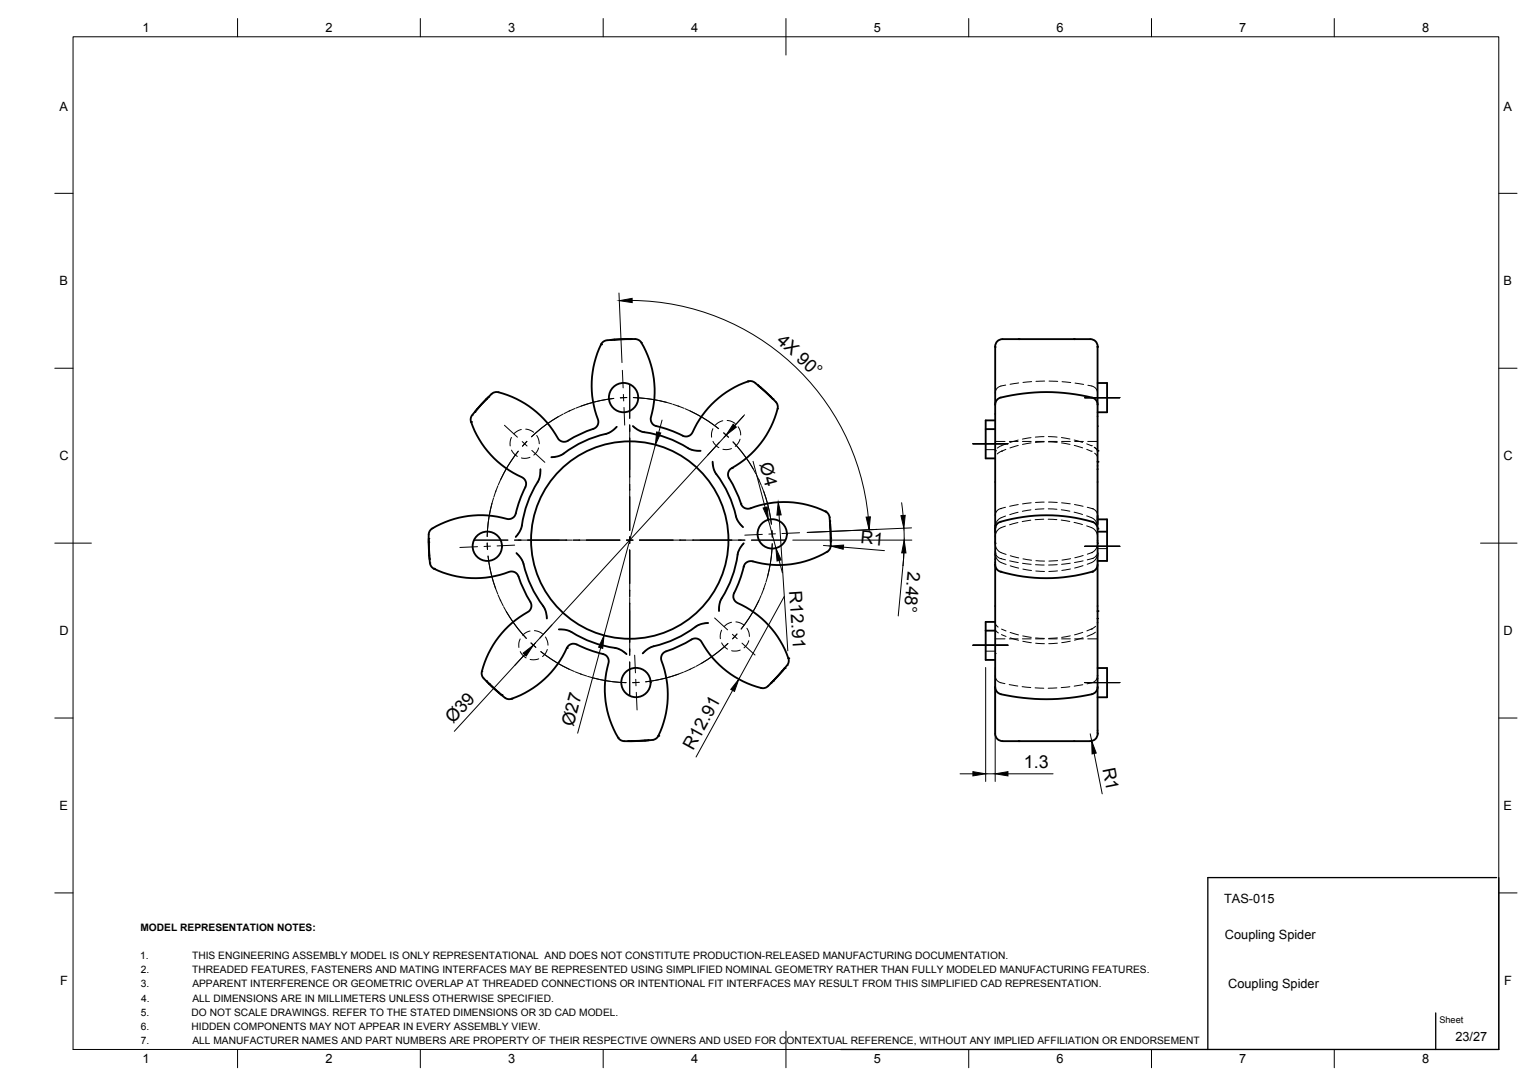
ISO-10303-21;
HEADER;
/* Generated by software containing ST-Developer
 * from STEP Tools, Inc. (www.steptools.com) 
 */

FILE_DESCRIPTION(
/* description */ ('STEP AP214'),
/* implementation_level */ '2;1');

FILE_NAME(
/* name */ 'Coupling Spider.step',
/* time_stamp */ '2026-11-15T14:49:54-08:00',
/* author */ (''),
/* organization */ (''),
/* preprocessor_version */ 'ST-DEVELOPER v20.2',
/* originating_system */ 'Autodesk Translation Framework v15.17.0.0',
/* authorisation */ '');

FILE_SCHEMA (('AUTOMOTIVE_DESIGN { 1 0 10303 214 3 1 1 }'));
ENDSEC;

DATA;
#10=MECHANICAL_DESIGN_GEOMETRIC_PRESENTATION_REPRESENTATION('',(#1115),#66721);
#11=B_SPLINE_SURFACE_WITH_KNOTS('',3,3,((#41982,#41983,#41984,#41985,#41986),
(#41987,#41988,#41989,#41990,#41991),(#41992,#41993,#41994,#41995,#41996),
(#41997,#41998,#41999,#42000,#42001),(#42002,#42003,#42004,#42005,#42006),
(#42007,#42008,#42009,#42010,#42011),(#42012,#42013,#42014,#42015,#42016)),
 .UNSPECIFIED.,.F.,.F.,.F.,(4,1,1,1,4),(4,1,4),(0.02704890409976,0.25,0.5,
0.75,0.9277040914243),(0.6266253876044,7.194455259721,13.76279800701),
 .UNSPECIFIED.);
#12=B_SPLINE_SURFACE_WITH_KNOTS('',3,3,((#43036,#43037,#43038,#43039,#43040),
(#43041,#43042,#43043,#43044,#43045),(#43046,#43047,#43048,#43049,#43050),
(#43051,#43052,#43053,#43054,#43055)),.UNSPECIFIED.,.F.,.F.,.F.,(4,4),(4,
1,4),(0.07560247213886,0.9246170074165),(0.97123707704753,7.194455259721,
13.4176757847934),.UNSPECIFIED.);
#13=B_SPLINE_SURFACE_WITH_KNOTS('',3,3,((#43854,#43855,#43856,#43857,#43858),
(#43859,#43860,#43861,#43862,#43863),(#43864,#43865,#43866,#43867,#43868),
(#43869,#43870,#43871,#43872,#43873),(#43874,#43875,#43876,#43877,#43878),
(#43879,#43880,#43881,#43882,#43883),(#43884,#43885,#43886,#43887,#43888)),
 .UNSPECIFIED.,.F.,.F.,.F.,(4,1,1,1,4),(4,1,4),(0.07229619653719,0.25,0.5,
0.75,0.9729510902578),(0.6266257504199,7.194455259721,13.76275812373),
 .UNSPECIFIED.);
#14=B_SPLINE_SURFACE_WITH_KNOTS('',3,3,((#44879,#44880,#44881,#44882,#44883),
(#44884,#44885,#44886,#44887,#44888),(#44889,#44890,#44891,#44892,#44893),
(#44894,#44895,#44896,#44897,#44898),(#44899,#44900,#44901,#44902,#44903),
(#44904,#44905,#44906,#44907,#44908),(#44909,#44910,#44911,#44912,#44913)),
 .UNSPECIFIED.,.F.,.F.,.F.,(4,1,1,1,4),(4,1,4),(0.02704960022791,0.25,0.5,
0.75,0.9276685882704),(0.6266253876465,7.194455259721,13.76279800699),
 .UNSPECIFIED.);
#15=B_SPLINE_SURFACE_WITH_KNOTS('',3,3,((#45852,#45853,#45854,#45855,#45856),
(#45857,#45858,#45859,#45860,#45861),(#45862,#45863,#45864,#45865,#45866),
(#45867,#45868,#45869,#45870,#45871)),.UNSPECIFIED.,.F.,.F.,.F.,(4,4),(4,
1,4),(0.07560247213886,0.9246170074164),(0.971237077045854,7.194455259721,
13.4176757847952),.UNSPECIFIED.);
#16=B_SPLINE_SURFACE_WITH_KNOTS('',3,3,((#46672,#46673,#46674,#46675,#46676),
(#46677,#46678,#46679,#46680,#46681),(#46682,#46683,#46684,#46685,#46686),
(#46687,#46688,#46689,#46690,#46691),(#46692,#46693,#46694,#46695,#46696),
(#46697,#46698,#46699,#46700,#46701),(#46702,#46703,#46704,#46705,#46706)),
 .UNSPECIFIED.,.F.,.F.,.F.,(4,1,1,1,4),(4,1,4),(0.07233141172687,0.25,0.5,
0.75,0.972950399776),(0.6266257504498,7.194455259721,13.76275812375),
 .UNSPECIFIED.);
#17=B_SPLINE_SURFACE_WITH_KNOTS('',3,3,((#47663,#47664,#47665,#47666,#47667),
(#47668,#47669,#47670,#47671,#47672),(#47673,#47674,#47675,#47676,#47677),
(#47678,#47679,#47680,#47681,#47682),(#47683,#47684,#47685,#47686,#47687),
(#47688,#47689,#47690,#47691,#47692),(#47693,#47694,#47695,#47696,#47697)),
 .UNSPECIFIED.,.F.,.F.,.F.,(4,1,1,1,4),(4,1,4),(0.02704894056375,0.25,0.5,
0.75,0.9277022317281),(0.6266253876037,7.194455259721,13.76279800701),
 .UNSPECIFIED.);
#18=B_SPLINE_SURFACE_WITH_KNOTS('',3,3,((#48705,#48706,#48707,#48708,#48709),
(#48710,#48711,#48712,#48713,#48714),(#48715,#48716,#48717,#48718,#48719),
(#48720,#48721,#48722,#48723,#48724)),.UNSPECIFIED.,.F.,.F.,.F.,(4,4),(4,
1,4),(0.07561105541477,0.9246169072522),(0.971199375698935,7.194455259721,
13.4177134902227),.UNSPECIFIED.);
#19=B_SPLINE_SURFACE_WITH_KNOTS('',3,3,((#49555,#49556,#49557,#49558,#49559),
(#49560,#49561,#49562,#49563,#49564),(#49565,#49566,#49567,#49568,#49569),
(#49570,#49571,#49572,#49573,#49574),(#49575,#49576,#49577,#49578,#49579),
(#49580,#49581,#49582,#49583,#49584),(#49585,#49586,#49587,#49588,#49589)),
 .UNSPECIFIED.,.F.,.F.,.F.,(4,1,1,1,4),(4,1,4),(0.07233141172959,0.25,0.5,
0.75,0.9729503997759),(0.6266257504616,7.194455259721,13.76275812376),
 .UNSPECIFIED.);
#20=B_SPLINE_SURFACE_WITH_KNOTS('',3,3,((#50503,#50504,#50505,#50506,#50507),
(#50508,#50509,#50510,#50511,#50512),(#50513,#50514,#50515,#50516,#50517),
(#50518,#50519,#50520,#50521,#50522),(#50523,#50524,#50525,#50526,#50527),
(#50528,#50529,#50530,#50531,#50532),(#50533,#50534,#50535,#50536,#50537)),
 .UNSPECIFIED.,.F.,.F.,.F.,(4,1,1,1,4),(4,1,4),(0.0270489040004,0.25,0.5,
0.75,0.9277040964915),(0.6266253875094,7.194455259721,13.76279800735),
 .UNSPECIFIED.);
#21=B_SPLINE_SURFACE_WITH_KNOTS('',3,3,((#51508,#51509,#51510,#51511,#51512),
(#51513,#51514,#51515,#51516,#51517),(#51518,#51519,#51520,#51521,#51522),
(#51523,#51524,#51525,#51526,#51527)),.UNSPECIFIED.,.F.,.F.,.F.,(4,4),(4,
1,4),(0.07561105541523,0.9246169072518),(0.971199375716696,7.194455259721,
13.4177134861273),.UNSPECIFIED.);
#22=B_SPLINE_SURFACE_WITH_KNOTS('',3,3,((#52356,#52357,#52358,#52359,#52360),
(#52361,#52362,#52363,#52364,#52365),(#52366,#52367,#52368,#52369,#52370),
(#52371,#52372,#52373,#52374,#52375),(#52376,#52377,#52378,#52379,#52380),
(#52381,#52382,#52383,#52384,#52385),(#52386,#52387,#52388,#52389,#52390)),
 .UNSPECIFIED.,.F.,.F.,.F.,(4,1,1,1,4),(4,1,4),(0.07229571648343,0.25,0.5,
0.75,0.9729510996705),(0.6266257503296,7.194455259721,13.76275812362),
 .UNSPECIFIED.);
#23=B_SPLINE_SURFACE_WITH_KNOTS('',3,3,((#53369,#53370,#53371,#53372,#53373),
(#53374,#53375,#53376,#53377,#53378),(#53379,#53380,#53381,#53382,#53383),
(#53384,#53385,#53386,#53387,#53388),(#53389,#53390,#53391,#53392,#53393),
(#53394,#53395,#53396,#53397,#53398),(#53399,#53400,#53401,#53402,#53403)),
 .UNSPECIFIED.,.F.,.F.,.F.,(4,1,1,1,4),(4,1,4),(0.02704960022791,0.25,0.5,
0.75,0.9276685882704),(0.6266253875523,7.194455259721,13.76279800732),
 .UNSPECIFIED.);
#24=B_SPLINE_SURFACE_WITH_KNOTS('',3,3,((#54369,#54370,#54371,#54372,#54373),
(#54374,#54375,#54376,#54377,#54378),(#54379,#54380,#54381,#54382,#54383),
(#54384,#54385,#54386,#54387,#54388)),.UNSPECIFIED.,.F.,.F.,.F.,(4,4),(4,
1,4),(0.07561112179917,0.9246168071327),(0.971161649229297,7.194455259721,
13.4177512126147),.UNSPECIFIED.);
#25=B_SPLINE_SURFACE_WITH_KNOTS('',3,3,((#55289,#55290,#55291,#55292,#55293),
(#55294,#55295,#55296,#55297,#55298),(#55299,#55300,#55301,#55302,#55303),
(#55304,#55305,#55306,#55307,#55308),(#55309,#55310,#55311,#55312,#55313),
(#55314,#55315,#55316,#55317,#55318),(#55319,#55320,#55321,#55322,#55323)),
 .UNSPECIFIED.,.F.,.F.,.F.,(4,1,1,1,4),(4,1,4),(0.07230494309637,0.25,0.5,
0.75,0.9729509187597),(0.626625750321,7.194455259721,13.76275812361),
 .UNSPECIFIED.);
#26=B_SPLINE_SURFACE_WITH_KNOTS('',3,3,((#56290,#56291,#56292,#56293,#56294),
(#56295,#56296,#56297,#56298,#56299),(#56300,#56301,#56302,#56303,#56304),
(#56305,#56306,#56307,#56308,#56309),(#56310,#56311,#56312,#56313,#56314),
(#56315,#56316,#56317,#56318,#56319),(#56320,#56321,#56322,#56323,#56324)),
 .UNSPECIFIED.,.F.,.F.,.F.,(4,1,1,1,4),(4,1,4),(0.02704894454492,0.25,0.5,
0.75,0.927702028685),(0.6266253875099,7.194455259721,13.76279800735),
 .UNSPECIFIED.);
#27=B_SPLINE_SURFACE_WITH_KNOTS('',3,3,((#57264,#57265,#57266,#57267,#57268),
(#57269,#57270,#57271,#57272,#57273),(#57274,#57275,#57276,#57277,#57278),
(#57279,#57280,#57281,#57282,#57283)),.UNSPECIFIED.,.F.,.F.,.F.,(4,4),(4,
1,4),(0.07561112179916,0.9246168071327),(0.971161649224581,7.194455259721,
13.4177512126194),.UNSPECIFIED.);
#28=B_SPLINE_SURFACE_WITH_KNOTS('',3,3,((#58109,#58110,#58111,#58112,#58113),
(#58114,#58115,#58116,#58117,#58118),(#58119,#58120,#58121,#58122,#58123),
(#58124,#58125,#58126,#58127,#58128),(#58129,#58130,#58131,#58132,#58133),
(#58134,#58135,#58136,#58137,#58138),(#58139,#58140,#58141,#58142,#58143)),
 .UNSPECIFIED.,.F.,.F.,.F.,(4,1,1,1,4),(4,1,4),(0.07233141172959,0.25,0.5,
0.75,0.9729503997759),(0.6266257503696,7.194455259721,13.76275812364),
 .UNSPECIFIED.);
#29=B_SPLINE_SURFACE_WITH_KNOTS('',3,3,((#58957,#58958,#58959,#58960,#58961),
(#58962,#58963,#58964,#58965,#58966),(#58967,#58968,#58969,#58970,#58971),
(#58972,#58973,#58974,#58975,#58976),(#58977,#58978,#58979,#58980,#58981),
(#58982,#58983,#58984,#58985,#58986),(#58987,#58988,#58989,#58990,#58991)),
 .UNSPECIFIED.,.F.,.F.,.F.,(4,1,1,1,4),(4,1,4),(0.02704893649799,0.25,0.5,
0.75,0.9277024390857),(0.6266253876044,7.194455259721,13.76279800701),
 .UNSPECIFIED.);
#30=B_SPLINE_SURFACE_WITH_KNOTS('',3,3,((#59443,#59444,#59445,#59446,#59447),
(#59448,#59449,#59450,#59451,#59452),(#59453,#59454,#59455,#59456,#59457),
(#59458,#59459,#59460,#59461,#59462)),.UNSPECIFIED.,.F.,.F.,.F.,(4,4),(4,
1,4),(0.07560233772369,0.9246171082587),(0.971274990731998,7.194455259721,
13.4176378711108),.UNSPECIFIED.);
#31=B_SPLINE_SURFACE_WITH_KNOTS('',3,3,((#60261,#60262,#60263,#60264,#60265),
(#60266,#60267,#60268,#60269,#60270),(#60271,#60272,#60273,#60274,#60275),
(#60276,#60277,#60278,#60279,#60280),(#60281,#60282,#60283,#60284,#60285),
(#60286,#60287,#60288,#60289,#60290),(#60291,#60292,#60293,#60294,#60295)),
 .UNSPECIFIED.,.F.,.F.,.F.,(4,1,1,1,4),(4,1,4),(0.07233141172722,0.25,0.5,
0.75,0.9729503997759),(0.6266257504058,7.194455259721,13.76275812373),
 .UNSPECIFIED.);
#32=B_SPLINE_SURFACE_WITH_KNOTS('',3,3,((#61841,#61842,#61843,#61844,#61845),
(#61846,#61847,#61848,#61849,#61850),(#61851,#61852,#61853,#61854,#61855),
(#61856,#61857,#61858,#61859,#61860),(#61861,#61862,#61863,#61864,#61865),
(#61866,#61867,#61868,#61869,#61870),(#61871,#61872,#61873,#61874,#61875)),
 .UNSPECIFIED.,.F.,.F.,.F.,(4,1,1,1,4),(4,1,4),(0.02704957693913,0.25,0.5,
0.75,0.9276697760189),(0.6266253874895,7.194455259721,13.76279800736),
 .UNSPECIFIED.);
#33=B_SPLINE_SURFACE_WITH_KNOTS('',3,3,((#62817,#62818,#62819,#62820,#62821),
(#62822,#62823,#62824,#62825,#62826),(#62827,#62828,#62829,#62830,#62831),
(#62832,#62833,#62834,#62835,#62836)),.UNSPECIFIED.,.F.,.F.,.F.,(4,4),(4,
1,4),(0.07561118765193,0.9246167076829),(0.971124132828661,7.194455259721,
13.4177887331011),.UNSPECIFIED.);
#34=B_SPLINE_SURFACE_WITH_KNOTS('',3,3,((#63659,#63660,#63661,#63662,#63663),
(#63664,#63665,#63666,#63667,#63668),(#63669,#63670,#63671,#63672,#63673),
(#63674,#63675,#63676,#63677,#63678),(#63679,#63680,#63681,#63682,#63683),
(#63684,#63685,#63686,#63687,#63688),(#63689,#63690,#63691,#63692,#63693)),
 .UNSPECIFIED.,.F.,.F.,.F.,(4,1,1,1,4),(4,1,4),(0.07233021543657,0.25,0.5,
0.75,0.9729504232322),(0.6266257503101,7.194455259721,13.7627581236),
 .UNSPECIFIED.);
#37=SPHERICAL_SURFACE('',#27729,1.000000122615);
#38=SPHERICAL_SURFACE('',#27733,1.000005019194);
#39=SPHERICAL_SURFACE('',#27736,1.000005006638);
#40=SPHERICAL_SURFACE('',#27742,1.000000000939);
#41=SPHERICAL_SURFACE('',#27750,1.000000122615);
#42=SPHERICAL_SURFACE('',#27755,1.000005019194);
#43=SPHERICAL_SURFACE('',#27758,1.000005006638);
#44=SPHERICAL_SURFACE('',#27764,1.000000000939);
#45=SPHERICAL_SURFACE('',#27772,1.000000122615);
#46=SPHERICAL_SURFACE('',#27776,1.000005019194);
#47=SPHERICAL_SURFACE('',#27779,1.000005006638);
#48=SPHERICAL_SURFACE('',#27785,1.000000000939);
#49=SPHERICAL_SURFACE('',#27794,1.000000122615);
#50=SPHERICAL_SURFACE('',#27798,1.0000050192);
#51=SPHERICAL_SURFACE('',#27802,1.000005006635);
#52=SPHERICAL_SURFACE('',#27808,1.000000000939);
#53=SPHERICAL_SURFACE('',#27816,1.000000122616);
#54=SPHERICAL_SURFACE('',#27821,1.0000050192);
#55=SPHERICAL_SURFACE('',#27824,1.000005006635);
#56=SPHERICAL_SURFACE('',#27830,1.000000000939);
#57=SPHERICAL_SURFACE('',#27837,1.000000122616);
#58=SPHERICAL_SURFACE('',#27841,1.0000050192);
#59=SPHERICAL_SURFACE('',#27845,1.000005006635);
#60=SPHERICAL_SURFACE('',#27851,1.000000000939);
#61=SPHERICAL_SURFACE('',#27857,1.000000122614);
#62=SPHERICAL_SURFACE('',#27865,1.00000000094);
#63=SPHERICAL_SURFACE('',#27870,1.000005006638);
#64=SPHERICAL_SURFACE('',#27874,1.000005019194);
#65=SPHERICAL_SURFACE('',#27882,1.000000122616);
#66=SPHERICAL_SURFACE('',#27887,1.0000050192);
#67=SPHERICAL_SURFACE('',#27890,1.000005006635);
#68=SPHERICAL_SURFACE('',#27896,1.000000000939);
#134=B_SPLINE_CURVE_WITH_KNOTS('',3,(#41289,#41290,#41291,#41292,#41293,
#41294,#41295,#41296,#41297,#41298,#41299,#41300,#41301,#41302,#41303,#41304,
#41305,#41306,#41307,#41308,#41309,#41310,#41311,#41312,#41313),
 .UNSPECIFIED.,.F.,.F.,(4,3,3,3,3,3,3,3,4),(9.24769724780462E-8,0.181995241036136,
0.253432963792377,0.436116740020438,0.5,0.680286934730948,0.806407517387765,
0.983702854489084,0.999931275933686),.UNSPECIFIED.);
#135=B_SPLINE_CURVE_WITH_KNOTS('',3,(#41315,#41316,#41317,#41318,#41319,
#41320,#41321,#41322),.UNSPECIFIED.,.F.,.F.,(4,2,2,4),(-0.00419299133317873,
0.,0.077185673586945,0.146698242999108),.UNSPECIFIED.);
#136=B_SPLINE_CURVE_WITH_KNOTS('',3,(#41323,#41324,#41325,#41326,#41327,
#41328,#41329,#41330,#41331,#41332,#41333,#41334,#41335,#41336,#41337,#41338,
#41339,#41340,#41341,#41342,#41343,#41344,#41345,#41346,#41347,#41348,#41349,
#41350,#41351,#41352,#41353,#41354,#41355,#41356,#41357,#41358,#41359,#41360,
#41361,#41362,#41363,#41364,#41365,#41366,#41367,#41368,#41369,#41370,#41371,
#41372,#41373,#41374,#41375,#41376,#41377,#41378,#41379,#41380),
 .UNSPECIFIED.,.F.,.F.,(4,3,3,3,3,3,3,3,3,3,3,3,3,3,3,3,3,3,3,4),(4.16556781324293E-6,
0.0545549619977905,0.125044525011968,0.198839838903777,0.203311262230742,
0.250000000000011,0.329872235461808,0.393021743570836,0.437500000000021,
0.468750000000022,0.484375000000022,0.492187500000022,0.498252272700136,
0.500000000000022,0.587854638271154,0.686590869203439,0.758727477162275,
0.861163120425338,0.935778689900579,0.999972466661225),.UNSPECIFIED.);
#137=B_SPLINE_CURVE_WITH_KNOTS('',3,(#41426,#41427,#41428,#41429,#41430,
#41431,#41432,#41433,#41434,#41435,#41436,#41437,#41438,#41439,#41440,#41441,
#41442,#41443,#41444,#41445,#41446,#41447,#41448,#41449,#41450,#41451,#41452,
#41453,#41454,#41455,#41456,#41457,#41458,#41459,#41460,#41461,#41462,#41463,
#41464,#41465,#41466,#41467,#41468,#41469,#41470,#41471,#41472,#41473,#41474,
#41475,#41476,#41477,#41478,#41479,#41480,#41481,#41482,#41483,#41484,#41485,
#41486,#41487,#41488,#41489,#41490,#41491,#41492,#41493,#41494,#41495,#41496,
#41497,#41498),.UNSPECIFIED.,.F.,.F.,(4,3,3,3,3,3,3,3,3,3,3,3,3,3,3,3,3,
3,3,3,3,3,3,3,4),(1.45421582652742E-9,0.0431191288977147,0.0863267801336832,
0.129382372680128,0.1428571428571,0.153643687206596,0.204633364771825,0.255730828842296,
0.2857142857143,0.306392920688462,0.370923133763148,0.4285714285714,0.459411527501898,
0.526892611023658,0.5714285714286,0.61248828595501,0.677675114413515,0.7142857142857,
0.765391735319569,0.819871243515933,0.8571428571429,0.900979351776543,0.918140216543459,
0.961789699495013,0.999999262769871),.UNSPECIFIED.);
#138=B_SPLINE_CURVE_WITH_KNOTS('',3,(#41501,#41502,#41503,#41504,#41505,
#41506,#41507,#41508,#41509,#41510,#41511,#41512,#41513,#41514,#41515,#41516,
#41517,#41518,#41519,#41520,#41521,#41522,#41523,#41524,#41525,#41526,#41527,
#41528,#41529,#41530,#41531,#41532,#41533,#41534,#41535,#41536,#41537,#41538,
#41539,#41540,#41541,#41542,#41543,#41544,#41545,#41546,#41547,#41548,#41549,
#41550,#41551,#41552,#41553,#41554,#41555,#41556,#41557,#41558,#41559,#41560,
#41561,#41562,#41563,#41564,#41565,#41566,#41567,#41568,#41569,#41570,#41571,
#41572,#41573),.UNSPECIFIED.,.F.,.F.,(4,3,3,3,3,3,3,3,3,3,3,3,3,3,3,3,3,
3,3,3,3,3,3,3,4),(0.,0.0558892508712823,0.112669232828285,0.156953133493156,
0.215051931585836,0.249999999999996,0.30931624195629,0.324310166689452,
0.385390344530509,0.437499999999994,0.468749999999994,0.484374999999995,
0.492187499999994,0.498949344576874,0.499999999999994,0.504582992163155,
0.573408026089892,0.641343139258655,0.680145622776148,0.749999999999997,
0.815926535907529,0.847891707736826,0.914669445287438,0.980716713244497,
1.),.UNSPECIFIED.);
#139=B_SPLINE_CURVE_WITH_KNOTS('',3,(#41672,#41673,#41674,#41675,#41676,
#41677,#41678,#41679,#41680,#41681,#41682,#41683,#41684,#41685,#41686,#41687,
#41688,#41689,#41690,#41691,#41692,#41693,#41694,#41695,#41696,#41697,#41698,
#41699,#41700,#41701,#41702,#41703,#41704,#41705,#41706,#41707,#41708,#41709,
#41710,#41711,#41712,#41713,#41714,#41715,#41716,#41717,#41718,#41719,#41720,
#41721,#41722,#41723,#41724,#41725,#41726,#41727,#41728,#41729,#41730,#41731,
#41732,#41733,#41734,#41735,#41736,#41737,#41738,#41739,#41740,#41741,#41742,
#41743,#41744,#41745,#41746,#41747,#41748,#41749,#41750,#41751,#41752,#41753,
#41754,#41755,#41756,#41757,#41758,#41759,#41760,#41761,#41762,#41763,#41764,
#41765,#41766,#41767,#41768,#41769,#41770,#41771,#41772,#41773,#41774,#41775,
#41776,#41777,#41778,#41779,#41780,#41781,#41782,#41783,#41784,#41785,#41786,
#41787,#41788,#41789,#41790,#41791,#41792,#41793,#41794,#41795,#41796,#41797,
#41798,#41799,#41800,#41801,#41802,#41803,#41804,#41805,#41806,#41807,#41808,
#41809,#41810,#41811,#41812,#41813,#41814,#41815,#41816,#41817,#41818,#41819,
#41820,#41821,#41822,#41823,#41824,#41825,#41826,#41827,#41828,#41829,#41830,
#41831,#41832,#41833,#41834,#41835,#41836,#41837),.UNSPECIFIED.,.F.,.F.,
(4,3,3,3,3,3,3,3,3,3,3,3,3,3,3,3,3,3,3,3,3,3,3,3,3,3,3,3,3,3,3,3,3,3,3,
3,3,3,3,3,3,3,3,3,3,3,3,3,3,3,3,3,3,3,3,4),(8.91960532295663E-8,0.0341912247086381,
0.0625000000000045,0.0800358633121934,0.0937500000000066,0.109375000000008,
0.117187500000008,0.121093750000008,0.123046875000008,0.125000000000009,
0.156917166494981,0.187500000000006,0.218750000000004,0.234375000000004,
0.237569461420448,0.242187500000003,0.246093750000003,0.248046875000003,
0.250000000000003,0.29085498421434,0.312500000000001,0.328958102746394,
0.343750000000001,0.359375,0.3671875,0.37109375,0.373046875,0.375,0.425233690755064,
0.437499999999999,0.468749999999999,0.484374999999998,0.492187499999998,
0.496093749999998,0.499999999999998,0.520148610503687,0.572572263765387,
0.616888106029241,0.624999999999998,0.651356261923537,0.678280550361872,
0.687499999999997,0.709145029414828,0.749999999999997,0.781249999999997,
0.789062499999997,0.796874999999997,0.799058374611912,0.812499999999997,
0.858403727307891,0.874999999999998,0.885484813980563,0.932677545234238,
0.980789386086282,0.985729992648815,1.),.UNSPECIFIED.);
#140=B_SPLINE_CURVE_WITH_KNOTS('',3,(#41840,#41841,#41842,#41843,#41844,
#41845,#41846,#41847,#41848,#41849,#41850,#41851,#41852,#41853,#41854,#41855,
#41856,#41857,#41858,#41859,#41860,#41861,#41862,#41863,#41864,#41865,#41866,
#41867,#41868,#41869,#41870,#41871,#41872,#41873,#41874,#41875,#41876,#41877,
#41878,#41879,#41880,#41881,#41882,#41883,#41884,#41885,#41886,#41887,#41888,
#41889,#41890,#41891,#41892,#41893,#41894,#41895,#41896,#41897,#41898,#41899,
#41900,#41901,#41902,#41903,#41904,#41905,#41906,#41907,#41908,#41909,#41910,
#41911,#41912,#41913,#41914,#41915,#41916,#41917,#41918,#41919,#41920,#41921,
#41922,#41923,#41924,#41925,#41926,#41927,#41928,#41929,#41930,#41931,#41932,
#41933,#41934,#41935,#41936,#41937,#41938,#41939,#41940,#41941,#41942,#41943,
#41944,#41945,#41946,#41947,#41948,#41949,#41950,#41951,#41952,#41953,#41954,
#41955,#41956,#41957,#41958,#41959,#41960,#41961,#41962,#41963,#41964,#41965,
#41966,#41967,#41968,#41969,#41970,#41971,#41972,#41973,#41974,#41975,#41976,
#41977,#41978,#41979,#41980,#41981),.UNSPECIFIED.,.F.,.F.,(4,3,3,3,3,3,
3,3,3,3,3,3,3,3,3,3,3,3,3,3,3,3,3,3,3,3,3,3,3,3,3,3,3,3,3,3,3,3,3,3,3,3,
3,3,3,3,3,4),(2.34638080134641E-7,0.0315958273278338,0.0628964684736565,
0.0937122522464384,0.104172084247666,0.125000000000001,0.15483717259373,
0.184674345187458,0.213175665860292,0.218750000000002,0.234375000000002,
0.242187500000002,0.246093750000002,0.248046875000002,0.250000000000002,
0.257790219373145,0.29564225982583,0.334483268009838,0.354335017264441,
0.392683323993403,0.431399052907306,0.470482126073725,0.482380370753286,
0.484375,0.496585862215116,0.5,0.540377620125422,0.580372331205939,0.609458164571178,
0.649168975008536,0.687499999999999,0.700833597540945,0.718749999999998,
0.734374999999998,0.742187499999998,0.746093749999998,0.748046874999998,
0.749999999999998,0.769092149884525,0.798967231624578,0.82884231336463,
0.858577220360793,0.874999999999999,0.896782429934653,0.927914366070493,
0.95958256675185,0.98564178257925,1.),.UNSPECIFIED.);
#141=B_SPLINE_CURVE_WITH_KNOTS('',3,(#42018,#42019,#42020,#42021,#42022,
#42023,#42024,#42025,#42026,#42027,#42028,#42029,#42030,#42031,#42032,#42033,
#42034,#42035,#42036,#42037,#42038,#42039,#42040,#42041,#42042,#42043,#42044,
#42045,#42046,#42047,#42048,#42049,#42050,#42051,#42052,#42053,#42054,#42055,
#42056,#42057,#42058,#42059,#42060,#42061,#42062,#42063,#42064,#42065,#42066,
#42067,#42068,#42069,#42070,#42071,#42072,#42073,#42074,#42075,#42076,#42077,
#42078),.UNSPECIFIED.,.F.,.F.,(4,3,3,3,3,3,3,3,3,3,3,3,3,3,3,3,3,3,3,3,
4),(3.81437103769371E-8,0.0594692300663259,0.119461345109324,0.180335245486518,
0.228233348289148,0.249999999999999,0.312499999999999,0.375,0.420629724919854,
0.466480844646722,0.5,0.532982688237145,0.595584389353294,0.657507323728288,
0.718468634500906,0.75,0.809830753855516,0.831293930438418,0.890887175430362,
0.949594406087391,1.),.UNSPECIFIED.);
#142=B_SPLINE_CURVE_WITH_KNOTS('',3,(#42079,#42080,#42081,#42082,#42083,
#42084,#42085,#42086,#42087,#42088,#42089,#42090,#42091,#42092,#42093,#42094,
#42095,#42096,#42097,#42098,#42099,#42100,#42101,#42102,#42103,#42104,#42105,
#42106,#42107,#42108,#42109,#42110,#42111,#42112,#42113,#42114,#42115,#42116,
#42117,#42118,#42119,#42120,#42121,#42122,#42123,#42124,#42125,#42126,#42127,
#42128,#42129,#42130,#42131,#42132,#42133,#42134,#42135,#42136),
 .UNSPECIFIED.,.F.,.F.,(4,3,3,3,3,3,3,3,3,3,3,3,3,3,3,3,3,3,3,4),(0.,0.0702349095256629,
0.13620442752083,0.197545800075418,0.25,0.30836677615071,0.365838196629605,
0.422901067133475,0.479527712569993,0.5,0.500089402413344,0.55569689606091,
0.61174830735272,0.66815419823378,0.725240325901832,0.75,0.8125,0.876775284237813,
0.947108494211004,1.),.UNSPECIFIED.);
#143=B_SPLINE_CURVE_WITH_KNOTS('',3,(#42182,#42183,#42184,#42185,#42186,
#42187,#42188,#42189,#42190,#42191,#42192,#42193,#42194,#42195,#42196,#42197,
#42198,#42199,#42200,#42201,#42202,#42203,#42204,#42205,#42206,#42207,#42208,
#42209,#42210,#42211,#42212,#42213,#42214,#42215,#42216,#42217,#42218,#42219,
#42220,#42221,#42222,#42223,#42224,#42225,#42226,#42227,#42228,#42229,#42230,
#42231,#42232,#42233,#42234,#42235,#42236,#42237,#42238,#42239),
 .UNSPECIFIED.,.F.,.F.,(4,3,3,3,3,3,3,3,3,3,3,3,3,3,3,3,3,3,3,4),(0.,0.0625,
0.123429278282135,0.183419387197853,0.242355422377173,0.25,0.30804097321092,
0.365338384048261,0.422299346255784,0.479067052552964,0.535783677854112,
0.592776690073264,0.649990216849972,0.707861099650818,0.75,0.80890331665661,
0.86915409584812,0.930297294952518,0.992906805699324,1.),.UNSPECIFIED.);
#144=B_SPLINE_CURVE_WITH_KNOTS('',3,(#42240,#42241,#42242,#42243,#42244,
#42245,#42246,#42247,#42248,#42249,#42250,#42251,#42252,#42253,#42254,#42255,
#42256,#42257,#42258,#42259,#42260,#42261,#42262,#42263,#42264,#42265,#42266,
#42267,#42268,#42269,#42270,#42271,#42272,#42273,#42274,#42275,#42276,#42277,
#42278,#42279,#42280,#42281,#42282,#42283,#42284,#42285,#42286,#42287,#42288,
#42289,#42290,#42291,#42292,#42293,#42294,#42295,#42296,#42297,#42298,#42299,
#42300,#42301,#42302,#42303,#42304,#42305,#42306,#42307,#42308,#42309,#42310,
#42311,#42312,#42313,#42314,#42315,#42316,#42317,#42318,#42319,#42320,#42321,
#42322,#42323,#42324,#42325,#42326,#42327,#42328,#42329,#42330,#42331,#42332,
#42333,#42334,#42335,#42336),.UNSPECIFIED.,.F.,.F.,(4,3,3,3,3,3,3,3,3,3,
3,3,3,3,3,3,3,3,3,3,3,3,3,3,3,3,3,3,3,3,3,3,4),(0.,0.00532220101307443,
0.0890067021312148,0.125000000000003,0.164995757695198,0.187500000000004,
0.218750000000005,0.234375000000005,0.242187500000005,0.246093750000005,
0.248046875000005,0.250000000000005,0.31582733556036,0.332758332189703,
0.397828850996205,0.462484106543816,0.499894434528747,0.500000000000007,
0.564413907449876,0.625000000000007,0.667038424876444,0.687500000000008,
0.718750000000008,0.734375000000008,0.742187500000008,0.746093750000008,
0.748046875000008,0.750000000000008,0.83044354525046,0.834793539095448,
0.91763781052554,0.994492135647195,1.),.UNSPECIFIED.);
#145=B_SPLINE_CURVE_WITH_KNOTS('',3,(#42379,#42380,#42381,#42382,#42383,
#42384,#42385,#42386,#42387,#42388,#42389,#42390,#42391,#42392,#42393,#42394,
#42395,#42396,#42397,#42398,#42399,#42400,#42401,#42402,#42403,#42404,#42405,
#42406,#42407,#42408,#42409),.UNSPECIFIED.,.F.,.F.,(4,3,3,3,3,3,3,3,3,3,
4),(0.,0.125,0.1875,0.218749999999999,0.234374999999999,0.2421875,0.250000000000002,
0.375000000000002,0.500000000000003,0.750000000000001,1.),.UNSPECIFIED.);
#146=B_SPLINE_CURVE_WITH_KNOTS('',3,(#42410,#42411,#42412,#42413,#42414,
#42415,#42416,#42417,#42418,#42419,#42420,#42421,#42422,#42423,#42424,#42425,
#42426,#42427,#42428,#42429,#42430,#42431,#42432,#42433,#42434),
 .UNSPECIFIED.,.F.,.F.,(4,3,3,3,3,3,3,3,4),(0.,0.177267179225085,0.212270675218487,
0.392511246506684,0.5,0.6825796579365,0.768811549889082,0.950690004118258,
0.999999216908986),.UNSPECIFIED.);
#147=B_SPLINE_CURVE_WITH_KNOTS('',3,(#42435,#42436,#42437,#42438,#42439,
#42440,#42441,#42442,#42443,#42444,#42445,#42446,#42447,#42448,#42449,#42450,
#42451,#42452,#42453,#42454,#42455,#42456,#42457,#42458,#42459,#42460,#42461,
#42462,#42463,#42464,#42465,#42466,#42467,#42468,#42469,#42470,#42471,#42472,
#42473,#42474,#42475,#42476,#42477,#42478,#42479,#42480,#42481,#42482,#42483,
#42484,#42485,#42486,#42487,#42488,#42489,#42490,#42491,#42492,#42493,#42494,
#42495),.UNSPECIFIED.,.F.,.F.,(4,3,3,3,3,3,3,3,3,3,3,3,3,3,3,3,3,3,3,3,
4),(1.62994004756316E-10,0.0701192575230677,0.172402183913519,0.247519373739165,
0.250000000000014,0.348340704489105,0.418430075331828,0.437500000000026,
0.468750000000027,0.484375000000028,0.492187500000028,0.497906193415308,
0.500000000000029,0.583530827624541,0.615517371368563,0.695249493382949,
0.750000000000014,0.803653832952724,0.877332170663887,0.95101050837505,
0.999999999995795),.UNSPECIFIED.);
#148=B_SPLINE_CURVE_WITH_KNOTS('',3,(#42538,#42539,#42540,#42541,#42542,
#42543,#42544,#42545,#42546,#42547,#42548,#42549,#42550,#42551,#42552,#42553,
#42554,#42555,#42556,#42557,#42558,#42559,#42560,#42561,#42562,#42563,#42564,
#42565,#42566,#42567,#42568,#42569,#42570,#42571,#42572,#42573,#42574,#42575,
#42576,#42577,#42578,#42579,#42580,#42581,#42582,#42583,#42584,#42585,#42586,
#42587,#42588,#42589,#42590,#42591,#42592,#42593,#42594,#42595,#42596,#42597,
#42598,#42599,#42600,#42601,#42602,#42603,#42604,#42605,#42606,#42607,#42608,
#42609,#42610,#42611,#42612,#42613,#42614,#42615,#42616,#42617,#42618,#42619,
#42620,#42621,#42622,#42623,#42624,#42625,#42626,#42627,#42628),
 .UNSPECIFIED.,.F.,.F.,(4,3,3,3,3,3,3,3,3,3,3,3,3,3,3,3,3,3,3,3,3,3,3,3,
3,3,3,3,3,3,4),(1.98871961878171E-7,0.0470903044064453,0.0950885766096769,
0.109526530581052,0.125000000000003,0.176685447285025,0.187500000000004,
0.195574875474865,0.203125000000005,0.218750000000006,0.250000000000007,
0.270621367580011,0.334103671117463,0.398264749549881,0.430414452825836,
0.437500000000011,0.468750000000012,0.484375000000012,0.492187500000012,
0.498034135032468,0.500000000000012,0.55992471255586,0.600124996024313,
0.65847531809809,0.715889408777046,0.764251055329571,0.821850438300925,
0.878616573497263,0.918179749391936,0.970963256196437,1.),.UNSPECIFIED.);
#149=B_SPLINE_CURVE_WITH_KNOTS('',3,(#42669,#42670,#42671,#42672,#42673,
#42674,#42675,#42676,#42677,#42678,#42679,#42680,#42681,#42682,#42683,#42684,
#42685,#42686,#42687,#42688,#42689,#42690,#42691,#42692,#42693,#42694,#42695,
#42696,#42697,#42698,#42699,#42700,#42701,#42702,#42703,#42704,#42705,#42706,
#42707,#42708,#42709,#42710,#42711,#42712,#42713,#42714,#42715,#42716,#42717,
#42718,#42719,#42720,#42721,#42722,#42723,#42724,#42725,#42726),
 .UNSPECIFIED.,.F.,.F.,(4,3,3,3,3,3,3,3,3,3,3,3,3,3,3,3,3,3,3,4),(0.,0.0625,
0.123439847866003,0.183439966319605,0.242385271483663,0.25,0.308039825256485,
0.365336094435668,0.422295901803994,0.47906242754066,0.535777838573044,
0.59276959415212,0.649981840047596,0.707851458465103,0.75,0.808901973781704,
0.869151463537593,0.930293405763861,0.992901748291823,1.),.UNSPECIFIED.);
#150=B_SPLINE_CURVE_WITH_KNOTS('',3,(#42728,#42729,#42730,#42731,#42732,
#42733,#42734,#42735,#42736,#42737,#42738,#42739,#42740,#42741,#42742,#42743,
#42744,#42745,#42746,#42747,#42748,#42749),.UNSPECIFIED.,.F.,.F.,(4,3,3,
3,3,3,3,4),(1.63034965610995E-6,0.120934083274333,0.310467041637166,0.5,
0.679851456363595,0.706412177213256,0.883436908989188,0.99999999999965),
 .UNSPECIFIED.);
#151=B_SPLINE_CURVE_WITH_KNOTS('',3,(#42751,#42752,#42753,#42754,#42755,
#42756,#42757,#42758,#42759,#42760,#42761),.UNSPECIFIED.,.F.,.F.,(4,1,2,
2,2,4),(0.,0.125000000000001,0.187500000000001,0.250000000000001,0.5,1.),
 .UNSPECIFIED.);
#152=B_SPLINE_CURVE_WITH_KNOTS('',3,(#42762,#42763,#42764,#42765,#42766,
#42767,#42768,#42769,#42770,#42771,#42772,#42773,#42774,#42775,#42776,#42777,
#42778,#42779,#42780,#42781,#42782,#42783,#42784,#42785,#42786,#42787,#42788,
#42789,#42790,#42791,#42792,#42793,#42794,#42795,#42796,#42797,#42798,#42799,
#42800,#42801,#42802,#42803,#42804,#42805,#42806,#42807,#42808,#42809,#42810,
#42811,#42812,#42813,#42814,#42815,#42816),.UNSPECIFIED.,.F.,.F.,(4,3,3,
3,3,3,3,3,3,3,3,3,3,3,3,3,3,3,4),(0.,0.0654579176760958,0.124936894080836,
0.195216251626205,0.250000000000005,0.306913806087027,0.375000000000006,
0.437500000000007,0.468750000000008,0.484375000000007,0.492187500000006,
0.498304645828867,0.500000000000006,0.531997326816961,0.633294552820071,
0.713452118082794,0.819819671501897,0.902138566641423,1.),.UNSPECIFIED.);
#153=B_SPLINE_CURVE_WITH_KNOTS('',3,(#42858,#42859,#42860,#42861,#42862,
#42863,#42864,#42865,#42866,#42867,#42868,#42869,#42870,#42871,#42872,#42873,
#42874,#42875,#42876,#42877,#42878,#42879,#42880,#42881,#42882,#42883,#42884,
#42885,#42886,#42887,#42888,#42889,#42890,#42891,#42892,#42893,#42894,#42895,
#42896,#42897,#42898,#42899,#42900,#42901,#42902,#42903,#42904,#42905,#42906,
#42907,#42908,#42909,#42910,#42911,#42912,#42913,#42914,#42915,#42916,#42917,
#42918,#42919,#42920,#42921,#42922,#42923,#42924,#42925,#42926,#42927,#42928,
#42929,#42930,#42931,#42932,#42933,#42934,#42935,#42936,#42937,#42938,#42939,
#42940,#42941,#42942,#42943,#42944,#42945),.UNSPECIFIED.,.F.,.F.,(4,3,3,
3,3,3,3,3,3,3,3,3,3,3,3,3,3,3,3,3,3,3,3,3,3,3,3,3,3,4),(1.06363783600673E-11,
0.0527820457982438,0.0818205403105205,0.13847230199092,0.195944376723133,
0.235749539973447,0.293011705111073,0.351192940284653,0.399875412946191,
0.437500000000032,0.468750000000034,0.484375000000035,0.492187500000036,
0.496093750000037,0.499508598162751,0.500000000000037,0.565860966296461,
0.629575210849187,0.693959314619374,0.725751295243402,0.78125000000002,
0.790730874186265,0.796875000000019,0.812500000000018,0.869043431531303,
0.875000000000012,0.884835807418444,0.938700912490986,0.993360836141555,
0.999999777750321),.UNSPECIFIED.);
#154=B_SPLINE_CURVE_WITH_KNOTS('',3,(#42948,#42949,#42950,#42951,#42952,
#42953,#42954,#42955,#42956,#42957,#42958,#42959,#42960,#42961,#42962,#42963,
#42964,#42965,#42966,#42967,#42968,#42969,#42970,#42971,#42972,#42973,#42974,
#42975,#42976,#42977,#42978,#42979,#42980,#42981,#42982,#42983,#42984,#42985,
#42986,#42987,#42988,#42989,#42990,#42991,#42992,#42993,#42994,#42995,#42996,
#42997,#42998,#42999,#43000,#43001,#43002,#43003,#43004,#43005),
 .UNSPECIFIED.,.F.,.F.,(4,3,3,3,3,3,3,3,3,3,3,3,3,3,3,3,3,3,3,4),(1.08539660247806E-11,
0.0585629649075452,0.117996402253644,0.168707850187142,0.228541404633181,
0.250000000000001,0.312500000000001,0.375,0.421054239194796,0.467108478389592,
0.5,0.563532901979659,0.626399534598786,0.688223254771881,0.75,0.771768828134012,
0.832605865340398,0.892881427639851,0.952306983535057,0.999999961863696),
 .UNSPECIFIED.);
#155=B_SPLINE_CURVE_WITH_KNOTS('',3,(#43056,#43057,#43058,#43059,#43060,
#43061,#43062,#43063,#43064,#43065,#43066,#43067,#43068,#43069,#43070,#43071,
#43072,#43073,#43074,#43075,#43076,#43077,#43078,#43079,#43080,#43081,#43082,
#43083,#43084,#43085,#43086,#43087,#43088,#43089,#43090,#43091,#43092,#43093,
#43094,#43095,#43096,#43097,#43098,#43099,#43100,#43101,#43102,#43103,#43104,
#43105,#43106,#43107,#43108,#43109,#43110,#43111,#43112,#43113,#43114,#43115,
#43116,#43117,#43118,#43119,#43120,#43121,#43122,#43123,#43124,#43125,#43126,
#43127,#43128,#43129,#43130,#43131,#43132,#43133,#43134,#43135,#43136,#43137,
#43138,#43139,#43140,#43141,#43142,#43143,#43144,#43145,#43146,#43147,#43148,
#43149,#43150,#43151,#43152,#43153,#43154,#43155,#43156,#43157,#43158,#43159,
#43160,#43161,#43162,#43163,#43164,#43165,#43166,#43167,#43168,#43169,#43170,
#43171,#43172,#43173,#43174,#43175,#43176,#43177,#43178,#43179,#43180,#43181,
#43182,#43183,#43184,#43185,#43186,#43187,#43188,#43189,#43190,#43191,#43192,
#43193,#43194,#43195,#43196,#43197,#43198,#43199,#43200,#43201,#43202,#43203,
#43204,#43205,#43206,#43207,#43208,#43209,#43210,#43211,#43212,#43213,#43214,
#43215,#43216,#43217,#43218,#43219,#43220,#43221,#43222,#43223,#43224,#43225,
#43226,#43227,#43228,#43229,#43230,#43231,#43232,#43233,#43234,#43235,#43236,
#43237,#43238,#43239,#43240,#43241,#43242,#43243,#43244,#43245,#43246,#43247,
#43248,#43249,#43250,#43251,#43252,#43253,#43254,#43255,#43256,#43257,#43258,
#43259,#43260,#43261,#43262,#43263,#43264,#43265,#43266,#43267,#43268,#43269),
 .UNSPECIFIED.,.F.,.F.,(4,3,3,3,3,3,3,3,3,3,3,3,3,3,3,3,3,3,3,3,3,3,3,3,
3,3,3,3,3,3,3,3,3,3,3,3,3,3,3,3,3,3,3,3,3,3,3,3,3,3,3,3,3,3,3,3,3,3,3,3,
3,3,3,3,3,3,3,3,3,3,3,4),(1.2412779566191E-7,0.0158915622078175,0.0300286939597752,
0.0432212519303281,0.0555779177000604,0.0624999999999985,0.0703124999999984,
0.0712890624999984,0.0722656249999983,0.0742187499999983,0.0781249999999982,
0.0928060999306038,0.0937499999999979,0.107515814939851,0.109374999999998,
0.117187499999998,0.121093749999997,0.123046874999997,0.124023437499998,
0.124999999999998,0.14566277553096,0.156249999999996,0.171874999999996,
0.179687499999995,0.186597992196647,0.187499999999995,0.218749999999993,
0.234374999999993,0.242187499999992,0.249023437499992,0.249999999999992,
0.273932641657877,0.297753405180433,0.312499999999987,0.336671055421645,
0.343749999999985,0.359374999999983,0.367187499999983,0.371093749999982,
0.373046874999982,0.374023437499982,0.374999999999982,0.40243511856254,
0.437499999999977,0.468749999999975,0.484374999999973,0.492187499999973,
0.496093749999972,0.498046874999972,0.499023437499972,0.499511718749972,
0.499999999999972,0.531460035353748,0.563796477714746,0.598894275607205,
0.624999999999975,0.661169639291458,0.687499999999976,0.712240746432469,
0.718749999999977,0.734374999999977,0.742187499999977,0.746093749999978,
0.748046874999978,0.749023437499978,0.749999999999978,0.795746766320124,
0.840593249693797,0.884608194904253,0.928337958215087,0.971865961827789,
1.),.UNSPECIFIED.);
#156=B_SPLINE_CURVE_WITH_KNOTS('',3,(#43352,#43353,#43354,#43355,#43356,
#43357,#43358,#43359,#43360,#43361,#43362,#43363,#43364,#43365,#43366,#43367,
#43368,#43369,#43370,#43371,#43372,#43373,#43374,#43375,#43376,#43377,#43378,
#43379,#43380,#43381,#43382,#43383,#43384,#43385,#43386,#43387,#43388,#43389,
#43390,#43391,#43392,#43393,#43394,#43395,#43396,#43397,#43398,#43399,#43400,
#43401,#43402,#43403,#43404,#43405,#43406,#43407,#43408,#43409,#43410,#43411,
#43412,#43413,#43414,#43415,#43416,#43417,#43418,#43419,#43420,#43421,#43422,
#43423,#43424,#43425,#43426,#43427,#43428,#43429,#43430,#43431,#43432,#43433,
#43434,#43435,#43436,#43437,#43438,#43439,#43440,#43441,#43442,#43443,#43444,
#43445,#43446,#43447,#43448,#43449,#43450,#43451,#43452,#43453,#43454,#43455,
#43456,#43457,#43458,#43459,#43460,#43461,#43462,#43463,#43464,#43465,#43466,
#43467,#43468,#43469,#43470,#43471,#43472,#43473,#43474,#43475,#43476,#43477,
#43478,#43479,#43480,#43481,#43482,#43483,#43484,#43485,#43486,#43487,#43488,
#43489,#43490,#43491,#43492,#43493,#43494,#43495,#43496,#43497,#43498,#43499,
#43500,#43501,#43502,#43503,#43504,#43505,#43506,#43507,#43508),
 .UNSPECIFIED.,.F.,.F.,(4,3,3,3,3,3,3,3,3,3,3,3,3,3,3,3,3,3,3,3,3,3,3,3,
3,3,3,3,3,3,3,3,3,3,3,3,3,3,3,3,3,3,3,3,3,3,3,3,3,3,3,3,4),(1.72726539323858E-7,
0.0434573072252328,0.0863338334529781,0.0932169511728678,0.125000000000006,
0.165840004054606,0.177273506760352,0.18750000000001,0.218750000000011,
0.234375000000012,0.242187500000012,0.246093750000012,0.249511718750012,
0.250000000000012,0.260113688380183,0.284905128547609,0.309602232522142,
0.312500000000013,0.33693232508302,0.343750000000013,0.359375000000013,
0.359741527395825,0.367187500000013,0.371093750000013,0.373046875000013,
0.374023437500013,0.375000000000013,0.427162056479387,0.437500000000012,
0.446539057397644,0.468750000000012,0.484375000000012,0.492187500000012,
0.499058238757587,0.500000000000012,0.529372232586504,0.59548856329429,
0.601624357332882,0.62500000000001,0.666786326506838,0.68750000000001,0.718750000000009,
0.726754195536815,0.734375000000009,0.746093750000009,0.750000000000009,
0.777564712781969,0.821930060067123,0.864143824382507,0.906141087264632,
0.949726024687935,0.995918324447688,0.999999956001254),.UNSPECIFIED.);
#157=B_SPLINE_CURVE_WITH_KNOTS('',3,(#43553,#43554,#43555,#43556,#43557,
#43558,#43559,#43560,#43561,#43562,#43563,#43564,#43565,#43566,#43567,#43568,
#43569,#43570,#43571,#43572,#43573,#43574,#43575,#43576,#43577,#43578,#43579,
#43580,#43581,#43582,#43583),.UNSPECIFIED.,.F.,.F.,(4,3,3,3,3,3,3,3,3,3,
4),(0.,0.125000000000005,0.187500000000009,0.21875000000001,0.234375000000012,
0.242187500000012,0.250000000000013,0.37500000000001,0.500000000000008,
0.750000000000004,1.),.UNSPECIFIED.);
#158=B_SPLINE_CURVE_WITH_KNOTS('',3,(#43585,#43586,#43587,#43588,#43589,
#43590,#43591,#43592,#43593,#43594,#43595,#43596,#43597,#43598,#43599,#43600,
#43601,#43602,#43603,#43604,#43605,#43606),.UNSPECIFIED.,.F.,.F.,(4,3,3,
3,3,3,3,4),(0.,0.177097286425541,0.275749261875936,0.455644460001368,0.5,
0.682208683855311,0.858274270782353,0.999997472804992),.UNSPECIFIED.);
#159=B_SPLINE_CURVE_WITH_KNOTS('',3,(#43609,#43610,#43611,#43612,#43613,
#43614,#43615,#43616,#43617,#43618,#43619,#43620,#43621,#43622,#43623,#43624,
#43625,#43626,#43627,#43628,#43629,#43630,#43631,#43632,#43633,#43634,#43635,
#43636,#43637,#43638,#43639,#43640,#43641,#43642,#43643,#43644,#43645,#43646,
#43647,#43648,#43649,#43650,#43651,#43652,#43653,#43654,#43655,#43656,#43657,
#43658,#43659,#43660,#43661,#43662,#43663,#43664,#43665,#43666,#43667,#43668,
#43669),.UNSPECIFIED.,.F.,.F.,(4,3,3,3,3,3,3,3,3,3,3,3,3,3,3,3,3,3,3,3,
4),(4.81164541590028E-11,0.0921587474837998,0.199886082229405,0.25000000000007,
0.280572618510311,0.383373795510249,0.437500000000123,0.46235563760934,
0.468750000000132,0.484375000000136,0.492187500000137,0.497992580687344,
0.500000000000139,0.58065428471115,0.656974692236562,0.686606290161625,
0.750000000000069,0.819755783565435,0.869885555531241,0.934942777765621,
1.),.UNSPECIFIED.);
#160=B_SPLINE_CURVE_WITH_KNOTS('',3,(#43714,#43715,#43716,#43717,#43718,
#43719,#43720,#43721,#43722,#43723,#43724,#43725,#43726,#43727,#43728,#43729,
#43730,#43731,#43732,#43733,#43734,#43735,#43736,#43737,#43738,#43739,#43740,
#43741,#43742,#43743,#43744,#43745,#43746,#43747,#43748,#43749,#43750,#43751,
#43752,#43753,#43754,#43755,#43756,#43757,#43758,#43759,#43760,#43761,#43762,
#43763,#43764,#43765,#43766,#43767,#43768,#43769,#43770,#43771,#43772,#43773,
#43774,#43775,#43776,#43777,#43778,#43779,#43780,#43781,#43782,#43783),
 .UNSPECIFIED.,.F.,.F.,(4,3,3,3,3,3,3,3,3,3,3,3,3,3,3,3,3,3,3,3,3,3,3,4),
(0.,0.0436825138500011,0.0764108556936313,0.12024489353654,0.125,0.179962631311872,
0.223835206461935,0.25,0.32005987930766,0.371520384359274,0.375,0.470560141195038,
0.5,0.519394716784299,0.625,0.667284314982272,0.741666952850946,0.75,0.808039667335501,
0.814941774796512,0.875,0.919746522907813,0.962448186336766,0.999999720265828),
 .UNSPECIFIED.);
#161=B_SPLINE_CURVE_WITH_KNOTS('',3,(#43784,#43785,#43786,#43787,#43788,
#43789,#43790,#43791,#43792,#43793,#43794,#43795,#43796,#43797,#43798,#43799,
#43800,#43801,#43802,#43803,#43804,#43805,#43806,#43807,#43808,#43809,#43810,
#43811,#43812,#43813,#43814,#43815,#43816,#43817,#43818,#43819,#43820,#43821,
#43822,#43823,#43824,#43825,#43826,#43827,#43828,#43829,#43830,#43831,#43832,
#43833,#43834,#43835,#43836,#43837,#43838,#43839,#43840,#43841,#43842,#43843,
#43844,#43845,#43846,#43847,#43848,#43849,#43850,#43851,#43852,#43853),
 .UNSPECIFIED.,.F.,.F.,(4,3,3,3,3,3,3,3,3,3,3,3,3,3,3,3,3,3,3,3,3,3,3,4),
(0.,0.0642449794749212,0.129222656061305,0.139648728602552,0.203363627428338,
0.249999999999998,0.300656431288555,0.369078215644276,0.437499999999997,
0.468749999999997,0.469711746121642,0.484374999999997,0.495155037334243,
0.499999999999997,0.563334769370525,0.625630857709008,0.644014771287496,
0.704246977442631,0.749999999999999,0.80787964620637,0.868482376177339,
0.928163403676397,0.961962296535731,0.99999999244352),.UNSPECIFIED.);
#162=B_SPLINE_CURVE_WITH_KNOTS('',3,(#43889,#43890,#43891,#43892,#43893,
#43894,#43895,#43896,#43897,#43898,#43899,#43900,#43901,#43902,#43903,#43904,
#43905,#43906,#43907,#43908,#43909,#43910,#43911,#43912,#43913,#43914,#43915,
#43916,#43917,#43918,#43919,#43920,#43921,#43922,#43923,#43924,#43925,#43926,
#43927,#43928,#43929,#43930,#43931,#43932,#43933,#43934,#43935,#43936,#43937,
#43938,#43939,#43940,#43941,#43942,#43943,#43944,#43945,#43946),
 .UNSPECIFIED.,.F.,.F.,(4,3,3,3,3,3,3,3,3,3,3,3,3,3,3,3,3,3,3,4),(4.71111344520772E-12,
0.0702702444833502,0.136263297817551,0.197619286303806,0.25,0.306673607267195,
0.362575654085062,0.418136880841742,0.473343199707359,0.5,0.500025791695673,
0.555648512148746,0.611709252031375,0.668121083567431,0.725208108345234,
0.75,0.8125,0.876728896060771,0.946991441238258,1.),.UNSPECIFIED.);
#163=B_SPLINE_CURVE_WITH_KNOTS('',3,(#43991,#43992,#43993,#43994,#43995,
#43996,#43997,#43998,#43999,#44000,#44001,#44002,#44003,#44004,#44005,#44006,
#44007,#44008,#44009,#44010,#44011,#44012,#44013,#44014,#44015,#44016,#44017,
#44018,#44019,#44020,#44021,#44022,#44023,#44024,#44025,#44026,#44027,#44028,
#44029,#44030,#44031,#44032,#44033,#44034,#44035,#44036,#44037,#44038,#44039,
#44040,#44041,#44042,#44043,#44044,#44045,#44046,#44047,#44048,#44049,#44050,
#44051,#44052,#44053,#44054,#44055,#44056,#44057,#44058,#44059,#44060,#44061,
#44062,#44063,#44064,#44065,#44066,#44067,#44068,#44069,#44070,#44071,#44072,
#44073,#44074,#44075,#44076,#44077,#44078,#44079,#44080,#44081,#44082,#44083,
#44084,#44085,#44086,#44087),.UNSPECIFIED.,.F.,.F.,(4,3,3,3,3,3,3,3,3,3,
3,3,3,3,3,3,3,3,3,3,3,3,3,3,3,3,3,3,3,3,3,3,4),(0.,0.00594665339781489,
0.0895009799070571,0.125,0.165331914099726,0.1875,0.218750000000001,0.234375000000001,
0.242187500000001,0.246093750000001,0.248046875000001,0.250000000000001,
0.316494860292734,0.33296054544575,0.39869139222638,0.463982918532056,0.499997299161403,
0.499999999999997,0.564240267140175,0.624999999999996,0.667039051318783,
0.687499999999995,0.718749999999995,0.734374999999994,0.742187499999994,
0.746093749999994,0.748046874999994,0.749999999999994,0.830398363043457,
0.834658925664481,0.917512726931569,0.994047937985235,1.),.UNSPECIFIED.);
#164=B_SPLINE_CURVE_WITH_KNOTS('',3,(#44130,#44131,#44132,#44133,#44134,
#44135,#44136,#44137,#44138,#44139,#44140,#44141,#44142,#44143,#44144,#44145,
#44146,#44147,#44148,#44149,#44150,#44151,#44152,#44153,#44154,#44155,#44156,
#44157,#44158,#44159,#44160,#44161,#44162,#44163,#44164,#44165,#44166,#44167,
#44168,#44169,#44170,#44171,#44172,#44173,#44174,#44175,#44176,#44177,#44178,
#44179,#44180,#44181,#44182,#44183,#44184,#44185,#44186,#44187),
 .UNSPECIFIED.,.F.,.F.,(4,3,3,3,3,3,3,3,3,3,3,3,3,3,3,3,3,3,3,4),(2.22959895026036E-11,
0.062500000016722,0.123437489174482,0.18343535644588,0.242378550489876,
0.25,0.308039612199808,0.365335670799369,0.422295269265173,0.47906158737644,
0.535776791619929,0.592768342853833,0.649980384318985,0.707849804328303,
0.75,0.808900802778059,0.869149031444851,0.930289647710724,0.99289660835092,
1.),.UNSPECIFIED.);
#165=B_SPLINE_CURVE_WITH_KNOTS('',3,(#44189,#44190,#44191,#44192,#44193,
#44194,#44195,#44196,#44197,#44198,#44199,#44200,#44201,#44202,#44203,#44204,
#44205,#44206,#44207,#44208,#44209,#44210),.UNSPECIFIED.,.F.,.F.,(4,3,3,
3,3,3,3,4),(1.50414810706118E-6,0.142631091283063,0.3248384812943,0.5,0.679893770870687,
0.7249391298164,0.902038302978679,1.),.UNSPECIFIED.);
#166=B_SPLINE_CURVE_WITH_KNOTS('',3,(#44212,#44213,#44214,#44215,#44216,
#44217,#44218,#44219,#44220,#44221,#44222),.UNSPECIFIED.,.F.,.F.,(4,1,2,
2,2,4),(0.,0.125000000000001,0.187500000000001,0.250000000000002,0.500000000000002,
1.),.UNSPECIFIED.);
#167=B_SPLINE_CURVE_WITH_KNOTS('',3,(#44223,#44224,#44225,#44226,#44227,
#44228,#44229,#44230,#44231,#44232,#44233,#44234,#44235,#44236,#44237,#44238,
#44239,#44240,#44241,#44242,#44243,#44244,#44245,#44246,#44247,#44248,#44249,
#44250,#44251,#44252,#44253,#44254,#44255,#44256,#44257,#44258,#44259,#44260,
#44261,#44262,#44263,#44264,#44265,#44266,#44267,#44268,#44269,#44270,#44271,
#44272,#44273,#44274,#44275,#44276,#44277),.UNSPECIFIED.,.F.,.F.,(4,3,3,
3,3,3,3,3,3,3,3,3,3,3,3,3,3,3,4),(0.,0.0650994509143261,0.130198901828652,
0.199793623724663,0.249999999999971,0.31347395756223,0.374999999999955,
0.437499999999947,0.468749999999944,0.484374999999942,0.492187499999943,
0.498312113079734,0.499999999999943,0.537870474179042,0.639813169747279,
0.719670993878168,0.826636066600404,0.908057815773878,0.999999999950719),
 .UNSPECIFIED.);
#168=B_SPLINE_CURVE_WITH_KNOTS('',3,(#44323,#44324,#44325,#44326,#44327,
#44328,#44329,#44330,#44331,#44332,#44333,#44334,#44335,#44336,#44337,#44338,
#44339,#44340,#44341,#44342,#44343,#44344,#44345,#44346,#44347,#44348,#44349,
#44350,#44351,#44352,#44353,#44354,#44355,#44356,#44357,#44358,#44359,#44360,
#44361,#44362,#44363,#44364,#44365,#44366,#44367,#44368,#44369,#44370,#44371,
#44372,#44373,#44374,#44375,#44376,#44377,#44378,#44379,#44380,#44381,#44382,
#44383,#44384,#44385,#44386,#44387,#44388,#44389,#44390,#44391,#44392,#44393,
#44394,#44395),.UNSPECIFIED.,.F.,.F.,(4,3,3,3,3,3,3,3,3,3,3,3,3,3,3,3,3,
3,3,3,3,3,3,3,4),(1.45412474122944E-9,0.0431191288920647,0.0863267801229386,
0.129382372664879,0.1428571428571,0.153643687206222,0.204633364768752,0.255730828837679,
0.2857142857143,0.30639292068803,0.370923133797652,0.4285714285714,0.459411527501627,
0.526892611231432,0.5714285714286,0.612488285952903,0.677675115314794,0.7142857142857,
0.765391735325212,0.819871244956775,0.8571428571429,0.900979355292703,0.918140216524895,
0.961789700094182,1.),.UNSPECIFIED.);
#169=B_SPLINE_CURVE_WITH_KNOTS('',3,(#44398,#44399,#44400,#44401,#44402,
#44403,#44404,#44405,#44406,#44407,#44408,#44409,#44410,#44411,#44412,#44413,
#44414,#44415,#44416,#44417,#44418,#44419,#44420,#44421,#44422,#44423,#44424,
#44425,#44426,#44427,#44428,#44429,#44430,#44431,#44432,#44433,#44434,#44435,
#44436,#44437,#44438,#44439,#44440,#44441,#44442,#44443,#44444,#44445,#44446,
#44447,#44448,#44449,#44450,#44451,#44452,#44453,#44454,#44455,#44456,#44457,
#44458,#44459,#44460,#44461,#44462,#44463,#44464,#44465,#44466,#44467,#44468,
#44469,#44470),.UNSPECIFIED.,.F.,.F.,(4,3,3,3,3,3,3,3,3,3,3,3,3,3,3,3,3,
3,3,3,3,3,3,3,4),(0.,0.0558892468671691,0.112669224393364,0.156953102315014,
0.215051895881817,0.249999999999986,0.309316236751042,0.32431009672252,
0.38539026908212,0.437499999999976,0.468749999999975,0.484374999999974,
0.492187499999974,0.49894938686157,0.499999999999974,0.504582882651568,
0.573407791512473,0.641342774132795,0.68014561739347,0.749999999999987,
0.815926296753662,0.847891736141458,0.914669262374538,0.980716193528038,
1.),.UNSPECIFIED.);
#170=B_SPLINE_CURVE_WITH_KNOTS('',3,(#44569,#44570,#44571,#44572,#44573,
#44574,#44575,#44576,#44577,#44578,#44579,#44580,#44581,#44582,#44583,#44584,
#44585,#44586,#44587,#44588,#44589,#44590,#44591,#44592,#44593,#44594,#44595,
#44596,#44597,#44598,#44599,#44600,#44601,#44602,#44603,#44604,#44605,#44606,
#44607,#44608,#44609,#44610,#44611,#44612,#44613,#44614,#44615,#44616,#44617,
#44618,#44619,#44620,#44621,#44622,#44623,#44624,#44625,#44626,#44627,#44628,
#44629,#44630,#44631,#44632,#44633,#44634,#44635,#44636,#44637,#44638,#44639,
#44640,#44641,#44642,#44643,#44644,#44645,#44646,#44647,#44648,#44649,#44650,
#44651,#44652,#44653,#44654,#44655,#44656,#44657,#44658,#44659,#44660,#44661,
#44662,#44663,#44664,#44665,#44666,#44667,#44668,#44669,#44670,#44671,#44672,
#44673,#44674,#44675,#44676,#44677,#44678,#44679,#44680,#44681,#44682,#44683,
#44684,#44685,#44686,#44687,#44688,#44689,#44690,#44691,#44692,#44693,#44694,
#44695,#44696,#44697,#44698,#44699,#44700,#44701,#44702,#44703,#44704,#44705,
#44706,#44707,#44708,#44709,#44710,#44711,#44712,#44713,#44714,#44715,#44716,
#44717,#44718,#44719,#44720,#44721,#44722,#44723,#44724,#44725,#44726,#44727,
#44728,#44729,#44730,#44731,#44732,#44733,#44734),.UNSPECIFIED.,.F.,.F.,
(4,3,3,3,3,3,3,3,3,3,3,3,3,3,3,3,3,3,3,3,3,3,3,3,3,3,3,3,3,3,3,3,3,3,3,
3,3,3,3,3,3,3,3,3,3,3,3,3,3,3,3,3,3,3,3,4),(8.91959169339166E-8,0.034191224757925,
0.0624999999999919,0.0800358633020966,0.0937499999999878,0.109374999999986,
0.117187499999985,0.121093749999984,0.123046874999984,0.124999999999984,
0.15691716645829,0.187499999999983,0.218749999999983,0.234374999999983,
0.2375694614058,0.242187499999983,0.246093749999983,0.248046874999983,0.249999999999983,
0.290854984415917,0.312499999999984,0.328958102706763,0.343749999999985,
0.359374999999985,0.367187499999986,0.371093749999986,0.373046874999986,
0.374999999999986,0.425233690794145,0.437499999999987,0.468749999999988,
0.484374999999988,0.492187499999988,0.496093749999988,0.499999999999989,
0.520148610554065,0.572572264461685,0.616888106095276,0.624999999999991,
0.651356262019081,0.678280550572746,0.687499999999993,0.709145029379915,
0.749999999999994,0.781249999999995,0.789062499999995,0.796874999999995,
0.799058374602463,0.812499999999995,0.858403727209328,0.874999999999997,
0.885484813929701,0.932677545181923,0.980789386022011,0.985729992633788,
1.),.UNSPECIFIED.);
#171=B_SPLINE_CURVE_WITH_KNOTS('',3,(#44737,#44738,#44739,#44740,#44741,
#44742,#44743,#44744,#44745,#44746,#44747,#44748,#44749,#44750,#44751,#44752,
#44753,#44754,#44755,#44756,#44757,#44758,#44759,#44760,#44761,#44762,#44763,
#44764,#44765,#44766,#44767,#44768,#44769,#44770,#44771,#44772,#44773,#44774,
#44775,#44776,#44777,#44778,#44779,#44780,#44781,#44782,#44783,#44784,#44785,
#44786,#44787,#44788,#44789,#44790,#44791,#44792,#44793,#44794,#44795,#44796,
#44797,#44798,#44799,#44800,#44801,#44802,#44803,#44804,#44805,#44806,#44807,
#44808,#44809,#44810,#44811,#44812,#44813,#44814,#44815,#44816,#44817,#44818,
#44819,#44820,#44821,#44822,#44823,#44824,#44825,#44826,#44827,#44828,#44829,
#44830,#44831,#44832,#44833,#44834,#44835,#44836,#44837,#44838,#44839,#44840,
#44841,#44842,#44843,#44844,#44845,#44846,#44847,#44848,#44849,#44850,#44851,
#44852,#44853,#44854,#44855,#44856,#44857,#44858,#44859,#44860,#44861,#44862,
#44863,#44864,#44865,#44866,#44867,#44868,#44869,#44870,#44871,#44872,#44873,
#44874,#44875,#44876,#44877,#44878),.UNSPECIFIED.,.F.,.F.,(4,3,3,3,3,3,
3,3,3,3,3,3,3,3,3,3,3,3,3,3,3,3,3,3,3,3,3,3,3,3,3,3,3,3,3,3,3,3,3,3,3,3,
3,3,3,3,3,4),(2.34637977869052E-7,0.0315958280909132,0.0628964699770943,
0.0937122544741528,0.104172082727763,0.124999999999996,0.154837172127899,
0.184674344255801,0.213175665615131,0.218749999999993,0.234374999999993,
0.242187499999993,0.246093749999993,0.248046874999992,0.249999999999992,
0.257790219441197,0.295642260513954,0.33448326935675,0.35433501791698,0.392683325318844,
0.431399054924811,0.47048212880613,0.482380370998591,0.484374999999998,
0.496585862827081,0.499999999999998,0.540377620589275,0.580372332112356,
0.609458164164579,0.649168974998843,0.687500000000002,0.700833597323562,
0.718750000000003,0.734375000000003,0.742187500000004,0.746093750000004,
0.748046875000004,0.750000000000004,0.769092149904531,0.798967231669278,
0.828842313434025,0.858577220457806,0.875000000000002,0.896782430031144,
0.927914366240707,0.959582566990659,0.985641782611402,1.),.UNSPECIFIED.);
#172=B_SPLINE_CURVE_WITH_KNOTS('',3,(#44915,#44916,#44917,#44918,#44919,
#44920,#44921,#44922,#44923,#44924,#44925,#44926,#44927,#44928,#44929,#44930,
#44931,#44932,#44933,#44934,#44935,#44936,#44937,#44938,#44939,#44940,#44941,
#44942,#44943,#44944,#44945,#44946,#44947,#44948,#44949,#44950,#44951,#44952,
#44953,#44954,#44955,#44956,#44957,#44958,#44959,#44960,#44961,#44962,#44963,
#44964,#44965,#44966,#44967,#44968,#44969,#44970,#44971,#44972,#44973,#44974,
#44975),.UNSPECIFIED.,.F.,.F.,(4,3,3,3,3,3,3,3,3,3,3,3,3,3,3,3,3,3,3,3,
4),(3.81436882533441E-8,0.0594692292641814,0.119461343227841,0.180335241910882,
0.228233302192543,0.25,0.3125,0.375,0.420627292107485,0.46647604053592,
0.499999999999999,0.532982596178094,0.595584220707157,0.657507075875902,
0.718468302664308,0.75,0.809830575581488,0.831293958244676,0.890887062348566,
0.949594080453884,1.),.UNSPECIFIED.);
#173=B_SPLINE_CURVE_WITH_KNOTS('',3,(#44976,#44977,#44978,#44979,#44980,
#44981,#44982,#44983,#44984,#44985,#44986,#44987,#44988,#44989,#44990,#44991,
#44992,#44993,#44994,#44995,#44996,#44997,#44998,#44999,#45000,#45001,#45002,
#45003,#45004,#45005,#45006,#45007,#45008,#45009,#45010,#45011,#45012,#45013,
#45014,#45015,#45016,#45017,#45018,#45019,#45020,#45021,#45022,#45023,#45024,
#45025,#45026,#45027,#45028,#45029,#45030,#45031,#45032,#45033),
 .UNSPECIFIED.,.F.,.F.,(4,3,3,3,3,3,3,3,3,3,3,3,3,3,3,3,3,3,3,4),(0.,0.0707847140878596,
0.137148906725362,0.198769341270042,0.25,0.307617645699735,0.364360102685869,
0.4207050229385,0.476620929621341,0.499999807619985,0.5,0.555639372550431,
0.61176570697656,0.668272077500309,0.725497591406648,0.75,0.8125,0.877170019129078,
0.948088467729899,1.),.UNSPECIFIED.);
#174=B_SPLINE_CURVE_WITH_KNOTS('',3,(#45072,#45073,#45074,#45075,#45076,
#45077,#45078,#45079,#45080,#45081,#45082,#45083,#45084,#45085,#45086,#45087,
#45088,#45089,#45090,#45091,#45092,#45093,#45094,#45095,#45096,#45097,#45098,
#45099,#45100,#45101,#45102,#45103,#45104,#45105,#45106,#45107,#45108,#45109,
#45110,#45111,#45112,#45113,#45114,#45115,#45116,#45117,#45118,#45119,#45120,
#45121,#45122,#45123,#45124,#45125,#45126,#45127,#45128,#45129,#45130,#45131,
#45132,#45133,#45134,#45135,#45136,#45137,#45138,#45139,#45140,#45141,#45142,
#45143,#45144,#45145,#45146,#45147,#45148,#45149,#45150,#45151,#45152,#45153),
 .UNSPECIFIED.,.F.,.F.,(4,3,3,3,3,3,3,3,3,3,3,3,3,3,3,3,3,3,3,3,3,3,3,3,
3,3,3,4),(0.,0.0730383845014315,0.124999999999999,0.126434974013761,0.187499999999999,
0.218749999999999,0.234374999999999,0.242187499999999,0.248228963404092,
0.249999999999999,0.312644125642674,0.385286363662978,0.457286745548691,
0.499988468763114,0.499999999999998,0.570610476397242,0.624999999999998,
0.687338261753051,0.687499999999998,0.718749999999998,0.734374999999998,
0.742187499999998,0.748270407592068,0.749999999999998,0.819257343725233,
0.873533773999793,0.945731297648729,1.),.UNSPECIFIED.);
#175=B_SPLINE_CURVE_WITH_KNOTS('',3,(#45192,#45193,#45194,#45195,#45196,
#45197,#45198,#45199,#45200,#45201,#45202,#45203,#45204,#45205,#45206,#45207,
#45208,#45209,#45210,#45211,#45212,#45213,#45214,#45215,#45216,#45217,#45218,
#45219,#45220,#45221,#45222),.UNSPECIFIED.,.F.,.F.,(4,3,3,3,3,3,3,3,3,3,
4),(0.,0.125000000000001,0.187500000000002,0.218750000000002,0.234375000000002,
0.242187500000002,0.250000000000001,0.375000000000001,0.5,0.75,1.),
 .UNSPECIFIED.);
#176=B_SPLINE_CURVE_WITH_KNOTS('',3,(#45223,#45224,#45225,#45226,#45227,
#45228,#45229,#45230,#45231,#45232,#45233,#45234,#45235,#45236,#45237,#45238,
#45239,#45240,#45241,#45242,#45243,#45244),.UNSPECIFIED.,.F.,.F.,(4,3,3,
3,3,3,3,4),(4.84241338254634E-12,0.177024513735652,0.292989133330021,0.472837100420863,
0.5,0.689142380603627,0.878284761207255,0.999997308141097),
 .UNSPECIFIED.);
#177=B_SPLINE_CURVE_WITH_KNOTS('',3,(#45245,#45246,#45247,#45248,#45249,
#45250,#45251,#45252,#45253,#45254,#45255,#45256,#45257,#45258,#45259,#45260,
#45261,#45262,#45263,#45264,#45265,#45266,#45267,#45268,#45269,#45270,#45271,
#45272,#45273,#45274,#45275,#45276,#45277,#45278,#45279,#45280,#45281,#45282,
#45283,#45284,#45285,#45286,#45287,#45288,#45289,#45290,#45291,#45292,#45293,
#45294,#45295,#45296,#45297,#45298,#45299,#45300,#45301,#45302,#45303,#45304,
#45305),.UNSPECIFIED.,.F.,.F.,(4,3,3,3,3,3,3,3,3,3,3,3,3,3,3,3,3,3,3,3,
4),(0.,0.0976856411360946,0.205020683798958,0.250000000000005,0.286357315729757,
0.375000000000006,0.437500000000007,0.467815787221745,0.468750000000008,
0.484375000000009,0.49218750000001,0.497983320418243,0.500000000000011,
0.581183162052572,0.657948135236424,0.692880007830916,0.750000000000006,
0.820238740720444,0.874892108161841,0.940309020316848,0.999999999888383),
 .UNSPECIFIED.);
#178=B_SPLINE_CURVE_WITH_KNOTS('',3,(#45348,#45349,#45350,#45351,#45352,
#45353,#45354,#45355,#45356,#45357,#45358,#45359,#45360,#45361,#45362,#45363,
#45364,#45365,#45366,#45367,#45368,#45369,#45370,#45371,#45372,#45373,#45374,
#45375,#45376,#45377,#45378,#45379,#45380,#45381,#45382,#45383,#45384,#45385,
#45386,#45387,#45388,#45389,#45390,#45391,#45392,#45393,#45394,#45395,#45396,
#45397,#45398,#45399,#45400,#45401,#45402,#45403,#45404,#45405,#45406,#45407,
#45408,#45409,#45410,#45411,#45412,#45413,#45414,#45415,#45416,#45417,#45418,
#45419,#45420,#45421,#45422,#45423,#45424,#45425,#45426,#45427,#45428,#45429,
#45430,#45431,#45432,#45433,#45434,#45435,#45436,#45437,#45438),
 .UNSPECIFIED.,.F.,.F.,(4,3,3,3,3,3,3,3,3,3,3,3,3,3,3,3,3,3,3,3,3,3,3,3,
3,3,3,3,3,3,4),(1.98906711270074E-7,0.0470898341245432,0.0950876494948429,
0.1095264169096,0.125000000000007,0.176684966067105,0.187500000000011,0.195574834408008,
0.203125000000011,0.218750000000012,0.250000000000014,0.27062137095328,
0.33410369741832,0.398264798166895,0.430414456184177,0.437500000000022,
0.468750000000023,0.484375000000023,0.492187500000023,0.498034134485692,
0.500000000000023,0.55992471700438,0.600124993316173,0.658475320026033,
0.715889417182772,0.764251050351263,0.821850438516385,0.878616579115469,
0.918179745628572,0.970963257604969,1.),.UNSPECIFIED.);
#179=B_SPLINE_CURVE_WITH_KNOTS('',3,(#45479,#45480,#45481,#45482,#45483,
#45484,#45485,#45486,#45487,#45488,#45489,#45490,#45491,#45492,#45493,#45494,
#45495,#45496,#45497,#45498,#45499,#45500,#45501,#45502,#45503,#45504,#45505,
#45506,#45507,#45508,#45509,#45510,#45511,#45512,#45513,#45514,#45515,#45516,
#45517,#45518,#45519,#45520,#45521,#45522,#45523,#45524,#45525,#45526,#45527,
#45528,#45529,#45530,#45531,#45532,#45533,#45534,#45535,#45536),
 .UNSPECIFIED.,.F.,.F.,(4,3,3,3,3,3,3,3,3,3,3,3,3,3,3,3,3,3,3,4),(0.,0.0625,
0.123439752661815,0.183439781150676,0.24238500236667,0.25,0.308039822981183,
0.365336089933782,0.422295895259794,0.479062419223563,0.535777828796871,
0.592769583389136,0.649981828485573,0.707851446289196,0.75,0.808901159247775,
0.869149758611648,0.930290761113668,0.992898128268879,0.999999999982197),
 .UNSPECIFIED.);
#180=B_SPLINE_CURVE_WITH_KNOTS('',3,(#45538,#45539,#45540,#45541,#45542,
#45543,#45544,#45545,#45546,#45547,#45548,#45549,#45550,#45551,#45552,#45553,
#45554,#45555,#45556,#45557,#45558,#45559,#45560,#45561,#45562),
 .UNSPECIFIED.,.F.,.F.,(4,3,3,3,3,3,3,3,4),(4.25096523957949E-6,0.113054396572424,
0.286551692876521,0.3333333333333,0.588518474908942,0.6666666666667,0.699795484080798,
0.8687115644679,1.),.UNSPECIFIED.);
#181=B_SPLINE_CURVE_WITH_KNOTS('',3,(#45564,#45565,#45566,#45567,#45568,
#45569,#45570,#45571),.UNSPECIFIED.,.F.,.F.,(4,2,2,4),(-0.13616939866078,
-0.132213942079058,-0.0631200687627756,-1.0304878651527E-6),
 .UNSPECIFIED.);
#182=B_SPLINE_CURVE_WITH_KNOTS('',3,(#45572,#45573,#45574,#45575,#45576,
#45577,#45578,#45579,#45580,#45581,#45582,#45583,#45584,#45585,#45586,#45587,
#45588,#45589,#45590,#45591,#45592,#45593,#45594,#45595,#45596,#45597,#45598,
#45599,#45600,#45601,#45602,#45603,#45604,#45605,#45606,#45607,#45608,#45609,
#45610,#45611,#45612,#45613,#45614,#45615,#45616,#45617,#45618,#45619,#45620,
#45621,#45622,#45623,#45624,#45625,#45626,#45627,#45628,#45629,#45630,#45631,
#45632),.UNSPECIFIED.,.F.,.F.,(4,3,3,3,3,3,3,3,3,3,3,3,3,3,3,3,3,3,3,3,
4),(0.,0.0668222533452538,0.087636582994685,0.15721165197603,0.23020818876474,
0.25000000000003,0.275402007440453,0.35162875929872,0.431503649816666,0.437500000000052,
0.468750000000056,0.484375000000057,0.492187500000057,0.49890918886054,
0.500000000000057,0.504259889031405,0.612227588888961,0.697520590118762,
0.811484576508768,0.895767648762923,1.),.UNSPECIFIED.);
#183=B_SPLINE_CURVE_WITH_KNOTS('',3,(#45674,#45675,#45676,#45677,#45678,
#45679,#45680,#45681,#45682,#45683,#45684,#45685,#45686,#45687,#45688,#45689,
#45690,#45691,#45692,#45693,#45694,#45695,#45696,#45697,#45698,#45699,#45700,
#45701,#45702,#45703,#45704,#45705,#45706,#45707,#45708,#45709,#45710,#45711,
#45712,#45713,#45714,#45715,#45716,#45717,#45718,#45719,#45720,#45721,#45722,
#45723,#45724,#45725,#45726,#45727,#45728,#45729,#45730,#45731,#45732,#45733,
#45734,#45735,#45736,#45737,#45738,#45739,#45740,#45741,#45742,#45743,#45744,
#45745,#45746,#45747,#45748,#45749,#45750,#45751,#45752,#45753,#45754,#45755,
#45756,#45757,#45758,#45759,#45760,#45761),.UNSPECIFIED.,.F.,.F.,(4,3,3,
3,3,3,3,3,3,3,3,3,3,3,3,3,3,3,3,3,3,3,3,3,3,3,3,3,3,4),(0.,0.0527820478293045,
0.0818205404607765,0.138472304327033,0.195944381325339,0.235749541322639,
0.293011700541857,0.351192937824961,0.399875414183099,0.437499999999972,
0.46874999999997,0.484374999999969,0.492187499999969,0.496093749999968,
0.499508598312834,0.499999999999968,0.565860967008055,0.629575216253443,
0.693959324596289,0.725751295992003,0.781249999999986,0.790730946880879,
0.796874999999988,0.812499999999989,0.869044149651082,0.874999999999992,
0.884835922785512,0.938701683102266,0.993362240378366,0.999999777713918),
 .UNSPECIFIED.);
#184=B_SPLINE_CURVE_WITH_KNOTS('',3,(#45764,#45765,#45766,#45767,#45768,
#45769,#45770,#45771,#45772,#45773,#45774,#45775,#45776,#45777,#45778,#45779,
#45780,#45781,#45782,#45783,#45784,#45785,#45786,#45787,#45788,#45789,#45790,
#45791,#45792,#45793,#45794,#45795,#45796,#45797,#45798,#45799,#45800,#45801,
#45802,#45803,#45804,#45805,#45806,#45807,#45808,#45809,#45810,#45811,#45812,
#45813,#45814,#45815,#45816,#45817,#45818,#45819,#45820,#45821),
 .UNSPECIFIED.,.F.,.F.,(4,3,3,3,3,3,3,3,3,3,3,3,3,3,3,3,3,3,3,4),(1.54018677598839E-11,
0.0585628929030956,0.117996269618339,0.168707840865122,0.228541332439228,
0.25,0.3125,0.375,0.421054279485964,0.467108558971928,0.5,0.563532900722117,
0.626399532373606,0.688223252003269,0.75,0.771768860363025,0.832605896968812,
0.892881458907284,0.952307014882936,0.999999961863681),.UNSPECIFIED.);
#185=B_SPLINE_CURVE_WITH_KNOTS('',3,(#45872,#45873,#45874,#45875,#45876,
#45877,#45878,#45879,#45880,#45881,#45882,#45883,#45884,#45885,#45886,#45887,
#45888,#45889,#45890,#45891,#45892,#45893,#45894,#45895,#45896,#45897,#45898,
#45899,#45900,#45901,#45902,#45903,#45904,#45905,#45906,#45907,#45908,#45909,
#45910,#45911,#45912,#45913,#45914,#45915,#45916,#45917,#45918,#45919,#45920,
#45921,#45922,#45923,#45924,#45925,#45926,#45927,#45928,#45929,#45930,#45931,
#45932,#45933,#45934,#45935,#45936,#45937,#45938,#45939,#45940,#45941,#45942,
#45943,#45944,#45945,#45946,#45947,#45948,#45949,#45950,#45951,#45952,#45953,
#45954,#45955,#45956,#45957,#45958,#45959,#45960,#45961,#45962,#45963,#45964,
#45965,#45966,#45967,#45968,#45969,#45970,#45971,#45972,#45973,#45974,#45975,
#45976,#45977,#45978,#45979,#45980,#45981,#45982,#45983,#45984,#45985,#45986,
#45987,#45988,#45989,#45990,#45991,#45992,#45993,#45994,#45995,#45996,#45997,
#45998,#45999,#46000,#46001,#46002,#46003,#46004,#46005,#46006,#46007,#46008,
#46009,#46010,#46011,#46012,#46013,#46014,#46015,#46016,#46017,#46018,#46019,
#46020,#46021,#46022,#46023,#46024,#46025,#46026,#46027,#46028,#46029,#46030,
#46031,#46032,#46033,#46034,#46035,#46036,#46037,#46038,#46039,#46040,#46041,
#46042,#46043,#46044,#46045,#46046,#46047,#46048,#46049,#46050,#46051,#46052,
#46053,#46054,#46055,#46056,#46057,#46058,#46059,#46060,#46061,#46062,#46063,
#46064,#46065,#46066,#46067,#46068,#46069,#46070,#46071,#46072,#46073,#46074,
#46075,#46076,#46077,#46078,#46079,#46080,#46081,#46082,#46083,#46084,#46085),
 .UNSPECIFIED.,.F.,.F.,(4,3,3,3,3,3,3,3,3,3,3,3,3,3,3,3,3,3,3,3,3,3,3,3,
3,3,3,3,3,3,3,3,3,3,3,3,3,3,3,3,3,3,3,3,3,3,3,3,3,3,3,3,3,3,3,3,3,3,3,3,
3,3,3,3,3,3,3,3,3,3,3,4),(1.24128043371927E-7,0.015891562160926,0.0300286940322461,
0.0432212521704566,0.05557791814208,0.0625000000000095,0.0703125000000105,
0.0712890625000107,0.0722656250000108,0.0742187500000111,0.0781250000000118,
0.0928053510640078,0.0937500000000149,0.107516496092903,0.109375000000018,
0.117187500000019,0.12109375000002,0.12304687500002,0.124023437500021,0.125000000000021,
0.145662774835165,0.156250000000027,0.17187500000003,0.179687500000032,
0.186597991532914,0.187500000000034,0.21875000000004,0.234375000000043,
0.242187500000045,0.249023437500046,0.250000000000046,0.273932641896201,
0.297753405674291,0.312500000000052,0.336671055712276,0.343750000000055,
0.359375000000056,0.367187500000057,0.371093750000057,0.373046875000057,
0.374023437500057,0.375000000000057,0.402435118120539,0.437500000000063,
0.468750000000065,0.484375000000066,0.492187500000067,0.496093750000067,
0.498046875000068,0.499023437500068,0.499511718750068,0.500000000000068,
0.531460033117952,0.563796472906449,0.598894267150548,0.625000000000055,
0.661169640469963,0.687500000000049,0.712240745703438,0.718750000000046,
0.734375000000044,0.742187500000043,0.746093750000043,0.748046875000043,
0.749023437500043,0.750000000000043,0.795746761194119,0.840593239925973,
0.884608181145608,0.928337940845234,0.971865941438119,1.),.UNSPECIFIED.);
#186=B_SPLINE_CURVE_WITH_KNOTS('',3,(#46168,#46169,#46170,#46171,#46172,
#46173,#46174,#46175,#46176,#46177,#46178,#46179,#46180,#46181,#46182,#46183,
#46184,#46185,#46186,#46187,#46188,#46189,#46190,#46191,#46192,#46193,#46194,
#46195,#46196,#46197,#46198,#46199,#46200,#46201,#46202,#46203,#46204,#46205,
#46206,#46207,#46208,#46209,#46210,#46211,#46212,#46213,#46214,#46215,#46216,
#46217,#46218,#46219,#46220,#46221,#46222,#46223,#46224,#46225,#46226,#46227,
#46228,#46229,#46230,#46231,#46232,#46233,#46234,#46235,#46236,#46237,#46238,
#46239,#46240,#46241,#46242,#46243,#46244,#46245,#46246,#46247,#46248,#46249,
#46250,#46251,#46252,#46253,#46254,#46255,#46256,#46257,#46258,#46259,#46260,
#46261,#46262,#46263,#46264,#46265,#46266,#46267,#46268,#46269,#46270,#46271,
#46272,#46273,#46274,#46275,#46276,#46277,#46278,#46279,#46280,#46281,#46282,
#46283,#46284,#46285,#46286,#46287,#46288,#46289,#46290,#46291,#46292,#46293,
#46294,#46295,#46296,#46297,#46298,#46299,#46300,#46301,#46302,#46303,#46304,
#46305,#46306,#46307,#46308,#46309,#46310,#46311,#46312,#46313,#46314,#46315,
#46316,#46317,#46318,#46319,#46320,#46321,#46322,#46323,#46324),
 .UNSPECIFIED.,.F.,.F.,(4,3,3,3,3,3,3,3,3,3,3,3,3,3,3,3,3,3,3,3,3,3,3,3,
3,3,3,3,3,3,3,3,3,3,3,3,3,3,3,3,3,3,3,3,3,3,3,3,3,3,3,3,4),(1.72726522874983E-7,
0.0434573072685472,0.0863338335472871,0.0932169511630213,0.12499999999998,
0.165840004073318,0.177273506753014,0.18749999999997,0.218749999999965,
0.234374999999962,0.242187499999961,0.246093749999961,0.24951171874996,
0.24999999999996,0.260113690588123,0.284905125085302,0.309602223495068,
0.312499999999967,0.336932319725918,0.34374999999997,0.359374999999972,
0.359741529143133,0.367187499999972,0.371093749999973,0.373046874999973,
0.374023437499973,0.374999999999973,0.427161963218175,0.437499999999976,
0.446539047580839,0.468749999999977,0.484374999999978,0.492187499999978,
0.49905822671156,0.499999999999979,0.529372232587649,0.595488563256059,
0.601624357332451,0.624999999999984,0.666786326505097,0.687499999999987,
0.718749999999988,0.726754195533532,0.734374999999989,0.746093749999989,
0.74999999999999,0.777564712519763,0.821930059504363,0.864143823680217,
0.906141086582859,0.94972602421565,0.995918324433868,0.999999956010986),
 .UNSPECIFIED.);
#187=B_SPLINE_CURVE_WITH_KNOTS('',3,(#46365,#46366,#46367,#46368,#46369,
#46370,#46371,#46372,#46373,#46374,#46375,#46376,#46377,#46378,#46379,#46380,
#46381,#46382,#46383,#46384,#46385,#46386,#46387,#46388,#46389,#46390,#46391,
#46392,#46393,#46394,#46395),.UNSPECIFIED.,.F.,.F.,(4,3,3,3,3,3,3,3,3,3,
4),(0.,0.125000000000005,0.187500000000008,0.218750000000008,0.234375000000008,
0.242187500000007,0.250000000000007,0.375000000000007,0.500000000000006,
0.750000000000003,1.),.UNSPECIFIED.);
#188=B_SPLINE_CURVE_WITH_KNOTS('',3,(#46397,#46398,#46399,#46400,#46401,
#46402,#46403,#46404,#46405,#46406,#46407,#46408,#46409,#46410,#46411,#46412,
#46413,#46414,#46415,#46416,#46417,#46418,#46419,#46420,#46421),
 .UNSPECIFIED.,.F.,.F.,(4,3,3,3,3,3,3,3,4),(6.00778538742285E-12,0.168745739560462,
0.282139878481535,0.3333333333333,0.590532057928784,0.6666666666667,0.840266058577053,
0.865637391095598,0.999997478430659),.UNSPECIFIED.);
#189=B_SPLINE_CURVE_WITH_KNOTS('',3,(#46424,#46425,#46426,#46427,#46428,
#46429,#46430,#46431,#46432,#46433,#46434,#46435,#46436,#46437,#46438,#46439,
#46440,#46441,#46442,#46443,#46444,#46445,#46446,#46447,#46448,#46449,#46450,
#46451,#46452,#46453,#46454,#46455,#46456,#46457,#46458,#46459,#46460,#46461,
#46462,#46463,#46464,#46465,#46466,#46467,#46468,#46469,#46470,#46471,#46472,
#46473,#46474,#46475,#46476,#46477,#46478,#46479,#46480,#46481,#46482,#46483,
#46484,#46485,#46486,#46487),.UNSPECIFIED.,.F.,.F.,(4,3,3,3,3,3,3,3,3,3,
3,3,3,3,3,3,3,3,3,3,3,4),(0.,0.0982799701893736,0.213482755431675,0.250000000000042,
0.295950559396774,0.375000000000063,0.437500000000075,0.468750000000081,
0.484375000000084,0.488569176919273,0.492187500000084,0.498693625937138,
0.500000000000084,0.581892466489566,0.659367760809361,0.71516477614781,
0.750000000000042,0.822980248697091,0.892544871534579,0.904183472300278,
0.970836803729396,1.),.UNSPECIFIED.);
#190=B_SPLINE_CURVE_WITH_KNOTS('',3,(#46532,#46533,#46534,#46535,#46536,
#46537,#46538,#46539,#46540,#46541,#46542,#46543,#46544,#46545,#46546,#46547,
#46548,#46549,#46550,#46551,#46552,#46553,#46554,#46555,#46556,#46557,#46558,
#46559,#46560,#46561,#46562,#46563,#46564,#46565,#46566,#46567,#46568,#46569,
#46570,#46571,#46572,#46573,#46574,#46575,#46576,#46577,#46578,#46579,#46580,
#46581,#46582,#46583,#46584,#46585,#46586,#46587,#46588,#46589,#46590,#46591,
#46592,#46593,#46594,#46595,#46596,#46597,#46598,#46599,#46600,#46601),
 .UNSPECIFIED.,.F.,.F.,(4,3,3,3,3,3,3,3,3,3,3,3,3,3,3,3,3,3,3,3,3,3,3,4),
(0.,0.0435516393491532,0.076471965080317,0.120148484350007,0.125,0.178495710860988,
0.223908387543282,0.25,0.318709089634349,0.371577560495655,0.375,0.469052171169697,
0.5,0.519438375467887,0.625,0.667314602754769,0.741711825535796,0.75,0.808035501625466,
0.814958553106824,0.875,0.91974261032604,0.962451614850442,0.999999720291478),
 .UNSPECIFIED.);
#191=B_SPLINE_CURVE_WITH_KNOTS('',3,(#46602,#46603,#46604,#46605,#46606,
#46607,#46608,#46609,#46610,#46611,#46612,#46613,#46614,#46615,#46616,#46617,
#46618,#46619,#46620,#46621,#46622,#46623,#46624,#46625,#46626,#46627,#46628,
#46629,#46630,#46631,#46632,#46633,#46634,#46635,#46636,#46637,#46638,#46639,
#46640,#46641,#46642,#46643,#46644,#46645,#46646,#46647,#46648,#46649,#46650,
#46651,#46652,#46653,#46654,#46655,#46656,#46657,#46658,#46659,#46660,#46661,
#46662,#46663,#46664,#46665,#46666,#46667,#46668,#46669,#46670,#46671),
 .UNSPECIFIED.,.F.,.F.,(4,3,3,3,3,3,3,3,3,3,3,3,3,3,3,3,3,3,3,3,3,3,3,4),
(0.,0.0642448454708453,0.129222404838902,0.139648705363206,0.20336349094211,
0.25,0.30065642377295,0.369078211886475,0.437500000000001,0.468750000000001,
0.469711808549797,0.484375000000001,0.495155161137369,0.5,0.563334814263254,
0.625630949976613,0.644014791014155,0.704247046610669,0.75,0.807879635213996,
0.868482419985881,0.928163504115579,0.9619622907836,0.999999992443124),
 .UNSPECIFIED.);
#192=B_SPLINE_CURVE_WITH_KNOTS('',3,(#46707,#46708,#46709,#46710,#46711,
#46712,#46713,#46714,#46715,#46716,#46717,#46718,#46719,#46720,#46721,#46722,
#46723,#46724,#46725,#46726,#46727,#46728,#46729,#46730,#46731,#46732,#46733,
#46734,#46735,#46736,#46737,#46738,#46739,#46740,#46741,#46742,#46743,#46744,
#46745,#46746,#46747,#46748,#46749,#46750,#46751,#46752,#46753,#46754,#46755,
#46756,#46757,#46758,#46759,#46760,#46761,#46762,#46763,#46764),
 .UNSPECIFIED.,.F.,.F.,(4,3,3,3,3,3,3,3,3,3,3,3,3,3,3,3,3,3,3,4),(1.01449595492675E-11,
0.0705966753463834,0.136832386883981,0.198363721951571,0.25,0.306585362611179,
0.362372014726767,0.417803058925887,0.472856063303982,0.499998113896311,
0.5,0.555653427215775,0.611786177000757,0.668294513633687,0.725515077026516,
0.75,0.8125,0.876968707688738,0.94757495842845,1.),.UNSPECIFIED.);
#193=B_SPLINE_CURVE_WITH_KNOTS('',3,(#46801,#46802,#46803,#46804,#46805,
#46806,#46807,#46808,#46809,#46810,#46811,#46812,#46813,#46814,#46815,#46816,
#46817,#46818,#46819,#46820,#46821,#46822,#46823,#46824,#46825,#46826,#46827,
#46828,#46829,#46830,#46831,#46832,#46833,#46834,#46835,#46836,#46837,#46838,
#46839,#46840,#46841,#46842,#46843,#46844,#46845,#46846,#46847,#46848,#46849,
#46850,#46851,#46852,#46853,#46854,#46855,#46856,#46857,#46858,#46859,#46860,
#46861,#46862,#46863,#46864,#46865,#46866,#46867,#46868,#46869,#46870),
 .UNSPECIFIED.,.F.,.F.,(4,3,3,3,3,3,3,3,3,3,3,3,3,3,3,3,3,3,3,3,3,3,3,4),
(0.,0.080844790934893,0.125,0.133450088539653,0.1875,0.21875,0.235735057515083,
0.25,0.318589046603858,0.38951330554323,0.461228032467734,0.5,0.500070526558878,
0.569716537362397,0.625,0.681559788616792,0.6875,0.71875,0.735656425285893,
0.75,0.825645197998783,0.866690726110233,0.943548522664466,1.),
 .UNSPECIFIED.);
#194=B_SPLINE_CURVE_WITH_KNOTS('',3,(#46909,#46910,#46911,#46912,#46913,
#46914,#46915,#46916,#46917,#46918,#46919,#46920,#46921,#46922,#46923,#46924,
#46925,#46926,#46927,#46928,#46929,#46930,#46931,#46932,#46933,#46934,#46935,
#46936,#46937,#46938,#46939,#46940,#46941,#46942,#46943,#46944,#46945,#46946,
#46947,#46948,#46949,#46950,#46951,#46952,#46953,#46954,#46955,#46956,#46957,
#46958,#46959,#46960,#46961,#46962,#46963,#46964,#46965,#46966),
 .UNSPECIFIED.,.F.,.F.,(4,3,3,3,3,3,3,3,3,3,3,3,3,3,3,3,3,3,3,4),(2.82054536219499E-11,
0.0625000000211541,0.123435816746246,0.183432146452882,0.242373947342859,
0.25,0.308039798384561,0.365336042404427,0.422295827820954,0.479062336025,
0.535777734589141,0.592769485322273,0.649981729622503,0.707851349801787,
0.75,0.80890213970272,0.869151808551022,0.93029395044618,0.992902535032498,
1.),.UNSPECIFIED.);
#195=B_SPLINE_CURVE_WITH_KNOTS('',3,(#46968,#46969,#46970,#46971,#46972,
#46973,#46974,#46975,#46976,#46977,#46978,#46979,#46980,#46981,#46982,#46983,
#46984,#46985,#46986,#46987,#46988,#46989,#46990,#46991,#46992),
 .UNSPECIFIED.,.F.,.F.,(4,3,3,3,3,3,3,3,4),(1.26985457340339E-6,0.173312592767027,
0.210273395635445,0.3333333333333,0.613202238647455,0.6666666666667,0.775173469127502,
0.943222799720604,0.999999999999632),.UNSPECIFIED.);
#196=B_SPLINE_CURVE_WITH_KNOTS('',3,(#46994,#46995,#46996,#46997,#46998,
#46999,#47000,#47001,#47002,#47003,#47004,#47005,#47006),.UNSPECIFIED.,
 .F.,.F.,(4,3,3,3,4),(0.,0.187500000000003,0.250000000000004,0.500000000000003,
1.),.UNSPECIFIED.);
#197=B_SPLINE_CURVE_WITH_KNOTS('',3,(#47007,#47008,#47009,#47010,#47011,
#47012,#47013,#47014,#47015,#47016,#47017,#47018,#47019,#47020,#47021,#47022,
#47023,#47024,#47025,#47026,#47027,#47028,#47029,#47030,#47031,#47032,#47033,
#47034,#47035,#47036,#47037,#47038,#47039,#47040,#47041,#47042,#47043,#47044,
#47045,#47046,#47047,#47048,#47049,#47050,#47051,#47052,#47053,#47054,#47055,
#47056,#47057,#47058,#47059,#47060,#47061),.UNSPECIFIED.,.F.,.F.,(4,3,3,
3,3,3,3,3,3,3,3,3,3,3,3,3,3,3,4),(0.,0.0638950390766455,0.126878094455892,
0.195427827297906,0.249999999999974,0.317220939245595,0.392664016611647,
0.437499999999954,0.46874999999995,0.484374999999948,0.492187499999948,
0.498924460179924,0.499999999999948,0.53547877547165,0.642764494845113,
0.725136941874545,0.836917893499071,0.92006383085474,0.999999999858759),
 .UNSPECIFIED.);
#198=B_SPLINE_CURVE_WITH_KNOTS('',3,(#47107,#47108,#47109,#47110,#47111,
#47112,#47113,#47114,#47115,#47116,#47117,#47118,#47119,#47120,#47121,#47122,
#47123,#47124,#47125,#47126,#47127,#47128,#47129,#47130,#47131,#47132,#47133,
#47134,#47135,#47136,#47137,#47138,#47139,#47140,#47141,#47142,#47143,#47144,
#47145,#47146,#47147,#47148,#47149,#47150,#47151,#47152,#47153,#47154,#47155,
#47156,#47157,#47158,#47159,#47160,#47161,#47162,#47163,#47164,#47165,#47166,
#47167,#47168,#47169,#47170,#47171,#47172,#47173,#47174,#47175,#47176,#47177,
#47178,#47179),.UNSPECIFIED.,.F.,.F.,(4,3,3,3,3,3,3,3,3,3,3,3,3,3,3,3,3,
3,3,3,3,3,3,3,4),(1.45401629951061E-9,0.0431123239999773,0.0863131632793753,
0.129361943345478,0.1428571428571,0.153622120796769,0.204599117366318,0.255683865453928,
0.2857142857143,0.306349836570465,0.370801351683843,0.4285714285714,0.459346573254742,
0.526502052474814,0.5714285714286,0.6124033147054,0.676566373102767,0.7142857142857,
0.765276986306117,0.818291690290777,0.8571428571429,0.900814093153431,0.918051250558587,
0.961570051922101,1.),.UNSPECIFIED.);
#199=B_SPLINE_CURVE_WITH_KNOTS('',3,(#47182,#47183,#47184,#47185,#47186,
#47187,#47188,#47189,#47190,#47191,#47192,#47193,#47194,#47195,#47196,#47197,
#47198,#47199,#47200,#47201,#47202,#47203,#47204,#47205,#47206,#47207,#47208,
#47209,#47210,#47211,#47212,#47213,#47214,#47215,#47216,#47217,#47218,#47219,
#47220,#47221,#47222,#47223,#47224,#47225,#47226,#47227,#47228,#47229,#47230,
#47231,#47232,#47233,#47234,#47235,#47236,#47237,#47238,#47239,#47240,#47241,
#47242,#47243,#47244,#47245,#47246,#47247,#47248,#47249,#47250,#47251,#47252,
#47253,#47254),.UNSPECIFIED.,.F.,.F.,(4,3,3,3,3,3,3,3,3,3,3,3,3,3,3,3,3,
3,3,3,3,3,3,3,4),(0.,0.0558892484596122,0.112669228063845,0.156953132120896,
0.215051927917948,0.249999999999994,0.309316239775135,0.324310165349072,
0.385390341081382,0.437499999999991,0.468749999999991,0.484374999999991,
0.49218749999999,0.498949344757548,0.499999999999989,0.504582992961993,
0.573408021618643,0.641343129323671,0.680145625695793,0.749999999999995,
0.815926496427531,0.847891711430229,0.914669420517686,0.980716617979016,
1.),.UNSPECIFIED.);
#200=B_SPLINE_CURVE_WITH_KNOTS('',3,(#47353,#47354,#47355,#47356,#47357,
#47358,#47359,#47360,#47361,#47362,#47363,#47364,#47365,#47366,#47367,#47368,
#47369,#47370,#47371,#47372,#47373,#47374,#47375,#47376,#47377,#47378,#47379,
#47380,#47381,#47382,#47383,#47384,#47385,#47386,#47387,#47388,#47389,#47390,
#47391,#47392,#47393,#47394,#47395,#47396,#47397,#47398,#47399,#47400,#47401,
#47402,#47403,#47404,#47405,#47406,#47407,#47408,#47409,#47410,#47411,#47412,
#47413,#47414,#47415,#47416,#47417,#47418,#47419,#47420,#47421,#47422,#47423,
#47424,#47425,#47426,#47427,#47428,#47429,#47430,#47431,#47432,#47433,#47434,
#47435,#47436,#47437,#47438,#47439,#47440,#47441,#47442,#47443,#47444,#47445,
#47446,#47447,#47448,#47449,#47450,#47451,#47452,#47453,#47454,#47455,#47456,
#47457,#47458,#47459,#47460,#47461,#47462,#47463,#47464,#47465,#47466,#47467,
#47468,#47469,#47470,#47471,#47472,#47473,#47474,#47475,#47476,#47477,#47478,
#47479,#47480,#47481,#47482,#47483,#47484,#47485,#47486,#47487,#47488,#47489,
#47490,#47491,#47492,#47493,#47494,#47495,#47496,#47497,#47498,#47499,#47500,
#47501,#47502,#47503,#47504,#47505,#47506,#47507,#47508,#47509,#47510,#47511,
#47512,#47513,#47514,#47515,#47516,#47517,#47518),.UNSPECIFIED.,.F.,.F.,
(4,3,3,3,3,3,3,3,3,3,3,3,3,3,3,3,3,3,3,3,3,3,3,3,3,3,3,3,3,3,3,3,3,3,3,
3,3,3,3,3,3,3,3,3,3,3,3,3,3,3,3,3,3,3,3,4),(8.91796408023666E-8,0.0341889233158358,
0.0625000000000036,0.0800235801138546,0.0937500000000054,0.109375000000006,
0.117187500000007,0.121093750000007,0.123046875000007,0.125000000000007,
0.156896093638754,0.187500000000008,0.218750000000008,0.234375000000008,
0.237544069792359,0.242187500000008,0.246093750000008,0.248046875000008,
0.250000000000008,0.29085297613211,0.312500000000008,0.328940100260377,
0.343750000000007,0.359375000000007,0.367187500000007,0.371093750000007,
0.373046875000007,0.375000000000007,0.425222667492041,0.437500000000007,
0.468750000000007,0.484375000000007,0.492187500000007,0.496093750000007,
0.500000000000007,0.520152743002406,0.572584842158793,0.616900729702386,
0.625000000000005,0.651342131071929,0.678251292688293,0.687500000000004,
0.709160584351542,0.750000000000004,0.781250000000003,0.789062500000003,
0.796875000000003,0.799072641440133,0.812500000000003,0.858399949290242,
0.875000000000002,0.885492822282815,0.932681905157277,0.980790028010998,
0.985730934543369,1.),.UNSPECIFIED.);
#201=B_SPLINE_CURVE_WITH_KNOTS('',3,(#47521,#47522,#47523,#47524,#47525,
#47526,#47527,#47528,#47529,#47530,#47531,#47532,#47533,#47534,#47535,#47536,
#47537,#47538,#47539,#47540,#47541,#47542,#47543,#47544,#47545,#47546,#47547,
#47548,#47549,#47550,#47551,#47552,#47553,#47554,#47555,#47556,#47557,#47558,
#47559,#47560,#47561,#47562,#47563,#47564,#47565,#47566,#47567,#47568,#47569,
#47570,#47571,#47572,#47573,#47574,#47575,#47576,#47577,#47578,#47579,#47580,
#47581,#47582,#47583,#47584,#47585,#47586,#47587,#47588,#47589,#47590,#47591,
#47592,#47593,#47594,#47595,#47596,#47597,#47598,#47599,#47600,#47601,#47602,
#47603,#47604,#47605,#47606,#47607,#47608,#47609,#47610,#47611,#47612,#47613,
#47614,#47615,#47616,#47617,#47618,#47619,#47620,#47621,#47622,#47623,#47624,
#47625,#47626,#47627,#47628,#47629,#47630,#47631,#47632,#47633,#47634,#47635,
#47636,#47637,#47638,#47639,#47640,#47641,#47642,#47643,#47644,#47645,#47646,
#47647,#47648,#47649,#47650,#47651,#47652,#47653,#47654,#47655,#47656,#47657,
#47658,#47659,#47660,#47661,#47662),.UNSPECIFIED.,.F.,.F.,(4,3,3,3,3,3,
3,3,3,3,3,3,3,3,3,3,3,3,3,3,3,3,3,3,3,3,3,3,3,3,3,3,3,3,3,3,3,3,3,3,3,3,
3,3,3,3,3,4),(2.34638067050473E-7,0.0315958280048414,0.0628964697291262,
0.0937122537280348,0.104172143004049,0.125000000000003,0.154837231687147,
0.184674463374292,0.213175783877095,0.218750000000005,0.234375000000006,
0.242187500000006,0.246093750000006,0.248046875000006,0.250000000000006,
0.257790373821085,0.295642404986771,0.334483401403744,0.354334938901152,
0.392683241215207,0.431398966624688,0.470482034495911,0.482378819653905,
0.484375000000001,0.496585822661942,0.500000000000001,0.540377618734413,
0.580372331510874,0.609456767722748,0.649167581317096,0.687499999999997,
0.700832884820975,0.718749999999996,0.734374999999996,0.742187499999996,
0.746093749999996,0.748046874999996,0.749999999999996,0.76909192808113,
0.798967073993967,0.828842219906804,0.858577127007425,0.874999999999998,
0.896782378211392,0.927914314370241,0.959582515324487,0.985641745354497,
1.),.UNSPECIFIED.);
#202=B_SPLINE_CURVE_WITH_KNOTS('',3,(#47699,#47700,#47701,#47702,#47703,
#47704,#47705,#47706,#47707,#47708,#47709,#47710,#47711,#47712,#47713,#47714,
#47715,#47716,#47717,#47718,#47719,#47720,#47721,#47722,#47723,#47724,#47725,
#47726,#47727,#47728,#47729,#47730,#47731,#47732,#47733,#47734,#47735,#47736,
#47737,#47738,#47739,#47740,#47741,#47742,#47743,#47744,#47745,#47746,#47747,
#47748,#47749,#47750,#47751,#47752,#47753,#47754,#47755,#47756,#47757,#47758,
#47759),.UNSPECIFIED.,.F.,.F.,(4,3,3,3,3,3,3,3,3,3,3,3,3,3,3,3,3,3,3,3,
4),(3.81437099953529E-8,0.0594692301267317,0.11946134523179,0.180335245674018,
0.22823334864808,0.25,0.3125,0.375,0.420629664625766,0.4664807256031,0.5,
0.532982689971054,0.595584386743332,0.657507316660725,0.71846862277759,
0.75,0.809830725006028,0.831293934527991,0.890887161148583,0.949594354583762,
1.),.UNSPECIFIED.);
#203=B_SPLINE_CURVE_WITH_KNOTS('',3,(#47760,#47761,#47762,#47763,#47764,
#47765,#47766,#47767,#47768,#47769,#47770,#47771,#47772,#47773,#47774,#47775,
#47776,#47777,#47778,#47779,#47780,#47781,#47782,#47783,#47784,#47785,#47786,
#47787,#47788,#47789,#47790,#47791,#47792,#47793,#47794,#47795,#47796,#47797,
#47798,#47799,#47800,#47801,#47802,#47803,#47804,#47805,#47806,#47807,#47808,
#47809,#47810,#47811,#47812,#47813,#47814,#47815,#47816,#47817),
 .UNSPECIFIED.,.F.,.F.,(4,3,3,3,3,3,3,3,3,3,3,3,3,3,3,3,3,3,3,4),(0.,0.0701431897639297,
0.13604417473497,0.197334652086801,0.25,0.307833948589721,0.364819438044064,
0.421421997850492,0.477619532142297,0.5,0.500034450215325,0.555641456198574,
0.611685710202809,0.668080534996765,0.725149887541437,0.75,0.8125,0.876721757771727,
0.946972970382545,1.),.UNSPECIFIED.);
#204=B_SPLINE_CURVE_WITH_KNOTS('',3,(#47863,#47864,#47865,#47866,#47867,
#47868,#47869,#47870,#47871,#47872,#47873,#47874,#47875,#47876,#47877,#47878,
#47879,#47880,#47881,#47882,#47883,#47884,#47885,#47886,#47887,#47888,#47889,
#47890,#47891,#47892,#47893,#47894,#47895,#47896,#47897,#47898,#47899,#47900,
#47901,#47902,#47903,#47904,#47905,#47906,#47907,#47908,#47909,#47910,#47911,
#47912,#47913,#47914,#47915,#47916,#47917,#47918,#47919,#47920),
 .UNSPECIFIED.,.F.,.F.,(4,3,3,3,3,3,3,3,3,3,3,3,3,3,3,3,3,3,3,4),(0.,0.0625,
0.123429164348376,0.183419166724562,0.24235510130439,0.25,0.308040960610337,
0.365338359396875,0.422299309833655,0.479067004587782,0.535783618539891,
0.592776619814919,0.649990135834089,0.707861008608383,0.75,0.808903107716075,
0.869153662199582,0.930296626253199,0.992905895259067,1.),.UNSPECIFIED.);
#205=B_SPLINE_CURVE_WITH_KNOTS('',3,(#47921,#47922,#47923,#47924,#47925,
#47926,#47927,#47928,#47929,#47930,#47931,#47932,#47933,#47934,#47935,#47936,
#47937,#47938,#47939,#47940,#47941,#47942,#47943,#47944,#47945,#47946,#47947,
#47948,#47949,#47950,#47951,#47952,#47953,#47954,#47955,#47956,#47957,#47958,
#47959,#47960,#47961,#47962,#47963,#47964,#47965,#47966,#47967,#47968,#47969,
#47970,#47971,#47972,#47973,#47974,#47975,#47976,#47977,#47978,#47979,#47980,
#47981,#47982,#47983,#47984,#47985,#47986,#47987,#47988,#47989,#47990,#47991,
#47992,#47993,#47994,#47995,#47996,#47997,#47998,#47999,#48000,#48001,#48002,
#48003,#48004,#48005,#48006,#48007,#48008,#48009,#48010,#48011,#48012,#48013,
#48014,#48015,#48016,#48017,#48018,#48019,#48020),.UNSPECIFIED.,.F.,.F.,
(4,3,3,3,3,3,3,3,3,3,3,3,3,3,3,3,3,3,3,3,3,3,3,3,3,3,3,3,3,3,3,3,3,4),(0.,
0.00328733869888417,0.0753749786215322,0.124999999999997,0.164356278458853,
0.187499999999995,0.218749999999994,0.234374999999994,0.242187499999994,
0.246093749999994,0.24961089402613,0.249999999999994,0.315510705211053,
0.331931331987761,0.396997846930877,0.460736474732702,0.499909864635484,
0.499999999999991,0.563260702089509,0.624999999999989,0.667901539577085,
0.687499999999989,0.718749999999988,0.734374999999988,0.742187499999988,
0.746093749999988,0.749555837689128,0.749999999999988,0.820384404417581,
0.835461566544658,0.907599319949528,0.981379542643532,0.996551188491584,
1.),.UNSPECIFIED.);
#206=B_SPLINE_CURVE_WITH_KNOTS('',3,(#48059,#48060,#48061,#48062,#48063,
#48064,#48065,#48066,#48067,#48068,#48069,#48070,#48071,#48072,#48073,#48074,
#48075,#48076,#48077,#48078,#48079,#48080,#48081,#48082,#48083,#48084,#48085,
#48086,#48087,#48088,#48089),.UNSPECIFIED.,.F.,.F.,(4,3,3,3,3,3,3,3,3,3,
4),(0.,0.124999999999988,0.187499999999983,0.21874999999998,0.234374999999979,
0.24218749999998,0.24999999999998,0.374999999999982,0.499999999999985,0.749999999999992,
1.),.UNSPECIFIED.);
#207=B_SPLINE_CURVE_WITH_KNOTS('',3,(#48090,#48091,#48092,#48093,#48094,
#48095),.UNSPECIFIED.,.F.,.F.,(4,1,1,4),(0.,0.3333333333333,0.6666666666667,
0.999998511429527),.UNSPECIFIED.);
#208=B_SPLINE_CURVE_WITH_KNOTS('',3,(#48096,#48097,#48098,#48099,#48100,
#48101,#48102,#48103,#48104,#48105,#48106,#48107,#48108,#48109,#48110,#48111,
#48112,#48113,#48114,#48115,#48116,#48117,#48118,#48119,#48120,#48121,#48122,
#48123,#48124,#48125,#48126,#48127,#48128,#48129,#48130,#48131,#48132,#48133,
#48134,#48135,#48136,#48137,#48138,#48139,#48140,#48141,#48142,#48143,#48144,
#48145,#48146,#48147,#48148,#48149,#48150,#48151,#48152,#48153,#48154,#48155,
#48156),.UNSPECIFIED.,.F.,.F.,(4,3,3,3,3,3,3,3,3,3,3,3,3,3,3,3,3,3,3,3,
4),(1.42553447152832E-10,0.0839810989411267,0.196377742902089,0.24999999999996,
0.279015455686927,0.37499999999994,0.437499999999929,0.468749999999923,
0.468865232487923,0.484374999999921,0.492187499999922,0.498689296997412,
0.499999999999923,0.579361224328497,0.654563668474195,0.68797699979001,
0.749999999999961,0.818702539099431,0.877832781625891,0.941885020163088,
0.999999999925446),.UNSPECIFIED.);
#209=B_SPLINE_CURVE_WITH_KNOTS('',3,(#48199,#48200,#48201,#48202,#48203,
#48204,#48205,#48206,#48207,#48208,#48209,#48210,#48211,#48212,#48213,#48214,
#48215,#48216,#48217,#48218,#48219,#48220,#48221,#48222,#48223,#48224,#48225,
#48226,#48227,#48228,#48229,#48230,#48231,#48232,#48233,#48234,#48235,#48236,
#48237,#48238,#48239,#48240,#48241,#48242,#48243,#48244,#48245,#48246,#48247,
#48248,#48249,#48250,#48251,#48252,#48253,#48254,#48255,#48256,#48257,#48258,
#48259,#48260,#48261,#48262,#48263,#48264,#48265,#48266,#48267,#48268,#48269,
#48270,#48271,#48272,#48273,#48274,#48275,#48276,#48277,#48278,#48279,#48280,
#48281,#48282,#48283,#48284,#48285,#48286,#48287,#48288,#48289),
 .UNSPECIFIED.,.F.,.F.,(4,3,3,3,3,3,3,3,3,3,3,3,3,3,3,3,3,3,3,3,3,3,3,3,
3,3,3,3,3,3,4),(1.9887196109883E-7,0.0470903055258525,0.0950885788175302,
0.109526530949826,0.125000000000002,0.176685448395246,0.187500000000003,
0.195574875832608,0.203125000000002,0.218750000000002,0.250000000000001,
0.270621369536984,0.334103679086635,0.398264763362707,0.43041445463061,
0.437499999999997,0.468749999999996,0.484374999999996,0.492187499999997,
0.498034134221128,0.499999999999997,0.559924709834862,0.600124997687488,
0.658475316866043,0.715889402365164,0.764251055692731,0.821850435693596,
0.87861656776704,0.918179747173176,0.97096325070799,1.),.UNSPECIFIED.);
#210=B_SPLINE_CURVE_WITH_KNOTS('',3,(#48330,#48331,#48332,#48333,#48334,
#48335,#48336,#48337,#48338,#48339,#48340,#48341,#48342,#48343,#48344,#48345,
#48346,#48347,#48348,#48349,#48350,#48351,#48352,#48353,#48354,#48355,#48356,
#48357,#48358,#48359,#48360,#48361,#48362,#48363,#48364,#48365,#48366,#48367,
#48368,#48369,#48370,#48371,#48372,#48373,#48374,#48375,#48376,#48377,#48378,
#48379,#48380,#48381,#48382,#48383,#48384,#48385,#48386,#48387),
 .UNSPECIFIED.,.F.,.F.,(4,3,3,3,3,3,3,3,3,3,3,3,3,3,3,3,3,3,3,4),(0.,0.0625,
0.123439667231836,0.183439614487077,0.242384759211611,0.25,0.308039807183335,
0.365336058327834,0.422295847686103,0.479062355395686,0.535777748341937,
0.592769485850589,0.64998171356429,0.707851314182894,0.75,0.808900888439781,
0.869149194465956,0.930289889916406,0.992896943668474,1.),.UNSPECIFIED.);
#211=B_SPLINE_CURVE_WITH_KNOTS('',3,(#48389,#48390,#48391,#48392,#48393,
#48394,#48395,#48396,#48397,#48398,#48399,#48400,#48401,#48402,#48403,#48404,
#48405,#48406,#48407,#48408,#48409,#48410,#48411,#48412,#48413),
 .UNSPECIFIED.,.F.,.F.,(4,3,3,3,3,3,3,3,4),(2.75410129806085E-6,0.104998984641379,
0.285738798613509,0.468553914078819,0.5,0.679723771264366,0.694842839233207,
0.871856624429499,0.999999999992336),.UNSPECIFIED.);
#212=B_SPLINE_CURVE_WITH_KNOTS('',3,(#48415,#48416,#48417,#48418,#48419,
#48420,#48421,#48422,#48423,#48424,#48425,#48426,#48427),.UNSPECIFIED.,
 .F.,.F.,(4,3,3,3,4),(0.,0.218750000000002,0.250000000000002,0.500000000000001,
1.),.UNSPECIFIED.);
#213=B_SPLINE_CURVE_WITH_KNOTS('',3,(#48428,#48429,#48430,#48431,#48432,
#48433,#48434,#48435,#48436,#48437,#48438,#48439,#48440,#48441,#48442,#48443,
#48444,#48445,#48446,#48447,#48448,#48449,#48450,#48451,#48452,#48453,#48454,
#48455,#48456,#48457,#48458,#48459,#48460,#48461,#48462,#48463,#48464,#48465,
#48466,#48467,#48468,#48469,#48470,#48471,#48472,#48473,#48474,#48475,#48476,
#48477,#48478,#48479,#48480,#48481,#48482,#48483,#48484,#48485),
 .UNSPECIFIED.,.F.,.F.,(4,3,3,3,3,3,3,3,3,3,3,3,3,3,3,3,3,3,3,4),(0.,0.0665772925752716,
0.0719281228356136,0.141169980961546,0.214018425126579,0.249999999999986,
0.264563302840939,0.341169571707878,0.374999999999978,0.437499999999976,
0.468749999999975,0.484374999999976,0.486525989533565,0.496474805711493,
0.499999999999976,0.607879987507896,0.687145580677176,0.799955784674695,
0.890947396547385,1.),.UNSPECIFIED.);
#214=B_SPLINE_CURVE_WITH_KNOTS('',3,(#48527,#48528,#48529,#48530,#48531,
#48532,#48533,#48534,#48535,#48536,#48537,#48538,#48539,#48540,#48541,#48542,
#48543,#48544,#48545,#48546,#48547,#48548,#48549,#48550,#48551,#48552,#48553,
#48554,#48555,#48556,#48557,#48558,#48559,#48560,#48561,#48562,#48563,#48564,
#48565,#48566,#48567,#48568,#48569,#48570,#48571,#48572,#48573,#48574,#48575,
#48576,#48577,#48578,#48579,#48580,#48581,#48582,#48583,#48584,#48585,#48586,
#48587,#48588,#48589,#48590,#48591,#48592,#48593,#48594,#48595,#48596,#48597,
#48598,#48599,#48600,#48601,#48602,#48603,#48604,#48605,#48606,#48607,#48608,
#48609,#48610,#48611,#48612,#48613,#48614),.UNSPECIFIED.,.F.,.F.,(4,3,3,
3,3,3,3,3,3,3,3,3,3,3,3,3,3,3,3,3,3,3,3,3,3,3,3,3,3,4),(0.,0.0527820704689245,
0.081820550075384,0.138472337731971,0.195944438078264,0.23574955951297,
0.293011727177245,0.351192985818588,0.399875426522106,0.437499999999996,
0.468749999999997,0.484374999999997,0.492187499999997,0.496093749999997,
0.499508599033293,0.499999999999998,0.56586096599558,0.629575206715251,
0.693959306753081,0.725751294986733,0.781250000000004,0.790730946680812,
0.796875000000004,0.812500000000004,0.86904415250083,0.875000000000003,
0.884835923229597,0.938701686179648,0.993362246004367,0.999999777714025),
 .UNSPECIFIED.);
#215=B_SPLINE_CURVE_WITH_KNOTS('',3,(#48617,#48618,#48619,#48620,#48621,
#48622,#48623,#48624,#48625,#48626,#48627,#48628,#48629,#48630,#48631,#48632,
#48633,#48634,#48635,#48636,#48637,#48638,#48639,#48640,#48641,#48642,#48643,
#48644,#48645,#48646,#48647,#48648,#48649,#48650,#48651,#48652,#48653,#48654,
#48655,#48656,#48657,#48658,#48659,#48660,#48661,#48662,#48663,#48664,#48665,
#48666,#48667,#48668,#48669,#48670,#48671,#48672,#48673,#48674),
 .UNSPECIFIED.,.F.,.F.,(4,3,3,3,3,3,3,3,3,3,3,3,3,3,3,3,3,3,3,4),(1.82694913577423E-11,
0.0585628393002113,0.117996178041119,0.168707834458927,0.22854128310571,
0.249999999999999,0.312499999999999,0.374999999999999,0.421054295308903,
0.467108590617808,0.499999999999999,0.56353289982233,0.626399530677736,
0.688223249658798,0.749999999999999,0.771768873464095,0.832605909367747,
0.892881470692987,0.952307026214462,0.999999961863703),.UNSPECIFIED.);
#216=B_SPLINE_CURVE_WITH_KNOTS('',3,(#48725,#48726,#48727,#48728,#48729,
#48730,#48731,#48732,#48733,#48734,#48735,#48736,#48737,#48738,#48739,#48740,
#48741,#48742,#48743,#48744,#48745,#48746,#48747,#48748,#48749,#48750,#48751,
#48752,#48753,#48754,#48755,#48756,#48757,#48758,#48759,#48760,#48761,#48762,
#48763,#48764,#48765,#48766,#48767,#48768,#48769,#48770,#48771,#48772,#48773,
#48774,#48775,#48776,#48777,#48778,#48779,#48780,#48781,#48782,#48783,#48784,
#48785,#48786,#48787,#48788,#48789,#48790,#48791,#48792,#48793,#48794,#48795,
#48796,#48797,#48798,#48799,#48800,#48801,#48802,#48803,#48804,#48805,#48806,
#48807,#48808,#48809,#48810,#48811,#48812,#48813,#48814,#48815,#48816,#48817,
#48818,#48819,#48820,#48821,#48822,#48823,#48824,#48825,#48826,#48827,#48828,
#48829,#48830,#48831,#48832,#48833,#48834,#48835,#48836,#48837,#48838,#48839,
#48840,#48841,#48842,#48843,#48844,#48845,#48846,#48847,#48848,#48849,#48850,
#48851,#48852,#48853,#48854,#48855,#48856,#48857,#48858,#48859,#48860,#48861,
#48862,#48863,#48864,#48865,#48866,#48867,#48868,#48869,#48870,#48871,#48872,
#48873,#48874,#48875,#48876,#48877,#48878,#48879,#48880,#48881,#48882,#48883,
#48884,#48885,#48886,#48887,#48888,#48889,#48890,#48891,#48892,#48893,#48894,
#48895,#48896,#48897,#48898,#48899,#48900,#48901,#48902,#48903,#48904,#48905,
#48906,#48907,#48908,#48909,#48910,#48911,#48912,#48913,#48914,#48915,#48916,
#48917,#48918,#48919,#48920,#48921,#48922,#48923,#48924,#48925,#48926,#48927,
#48928,#48929,#48930,#48931,#48932,#48933,#48934,#48935,#48936,#48937,#48938,
#48939,#48940,#48941,#48942,#48943,#48944,#48945,#48946,#48947,#48948,#48949,
#48950,#48951,#48952,#48953,#48954,#48955,#48956,#48957,#48958,#48959,#48960,
#48961,#48962,#48963,#48964,#48965,#48966,#48967,#48968,#48969,#48970,#48971),
 .UNSPECIFIED.,.F.,.F.,(4,3,3,3,3,3,3,3,3,3,3,3,3,3,3,3,3,3,3,3,3,3,3,3,
3,3,3,3,3,3,3,3,3,3,3,3,3,3,3,3,3,3,3,3,3,3,3,3,3,3,3,3,3,3,3,3,3,3,3,3,
3,3,3,3,3,3,3,3,3,3,3,3,3,3,3,3,3,3,3,3,3,3,4),(9.75973301747209E-8,0.0159118695155719,
0.0312500000000116,0.0468750000000174,0.0546875000000203,0.0585937500000218,
0.0623038556224994,0.0625000000000233,0.064880126691803,0.0838067325806669,
0.102671826588194,0.109375000000042,0.117187500000045,0.121093750000046,
0.123046875000047,0.124023437500047,0.124511718750048,0.125000000000048,
0.130903386642066,0.145647760556128,0.16030635703608,0.171875000000055,
0.179687500000056,0.183593750000057,0.185546875000057,0.186523437500057,
0.187500000000057,0.198318862785137,0.209096158356209,0.213486683424382,
0.224229801399845,0.234902287104572,0.242187500000057,0.246093750000057,
0.248046875000057,0.249023437500057,0.249755859375057,0.250000000000057,
0.286148785115262,0.331156930318982,0.373125773103967,0.413994518747176,
0.43750000000003,0.442035565805872,0.468750000000026,0.484375000000024,
0.492187500000022,0.496093750000022,0.498046875000022,0.498793771580626,
0.499023437500022,0.499511718750022,0.500000000000021,0.52780801953624,
0.555633916578266,0.58020272164201,0.608271007010268,0.634689717609213,
0.640624999999996,0.645733764714709,0.648437499999995,0.665743528084154,
0.677861217283039,0.695360989880092,0.712946719081514,0.730621384502898,
0.734374999999979,0.742187499999977,0.746093749999977,0.748046874999976,
0.749023437499976,0.749511718749976,0.749999999999976,0.752465380543056,
0.797962909276469,0.804120644423907,0.850530768471112,0.858778904853475,
0.906286042923783,0.920200820756934,0.968991302096034,0.993035530701956,
1.),.UNSPECIFIED.);
#217=B_SPLINE_CURVE_WITH_KNOTS('',3,(#49054,#49055,#49056,#49057,#49058,
#49059,#49060,#49061,#49062,#49063,#49064,#49065,#49066,#49067,#49068,#49069,
#49070,#49071,#49072,#49073,#49074,#49075,#49076,#49077,#49078,#49079,#49080,
#49081,#49082,#49083,#49084,#49085,#49086,#49087,#49088,#49089,#49090,#49091,
#49092,#49093,#49094,#49095,#49096,#49097,#49098,#49099,#49100,#49101,#49102,
#49103,#49104,#49105,#49106,#49107,#49108,#49109,#49110,#49111,#49112,#49113,
#49114,#49115,#49116,#49117,#49118,#49119,#49120,#49121,#49122,#49123,#49124,
#49125,#49126,#49127,#49128,#49129,#49130,#49131,#49132,#49133,#49134,#49135,
#49136,#49137,#49138,#49139,#49140,#49141,#49142,#49143,#49144,#49145,#49146,
#49147,#49148,#49149,#49150,#49151,#49152,#49153,#49154,#49155,#49156,#49157,
#49158,#49159,#49160,#49161,#49162,#49163,#49164,#49165,#49166,#49167,#49168,
#49169,#49170,#49171,#49172,#49173,#49174,#49175,#49176,#49177,#49178,#49179,
#49180,#49181,#49182,#49183,#49184,#49185,#49186,#49187,#49188,#49189,#49190,
#49191,#49192,#49193,#49194,#49195,#49196,#49197,#49198,#49199,#49200,#49201,
#49202,#49203,#49204,#49205,#49206,#49207,#49208,#49209,#49210),
 .UNSPECIFIED.,.F.,.F.,(4,3,3,3,3,3,3,3,3,3,3,3,3,3,3,3,3,3,3,3,3,3,3,3,
3,3,3,3,3,3,3,3,3,3,3,3,3,3,3,3,3,3,3,3,3,3,3,3,3,3,3,3,4),(1.72726539092123E-7,
0.043457309737723,0.0863338395015235,0.0932167347872756,0.124999999999967,
0.165840006934032,0.177273215764065,0.18749999999995,0.218749999999942,
0.234374999999937,0.242187499999935,0.246093749999934,0.249511718749934,
0.249999999999933,0.260113268690261,0.284904696510657,0.309601788337845,
0.31249999999994,0.336932312064704,0.343749999999943,0.359374999999945,
0.359741477424532,0.367187499999946,0.371093749999946,0.373046874999946,
0.374023437499947,0.374999999999947,0.427161972770903,0.437499999999952,
0.446539278308906,0.468749999999955,0.484374999999956,0.492187499999957,
0.499058228052342,0.499999999999957,0.52937268418032,0.595489014678813,
0.601624978398085,0.624999999999968,0.666787080930481,0.687499999999974,
0.718749999999976,0.726755041126725,0.734374999999978,0.746093749999979,
0.749999999999979,0.777565452150545,0.821930738816808,0.864144411456503,
0.906141574463173,0.949726410631746,0.995918599599637,0.999999956001335),
 .UNSPECIFIED.);
#218=B_SPLINE_CURVE_WITH_KNOTS('',3,(#49251,#49252,#49253,#49254,#49255,
#49256,#49257,#49258,#49259,#49260,#49261,#49262,#49263,#49264,#49265,#49266,
#49267,#49268,#49269,#49270,#49271,#49272,#49273,#49274,#49275,#49276,#49277,
#49278,#49279,#49280,#49281),.UNSPECIFIED.,.F.,.F.,(4,3,3,3,3,3,3,3,3,3,
4),(0.,0.125,0.1875,0.218750000000001,0.234375000000001,0.242187500000001,
0.250000000000001,0.375000000000001,0.500000000000001,0.75,1.),
 .UNSPECIFIED.);
#219=B_SPLINE_CURVE_WITH_KNOTS('',3,(#49283,#49284,#49285,#49286,#49287,
#49288,#49289,#49290,#49291,#49292,#49293,#49294,#49295,#49296,#49297,#49298,
#49299,#49300,#49301,#49302,#49303,#49304,#49305,#49306,#49307),
 .UNSPECIFIED.,.F.,.F.,(4,3,3,3,3,3,3,3,4),(0.,0.177032879059826,0.297841464654054,
0.477609256376899,0.5,0.682857180362573,0.863757928480276,0.887961286767199,
0.999997248082941),.UNSPECIFIED.);
#220=B_SPLINE_CURVE_WITH_KNOTS('',3,(#49310,#49311,#49312,#49313,#49314,
#49315,#49316,#49317,#49318,#49319,#49320,#49321,#49322,#49323,#49324,#49325,
#49326,#49327,#49328,#49329,#49330,#49331,#49332,#49333,#49334,#49335,#49336,
#49337,#49338,#49339,#49340,#49341,#49342,#49343,#49344,#49345,#49346,#49347,
#49348,#49349,#49350,#49351,#49352,#49353,#49354,#49355,#49356,#49357,#49358,
#49359,#49360,#49361,#49362,#49363,#49364,#49365,#49366,#49367,#49368,#49369,
#49370),.UNSPECIFIED.,.F.,.F.,(4,3,3,3,3,3,3,3,3,3,3,3,3,3,3,3,3,3,3,3,
4),(0.,0.106434110907981,0.221226834799591,0.249999999999998,0.31037540950159,
0.374999999999998,0.437499999999997,0.468749999999998,0.484374999999999,
0.494167919221464,0.5,0.510705335967005,0.592733299703605,0.670419047251969,
0.732755379993678,0.75,0.823662512114083,0.893640330195904,0.925951097491995,
0.992933814532853,0.99999999981018),.UNSPECIFIED.);
#221=B_SPLINE_CURVE_WITH_KNOTS('',3,(#49415,#49416,#49417,#49418,#49419,
#49420,#49421,#49422,#49423,#49424,#49425,#49426,#49427,#49428,#49429,#49430,
#49431,#49432,#49433,#49434,#49435,#49436,#49437,#49438,#49439,#49440,#49441,
#49442,#49443,#49444,#49445,#49446,#49447,#49448,#49449,#49450,#49451,#49452,
#49453,#49454,#49455,#49456,#49457,#49458,#49459,#49460,#49461,#49462,#49463,
#49464,#49465,#49466,#49467,#49468,#49469,#49470,#49471,#49472,#49473,#49474,
#49475,#49476,#49477,#49478,#49479,#49480,#49481,#49482,#49483,#49484),
 .UNSPECIFIED.,.F.,.F.,(4,3,3,3,3,3,3,3,3,3,3,3,3,3,3,3,3,3,3,3,3,3,3,4),
(1.12531523137531E-11,0.0435574969286064,0.0764692287957928,0.120152779061659,
0.125,0.178557276903457,0.223905113123066,0.25,0.318766865591617,0.371575001885328,
0.375,0.469117767069314,0.5,0.519436421805622,0.625,0.667313247416635,0.741709817797934,
0.75,0.808035688025396,0.814957802298849,0.875,0.919742785397221,0.96245146142866,
0.999999720290089),.UNSPECIFIED.);
#222=B_SPLINE_CURVE_WITH_KNOTS('',3,(#49485,#49486,#49487,#49488,#49489,
#49490,#49491,#49492,#49493,#49494,#49495,#49496,#49497,#49498,#49499,#49500,
#49501,#49502,#49503,#49504,#49505,#49506,#49507,#49508,#49509,#49510,#49511,
#49512,#49513,#49514,#49515,#49516,#49517,#49518,#49519,#49520,#49521,#49522,
#49523,#49524,#49525,#49526,#49527,#49528,#49529,#49530,#49531,#49532,#49533,
#49534,#49535,#49536,#49537,#49538,#49539,#49540,#49541,#49542,#49543,#49544,
#49545,#49546,#49547,#49548,#49549,#49550,#49551,#49552,#49553,#49554),
 .UNSPECIFIED.,.F.,.F.,(4,3,3,3,3,3,3,3,3,3,3,3,3,3,3,3,3,3,3,3,3,3,3,4),
(0.,0.0642447266186201,0.129222196775793,0.139648686470079,0.203363383249967,
0.250000000000004,0.300656411054288,0.369078205527147,0.437500000000007,
0.468750000000006,0.469711834217933,0.484375000000006,0.495155243842182,
0.500000000000006,0.563334858178523,0.625631040088055,0.644014782496406,
0.704247086115865,0.750000000000003,0.807879611466452,0.868482449145389,
0.928163587732209,0.96196228291215,0.999999992441464),.UNSPECIFIED.);
#223=B_SPLINE_CURVE_WITH_KNOTS('',3,(#49590,#49591,#49592,#49593,#49594,
#49595,#49596,#49597,#49598,#49599,#49600,#49601,#49602,#49603,#49604,#49605,
#49606,#49607,#49608,#49609,#49610,#49611,#49612,#49613,#49614,#49615,#49616,
#49617,#49618,#49619,#49620,#49621,#49622,#49623,#49624,#49625,#49626,#49627,
#49628,#49629,#49630,#49631,#49632,#49633,#49634,#49635,#49636,#49637,#49638,
#49639,#49640,#49641,#49642,#49643,#49644,#49645,#49646,#49647),
 .UNSPECIFIED.,.F.,.F.,(4,3,3,3,3,3,3,3,3,3,3,3,3,3,3,3,3,3,3,4),(1.7829606324839E-11,
0.0708213913417186,0.13721260991132,0.198853000409921,0.25,0.306729430221608,
0.362647740453726,0.418203642728849,0.473372817506931,0.5,0.500000496896627,
0.555649586140288,0.611781191912524,0.668290257959578,0.725514453399843,
0.75,0.8125,0.877125626676368,0.947977205464318,1.),.UNSPECIFIED.);
#224=B_SPLINE_CURVE_WITH_KNOTS('',3,(#49684,#49685,#49686,#49687,#49688,
#49689,#49690,#49691,#49692,#49693,#49694,#49695,#49696,#49697,#49698,#49699,
#49700,#49701,#49702,#49703,#49704,#49705,#49706,#49707,#49708,#49709,#49710,
#49711,#49712,#49713,#49714,#49715,#49716,#49717,#49718,#49719,#49720,#49721,
#49722,#49723,#49724,#49725,#49726,#49727,#49728,#49729,#49730,#49731,#49732,
#49733,#49734,#49735,#49736,#49737,#49738,#49739,#49740,#49741,#49742,#49743,
#49744,#49745,#49746,#49747,#49748,#49749,#49750,#49751,#49752,#49753,#49754,
#49755,#49756,#49757,#49758,#49759,#49760,#49761,#49762,#49763,#49764,#49765),
 .UNSPECIFIED.,.F.,.F.,(4,3,3,3,3,3,3,3,3,3,3,3,3,3,3,3,3,3,3,3,3,3,3,3,
3,3,3,4),(0.,0.0665074781408924,0.124999999999997,0.128587305872536,0.187499999999996,
0.218749999999995,0.234374999999995,0.242187499999995,0.246093749999995,
0.249999999999995,0.31357815937848,0.385910368691815,0.457052959592689,
0.499999999999993,0.500014077280664,0.570198395648231,0.624999999999993,
0.686457107520193,0.687499999999992,0.718749999999992,0.734374999999992,
0.742187499999992,0.746093749999992,0.749999999999992,0.813997647135706,
0.871428993161989,0.938277857776933,1.),.UNSPECIFIED.);
#225=B_SPLINE_CURVE_WITH_KNOTS('',3,(#49810,#49811,#49812,#49813,#49814,
#49815,#49816,#49817,#49818,#49819,#49820,#49821,#49822,#49823,#49824,#49825,
#49826,#49827,#49828,#49829,#49830,#49831,#49832,#49833,#49834),
 .UNSPECIFIED.,.F.,.F.,(4,3,3,3,3,3,3,3,4),(1.36947301852406E-7,0.18198259021518,
0.249918134546699,0.432569342894789,0.5,0.68030149702564,0.803687769765186,
0.980976573749724,0.999933076643282),.UNSPECIFIED.);
#226=B_SPLINE_CURVE_WITH_KNOTS('',3,(#49836,#49837,#49838,#49839,#49840,
#49841,#49842,#49843),.UNSPECIFIED.,.F.,.F.,(4,2,2,4),(-0.00420679853302169,
0.,0.0656255554488885,0.124431075933089),.UNSPECIFIED.);
#227=B_SPLINE_CURVE_WITH_KNOTS('',3,(#49844,#49845,#49846,#49847,#49848,
#49849,#49850,#49851,#49852,#49853,#49854,#49855,#49856,#49857,#49858,#49859,
#49860,#49861,#49862,#49863,#49864,#49865,#49866,#49867,#49868,#49869,#49870,
#49871,#49872,#49873,#49874,#49875,#49876,#49877,#49878,#49879,#49880,#49881,
#49882,#49883,#49884,#49885,#49886,#49887,#49888,#49889,#49890,#49891,#49892,
#49893,#49894,#49895,#49896,#49897,#49898,#49899,#49900,#49901),
 .UNSPECIFIED.,.F.,.F.,(4,3,3,3,3,3,3,3,3,3,3,3,3,3,3,3,3,3,3,4),(4.63074357751375E-6,
0.0537910573104376,0.124260671753383,0.198033873731291,0.202362264714046,
0.250000000000014,0.329872316171993,0.391843303964045,0.437500000000024,
0.468750000000025,0.484375000000024,0.492187500000023,0.498247326271446,
0.500000000000022,0.586936000013064,0.685649851920606,0.757785027674918,
0.860226013175883,0.934923100363294,0.999973164507014),.UNSPECIFIED.);
#228=B_SPLINE_CURVE_WITH_KNOTS('',3,(#49947,#49948,#49949,#49950,#49951,
#49952,#49953,#49954,#49955,#49956,#49957,#49958,#49959,#49960,#49961,#49962,
#49963,#49964,#49965,#49966,#49967,#49968,#49969,#49970,#49971,#49972,#49973,
#49974,#49975,#49976,#49977,#49978,#49979,#49980,#49981,#49982,#49983,#49984,
#49985,#49986,#49987,#49988,#49989,#49990,#49991,#49992,#49993,#49994,#49995,
#49996,#49997,#49998,#49999,#50000,#50001,#50002,#50003,#50004,#50005,#50006,
#50007,#50008,#50009,#50010,#50011,#50012,#50013,#50014,#50015,#50016,#50017,
#50018,#50019),.UNSPECIFIED.,.F.,.F.,(4,3,3,3,3,3,3,3,3,3,3,3,3,3,3,3,3,
3,3,3,3,3,3,3,4),(1.4541246487959E-9,0.0431191253455669,0.0863267720301174,
0.129382358811508,0.1428571428571,0.153643952151576,0.204633581280749,0.255730997948089,
0.2857142857143,0.306393509456684,0.370923699443645,0.4285714285714,0.459412017999017,
0.526893092613459,0.5714285714286,0.612488429046519,0.677675308052048,0.7142857142857,
0.765391329809934,0.81987081595669,0.8571428571429,0.900979334814105,0.918139369307915,
0.961788840323352,0.999999180955248),.UNSPECIFIED.);
#229=B_SPLINE_CURVE_WITH_KNOTS('',3,(#50022,#50023,#50024,#50025,#50026,
#50027,#50028,#50029,#50030,#50031,#50032,#50033,#50034,#50035,#50036,#50037,
#50038,#50039,#50040,#50041,#50042,#50043,#50044,#50045,#50046,#50047,#50048,
#50049,#50050,#50051,#50052,#50053,#50054,#50055,#50056,#50057,#50058,#50059,
#50060,#50061,#50062,#50063,#50064,#50065,#50066,#50067,#50068,#50069,#50070,
#50071,#50072,#50073,#50074,#50075,#50076,#50077,#50078,#50079,#50080,#50081,
#50082,#50083,#50084,#50085,#50086,#50087,#50088,#50089,#50090,#50091,#50092,
#50093,#50094),.UNSPECIFIED.,.F.,.F.,(4,3,3,3,3,3,3,3,3,3,3,3,3,3,3,3,3,
3,3,3,3,3,3,3,4),(0.,0.0558892577558595,0.112669247365332,0.156953409719216,
0.215052214438557,0.25000000000001,0.309316250903252,0.324310832292704,
0.385391022432193,0.437500000000018,0.468750000000019,0.48437500000002,
0.49218750000002,0.4989493455236,0.500000000000019,0.504583562497372,0.573408597222544,
0.641343712531288,0.680145778473015,0.75000000000001,0.815926534003008,
0.847891270040952,0.91466903667937,0.980716328284555,1.),.UNSPECIFIED.);
#230=B_SPLINE_CURVE_WITH_KNOTS('',3,(#50193,#50194,#50195,#50196,#50197,
#50198,#50199,#50200,#50201,#50202,#50203,#50204,#50205,#50206,#50207,#50208,
#50209,#50210,#50211,#50212,#50213,#50214,#50215,#50216,#50217,#50218,#50219,
#50220,#50221,#50222,#50223,#50224,#50225,#50226,#50227,#50228,#50229,#50230,
#50231,#50232,#50233,#50234,#50235,#50236,#50237,#50238,#50239,#50240,#50241,
#50242,#50243,#50244,#50245,#50246,#50247,#50248,#50249,#50250,#50251,#50252,
#50253,#50254,#50255,#50256,#50257,#50258,#50259,#50260,#50261,#50262,#50263,
#50264,#50265,#50266,#50267,#50268,#50269,#50270,#50271,#50272,#50273,#50274,
#50275,#50276,#50277,#50278,#50279,#50280,#50281,#50282,#50283,#50284,#50285,
#50286,#50287,#50288,#50289,#50290,#50291,#50292,#50293,#50294,#50295,#50296,
#50297,#50298,#50299,#50300,#50301,#50302,#50303,#50304,#50305,#50306,#50307,
#50308,#50309,#50310,#50311,#50312,#50313,#50314,#50315,#50316,#50317,#50318,
#50319,#50320,#50321,#50322,#50323,#50324,#50325,#50326,#50327,#50328,#50329,
#50330,#50331,#50332,#50333,#50334,#50335,#50336,#50337,#50338,#50339,#50340,
#50341,#50342,#50343,#50344,#50345,#50346,#50347,#50348,#50349,#50350,#50351,
#50352,#50353,#50354,#50355,#50356,#50357,#50358),.UNSPECIFIED.,.F.,.F.,
(4,3,3,3,3,3,3,3,3,3,3,3,3,3,3,3,3,3,3,3,3,3,3,3,3,3,3,3,3,3,3,3,3,3,3,
3,3,3,3,3,3,3,3,3,3,3,3,3,3,3,3,3,3,3,3,4),(8.91796462514105E-8,0.0341889233486022,
0.0625000000000075,0.0800235801072087,0.0937500000000111,0.109375000000013,
0.117187500000014,0.121093750000014,0.123046875000014,0.125000000000014,
0.156896093632204,0.187500000000017,0.218750000000019,0.234375000000019,
0.237544069789223,0.242187500000019,0.24609375000002,0.248046875000019,
0.250000000000019,0.290852976477788,0.312500000000018,0.328940100187335,
0.343750000000017,0.359375000000017,0.367187500000017,0.371093750000017,
0.373046875000017,0.375000000000017,0.425222667670205,0.437500000000015,
0.468750000000014,0.484375000000014,0.492187500000013,0.496093750000013,
0.500000000000013,0.520152742598536,0.572584836177622,0.616900729170795,
0.62500000000001,0.65134213620691,0.678251303075323,0.687500000000008,0.709160585412811,
0.750000000000007,0.781250000000006,0.789062500000006,0.796875000000006,
0.799072644259708,0.812500000000005,0.858399969519928,0.875000000000003,
0.885492836009458,0.932681943708858,0.98079009164065,0.98573093829117,1.),
 .UNSPECIFIED.);
#231=B_SPLINE_CURVE_WITH_KNOTS('',3,(#50361,#50362,#50363,#50364,#50365,
#50366,#50367,#50368,#50369,#50370,#50371,#50372,#50373,#50374,#50375,#50376,
#50377,#50378,#50379,#50380,#50381,#50382,#50383,#50384,#50385,#50386,#50387,
#50388,#50389,#50390,#50391,#50392,#50393,#50394,#50395,#50396,#50397,#50398,
#50399,#50400,#50401,#50402,#50403,#50404,#50405,#50406,#50407,#50408,#50409,
#50410,#50411,#50412,#50413,#50414,#50415,#50416,#50417,#50418,#50419,#50420,
#50421,#50422,#50423,#50424,#50425,#50426,#50427,#50428,#50429,#50430,#50431,
#50432,#50433,#50434,#50435,#50436,#50437,#50438,#50439,#50440,#50441,#50442,
#50443,#50444,#50445,#50446,#50447,#50448,#50449,#50450,#50451,#50452,#50453,
#50454,#50455,#50456,#50457,#50458,#50459,#50460,#50461,#50462,#50463,#50464,
#50465,#50466,#50467,#50468,#50469,#50470,#50471,#50472,#50473,#50474,#50475,
#50476,#50477,#50478,#50479,#50480,#50481,#50482,#50483,#50484,#50485,#50486,
#50487,#50488,#50489,#50490,#50491,#50492,#50493,#50494,#50495,#50496,#50497,
#50498,#50499,#50500,#50501,#50502),.UNSPECIFIED.,.F.,.F.,(4,3,3,3,3,3,
3,3,3,3,3,3,3,3,3,3,3,3,3,3,3,3,3,3,3,3,3,3,3,3,3,3,3,3,3,3,3,3,3,3,3,3,
3,3,3,3,3,4),(2.34637988656816E-7,0.0315958274976916,0.0628964687251239,
0.0937122522318575,0.104172143984534,0.125,0.154837231987697,0.184674463975394,
0.213175784027995,0.218750000000001,0.234375000000001,0.242187500000001,
0.246093750000001,0.248046875000001,0.250000000000001,0.257790373752442,
0.295642404285767,0.33448340003201,0.354334938238437,0.392683239873593,
0.431398964572153,0.4704820316817,0.482378819405289,0.484374999999999,0.49658582239736,
0.499999999999999,0.540377618081788,0.580372330237114,0.609456768302146,
0.64916758132608,0.687499999999997,0.700832885131154,0.718749999999997,
0.734374999999997,0.742187499999997,0.746093749999997,0.748046874999997,
0.749999999999997,0.769091927835171,0.798967073430337,0.828842219025503,
0.858577125548687,0.874999999999998,0.896782376980454,0.927914312513236,
0.959582512827434,0.985641744950711,1.),.UNSPECIFIED.);
#232=B_SPLINE_CURVE_WITH_KNOTS('',3,(#50539,#50540,#50541,#50542,#50543,
#50544,#50545,#50546,#50547,#50548,#50549,#50550,#50551,#50552,#50553,#50554,
#50555,#50556,#50557,#50558,#50559,#50560,#50561,#50562,#50563,#50564,#50565,
#50566,#50567,#50568,#50569,#50570,#50571,#50572,#50573,#50574,#50575,#50576,
#50577,#50578,#50579,#50580,#50581,#50582,#50583,#50584,#50585,#50586,#50587,
#50588,#50589,#50590,#50591,#50592,#50593,#50594,#50595,#50596,#50597,#50598,
#50599),.UNSPECIFIED.,.F.,.F.,(4,3,3,3,3,3,3,3,3,3,3,3,3,3,3,3,3,3,3,3,
4),(3.81436954511069E-8,0.0594692266925058,0.119461338390937,0.180335235503925,
0.228233344473427,0.250000000000001,0.312500000000001,0.375000000000001,
0.420629555808829,0.466480510808558,0.500000000000001,0.532982686561363,
0.59558437717701,0.657507300746284,0.718468600168369,0.750000000000001,
0.809830738944292,0.831293936966436,0.890887168088582,0.94959438235366,
1.),.UNSPECIFIED.);
#233=B_SPLINE_CURVE_WITH_KNOTS('',3,(#50600,#50601,#50602,#50603,#50604,
#50605,#50606,#50607,#50608,#50609,#50610,#50611,#50612,#50613,#50614,#50615,
#50616,#50617,#50618,#50619,#50620,#50621,#50622,#50623,#50624,#50625,#50626,
#50627,#50628,#50629,#50630,#50631,#50632,#50633,#50634,#50635,#50636,#50637,
#50638,#50639,#50640,#50641,#50642,#50643,#50644,#50645,#50646,#50647,#50648,
#50649,#50650,#50651,#50652,#50653,#50654,#50655,#50656,#50657),
 .UNSPECIFIED.,.F.,.F.,(4,3,3,3,3,3,3,3,3,3,3,3,3,3,3,3,3,3,3,4),(0.,0.07023511355664,
0.136204759980801,0.197546204775853,0.25,0.308361863568339,0.365828750984795,
0.422887295093721,0.479509854680895,0.5,0.500088874817559,0.555696428953905,
0.611747912029764,0.668153881503749,0.725240099299435,0.75,0.8125,0.87677552836491,
0.947109081823081,1.),.UNSPECIFIED.);
#234=B_SPLINE_CURVE_WITH_KNOTS('',3,(#50703,#50704,#50705,#50706,#50707,
#50708,#50709,#50710,#50711,#50712,#50713,#50714,#50715,#50716,#50717,#50718,
#50719,#50720,#50721,#50722,#50723,#50724,#50725,#50726,#50727,#50728,#50729,
#50730,#50731,#50732,#50733,#50734,#50735,#50736,#50737,#50738,#50739,#50740,
#50741,#50742,#50743,#50744,#50745,#50746,#50747,#50748,#50749,#50750,#50751,
#50752,#50753,#50754,#50755,#50756,#50757,#50758,#50759,#50760),
 .UNSPECIFIED.,.F.,.F.,(4,3,3,3,3,3,3,3,3,3,3,3,3,3,3,3,3,3,3,4),(0.,0.0625,
0.123429255825999,0.183419343641415,0.242355359067083,0.25,0.308040972645323,
0.36533838298242,0.422299344729593,0.479067050605816,0.535783675525185,
0.592776687427881,0.649990213922836,0.707861096511507,0.75,0.808903293455612,
0.869154047623437,0.930297220487149,0.99290670407742,1.),.UNSPECIFIED.);
#235=B_SPLINE_CURVE_WITH_KNOTS('',3,(#50761,#50762,#50763,#50764,#50765,
#50766,#50767,#50768,#50769,#50770,#50771,#50772,#50773,#50774,#50775,#50776,
#50777,#50778,#50779,#50780,#50781,#50782,#50783,#50784,#50785,#50786,#50787,
#50788,#50789,#50790,#50791,#50792,#50793,#50794,#50795,#50796,#50797,#50798,
#50799,#50800,#50801,#50802,#50803,#50804,#50805,#50806,#50807,#50808,#50809,
#50810,#50811,#50812,#50813,#50814,#50815,#50816,#50817,#50818,#50819,#50820,
#50821,#50822,#50823,#50824,#50825,#50826,#50827,#50828,#50829,#50830,#50831,
#50832,#50833,#50834,#50835,#50836,#50837,#50838,#50839,#50840,#50841,#50842,
#50843,#50844,#50845,#50846,#50847,#50848,#50849,#50850,#50851,#50852,#50853,
#50854),.UNSPECIFIED.,.F.,.F.,(4,3,3,3,3,3,3,3,3,3,3,3,3,3,3,3,3,3,3,3,
3,3,3,3,3,3,3,3,3,3,3,4),(0.,0.00526477685132137,0.0911120621260249,0.124999999999999,
0.164492696482799,0.187499999999998,0.218749999999998,0.234374999999998,
0.242187499999998,0.246093749999998,0.248046874999998,0.249999999999997,
0.315561405830368,0.332546042754748,0.397233658308089,0.461991812577509,
0.499894561889816,0.499999999999991,0.564586350481157,0.624999999999988,
0.667250942464425,0.687499999999987,0.718749999999986,0.734374999999985,
0.742187499999985,0.746093749999985,0.748046874999985,0.749999999999985,
0.83529834404552,0.918975525864169,0.994552082753247,1.),.UNSPECIFIED.);
#236=B_SPLINE_CURVE_WITH_KNOTS('',3,(#50897,#50898,#50899,#50900,#50901,
#50902,#50903,#50904,#50905,#50906,#50907,#50908,#50909,#50910,#50911,#50912,
#50913,#50914,#50915,#50916,#50917,#50918,#50919,#50920,#50921,#50922,#50923,
#50924,#50925,#50926,#50927),.UNSPECIFIED.,.F.,.F.,(4,3,3,3,3,3,3,3,3,3,
4),(0.,0.124999999999993,0.18749999999999,0.218749999999989,0.234374999999987,
0.242187499999987,0.249999999999986,0.374999999999988,0.49999999999999,
0.749999999999995,1.),.UNSPECIFIED.);
#237=B_SPLINE_CURVE_WITH_KNOTS('',3,(#50928,#50929,#50930,#50931,#50932,
#50933,#50934,#50935,#50936,#50937,#50938,#50939,#50940,#50941,#50942,#50943,
#50944,#50945,#50946,#50947,#50948,#50949,#50950,#50951,#50952),
 .UNSPECIFIED.,.F.,.F.,(4,3,3,3,3,3,3,3,4),(0.,0.177256629021432,0.214956465801327,
0.395210606083471,0.5,0.682544097815536,0.772277414116928,0.954142569649918,
0.999999140627182),.UNSPECIFIED.);
#238=B_SPLINE_CURVE_WITH_KNOTS('',3,(#50953,#50954,#50955,#50956,#50957,
#50958,#50959,#50960,#50961,#50962,#50963,#50964,#50965,#50966,#50967,#50968,
#50969,#50970,#50971,#50972,#50973,#50974,#50975,#50976,#50977,#50978,#50979,
#50980,#50981,#50982,#50983,#50984,#50985,#50986,#50987,#50988,#50989,#50990,
#50991,#50992,#50993,#50994,#50995,#50996,#50997,#50998,#50999,#51000,#51001,
#51002,#51003,#51004,#51005,#51006,#51007,#51008,#51009,#51010,#51011,#51012,
#51013),.UNSPECIFIED.,.F.,.F.,(4,3,3,3,3,3,3,3,3,3,3,3,3,3,3,3,3,3,3,3,
4),(1.28199134739398E-10,0.070962309054426,0.173238035306535,0.248450970868743,
0.25,0.348335417086408,0.41932009272992,0.437499999999997,0.468749999999996,
0.484374999999996,0.492187499999996,0.497900248415515,0.499999999999997,
0.583530657236138,0.616659679343955,0.696381996825757,0.749999999999998,
0.804571254699382,0.878158467774757,0.951745680850132,0.999999999996763),
 .UNSPECIFIED.);
#239=B_SPLINE_CURVE_WITH_KNOTS('',3,(#51056,#51057,#51058,#51059,#51060,
#51061,#51062,#51063,#51064,#51065,#51066,#51067,#51068,#51069,#51070,#51071,
#51072,#51073,#51074,#51075,#51076,#51077,#51078,#51079,#51080,#51081,#51082,
#51083,#51084,#51085,#51086,#51087,#51088,#51089,#51090,#51091,#51092,#51093,
#51094,#51095,#51096,#51097,#51098,#51099,#51100,#51101,#51102,#51103,#51104,
#51105,#51106,#51107,#51108,#51109,#51110,#51111,#51112,#51113,#51114,#51115,
#51116,#51117,#51118,#51119,#51120,#51121,#51122,#51123,#51124,#51125,#51126,
#51127,#51128,#51129,#51130,#51131,#51132,#51133,#51134,#51135,#51136,#51137,
#51138,#51139,#51140,#51141,#51142,#51143,#51144,#51145,#51146),
 .UNSPECIFIED.,.F.,.F.,(4,3,3,3,3,3,3,3,3,3,3,3,3,3,3,3,3,3,3,3,3,3,3,3,
3,3,3,3,3,3,4),(1.98906495286848E-7,0.0470898563921683,0.0950876937980486,
0.109526430295898,0.125,0.176684971632146,0.1875,0.195574841813231,0.203125,
0.21875,0.25,0.270621653555496,0.334104133193722,0.398265383295987,0.430414688308331,
0.4375,0.46875,0.484375,0.4921875,0.498034123291998,0.500000000000001,0.559924704434065,
0.600124957473912,0.658475263308525,0.715889338441014,0.764250567660699,
0.8218499773925,0.878616139622934,0.918178964193708,0.970962436356723,1.),
 .UNSPECIFIED.);
#240=B_SPLINE_CURVE_WITH_KNOTS('',3,(#51197,#51198,#51199,#51200,#51201,
#51202,#51203,#51204,#51205,#51206,#51207,#51208,#51209,#51210,#51211,#51212,
#51213,#51214,#51215,#51216,#51217,#51218,#51219,#51220,#51221),
 .UNSPECIFIED.,.F.,.F.,(4,3,3,3,3,3,3,3,4),(8.00074943874998E-8,0.150887609476909,
0.211670949228306,0.3333333333333,0.508675768769221,0.623916433730383,0.6666666666667,
0.83333333333335,1.),.UNSPECIFIED.);
#241=B_SPLINE_CURVE_WITH_KNOTS('',3,(#51223,#51224,#51225,#51226,#51227,
#51228,#51229,#51230,#51231,#51232,#51233),.UNSPECIFIED.,.F.,.F.,(4,1,2,
2,2,4),(0.,0.124999999999996,0.218749999999993,0.249999999999992,0.499999999999995,
1.),.UNSPECIFIED.);
#242=B_SPLINE_CURVE_WITH_KNOTS('',3,(#51234,#51235,#51236,#51237,#51238,
#51239,#51240,#51241,#51242,#51243,#51244,#51245,#51246,#51247,#51248,#51249,
#51250,#51251,#51252,#51253,#51254,#51255,#51256,#51257,#51258,#51259,#51260,
#51261,#51262,#51263,#51264,#51265,#51266,#51267,#51268,#51269,#51270,#51271,
#51272,#51273,#51274,#51275,#51276,#51277,#51278,#51279,#51280,#51281,#51282,
#51283,#51284,#51285,#51286,#51287,#51288),.UNSPECIFIED.,.F.,.F.,(4,3,3,
3,3,3,3,3,3,3,3,3,3,3,3,3,3,3,4),(0.,0.0544322267884975,0.110762977555986,
0.168281172499134,0.227824949411008,0.250000000000006,0.315494399733559,
0.375000000000008,0.43750000000001,0.468750000000011,0.484375000000011,
0.494989881597992,0.500000000000011,0.59005681178326,0.685607308844679,
0.783754001548365,0.886959143600766,0.972258800028934,1.),.UNSPECIFIED.);
#243=B_SPLINE_CURVE_WITH_KNOTS('',3,(#51330,#51331,#51332,#51333,#51334,
#51335,#51336,#51337,#51338,#51339,#51340,#51341,#51342,#51343,#51344,#51345,
#51346,#51347,#51348,#51349,#51350,#51351,#51352,#51353,#51354,#51355,#51356,
#51357,#51358,#51359,#51360,#51361,#51362,#51363,#51364,#51365,#51366,#51367,
#51368,#51369,#51370,#51371,#51372,#51373,#51374,#51375,#51376,#51377,#51378,
#51379,#51380,#51381,#51382,#51383,#51384,#51385,#51386,#51387,#51388,#51389,
#51390,#51391,#51392,#51393,#51394,#51395,#51396,#51397,#51398,#51399,#51400,
#51401,#51402,#51403,#51404,#51405,#51406,#51407,#51408,#51409,#51410,#51411,
#51412,#51413,#51414,#51415,#51416,#51417),.UNSPECIFIED.,.F.,.F.,(4,3,3,
3,3,3,3,3,3,3,3,3,3,3,3,3,3,3,3,3,3,3,3,3,3,3,3,3,3,4),(0.,0.0527820095289333,
0.0818213288309768,0.138473111371745,0.195945206951966,0.235750026621739,
0.293012168939004,0.351193384242706,0.399875448565708,0.437500000000007,
0.468750000000007,0.484375000000007,0.492187500000006,0.496093750000006,
0.499508594967082,0.500000000000006,0.565860739773587,0.629574808670008,
0.693958741288855,0.725750998861238,0.781250000000002,0.790730932595577,
0.796875000000001,0.812500000000001,0.869044093253454,0.875000000000001,
0.884835905848476,0.938701632182115,0.99336215698859,0.999999777714142),
 .UNSPECIFIED.);
#244=B_SPLINE_CURVE_WITH_KNOTS('',3,(#51420,#51421,#51422,#51423,#51424,
#51425,#51426,#51427,#51428,#51429,#51430,#51431,#51432,#51433,#51434,#51435,
#51436,#51437,#51438,#51439,#51440,#51441,#51442,#51443,#51444,#51445,#51446,
#51447,#51448,#51449,#51450,#51451,#51452,#51453,#51454,#51455,#51456,#51457,
#51458,#51459,#51460,#51461,#51462,#51463,#51464,#51465,#51466,#51467,#51468,
#51469,#51470,#51471,#51472,#51473,#51474,#51475,#51476,#51477),
 .UNSPECIFIED.,.F.,.F.,(4,3,3,3,3,3,3,3,3,3,3,3,3,3,3,3,3,3,3,4),(8.78525880136469E-7,
0.0585642409233348,0.117997885332985,0.168707876010783,0.228541702004436,
0.25,0.3125,0.375,0.421054242624552,0.467108485249104,0.5,0.563532905950584,
0.626399542664273,0.688223267168837,0.75,0.771768826617254,0.83260586843843,
0.892881435436045,0.952306996196428,0.999999961863698),.UNSPECIFIED.);
#245=B_SPLINE_CURVE_WITH_KNOTS('',3,(#51528,#51529,#51530,#51531,#51532,
#51533,#51534,#51535,#51536,#51537,#51538,#51539,#51540,#51541,#51542,#51543,
#51544,#51545,#51546,#51547,#51548,#51549,#51550,#51551,#51552,#51553,#51554,
#51555,#51556,#51557,#51558,#51559,#51560,#51561,#51562,#51563,#51564,#51565,
#51566,#51567,#51568,#51569,#51570,#51571,#51572,#51573,#51574,#51575,#51576,
#51577,#51578,#51579,#51580,#51581,#51582,#51583,#51584,#51585,#51586,#51587,
#51588,#51589,#51590,#51591,#51592,#51593,#51594,#51595,#51596,#51597,#51598,
#51599,#51600,#51601,#51602,#51603,#51604,#51605,#51606,#51607,#51608,#51609,
#51610,#51611,#51612,#51613,#51614,#51615,#51616,#51617,#51618,#51619,#51620,
#51621,#51622,#51623,#51624,#51625,#51626,#51627,#51628,#51629,#51630,#51631,
#51632,#51633,#51634,#51635,#51636,#51637,#51638,#51639,#51640,#51641,#51642,
#51643,#51644,#51645,#51646,#51647,#51648,#51649,#51650,#51651,#51652,#51653,
#51654,#51655,#51656,#51657,#51658,#51659,#51660,#51661,#51662,#51663,#51664,
#51665,#51666,#51667,#51668,#51669,#51670,#51671,#51672,#51673,#51674,#51675,
#51676,#51677,#51678,#51679,#51680,#51681,#51682,#51683,#51684,#51685,#51686,
#51687,#51688,#51689,#51690,#51691,#51692,#51693,#51694,#51695,#51696,#51697,
#51698,#51699,#51700,#51701,#51702,#51703,#51704,#51705,#51706,#51707,#51708,
#51709,#51710,#51711,#51712,#51713,#51714,#51715,#51716,#51717,#51718,#51719,
#51720,#51721,#51722,#51723,#51724,#51725,#51726,#51727,#51728,#51729,#51730,
#51731,#51732,#51733,#51734,#51735,#51736,#51737,#51738,#51739,#51740,#51741,
#51742,#51743,#51744,#51745,#51746,#51747,#51748,#51749,#51750,#51751,#51752,
#51753,#51754,#51755,#51756,#51757,#51758,#51759,#51760,#51761,#51762,#51763,
#51764,#51765,#51766,#51767,#51768,#51769,#51770,#51771),.UNSPECIFIED.,
 .F.,.F.,(4,3,3,3,3,3,3,3,3,3,3,3,3,3,3,3,3,3,3,3,3,3,3,3,3,3,3,3,3,3,3,
3,3,3,3,3,3,3,3,3,3,3,3,3,3,3,3,3,3,3,3,3,3,3,3,3,3,3,3,3,3,3,3,3,3,3,3,
3,3,3,3,3,3,3,3,3,3,3,3,3,3,4),(9.75974323886041E-8,0.0159118694038098,
0.031250000000004,0.0468750000000061,0.0546875000000072,0.0585937500000077,
0.0623038553748027,0.0625000000000082,0.064880126712784,0.0838067330365208,
0.102671827483111,0.109375000000014,0.117187500000015,0.121093750000015,
0.123046875000016,0.124023437500016,0.124511718750016,0.125000000000016,
0.130903386566927,0.14564776013408,0.160306356267678,0.171875000000023,
0.179687500000024,0.183593750000025,0.185546875000025,0.186523437500025,
0.187500000000025,0.198318863007,0.209096158798105,0.213486682905972,0.224229801102837,
0.234902287027138,0.242187500000032,0.246093750000033,0.248046875000033,
0.249023437500033,0.249755859375033,0.250000000000033,0.28614878553653,
0.331156929523491,0.373125773860353,0.413936165812502,0.442035566291532,
0.468750000000073,0.484375000000075,0.492187500000077,0.496093750000077,
0.498046875000078,0.49879377159272,0.499023437500078,0.499511718750078,
0.500000000000078,0.527808016721212,0.555633910969737,0.580202724032766,
0.608271006625457,0.634689718024949,0.640625000000101,0.645733762002606,
0.648437500000103,0.665743521005006,0.677861205829731,0.695360971298973,
0.712946693311888,0.730621351505351,0.734375000000116,0.742187500000117,
0.746093750000118,0.748046875000119,0.749023437500118,0.749511718750118,
0.750000000000118,0.752465380464155,0.797962909864778,0.804120644560384,
0.850530769082291,0.858778905128583,0.906286043966465,0.920200821048477,
0.968991302762396,0.99303553074547,1.),.UNSPECIFIED.);
#246=B_SPLINE_CURVE_WITH_KNOTS('',3,(#51854,#51855,#51856,#51857,#51858,
#51859,#51860,#51861,#51862,#51863,#51864,#51865,#51866,#51867,#51868,#51869,
#51870,#51871,#51872,#51873,#51874,#51875,#51876,#51877,#51878,#51879,#51880,
#51881,#51882,#51883,#51884,#51885,#51886,#51887,#51888,#51889,#51890,#51891,
#51892,#51893,#51894,#51895,#51896,#51897,#51898,#51899,#51900,#51901,#51902,
#51903,#51904,#51905,#51906,#51907,#51908,#51909,#51910,#51911,#51912,#51913,
#51914,#51915,#51916,#51917,#51918,#51919,#51920,#51921,#51922,#51923,#51924,
#51925,#51926,#51927,#51928,#51929,#51930,#51931,#51932,#51933,#51934,#51935,
#51936,#51937,#51938,#51939,#51940,#51941,#51942,#51943,#51944,#51945,#51946,
#51947,#51948,#51949,#51950,#51951,#51952,#51953,#51954,#51955,#51956,#51957,
#51958,#51959,#51960,#51961,#51962,#51963,#51964,#51965,#51966,#51967,#51968,
#51969,#51970,#51971,#51972,#51973,#51974,#51975,#51976,#51977,#51978,#51979,
#51980,#51981,#51982,#51983,#51984,#51985,#51986,#51987,#51988,#51989,#51990,
#51991,#51992,#51993,#51994,#51995,#51996,#51997,#51998,#51999,#52000,#52001,
#52002,#52003,#52004,#52005,#52006,#52007,#52008,#52009,#52010),
 .UNSPECIFIED.,.F.,.F.,(4,3,3,3,3,3,3,3,3,3,3,3,3,3,3,3,3,3,3,3,3,3,3,3,
3,3,3,3,3,3,3,3,3,3,3,3,3,3,3,3,3,3,3,3,3,3,3,3,3,3,3,3,4),(1.72726422180961E-7,
0.0434573104264856,0.0863338408497661,0.0932167342994617,0.125000000000013,
0.165840007447092,0.177273215395186,0.18750000000002,0.218750000000023,
0.234375000000024,0.242187500000025,0.246093750000026,0.249511718750026,
0.250000000000026,0.260113267055131,0.284904699064489,0.309601795003255,
0.312500000000022,0.336932316022879,0.34375000000002,0.359375000000019,
0.359741476131033,0.367187500000018,0.371093750000018,0.373046875000018,
0.374023437500018,0.375000000000018,0.427161996877003,0.437500000000016,
0.446539280842715,0.468750000000016,0.484375000000016,0.492187500000015,
0.49905823116347,0.500000000000015,0.529372684176819,0.595489014668126,
0.601624978392567,0.625000000000013,0.66678708092323,0.687500000000012,
0.718750000000011,0.726755041117905,0.734375000000011,0.746093750000011,
0.750000000000011,0.777565452151945,0.821930738832105,0.864144411482225,
0.906141574496073,0.949726410668509,0.995918599635573,0.999999956010348),
 .UNSPECIFIED.);
#247=B_SPLINE_CURVE_WITH_KNOTS('',3,(#52055,#52056,#52057,#52058,#52059,
#52060,#52061,#52062,#52063,#52064,#52065,#52066,#52067,#52068,#52069,#52070,
#52071,#52072,#52073,#52074,#52075,#52076,#52077,#52078,#52079,#52080,#52081,
#52082,#52083,#52084,#52085),.UNSPECIFIED.,.F.,.F.,(4,3,3,3,3,3,3,3,3,3,
4),(0.,0.124999999999999,0.187499999999999,0.218750000000001,0.234375000000003,
0.242187500000003,0.250000000000002,0.375000000000001,0.5,0.75,1.),
 .UNSPECIFIED.);
#248=B_SPLINE_CURVE_WITH_KNOTS('',3,(#52087,#52088,#52089,#52090,#52091,
#52092,#52093,#52094,#52095,#52096,#52097,#52098,#52099,#52100,#52101,#52102,
#52103,#52104,#52105,#52106,#52107,#52108,#52109,#52110,#52111),
 .UNSPECIFIED.,.F.,.F.,(4,3,3,3,3,3,3,3,4),(0.,0.16666666666665,0.3333333333333,
0.34683559518902,0.517983212474509,0.6666666666667,0.757476212651963,0.908784227355494,
1.),.UNSPECIFIED.);
#249=B_SPLINE_CURVE_WITH_KNOTS('',3,(#52114,#52115,#52116,#52117,#52118,
#52119,#52120,#52121,#52122,#52123,#52124,#52125,#52126,#52127,#52128,#52129,
#52130,#52131,#52132,#52133,#52134,#52135,#52136,#52137,#52138,#52139,#52140,
#52141,#52142,#52143,#52144,#52145,#52146,#52147,#52148,#52149,#52150,#52151,
#52152,#52153,#52154,#52155,#52156,#52157,#52158,#52159,#52160,#52161,#52162,
#52163,#52164,#52165,#52166,#52167,#52168,#52169,#52170,#52171),
 .UNSPECIFIED.,.F.,.F.,(4,3,3,3,3,3,3,3,3,3,3,3,3,3,3,3,3,3,3,4),(0.,0.105109524119636,
0.210219048239273,0.250000000000008,0.34862072745125,0.375000000000012,
0.437500000000015,0.468750000000017,0.484375000000017,0.495049246442063,
0.500000000000017,0.569750769769646,0.637746941740444,0.703349698996779,
0.750000000000009,0.812499999999997,0.86990370050903,0.926035857903304,
0.980615255774514,0.999999999999961),.UNSPECIFIED.);
#250=B_SPLINE_CURVE_WITH_KNOTS('',3,(#52216,#52217,#52218,#52219,#52220,
#52221,#52222,#52223,#52224,#52225,#52226,#52227,#52228,#52229,#52230,#52231,
#52232,#52233,#52234,#52235,#52236,#52237,#52238,#52239,#52240,#52241,#52242,
#52243,#52244,#52245,#52246,#52247,#52248,#52249,#52250,#52251,#52252,#52253,
#52254,#52255,#52256,#52257,#52258,#52259,#52260,#52261,#52262,#52263,#52264,
#52265,#52266,#52267,#52268,#52269,#52270,#52271,#52272,#52273,#52274,#52275,
#52276,#52277,#52278,#52279,#52280,#52281,#52282,#52283,#52284,#52285),
 .UNSPECIFIED.,.F.,.F.,(4,3,3,3,3,3,3,3,3,3,3,3,3,3,3,3,3,3,3,3,3,3,3,4),
(0.,0.0435526678755794,0.0764717462981114,0.120149499615019,0.125,0.178506530376304,
0.223907959984569,0.25,0.31871927758898,0.371577094927995,0.375,0.469063824151086,
0.5,0.519438184278401,0.625,0.667314605350398,0.741711751481222,0.75,0.808035504284208,
0.814958211926088,0.875,0.919742637241602,0.962451077979713,0.999999720285091),
 .UNSPECIFIED.);
#251=B_SPLINE_CURVE_WITH_KNOTS('',3,(#52286,#52287,#52288,#52289,#52290,
#52291,#52292,#52293,#52294,#52295,#52296,#52297,#52298,#52299,#52300,#52301,
#52302,#52303,#52304,#52305,#52306,#52307,#52308,#52309,#52310,#52311,#52312,
#52313,#52314,#52315,#52316,#52317,#52318,#52319,#52320,#52321,#52322,#52323,
#52324,#52325,#52326,#52327,#52328,#52329,#52330,#52331,#52332,#52333,#52334,
#52335,#52336,#52337,#52338,#52339,#52340,#52341,#52342,#52343,#52344,#52345,
#52346,#52347,#52348,#52349,#52350,#52351,#52352,#52353,#52354,#52355),
 .UNSPECIFIED.,.F.,.F.,(4,3,3,3,3,3,3,3,3,3,3,3,3,3,3,3,3,3,3,3,3,3,3,4),
(1.03865533685802E-6,0.0642465706088212,0.129224553569229,0.139648939065381,
0.203364160200743,0.249999999999996,0.300656465499399,0.369078232749696,
0.437499999999993,0.468749999999993,0.469711939585008,0.484374999999993,
0.495154941811767,0.499999999999992,0.563334700450325,0.625630715657075,
0.644015096124142,0.704247231797919,0.749999999999996,0.807879474143196,
0.86848214525923,0.928163112418586,0.961961792804727,0.999999992445085),
 .UNSPECIFIED.);
#252=B_SPLINE_CURVE_WITH_KNOTS('',3,(#52391,#52392,#52393,#52394,#52395,
#52396,#52397,#52398,#52399,#52400,#52401,#52402,#52403,#52404,#52405,#52406,
#52407,#52408,#52409,#52410,#52411,#52412,#52413,#52414,#52415,#52416,#52417,
#52418,#52419,#52420,#52421,#52422,#52423,#52424,#52425,#52426,#52427,#52428,
#52429,#52430,#52431,#52432,#52433,#52434,#52435,#52436,#52437,#52438,#52439,
#52440,#52441,#52442,#52443,#52444,#52445,#52446,#52447,#52448),
 .UNSPECIFIED.,.F.,.F.,(4,3,3,3,3,3,3,3,3,3,3,3,3,3,3,3,3,3,3,4),(1.80896803019825E-6,
0.0702777913312772,0.136276551999961,0.197638148831127,0.25,0.306990176879288,
0.363185832858698,0.419028057645599,0.47449970114341,0.5,0.500063301622431,
0.555684146132839,0.611743964881915,0.668155434484592,0.725242836573191,
0.75,0.812499421639319,0.876725635073414,0.946985306096238,0.999997686557278),
 .UNSPECIFIED.);
#253=B_SPLINE_CURVE_WITH_KNOTS('',3,(#52493,#52494,#52495,#52496,#52497,
#52498,#52499,#52500,#52501,#52502,#52503,#52504,#52505,#52506,#52507,#52508,
#52509,#52510,#52511,#52512,#52513,#52514,#52515,#52516,#52517,#52518,#52519,
#52520,#52521,#52522,#52523,#52524,#52525,#52526,#52527,#52528,#52529,#52530,
#52531,#52532,#52533,#52534,#52535,#52536,#52537,#52538,#52539,#52540,#52541,
#52542,#52543,#52544,#52545,#52546,#52547,#52548,#52549,#52550,#52551,#52552,
#52553,#52554,#52555,#52556,#52557,#52558,#52559,#52560,#52561,#52562,#52563,
#52564,#52565,#52566,#52567,#52568,#52569,#52570,#52571,#52572,#52573,#52574,
#52575,#52576,#52577),.UNSPECIFIED.,.F.,.F.,(4,3,3,3,3,3,3,3,3,3,3,3,3,
3,3,3,3,3,3,3,3,3,3,3,3,3,3,3,4),(3.09998686814312E-6,0.071014663091211,
0.124999999999999,0.187499999999998,0.218749999999998,0.234374999999998,
0.242187499999998,0.246093749999998,0.249999999999998,0.307063177457838,
0.363609740399054,0.40239397193843,0.458356131953603,0.499999999999998,
0.55592354852836,0.61211112871015,0.624999999999998,0.681633993337571,0.687499999999998,
0.718749999999998,0.734374999999998,0.742187499999998,0.746093749999998,
0.749999999999998,0.817242329244051,0.886254599421192,0.923154825582442,
0.994899550913029,0.999994036117558),.UNSPECIFIED.);
#254=B_SPLINE_CURVE_WITH_KNOTS('',3,(#52620,#52621,#52622,#52623,#52624,
#52625,#52626,#52627,#52628,#52629,#52630,#52631,#52632,#52633,#52634,#52635,
#52636,#52637,#52638,#52639,#52640,#52641,#52642,#52643,#52644,#52645,#52646,
#52647,#52648,#52649,#52650,#52651,#52652,#52653,#52654,#52655,#52656,#52657,
#52658,#52659,#52660,#52661,#52662,#52663,#52664,#52665,#52666,#52667,#52668,
#52669,#52670,#52671,#52672,#52673,#52674,#52675,#52676,#52677),
 .UNSPECIFIED.,.F.,.F.,(4,3,3,3,3,3,3,3,3,3,3,3,3,3,3,3,3,3,3,4),(1.9911764389659E-11,
0.0625000000149338,0.123437488775076,0.183435355664403,0.242378549348057,
0.25,0.308039612188458,0.365335670776957,0.422295269231874,0.479061587332518,
0.5357767915656,0.592768342789219,0.649980384244181,0.707849804243744,0.75,
0.808900803033482,0.869149031981107,0.930289648544625,0.992896609496699,
0.999999999969533),.UNSPECIFIED.);
#255=B_SPLINE_CURVE_WITH_KNOTS('',3,(#52679,#52680,#52681,#52682,#52683,
#52684,#52685,#52686,#52687,#52688,#52689,#52690,#52691,#52692,#52693,#52694,
#52695,#52696,#52697,#52698,#52699,#52700),.UNSPECIFIED.,.F.,.F.,(4,3,3,
3,3,3,3,4),(1.5041390606593E-6,0.142631039269413,0.324838433643509,0.5,
0.67989376920272,0.724939089794903,0.90203826115051,0.999999999994462),
 .UNSPECIFIED.);
#256=B_SPLINE_CURVE_WITH_KNOTS('',3,(#52702,#52703,#52704,#52705,#52706,
#52707,#52708,#52709,#52710,#52711,#52712),.UNSPECIFIED.,.F.,.F.,(4,1,2,
2,2,4),(0.,0.124999999999997,0.187499999999997,0.249999999999997,0.499999999999997,
1.),.UNSPECIFIED.);
#257=B_SPLINE_CURVE_WITH_KNOTS('',3,(#52713,#52714,#52715,#52716,#52717,
#52718,#52719,#52720,#52721,#52722,#52723,#52724,#52725,#52726,#52727,#52728,
#52729,#52730,#52731,#52732,#52733,#52734,#52735,#52736,#52737,#52738,#52739,
#52740,#52741,#52742,#52743,#52744,#52745,#52746,#52747,#52748,#52749,#52750,
#52751,#52752,#52753,#52754,#52755,#52756,#52757,#52758,#52759,#52760,#52761,
#52762,#52763,#52764,#52765,#52766,#52767),.UNSPECIFIED.,.F.,.F.,(4,3,3,
3,3,3,3,3,3,3,3,3,3,3,3,3,3,3,4),(0.,0.0650994436402108,0.130198887280422,
0.199793608914402,0.25,0.313473939291271,0.390075348944641,0.437499999999999,
0.468749999999999,0.484374999999998,0.492187499999998,0.498312113050278,
0.499999999999998,0.537870461654632,0.639813161810115,0.71967098213258,
0.82663606314356,0.908057804663619,1.),.UNSPECIFIED.);
#258=B_SPLINE_CURVE_WITH_KNOTS('',3,(#52813,#52814,#52815,#52816,#52817,
#52818,#52819,#52820,#52821,#52822,#52823,#52824,#52825,#52826,#52827,#52828,
#52829,#52830,#52831,#52832,#52833,#52834,#52835,#52836,#52837,#52838,#52839,
#52840,#52841,#52842,#52843,#52844,#52845,#52846,#52847,#52848,#52849,#52850,
#52851,#52852,#52853,#52854,#52855,#52856,#52857,#52858,#52859,#52860,#52861,
#52862,#52863,#52864,#52865,#52866,#52867,#52868,#52869,#52870,#52871,#52872,
#52873,#52874,#52875,#52876,#52877,#52878,#52879,#52880,#52881,#52882,#52883,
#52884,#52885),.UNSPECIFIED.,.F.,.F.,(4,3,3,3,3,3,3,3,3,3,3,3,3,3,3,3,3,
3,3,3,3,3,3,3,4),(1.45421879214282E-9,0.0431191253427652,0.0863267720250147,
0.129382358804927,0.1428571428571,0.153643952151919,0.204633581287644,0.255730997960889,
0.2857142857143,0.306393509456594,0.370923699532922,0.4285714285714,0.45941201799842,
0.526893092898446,0.5714285714286,0.612488429044932,0.677675308974725,0.7142857142857,
0.765391329815468,0.819870817397087,0.8571428571429,0.900979338361016,0.918139369288227,
0.961788840617674,1.),.UNSPECIFIED.);
#259=B_SPLINE_CURVE_WITH_KNOTS('',3,(#52888,#52889,#52890,#52891,#52892,
#52893,#52894,#52895,#52896,#52897,#52898,#52899,#52900,#52901,#52902,#52903,
#52904,#52905,#52906,#52907,#52908,#52909,#52910,#52911,#52912,#52913,#52914,
#52915,#52916,#52917,#52918,#52919,#52920,#52921,#52922,#52923,#52924,#52925,
#52926,#52927,#52928,#52929,#52930,#52931,#52932,#52933,#52934,#52935,#52936,
#52937,#52938,#52939,#52940,#52941,#52942,#52943,#52944,#52945,#52946,#52947,
#52948,#52949,#52950,#52951,#52952,#52953,#52954,#52955,#52956,#52957,#52958,
#52959,#52960),.UNSPECIFIED.,.F.,.F.,(4,3,3,3,3,3,3,3,3,3,3,3,3,3,3,3,3,
3,3,3,3,3,3,3,4),(0.,0.0558892582289014,0.112669247781944,0.156953381452509,
0.215052185968344,0.249999999999993,0.309316249815091,0.32431076563434,
0.38539095426848,0.437499999999988,0.468749999999988,0.484374999999988,
0.492187499999988,0.498949390062523,0.499999999999988,0.504583453135758,
0.573408356689112,0.64134333511677,0.680145776021464,0.749999999999994,
0.815926291102209,0.847891300901525,0.914668851233571,0.980715804659358,
1.),.UNSPECIFIED.);
#260=B_SPLINE_CURVE_WITH_KNOTS('',3,(#53059,#53060,#53061,#53062,#53063,
#53064,#53065,#53066,#53067,#53068,#53069,#53070,#53071,#53072,#53073,#53074,
#53075,#53076,#53077,#53078,#53079,#53080,#53081,#53082,#53083,#53084,#53085,
#53086,#53087,#53088,#53089,#53090,#53091,#53092,#53093,#53094,#53095,#53096,
#53097,#53098,#53099,#53100,#53101,#53102,#53103,#53104,#53105,#53106,#53107,
#53108,#53109,#53110,#53111,#53112,#53113,#53114,#53115,#53116,#53117,#53118,
#53119,#53120,#53121,#53122,#53123,#53124,#53125,#53126,#53127,#53128,#53129,
#53130,#53131,#53132,#53133,#53134,#53135,#53136,#53137,#53138,#53139,#53140,
#53141,#53142,#53143,#53144,#53145,#53146,#53147,#53148,#53149,#53150,#53151,
#53152,#53153,#53154,#53155,#53156,#53157,#53158,#53159,#53160,#53161,#53162,
#53163,#53164,#53165,#53166,#53167,#53168,#53169,#53170,#53171,#53172,#53173,
#53174,#53175,#53176,#53177,#53178,#53179,#53180,#53181,#53182,#53183,#53184,
#53185,#53186,#53187,#53188,#53189,#53190,#53191,#53192,#53193,#53194,#53195,
#53196,#53197,#53198,#53199,#53200,#53201,#53202,#53203,#53204,#53205,#53206,
#53207,#53208,#53209,#53210,#53211,#53212,#53213,#53214,#53215,#53216,#53217,
#53218,#53219,#53220,#53221,#53222,#53223,#53224),.UNSPECIFIED.,.F.,.F.,
(4,3,3,3,3,3,3,3,3,3,3,3,3,3,3,3,3,3,3,3,3,3,3,3,3,3,3,3,3,3,3,3,3,3,3,
3,3,3,3,3,3,3,3,3,3,3,3,3,3,3,3,3,3,3,3,4),(8.91633426931597E-8,0.0341866200056338,
0.0624999999999992,0.0800113026486996,0.0937499999999987,0.109374999999998,
0.117187499999998,0.121093749999998,0.123046874999998,0.124999999999998,
0.156875028251668,0.1875,0.218750000000001,0.234375000000001,0.237518692308383,
0.242187500000002,0.246093750000002,0.248046875000002,0.250000000000002,
0.290850977675925,0.312500000000002,0.328922102328694,0.343750000000002,
0.359375000000002,0.367187500000002,0.371093750000002,0.373046875000002,
0.375000000000002,0.425211651263262,0.437500000000002,0.468750000000001,
0.484375000000001,0.492187500000001,0.496093750000001,0.500000000000001,
0.520156881115364,0.572597422442347,0.616913355571128,0.625000000000001,
0.651328060847,0.678222159827132,0.6875,0.709176140839145,0.75,0.78125,
0.7890625,0.796875,0.799086910217881,0.8125,0.858396212816867,0.875,0.885500856062245,
0.932686341515045,0.980790797833406,0.98573188374278,1.),.UNSPECIFIED.);
#261=B_SPLINE_CURVE_WITH_KNOTS('',3,(#53227,#53228,#53229,#53230,#53231,
#53232,#53233,#53234,#53235,#53236,#53237,#53238,#53239,#53240,#53241,#53242,
#53243,#53244,#53245,#53246,#53247,#53248,#53249,#53250,#53251,#53252,#53253,
#53254,#53255,#53256,#53257,#53258,#53259,#53260,#53261,#53262,#53263,#53264,
#53265,#53266,#53267,#53268,#53269,#53270,#53271,#53272,#53273,#53274,#53275,
#53276,#53277,#53278,#53279,#53280,#53281,#53282,#53283,#53284,#53285,#53286,
#53287,#53288,#53289,#53290,#53291,#53292,#53293,#53294,#53295,#53296,#53297,
#53298,#53299,#53300,#53301,#53302,#53303,#53304,#53305,#53306,#53307,#53308,
#53309,#53310,#53311,#53312,#53313,#53314,#53315,#53316,#53317,#53318,#53319,
#53320,#53321,#53322,#53323,#53324,#53325,#53326,#53327,#53328,#53329,#53330,
#53331,#53332,#53333,#53334,#53335,#53336,#53337,#53338,#53339,#53340,#53341,
#53342,#53343,#53344,#53345,#53346,#53347,#53348,#53349,#53350,#53351,#53352,
#53353,#53354,#53355,#53356,#53357,#53358,#53359,#53360,#53361,#53362,#53363,
#53364,#53365,#53366,#53367,#53368),.UNSPECIFIED.,.F.,.F.,(4,3,3,3,3,3,
3,3,3,3,3,3,3,3,3,3,3,3,3,3,3,3,3,3,3,3,3,3,3,3,3,3,3,3,3,3,3,3,3,3,3,3,
3,3,3,3,3,4),(2.34638000429566E-7,0.0315958252999231,0.0628964643186087,
0.0937122453289208,0.10417220844182,0.124999999999999,0.154837292802782,
0.184674585605564,0.213175902892385,0.218749999999999,0.234374999999999,
0.242187499999999,0.246093749999999,0.248046874999998,0.249999999999998,
0.257790527710696,0.295642545408796,0.334483525618913,0.354334856151428,
0.392683149567989,0.431398866791145,0.470481924430731,0.482377267678491,
0.484375000000002,0.496585772826167,0.500000000000002,0.540377617471143,
0.58037233206427,0.609455371445993,0.649166188301461,0.687500000000005,
0.700832172402015,0.718750000000005,0.734375000000005,0.742187500000005,
0.746093750000005,0.748046875000005,0.750000000000005,0.769091706308904,
0.79896691623487,0.828842126160835,0.858577033135406,0.875000000000003,
0.89678232603399,0.927914261958254,0.959582462922759,0.985641707998622,
1.),.UNSPECIFIED.);
#262=B_SPLINE_CURVE_WITH_KNOTS('',3,(#53405,#53406,#53407,#53408,#53409,
#53410,#53411,#53412,#53413,#53414,#53415,#53416,#53417,#53418,#53419,#53420,
#53421,#53422,#53423,#53424,#53425,#53426,#53427,#53428,#53429,#53430,#53431,
#53432,#53433,#53434,#53435,#53436,#53437,#53438,#53439,#53440,#53441,#53442,
#53443,#53444,#53445,#53446,#53447,#53448,#53449,#53450,#53451,#53452,#53453,
#53454,#53455,#53456,#53457,#53458,#53459,#53460,#53461,#53462,#53463,#53464,
#53465),.UNSPECIFIED.,.F.,.F.,(4,3,3,3,3,3,3,3,3,3,3,3,3,3,3,3,3,3,3,3,
4),(3.81436863215028E-8,0.0594692241135463,0.119461332976601,0.180335226693879,
0.228233297279517,0.25,0.3125,0.375,0.420627166446326,0.466475792531788,
0.500000000000001,0.532982594262802,0.595584209629977,0.657507055367544,
0.718468272244316,0.75,0.809830564880495,0.831293963743825,0.890887057024469,
0.949594063922645,0.999999999994814),.UNSPECIFIED.);
#263=B_SPLINE_CURVE_WITH_KNOTS('',3,(#53466,#53467,#53468,#53469,#53470,
#53471,#53472,#53473,#53474,#53475,#53476,#53477,#53478,#53479,#53480,#53481,
#53482,#53483,#53484,#53485,#53486,#53487,#53488,#53489,#53490,#53491,#53492,
#53493,#53494,#53495,#53496,#53497,#53498,#53499,#53500,#53501,#53502,#53503,
#53504,#53505,#53506,#53507,#53508,#53509,#53510,#53511,#53512,#53513,#53514,
#53515,#53516,#53517,#53518,#53519,#53520,#53521,#53522,#53523),
 .UNSPECIFIED.,.F.,.F.,(4,3,3,3,3,3,3,3,3,3,3,3,3,3,3,3,3,3,3,4),(0.,0.0707847540439358,
0.13714897876124,0.19876944030244,0.25,0.307617673205022,0.364360156798302,
0.42070510310328,0.476621035240063,0.49999980758445,0.5,0.555639382305717,
0.611765726333174,0.668272106356441,0.72549762942489,0.75,0.812499999999486,
0.877170052799808,0.948088545219367,0.999999999997942),.UNSPECIFIED.);
#264=B_SPLINE_CURVE_WITH_KNOTS('',3,(#53562,#53563,#53564,#53565,#53566,
#53567,#53568,#53569,#53570,#53571,#53572,#53573,#53574,#53575,#53576,#53577,
#53578,#53579,#53580,#53581,#53582,#53583,#53584,#53585,#53586,#53587,#53588,
#53589,#53590,#53591,#53592,#53593,#53594,#53595,#53596,#53597,#53598,#53599,
#53600,#53601,#53602,#53603,#53604,#53605,#53606,#53607,#53608,#53609,#53610,
#53611,#53612,#53613,#53614,#53615,#53616,#53617,#53618,#53619,#53620,#53621,
#53622,#53623,#53624,#53625,#53626,#53627,#53628,#53629,#53630,#53631,#53632,
#53633,#53634,#53635,#53636,#53637,#53638,#53639,#53640,#53641,#53642,#53643),
 .UNSPECIFIED.,.F.,.F.,(4,3,3,3,3,3,3,3,3,3,3,3,3,3,3,3,3,3,3,3,3,3,3,3,
3,3,3,4),(0.,0.0792150655842689,0.124999999999999,0.125921017487507,0.187499999999999,
0.218749999999999,0.234374999999999,0.242187499999999,0.248597221451861,
0.249999999999999,0.312515849372989,0.385046619809545,0.457415846192531,
0.499988433043988,0.499999999999998,0.570823904390727,0.624999999999998,
0.687466106592308,0.687499999999998,0.718749999999998,0.734374999999998,
0.742187499999998,0.748633296290449,0.749999999999998,0.823394013248657,
0.874049304626543,0.94994762549464,1.),.UNSPECIFIED.);
#265=B_SPLINE_CURVE_WITH_KNOTS('',3,(#53682,#53683,#53684,#53685,#53686,
#53687,#53688,#53689,#53690,#53691,#53692,#53693,#53694,#53695,#53696,#53697,
#53698,#53699,#53700,#53701,#53702,#53703,#53704,#53705,#53706,#53707,#53708,
#53709,#53710,#53711,#53712),.UNSPECIFIED.,.F.,.F.,(4,3,3,3,3,3,3,3,3,3,
4),(0.,0.124999999999982,0.187499999999974,0.218749999999971,0.234374999999969,
0.242187499999969,0.249999999999969,0.374999999999973,0.499999999999977,
0.749999999999989,1.),.UNSPECIFIED.);
#266=B_SPLINE_CURVE_WITH_KNOTS('',3,(#53713,#53714,#53715,#53716,#53717,
#53718,#53719,#53720,#53721,#53722,#53723,#53724,#53725,#53726,#53727,#53728,
#53729,#53730,#53731,#53732,#53733,#53734),.UNSPECIFIED.,.F.,.F.,(4,3,3,
3,3,3,3,4),(0.,0.177024512090844,0.292989167962771,0.472837133506511,0.5,
0.689142403121388,0.878284806242776,0.999997308150379),.UNSPECIFIED.);
#267=B_SPLINE_CURVE_WITH_KNOTS('',3,(#53735,#53736,#53737,#53738,#53739,
#53740,#53741,#53742,#53743,#53744,#53745,#53746,#53747,#53748,#53749,#53750,
#53751,#53752,#53753,#53754,#53755,#53756,#53757,#53758,#53759,#53760,#53761,
#53762,#53763,#53764,#53765,#53766,#53767,#53768,#53769,#53770,#53771,#53772,
#53773,#53774,#53775,#53776,#53777,#53778,#53779,#53780,#53781,#53782,#53783,
#53784,#53785,#53786,#53787,#53788,#53789,#53790,#53791,#53792,#53793,#53794,
#53795),.UNSPECIFIED.,.F.,.F.,(4,3,3,3,3,3,3,3,3,3,3,3,3,3,3,3,3,3,3,3,
4),(0.,0.0976856521887196,0.205020687001143,0.250000000000006,0.286357328179635,
0.375000000000008,0.437500000000008,0.467815798455655,0.468750000000008,
0.484375000000007,0.492187500000007,0.497983320289822,0.500000000000006,
0.581183162361599,0.657948135640541,0.692880023009447,0.750000000000003,
0.820238740768344,0.874892120286855,0.9403090323846,0.999999999888379),
 .UNSPECIFIED.);
#268=B_SPLINE_CURVE_WITH_KNOTS('',3,(#53838,#53839,#53840,#53841,#53842,
#53843,#53844,#53845,#53846,#53847,#53848,#53849,#53850,#53851,#53852,#53853,
#53854,#53855,#53856,#53857,#53858,#53859,#53860,#53861,#53862,#53863,#53864,
#53865,#53866,#53867,#53868,#53869,#53870,#53871,#53872,#53873,#53874,#53875,
#53876,#53877,#53878,#53879,#53880,#53881,#53882,#53883,#53884,#53885,#53886,
#53887,#53888,#53889,#53890,#53891,#53892,#53893,#53894,#53895,#53896,#53897,
#53898,#53899,#53900,#53901,#53902,#53903,#53904,#53905,#53906,#53907,#53908,
#53909,#53910,#53911,#53912,#53913,#53914,#53915,#53916,#53917,#53918,#53919,
#53920,#53921,#53922,#53923,#53924,#53925,#53926,#53927,#53928),
 .UNSPECIFIED.,.F.,.F.,(4,3,3,3,3,3,3,3,3,3,3,3,3,3,3,3,3,3,3,3,3,3,3,3,
3,3,3,3,3,3,4),(1.98871583907149E-7,0.0470903211130683,0.0950886099489182,
0.109526542541016,0.125000000000008,0.176685447236339,0.187500000000013,
0.19557488232977,0.203125000000014,0.218750000000014,0.250000000000015,
0.27062164890649,0.3341041042639,0.398265330724908,0.430414683829977,0.437500000000016,
0.468750000000016,0.484375000000016,0.492187500000016,0.49803412523616,
0.500000000000016,0.559924707782723,0.6001249554854,0.658475264874343,0.715889345308872,
0.764250567674328,0.821849981037566,0.878616147063133,0.918178967654373,
0.970962443959493,1.),.UNSPECIFIED.);
#269=B_SPLINE_CURVE_WITH_KNOTS('',3,(#53973,#53974,#53975,#53976,#53977,
#53978,#53979,#53980,#53981,#53982,#53983,#53984,#53985,#53986,#53987,#53988,
#53989,#53990,#53991,#53992,#53993,#53994,#53995,#53996,#53997,#53998,#53999,
#54000,#54001,#54002,#54003,#54004,#54005,#54006,#54007,#54008,#54009,#54010,
#54011,#54012,#54013,#54014,#54015,#54016,#54017,#54018,#54019,#54020,#54021,
#54022,#54023,#54024,#54025,#54026,#54027,#54028,#54029,#54030),
 .UNSPECIFIED.,.F.,.F.,(4,3,3,3,3,3,3,3,3,3,3,3,3,3,3,3,3,3,3,4),(0.,0.0625,
0.123437357561668,0.183435176402664,0.242378391891801,0.25,0.308040053618873,
0.365336549014984,0.422296583768566,0.479063340059895,0.535778986169599,
0.592770982238121,0.6499834721799,0.707853330673838,0.75,0.808902290745458,
0.869152098427341,0.930294379921426,0.992903114983252,1.),.UNSPECIFIED.);
#270=B_SPLINE_CURVE_WITH_KNOTS('',3,(#54032,#54033,#54034,#54035,#54036,
#54037,#54038,#54039,#54040,#54041,#54042,#54043,#54044,#54045,#54046,#54047,
#54048,#54049,#54050,#54051,#54052,#54053,#54054,#54055,#54056),
 .UNSPECIFIED.,.F.,.F.,(4,3,3,3,3,3,3,3,4),(1.330406108134E-6,0.181643406415568,
0.207927514662845,0.390638495071313,0.5,0.679764878140392,0.772661902357852,
0.949922356290452,1.),.UNSPECIFIED.);
#271=B_SPLINE_CURVE_WITH_KNOTS('',3,(#54058,#54059,#54060,#54061,#54062,
#54063,#54064,#54065,#54066,#54067,#54068,#54069,#54070),.UNSPECIFIED.,
 .F.,.F.,(4,3,3,3,4),(0.,0.187500000000001,0.250000000000001,0.500000000000001,
1.),.UNSPECIFIED.);
#272=B_SPLINE_CURVE_WITH_KNOTS('',3,(#54071,#54072,#54073,#54074,#54075,
#54076,#54077,#54078,#54079,#54080,#54081,#54082,#54083,#54084,#54085,#54086,
#54087,#54088,#54089,#54090,#54091,#54092,#54093,#54094,#54095,#54096,#54097,
#54098,#54099,#54100,#54101,#54102,#54103,#54104,#54105,#54106,#54107,#54108,
#54109,#54110,#54111,#54112,#54113,#54114,#54115,#54116,#54117,#54118,#54119,
#54120,#54121,#54122,#54123,#54124,#54125,#54126,#54127,#54128,#54129,#54130,
#54131,#54132,#54133,#54134,#54135,#54136,#54137,#54138,#54139,#54140,#54141,
#54142,#54143,#54144,#54145,#54146,#54147,#54148,#54149),.UNSPECIFIED.,
 .F.,.F.,(4,3,3,3,3,3,3,3,3,3,3,3,3,3,3,3,3,3,3,3,3,3,3,3,3,3,4),(1.45817479409027E-11,
0.00165012278096161,0.0447426246888551,0.0904394296673588,0.124999999999989,
0.158030392352972,0.187499999999984,0.218749999999981,0.23437499999998,
0.242187499999982,0.246093749999983,0.248046874999984,0.249999999999984,
0.335606080067904,0.366241870352233,0.374999999999973,0.437499999999968,
0.468749999999966,0.484374999999965,0.495318580094463,0.499999999999964,
0.553856462622792,0.656803820681865,0.736020610771133,0.84337533284278,
0.922615832922426,0.999999999885346),.UNSPECIFIED.);
#273=B_SPLINE_CURVE_WITH_KNOTS('',3,(#54191,#54192,#54193,#54194,#54195,
#54196,#54197,#54198,#54199,#54200,#54201,#54202,#54203,#54204,#54205,#54206,
#54207,#54208,#54209,#54210,#54211,#54212,#54213,#54214,#54215,#54216,#54217,
#54218,#54219,#54220,#54221,#54222,#54223,#54224,#54225,#54226,#54227,#54228,
#54229,#54230,#54231,#54232,#54233,#54234,#54235,#54236,#54237,#54238,#54239,
#54240,#54241,#54242,#54243,#54244,#54245,#54246,#54247,#54248,#54249,#54250,
#54251,#54252,#54253,#54254,#54255,#54256,#54257,#54258,#54259,#54260,#54261,
#54262,#54263,#54264,#54265,#54266,#54267,#54268,#54269,#54270,#54271,#54272,
#54273,#54274,#54275,#54276,#54277,#54278),.UNSPECIFIED.,.F.,.F.,(4,3,3,
3,3,3,3,3,3,3,3,3,3,3,3,3,3,3,3,3,3,3,3,3,3,3,3,3,3,4),(0.,0.0527820104074715,
0.0818213323246725,0.138473115952622,0.195945212509441,0.235750029132872,
0.293012176753044,0.351193392797035,0.39987544901493,0.437500000000017,
0.468750000000018,0.484375000000019,0.492187500000019,0.496093750000018,
0.499508594500751,0.500000000000018,0.565860735166544,0.629574768817817,
0.693958667104365,0.72575099412064,0.781250000000005,0.790730854104752,
0.796875000000005,0.812500000000005,0.869043334984336,0.875000000000003,
0.884835783967175,0.938700818461981,0.993360674255924,0.999999777750421),
 .UNSPECIFIED.);
#274=B_SPLINE_CURVE_WITH_KNOTS('',3,(#54281,#54282,#54283,#54284,#54285,
#54286,#54287,#54288,#54289,#54290,#54291,#54292,#54293,#54294,#54295,#54296,
#54297,#54298,#54299,#54300,#54301,#54302,#54303,#54304,#54305,#54306,#54307,
#54308,#54309,#54310,#54311,#54312,#54313,#54314,#54315,#54316,#54317,#54318,
#54319,#54320,#54321,#54322,#54323,#54324,#54325,#54326,#54327,#54328,#54329,
#54330,#54331,#54332,#54333,#54334,#54335,#54336,#54337,#54338),
 .UNSPECIFIED.,.F.,.F.,(4,3,3,3,3,3,3,3,3,3,3,3,3,3,3,3,3,3,3,4),(0.,0.0585630956581098,
0.11799660785587,0.16870786218184,0.228541511703754,0.250000000000001,0.312500000000001,
0.375000000000001,0.421054231074681,0.467108462149362,0.500000000000001,
0.563532899274307,0.626399529047779,0.688223246127237,0.750000000000001,
0.771768823660319,0.832605857581761,0.892881416492703,0.95230696880294,
0.999999961863694),.UNSPECIFIED.);
#275=B_SPLINE_CURVE_WITH_KNOTS('',3,(#54389,#54390,#54391,#54392,#54393,
#54394,#54395,#54396,#54397,#54398,#54399,#54400,#54401,#54402,#54403,#54404,
#54405,#54406,#54407,#54408,#54409,#54410,#54411,#54412,#54413,#54414,#54415,
#54416,#54417,#54418,#54419,#54420,#54421,#54422,#54423,#54424,#54425,#54426,
#54427,#54428,#54429,#54430,#54431,#54432,#54433,#54434,#54435,#54436,#54437,
#54438,#54439,#54440,#54441,#54442,#54443,#54444,#54445,#54446,#54447,#54448,
#54449,#54450,#54451,#54452,#54453,#54454,#54455,#54456,#54457,#54458,#54459,
#54460,#54461,#54462,#54463,#54464,#54465,#54466,#54467,#54468,#54469,#54470,
#54471,#54472,#54473,#54474,#54475,#54476,#54477,#54478,#54479,#54480,#54481,
#54482,#54483,#54484,#54485,#54486,#54487,#54488,#54489,#54490,#54491,#54492,
#54493,#54494,#54495,#54496,#54497,#54498,#54499,#54500,#54501,#54502,#54503,
#54504,#54505,#54506,#54507,#54508,#54509,#54510,#54511,#54512,#54513,#54514,
#54515,#54516,#54517,#54518,#54519,#54520,#54521,#54522,#54523,#54524,#54525,
#54526,#54527,#54528,#54529,#54530,#54531,#54532,#54533,#54534,#54535,#54536,
#54537,#54538,#54539,#54540,#54541,#54542,#54543,#54544,#54545,#54546,#54547,
#54548,#54549,#54550,#54551,#54552,#54553,#54554,#54555,#54556,#54557,#54558,
#54559,#54560,#54561,#54562,#54563,#54564,#54565,#54566,#54567,#54568,#54569,
#54570,#54571,#54572,#54573,#54574,#54575,#54576,#54577,#54578,#54579,#54580,
#54581,#54582,#54583,#54584,#54585,#54586,#54587,#54588,#54589,#54590,#54591,
#54592,#54593,#54594,#54595,#54596,#54597,#54598,#54599,#54600,#54601,#54602,
#54603,#54604,#54605,#54606,#54607,#54608,#54609,#54610,#54611,#54612,#54613,
#54614,#54615,#54616,#54617,#54618,#54619,#54620,#54621,#54622,#54623,#54624,
#54625,#54626,#54627,#54628,#54629,#54630,#54631,#54632),.UNSPECIFIED.,
 .F.,.F.,(4,3,3,3,3,3,3,3,3,3,3,3,3,3,3,3,3,3,3,3,3,3,3,3,3,3,3,3,3,3,3,
3,3,3,3,3,3,3,3,3,3,3,3,3,3,3,3,3,3,3,3,3,3,3,3,3,3,3,3,3,3,3,3,3,3,3,3,
3,3,3,3,3,3,3,3,3,3,3,3,3,3,4),(9.74885373639512E-8,0.0159200062587186,
0.031250000000024,0.0468750000000361,0.0546875000000421,0.0585937500000451,
0.0625000000000481,0.064860891737383,0.0837424297147262,0.10256194718207,
0.109375000000083,0.117187500000089,0.121093750000092,0.123046875000094,
0.124023437500095,0.124511718750095,0.125000000000095,0.13088113283216,
0.145623338057796,0.160279740929913,0.171875000000121,0.179687500000125,
0.183593750000127,0.185546875000129,0.186523437500129,0.18750000000013,
0.198322293578093,0.209103043160817,0.213452349241984,0.224198983077635,
0.234874954929346,0.242187500000162,0.246093750000164,0.248046875000165,
0.249023437500166,0.249755859375166,0.250000000000166,0.28612814128228,
0.331147428104677,0.373117414619281,0.413995852027384,0.437500000000167,
0.442038759562938,0.468750000000167,0.484375000000167,0.492187500000167,
0.496093750000167,0.498046875000167,0.4988073956278,0.499023437500167,0.499511718750167,
0.500000000000167,0.527809511524871,0.55563689272658,0.580222745701537,
0.608292500450986,0.634707899177733,0.640625000000145,0.645734470948701,
0.648437500000144,0.665746275460254,0.677886474696675,0.695389033000862,
0.712977553082935,0.73065498180394,0.734375000000131,0.74218750000013,0.74609375000013,
0.74804687500013,0.74902343750013,0.74951171875013,0.750000000000129,0.752487431508907,
0.797977655326278,0.804136709370455,0.850539439908008,0.858789251719635,
0.906288880937672,0.920205788064523,0.968988607968507,0.993036230187174,
1.),.UNSPECIFIED.);
#276=B_SPLINE_CURVE_WITH_KNOTS('',3,(#54715,#54716,#54717,#54718,#54719,
#54720,#54721,#54722,#54723,#54724,#54725,#54726,#54727,#54728,#54729,#54730,
#54731,#54732,#54733,#54734,#54735,#54736,#54737,#54738,#54739,#54740,#54741,
#54742,#54743,#54744,#54745,#54746,#54747,#54748,#54749,#54750,#54751,#54752,
#54753,#54754,#54755,#54756,#54757,#54758,#54759,#54760,#54761,#54762,#54763,
#54764,#54765,#54766,#54767,#54768,#54769,#54770,#54771,#54772,#54773,#54774,
#54775,#54776,#54777,#54778,#54779,#54780,#54781,#54782,#54783,#54784,#54785,
#54786,#54787,#54788,#54789,#54790,#54791,#54792,#54793,#54794,#54795,#54796,
#54797,#54798,#54799,#54800,#54801,#54802,#54803,#54804,#54805,#54806,#54807,
#54808,#54809,#54810,#54811,#54812,#54813,#54814,#54815,#54816,#54817,#54818,
#54819,#54820,#54821,#54822,#54823,#54824,#54825,#54826,#54827,#54828,#54829,
#54830,#54831,#54832,#54833,#54834,#54835,#54836,#54837,#54838,#54839,#54840,
#54841,#54842,#54843,#54844,#54845,#54846,#54847,#54848,#54849,#54850,#54851,
#54852,#54853,#54854,#54855,#54856,#54857,#54858,#54859,#54860,#54861,#54862,
#54863,#54864,#54865,#54866,#54867,#54868,#54869,#54870,#54871),
 .UNSPECIFIED.,.F.,.F.,(4,3,3,3,3,3,3,3,3,3,3,3,3,3,3,3,3,3,3,3,3,3,3,3,
3,3,3,3,3,3,3,3,3,3,3,3,3,3,3,3,3,3,3,3,3,3,3,3,3,3,3,3,4),(1.72726440594495E-7,
0.0434573132527648,0.0863338474990505,0.093216517716401,0.124999999999985,
0.165840010670402,0.177272924303734,0.187499999999978,0.218749999999974,
0.234374999999973,0.242187499999972,0.246093749999971,0.249511718749971,
0.249999999999971,0.260112842122813,0.284904275703955,0.309601373157129,
0.312499999999974,0.336932316158668,0.343749999999976,0.359374999999977,
0.359741421885534,0.367187499999977,0.371093749999978,0.373046874999978,
0.374023437499978,0.374999999999978,0.427162028762236,0.437499999999979,
0.446539513801691,0.468749999999979,0.48437499999998,0.49218749999998,0.499058235380736,
0.49999999999998,0.529373135558955,0.595489465840445,0.60162559917597,0.624999999999982,
0.666787835011797,0.687499999999983,0.718749999999984,0.726755886335632,
0.734374999999984,0.746093749999984,0.749999999999985,0.777566191164044,
0.821931417214387,0.864144998210834,0.906142061394322,0.949726796380935,
0.995918874659696,0.999999956010456),.UNSPECIFIED.);
#277=B_SPLINE_CURVE_WITH_KNOTS('',3,(#54916,#54917,#54918,#54919,#54920,
#54921,#54922,#54923,#54924,#54925,#54926,#54927,#54928,#54929,#54930,#54931,
#54932,#54933,#54934,#54935,#54936,#54937,#54938,#54939,#54940,#54941,#54942,
#54943,#54944,#54945,#54946),.UNSPECIFIED.,.F.,.F.,(4,3,3,3,3,3,3,3,3,3,
4),(0.,0.125000000000019,0.187500000000028,0.218750000000032,0.234375000000033,
0.242187500000033,0.250000000000033,0.375000000000028,0.500000000000022,
0.750000000000011,1.),.UNSPECIFIED.);
#278=B_SPLINE_CURVE_WITH_KNOTS('',3,(#54948,#54949,#54950,#54951,#54952,
#54953,#54954,#54955,#54956,#54957,#54958,#54959,#54960,#54961,#54962,#54963,
#54964,#54965,#54966,#54967,#54968,#54969,#54970,#54971,#54972),
 .UNSPECIFIED.,.F.,.F.,(4,3,3,3,3,3,3,3,4),(0.,0.177282336143491,0.213907941281364,
0.393665915351053,0.5,0.682805729838532,0.77695616943279,0.958668461365049,
0.999998980185047),.UNSPECIFIED.);
#279=B_SPLINE_CURVE_WITH_KNOTS('',3,(#54974,#54975,#54976,#54977,#54978,
#54979,#54980,#54981,#54982,#54983,#54984,#54985,#54986,#54987,#54988,#54989,
#54990,#54991,#54992,#54993,#54994,#54995,#54996,#54997,#54998,#54999,#55000,
#55001,#55002,#55003,#55004,#55005,#55006,#55007,#55008,#55009,#55010,#55011,
#55012,#55013,#55014,#55015,#55016,#55017,#55018,#55019,#55020,#55021,#55022,
#55023,#55024,#55025,#55026,#55027,#55028,#55029,#55030,#55031,#55032,#55033,
#55034),.UNSPECIFIED.,.F.,.F.,(4,3,3,3,3,3,3,3,3,3,3,3,3,3,3,3,3,3,3,3,
4),(5.73167048359177E-11,0.0625000000429875,0.123430758022991,0.183422273868319,
0.24235958000366,0.25,0.308040146146061,0.365368965521203,0.422365343403545,
0.479130682341562,0.5,0.55673209842876,0.61379107282782,0.671113553585964,
0.729073370544327,0.75,0.808901353783578,0.869150170975925,0.930291454539829,
0.992899267799122,1.),.UNSPECIFIED.);
#280=B_SPLINE_CURVE_WITH_KNOTS('',3,(#55035,#55036,#55037,#55038,#55039,
#55040,#55041,#55042,#55043,#55044,#55045,#55046,#55047,#55048,#55049,#55050,
#55051,#55052,#55053,#55054,#55055,#55056,#55057,#55058,#55059,#55060,#55061,
#55062,#55063,#55064,#55065,#55066,#55067,#55068,#55069,#55070,#55071,#55072,
#55073,#55074,#55075,#55076,#55077,#55078,#55079,#55080,#55081,#55082,#55083,
#55084,#55085,#55086,#55087,#55088,#55089,#55090,#55091,#55092,#55093,#55094,
#55095,#55096,#55097,#55098,#55099,#55100,#55101,#55102,#55103,#55104),
 .UNSPECIFIED.,.F.,.F.,(4,3,3,3,3,3,3,3,3,3,3,3,3,3,3,3,3,3,3,3,3,3,3,4),
(1.15604835473446E-10,0.072945956146836,0.180557791681298,0.25000000000002,
0.259407485718546,0.362622524995456,0.437500000000034,0.441690815636676,
0.468750000000037,0.484375000000039,0.492187500000039,0.498125154992541,
0.500000000000039,0.580027879028248,0.655074895560498,0.660055758056458,
0.732990214315364,0.75000000000002,0.818419921927436,0.849001518755108,
0.914551347658443,0.976944079464395,0.994828975829166,1.),.UNSPECIFIED.);
#281=B_SPLINE_CURVE_WITH_KNOTS('',3,(#55149,#55150,#55151,#55152,#55153,
#55154,#55155,#55156,#55157,#55158,#55159,#55160,#55161,#55162,#55163,#55164,
#55165,#55166,#55167,#55168,#55169,#55170,#55171,#55172,#55173,#55174,#55175,
#55176,#55177,#55178,#55179,#55180,#55181,#55182,#55183,#55184,#55185,#55186,
#55187,#55188,#55189,#55190,#55191,#55192,#55193,#55194,#55195,#55196,#55197,
#55198,#55199,#55200,#55201,#55202,#55203,#55204,#55205,#55206,#55207,#55208,
#55209,#55210,#55211,#55212,#55213,#55214,#55215,#55216,#55217,#55218),
 .UNSPECIFIED.,.F.,.F.,(4,3,3,3,3,3,3,3,3,3,3,3,3,3,3,3,3,3,3,3,3,3,3,4),
(0.,0.0435551679386673,0.076470578260204,0.120151332451966,0.125,0.178532794167066,
0.223906562246117,0.25,0.318743929132965,0.371576002742637,0.375,0.469091817166418,
0.5,0.519437350326105,0.625,0.667314026802467,0.7417108943593,0.75,0.808035583839871,
0.814957891431279,0.875,0.919742711947922,0.962451012488657,0.999999720284603),
 .UNSPECIFIED.);
#282=B_SPLINE_CURVE_WITH_KNOTS('',3,(#55219,#55220,#55221,#55222,#55223,
#55224,#55225,#55226,#55227,#55228,#55229,#55230,#55231,#55232,#55233,#55234,
#55235,#55236,#55237,#55238,#55239,#55240,#55241,#55242,#55243,#55244,#55245,
#55246,#55247,#55248,#55249,#55250,#55251,#55252,#55253,#55254,#55255,#55256,
#55257,#55258,#55259,#55260,#55261,#55262,#55263,#55264,#55265,#55266,#55267,
#55268,#55269,#55270,#55271,#55272,#55273,#55274,#55275,#55276,#55277,#55278,
#55279,#55280,#55281,#55282,#55283,#55284,#55285,#55286,#55287,#55288),
 .UNSPECIFIED.,.F.,.F.,(4,3,3,3,3,3,3,3,3,3,3,3,3,3,3,3,3,3,3,3,3,3,3,4),
(0.,0.0642452018256955,0.129223022111387,0.139648916649683,0.203363964417562,
0.250000000000005,0.300656440952451,0.36907822047623,0.43750000000001,0.468750000000011,
0.469711915463756,0.484375000000011,0.495154959267717,0.500000000000011,
0.563334722729026,0.625630761231619,0.644015065163845,0.704247224853198,
0.750000000000005,0.807879449656103,0.8684821469436,0.928163140833693,0.961961786669929,
0.999999992443035),.UNSPECIFIED.);
#283=B_SPLINE_CURVE_WITH_KNOTS('',3,(#55324,#55325,#55326,#55327,#55328,
#55329,#55330,#55331,#55332,#55333,#55334,#55335,#55336,#55337,#55338,#55339,
#55340,#55341,#55342,#55343,#55344,#55345,#55346,#55347,#55348,#55349,#55350,
#55351,#55352,#55353,#55354,#55355,#55356,#55357,#55358,#55359,#55360,#55361,
#55362,#55363,#55364,#55365,#55366,#55367,#55368,#55369,#55370,#55371,#55372,
#55373,#55374,#55375,#55376,#55377,#55378,#55379,#55380,#55381),
 .UNSPECIFIED.,.F.,.F.,(4,3,3,3,3,3,3,3,3,3,3,3,3,3,3,3,3,3,3,4),(0.,0.0339753543803814,
0.109950566125709,0.168097066017028,0.245117177635656,0.25,0.324143694588969,
0.40341117828457,0.483062939160984,0.5,0.500074284948893,0.580013729768816,
0.658971793933605,0.676028229049525,0.75,0.826841345162694,0.832059158171015,
0.907853033409699,0.966136292621797,1.),.UNSPECIFIED.);
#284=B_SPLINE_CURVE_WITH_KNOTS('',3,(#55426,#55427,#55428,#55429,#55430,
#55431,#55432,#55433,#55434,#55435,#55436,#55437,#55438,#55439,#55440,#55441,
#55442,#55443,#55444,#55445,#55446,#55447,#55448,#55449,#55450,#55451,#55452,
#55453,#55454,#55455,#55456,#55457,#55458,#55459,#55460,#55461,#55462,#55463,
#55464,#55465,#55466,#55467,#55468,#55469,#55470,#55471,#55472,#55473,#55474,
#55475,#55476,#55477,#55478,#55479,#55480,#55481,#55482,#55483,#55484,#55485,
#55486,#55487,#55488,#55489,#55490,#55491,#55492,#55493,#55494,#55495,#55496,
#55497,#55498,#55499,#55500,#55501,#55502,#55503,#55504,#55505,#55506,#55507,
#55508,#55509,#55510,#55511,#55512,#55513,#55514,#55515,#55516),
 .UNSPECIFIED.,.F.,.F.,(4,3,3,3,3,3,3,3,3,3,3,3,3,3,3,3,3,3,3,3,3,3,3,3,
3,3,3,3,3,3,4),(0.,0.0388645141120945,0.125000000000002,0.187500000000003,
0.190146043466364,0.218750000000003,0.234375000000003,0.242187500000003,
0.246093750000004,0.248046875000004,0.250000000000004,0.315771796321043,
0.342916849517666,0.407904968457705,0.472592506143607,0.499999999999999,
0.500065465413701,0.563235050528544,0.624999999999997,0.657214404683583,
0.687499999999995,0.718749999999995,0.734374999999995,0.742187499999994,
0.746093749999994,0.748046874999994,0.749999999999994,0.809981507440316,
0.896400830417988,0.961249318093161,1.),.UNSPECIFIED.);
#285=B_SPLINE_CURVE_WITH_KNOTS('',3,(#55555,#55556,#55557,#55558,#55559,
#55560,#55561,#55562,#55563,#55564,#55565,#55566,#55567,#55568,#55569,#55570,
#55571,#55572,#55573,#55574,#55575,#55576,#55577,#55578,#55579,#55580,#55581,
#55582,#55583,#55584,#55585,#55586,#55587,#55588,#55589,#55590,#55591,#55592,
#55593,#55594,#55595,#55596,#55597,#55598,#55599,#55600,#55601,#55602,#55603,
#55604,#55605,#55606,#55607,#55608,#55609,#55610,#55611,#55612),
 .UNSPECIFIED.,.F.,.F.,(4,3,3,3,3,3,3,3,3,3,3,3,3,3,3,3,3,3,3,4),(0.,0.0625,
0.123436056759143,0.18343260413623,0.24237460068037,0.25,0.308039776325257,
0.365335998405921,0.422295761702448,0.479062247404443,0.535777622950034,
0.592769350027535,0.649981570270837,0.70785116671443,0.75,0.808902110291868,
0.869151749075464,0.930293857117356,0.992902397598166,1.),.UNSPECIFIED.);
#286=B_SPLINE_CURVE_WITH_KNOTS('',3,(#55614,#55615,#55616,#55617,#55618,
#55619),.UNSPECIFIED.,.F.,.F.,(4,1,1,4),(1.40740795308042E-6,0.3333333333333,
0.6666666666667,1.),.UNSPECIFIED.);
#287=B_SPLINE_CURVE_WITH_KNOTS('',3,(#55621,#55622,#55623,#55624,#55625,
#55626,#55627,#55628,#55629,#55630,#55631,#55632,#55633),.UNSPECIFIED.,
 .F.,.F.,(4,3,3,3,4),(0.,0.1875,0.249999999999999,0.499999999999999,1.),
 .UNSPECIFIED.);
#288=B_SPLINE_CURVE_WITH_KNOTS('',3,(#55634,#55635,#55636,#55637,#55638,
#55639,#55640,#55641,#55642,#55643,#55644,#55645,#55646,#55647,#55648,#55649,
#55650,#55651,#55652,#55653,#55654,#55655,#55656,#55657,#55658,#55659,#55660,
#55661,#55662,#55663,#55664,#55665,#55666,#55667,#55668,#55669,#55670,#55671,
#55672,#55673,#55674,#55675,#55676,#55677,#55678,#55679,#55680,#55681,#55682,
#55683,#55684,#55685,#55686,#55687,#55688),.UNSPECIFIED.,.F.,.F.,(4,3,3,
3,3,3,3,3,3,3,3,3,3,3,3,3,3,3,4),(0.,0.0642483351342427,0.123631513668559,
0.192521447460844,0.250000000000009,0.313929035664213,0.389698805114818,
0.437500000000014,0.468750000000015,0.484375000000016,0.492187500000016,
0.49892305110334,0.500000000000016,0.532968101520917,0.640208044354892,
0.723028006675871,0.834863768936946,0.918219616793671,0.999999999866653),
 .UNSPECIFIED.);
#289=B_SPLINE_CURVE_WITH_KNOTS('',3,(#55734,#55735,#55736,#55737,#55738,
#55739,#55740,#55741,#55742,#55743,#55744,#55745,#55746,#55747,#55748,#55749,
#55750,#55751,#55752,#55753,#55754,#55755,#55756,#55757,#55758,#55759,#55760,
#55761,#55762,#55763,#55764,#55765,#55766,#55767,#55768,#55769,#55770,#55771,
#55772,#55773,#55774,#55775,#55776,#55777,#55778,#55779,#55780,#55781,#55782,
#55783,#55784,#55785,#55786,#55787,#55788,#55789,#55790,#55791,#55792,#55793,
#55794,#55795,#55796,#55797,#55798,#55799,#55800,#55801,#55802,#55803,#55804,
#55805,#55806),.UNSPECIFIED.,.F.,.F.,(4,3,3,3,3,3,3,3,3,3,3,3,3,3,3,3,3,
3,3,3,3,3,3,3,4),(1.45391862059565E-9,0.0431123241756327,0.086313162635294,
0.129361940668342,0.1428571428571,0.153622397531604,0.204599352639357,0.255684060316847,
0.2857142857143,0.306350448882393,0.37080198399618,0.4285714285714,0.459347099296346,
0.526502746439944,0.5714285714286,0.612403504379262,0.676567149297245,0.7142857142857,
0.76527664382255,0.818292079191637,0.8571428571429,0.90081416683432,0.918050451477613,
0.961569312477636,1.),.UNSPECIFIED.);
#290=B_SPLINE_CURVE_WITH_KNOTS('',3,(#55809,#55810,#55811,#55812,#55813,
#55814,#55815,#55816,#55817,#55818,#55819,#55820,#55821,#55822,#55823,#55824,
#55825,#55826,#55827,#55828,#55829,#55830,#55831,#55832,#55833,#55834,#55835,
#55836,#55837,#55838,#55839,#55840,#55841,#55842,#55843,#55844,#55845,#55846,
#55847,#55848,#55849,#55850,#55851,#55852,#55853,#55854,#55855,#55856,#55857,
#55858,#55859,#55860,#55861,#55862,#55863,#55864,#55865,#55866,#55867,#55868,
#55869,#55870,#55871,#55872,#55873,#55874,#55875,#55876,#55877,#55878,#55879,
#55880,#55881),.UNSPECIFIED.,.F.,.F.,(4,3,3,3,3,3,3,3,3,3,3,3,3,3,3,3,3,
3,3,3,3,3,3,3,4),(0.,0.0558892574716291,0.112669246806468,0.156953409715992,
0.215052214168376,0.250000000000006,0.309316250654647,0.324310832507047,
0.385391022398012,0.43750000000001,0.46875000000001,0.48437500000001,0.49218750000001,
0.498949346899948,0.50000000000001,0.504583563377448,0.573408589202907,
0.641343695284019,0.680145783129569,0.750000000000005,0.815926487813902,
0.847891275365318,0.914669007590066,0.98071621931426,1.),.UNSPECIFIED.);
#291=B_SPLINE_CURVE_WITH_KNOTS('',3,(#55980,#55981,#55982,#55983,#55984,
#55985,#55986,#55987,#55988,#55989,#55990,#55991,#55992,#55993,#55994,#55995,
#55996,#55997,#55998,#55999,#56000,#56001,#56002,#56003,#56004,#56005,#56006,
#56007,#56008,#56009,#56010,#56011,#56012,#56013,#56014,#56015,#56016,#56017,
#56018,#56019,#56020,#56021,#56022,#56023,#56024,#56025,#56026,#56027,#56028,
#56029,#56030,#56031,#56032,#56033,#56034,#56035,#56036,#56037,#56038,#56039,
#56040,#56041,#56042,#56043,#56044,#56045,#56046,#56047,#56048,#56049,#56050,
#56051,#56052,#56053,#56054,#56055,#56056,#56057,#56058,#56059,#56060,#56061,
#56062,#56063,#56064,#56065,#56066,#56067,#56068,#56069,#56070,#56071,#56072,
#56073,#56074,#56075,#56076,#56077,#56078,#56079,#56080,#56081,#56082,#56083,
#56084,#56085,#56086,#56087,#56088,#56089,#56090,#56091,#56092,#56093,#56094,
#56095,#56096,#56097,#56098,#56099,#56100,#56101,#56102,#56103,#56104,#56105,
#56106,#56107,#56108,#56109,#56110,#56111,#56112,#56113,#56114,#56115,#56116,
#56117,#56118,#56119,#56120,#56121,#56122,#56123,#56124,#56125,#56126,#56127,
#56128,#56129,#56130,#56131,#56132,#56133,#56134,#56135,#56136,#56137,#56138,
#56139,#56140,#56141,#56142,#56143,#56144,#56145),.UNSPECIFIED.,.F.,.F.,
(4,3,3,3,3,3,3,3,3,3,3,3,3,3,3,3,3,3,3,3,3,3,3,3,3,3,3,3,3,3,3,3,3,3,3,
3,3,3,3,3,3,3,3,3,3,3,3,3,3,3,3,3,3,3,3,4),(8.91632442143459E-8,0.0341866199909269,
0.0625000000000018,0.0800113026638258,0.0937500000000027,0.109375000000003,
0.117187500000003,0.121093750000003,0.123046875000003,0.125000000000003,
0.156875028287151,0.187500000000004,0.218750000000004,0.234375000000004,
0.237518692323063,0.242187500000004,0.246093750000004,0.248046875000004,
0.250000000000004,0.290850977616787,0.312500000000003,0.328922102341607,
0.343750000000002,0.359375000000002,0.367187500000002,0.371093750000002,
0.373046875000002,0.375000000000002,0.425211651225354,0.437500000000001,
0.468750000000001,0.484375,0.4921875,0.49609375,0.5,0.520156881116544,0.572597422472742,
0.616913355572735,0.624999999999999,0.651328060799945,0.678222159731897,
0.687499999999998,0.709176140832686,0.749999999999997,0.781249999999997,
0.789062499999997,0.796874999999997,0.799086910214249,0.812499999999997,
0.858396212764482,0.874999999999998,0.885500856041081,0.93268634150154,
0.980790797824736,0.985731883736702,1.),.UNSPECIFIED.);
#292=B_SPLINE_CURVE_WITH_KNOTS('',3,(#56148,#56149,#56150,#56151,#56152,
#56153,#56154,#56155,#56156,#56157,#56158,#56159,#56160,#56161,#56162,#56163,
#56164,#56165,#56166,#56167,#56168,#56169,#56170,#56171,#56172,#56173,#56174,
#56175,#56176,#56177,#56178,#56179,#56180,#56181,#56182,#56183,#56184,#56185,
#56186,#56187,#56188,#56189,#56190,#56191,#56192,#56193,#56194,#56195,#56196,
#56197,#56198,#56199,#56200,#56201,#56202,#56203,#56204,#56205,#56206,#56207,
#56208,#56209,#56210,#56211,#56212,#56213,#56214,#56215,#56216,#56217,#56218,
#56219,#56220,#56221,#56222,#56223,#56224,#56225,#56226,#56227,#56228,#56229,
#56230,#56231,#56232,#56233,#56234,#56235,#56236,#56237,#56238,#56239,#56240,
#56241,#56242,#56243,#56244,#56245,#56246,#56247,#56248,#56249,#56250,#56251,
#56252,#56253,#56254,#56255,#56256,#56257,#56258,#56259,#56260,#56261,#56262,
#56263,#56264,#56265,#56266,#56267,#56268,#56269,#56270,#56271,#56272,#56273,
#56274,#56275,#56276,#56277,#56278,#56279,#56280,#56281,#56282,#56283,#56284,
#56285,#56286,#56287,#56288,#56289),.UNSPECIFIED.,.F.,.F.,(4,3,3,3,3,3,
3,3,3,3,3,3,3,3,3,3,3,3,3,3,3,3,3,3,3,3,3,3,3,3,3,3,3,3,3,3,3,3,3,3,3,3,
3,3,3,3,3,4),(2.34637983009399E-7,0.0315958275913751,0.0628964688330882,
0.093712252016794,0.104172203871702,0.124999999999996,0.154837291401328,
0.184674582802659,0.213175902159575,0.218749999999994,0.234374999999994,
0.242187499999993,0.246093749999993,0.248046874999993,0.249999999999993,
0.257790527886997,0.295642547232279,0.334483529193173,0.354334857867753,
0.39268315304614,0.431398872128228,0.470481931727138,0.482377268318766,
0.484374999999996,0.496585777244764,0.499999999999997,0.540377617220931,
0.580372331573253,0.609455371665288,0.649166188311503,0.687499999999999,
0.700832172519671,0.718749999999999,0.734375,0.7421875,0.74609375,0.748046875,
0.75,0.769091705922879,0.798966915348658,0.828842124774437,0.858577030826336,
0.875,0.896782324096875,0.927914259072886,0.959582459056515,0.985641707363427,
1.),.UNSPECIFIED.);
#293=B_SPLINE_CURVE_WITH_KNOTS('',3,(#56326,#56327,#56328,#56329,#56330,
#56331,#56332,#56333,#56334,#56335,#56336,#56337,#56338,#56339,#56340,#56341,
#56342,#56343,#56344,#56345,#56346,#56347,#56348,#56349,#56350,#56351,#56352,
#56353,#56354,#56355,#56356,#56357,#56358,#56359,#56360,#56361,#56362,#56363,
#56364,#56365,#56366,#56367,#56368,#56369,#56370,#56371,#56372,#56373,#56374,
#56375,#56376,#56377,#56378,#56379,#56380,#56381,#56382,#56383,#56384,#56385,
#56386),.UNSPECIFIED.,.F.,.F.,(4,3,3,3,3,3,3,3,3,3,3,3,3,3,3,3,3,3,3,3,
4),(3.81436950412107E-8,0.0594692249681252,0.119461334964787,0.180335230433945,
0.228233343725019,0.25,0.3125,0.375,0.420629521267839,0.466480442658904,
0.5,0.532982688308766,0.595584374784075,0.657507294105254,0.718468589090622,
0.75,0.809830707906453,0.831293941004929,0.890887152636801,0.949594326669872,
1.),.UNSPECIFIED.);
#294=B_SPLINE_CURVE_WITH_KNOTS('',3,(#56387,#56388,#56389,#56390,#56391,
#56392,#56393,#56394,#56395,#56396,#56397,#56398,#56399,#56400,#56401,#56402,
#56403,#56404,#56405,#56406,#56407,#56408,#56409,#56410,#56411,#56412,#56413,
#56414,#56415,#56416,#56417,#56418,#56419,#56420,#56421,#56422,#56423,#56424,
#56425,#56426,#56427,#56428,#56429,#56430,#56431,#56432,#56433,#56434,#56435,
#56436,#56437,#56438,#56439,#56440,#56441,#56442,#56443,#56444),
 .UNSPECIFIED.,.F.,.F.,(4,3,3,3,3,3,3,3,3,3,3,3,3,3,3,3,3,3,3,4),(0.,0.070136586784253,
0.13603270626599,0.197319690970826,0.25,0.307828697463722,0.364809836743389,
0.421408542734098,0.477602898251202,0.5,0.500034296737292,0.555640241024459,
0.611682773460639,0.668075486783373,0.72514215037561,0.75,0.8125,0.876717029865349,
0.946961303728935,1.),.UNSPECIFIED.);
#295=B_SPLINE_CURVE_WITH_KNOTS('',3,(#56490,#56491,#56492,#56493,#56494,
#56495,#56496,#56497,#56498,#56499,#56500,#56501,#56502,#56503,#56504,#56505,
#56506,#56507,#56508,#56509,#56510,#56511,#56512,#56513,#56514,#56515,#56516,
#56517,#56518,#56519,#56520,#56521,#56522,#56523,#56524,#56525,#56526,#56527,
#56528,#56529,#56530,#56531,#56532,#56533,#56534,#56535,#56536,#56537,#56538,
#56539,#56540,#56541,#56542,#56543,#56544,#56545,#56546,#56547),
 .UNSPECIFIED.,.F.,.F.,(4,3,3,3,3,3,3,3,3,3,3,3,3,3,3,3,3,3,3,4),(0.,0.0625,
0.123429142320394,0.183419124217513,0.242355039406308,0.25,0.308040957847518,
0.365338354022302,0.422299301931396,0.479066994233144,0.535783605802587,
0.592776604825274,0.64999011865553,0.70786098943061,0.75,0.808903052638457,
0.869153547680589,0.930296449526362,0.992905654827065,1.),.UNSPECIFIED.);
#296=B_SPLINE_CURVE_WITH_KNOTS('',3,(#56548,#56549,#56550,#56551,#56552,
#56553,#56554,#56555,#56556,#56557,#56558,#56559,#56560,#56561,#56562,#56563,
#56564,#56565,#56566,#56567,#56568,#56569,#56570,#56571,#56572,#56573,#56574,
#56575,#56576,#56577,#56578,#56579,#56580,#56581,#56582,#56583,#56584,#56585,
#56586,#56587,#56588,#56589,#56590,#56591,#56592,#56593,#56594,#56595,#56596,
#56597,#56598,#56599,#56600,#56601,#56602,#56603,#56604,#56605,#56606,#56607,
#56608,#56609,#56610,#56611,#56612,#56613,#56614,#56615,#56616,#56617,#56618,
#56619,#56620,#56621,#56622,#56623,#56624,#56625,#56626,#56627,#56628,#56629,
#56630,#56631,#56632,#56633,#56634,#56635,#56636,#56637,#56638,#56639,#56640,
#56641,#56642,#56643,#56644),.UNSPECIFIED.,.F.,.F.,(4,3,3,3,3,3,3,3,3,3,
3,3,3,3,3,3,3,3,3,3,3,3,3,3,3,3,3,3,3,3,3,3,4),(0.,0.00285452287324627,
0.0810898927209212,0.124999999999997,0.163513621542303,0.187499999999996,
0.218749999999995,0.234374999999995,0.242187499999995,0.246093749999995,
0.248046874999995,0.249999999999995,0.316063805229939,0.331496676299031,
0.396932120474405,0.461480984752616,0.499909644740874,0.499999999999995,
0.563689652381694,0.624999999999995,0.668335900347379,0.687499999999995,
0.718749999999995,0.734374999999995,0.742187499999995,0.746093749999995,
0.748046874999995,0.749999999999995,0.826034220731771,0.836305307418583,
0.916645663493165,0.996986019567746,1.),.UNSPECIFIED.);
#297=B_SPLINE_CURVE_WITH_KNOTS('',3,(#56683,#56684,#56685,#56686,#56687,
#56688,#56689,#56690,#56691,#56692,#56693,#56694,#56695,#56696,#56697,#56698,
#56699,#56700,#56701,#56702,#56703,#56704,#56705,#56706,#56707,#56708,#56709,
#56710,#56711,#56712,#56713),.UNSPECIFIED.,.F.,.F.,(4,3,3,3,3,3,3,3,3,3,
4),(0.,0.124999999999991,0.187499999999986,0.218749999999983,0.234374999999982,
0.242187499999982,0.249999999999982,0.374999999999986,0.49999999999999,
0.749999999999995,1.),.UNSPECIFIED.);
#298=B_SPLINE_CURVE_WITH_KNOTS('',3,(#56714,#56715,#56716,#56717,#56718,
#56719),.UNSPECIFIED.,.F.,.F.,(4,1,1,4),(0.,0.3333333333333,0.6666666666667,
0.999998328036297),.UNSPECIFIED.);
#299=B_SPLINE_CURVE_WITH_KNOTS('',3,(#56720,#56721,#56722,#56723,#56724,
#56725,#56726,#56727,#56728,#56729,#56730,#56731,#56732,#56733,#56734,#56735,
#56736,#56737,#56738,#56739,#56740,#56741,#56742,#56743,#56744,#56745,#56746,
#56747,#56748,#56749,#56750,#56751,#56752,#56753,#56754,#56755,#56756,#56757,
#56758,#56759,#56760,#56761,#56762,#56763,#56764,#56765,#56766,#56767,#56768,
#56769,#56770,#56771,#56772,#56773,#56774,#56775,#56776,#56777,#56778,#56779,
#56780),.UNSPECIFIED.,.F.,.F.,(4,3,3,3,3,3,3,3,3,3,3,3,3,3,3,3,3,3,3,3,
4),(1.03820017360987E-10,0.0858140043459224,0.198337968205613,0.250000000000019,
0.281117634573999,0.37500000000003,0.437500000000035,0.468750000000038,
0.471374013083689,0.484375000000041,0.492187500000042,0.498687480577556,
0.500000000000043,0.57969855306797,0.655204256162074,0.69128810718509,0.750000000000021,
0.819024361205775,0.881081173000778,0.945467811578077,0.999999999939057),
 .UNSPECIFIED.);
#300=B_SPLINE_CURVE_WITH_KNOTS('',3,(#56823,#56824,#56825,#56826,#56827,
#56828,#56829,#56830,#56831,#56832,#56833,#56834,#56835,#56836,#56837,#56838,
#56839,#56840,#56841,#56842,#56843,#56844,#56845,#56846,#56847,#56848,#56849,
#56850,#56851,#56852,#56853,#56854,#56855,#56856,#56857,#56858,#56859,#56860,
#56861,#56862,#56863,#56864,#56865,#56866,#56867,#56868,#56869,#56870,#56871,
#56872,#56873,#56874,#56875,#56876,#56877,#56878,#56879,#56880,#56881,#56882,
#56883,#56884,#56885,#56886,#56887,#56888,#56889,#56890,#56891,#56892,#56893,
#56894,#56895,#56896,#56897,#56898,#56899,#56900,#56901,#56902,#56903,#56904,
#56905,#56906,#56907,#56908,#56909,#56910,#56911,#56912,#56913),
 .UNSPECIFIED.,.F.,.F.,(4,3,3,3,3,3,3,3,3,3,3,3,3,3,3,3,3,3,3,3,3,3,3,3,
3,3,3,3,3,3,4),(1.98906479309072E-7,0.047089838900463,0.0950876593119024,
0.109526425869498,0.124999999999998,0.176684953882968,0.187499999999997,
0.195574839395448,0.203124999999996,0.218749999999996,0.249999999999996,
0.270621648562703,0.334104108208607,0.398265338859945,0.430414683614596,
0.4375,0.46875,0.484375000000001,0.492187500000001,0.498034123720945,0.500000000000001,
0.55992470032944,0.600124960067209,0.658475261666886,0.7158893297449,0.764250575765468,
0.821849980430899,0.878616137371232,0.918178973503123,0.970962441134751,
1.),.UNSPECIFIED.);
#301=B_SPLINE_CURVE_WITH_KNOTS('',3,(#56956,#56957,#56958,#56959,#56960,
#56961,#56962,#56963,#56964,#56965,#56966,#56967,#56968,#56969,#56970,#56971,
#56972,#56973,#56974,#56975,#56976,#56977),.UNSPECIFIED.,.F.,.F.,(4,3,3,
3,3,3,3,4),(1.63033535856655E-6,0.120934032136536,0.310467016068268,0.5,
0.679851327939551,0.7064121488131,0.883436743746198,1.),.UNSPECIFIED.);
#302=B_SPLINE_CURVE_WITH_KNOTS('',3,(#56979,#56980,#56981,#56982,#56983,
#56984,#56985,#56986,#56987,#56988,#56989),.UNSPECIFIED.,.F.,.F.,(4,1,2,
2,2,4),(0.,0.125,0.1875,0.249999999999999,0.5,1.),.UNSPECIFIED.);
#303=B_SPLINE_CURVE_WITH_KNOTS('',3,(#56990,#56991,#56992,#56993,#56994,
#56995,#56996,#56997,#56998,#56999,#57000,#57001,#57002,#57003,#57004,#57005,
#57006,#57007,#57008,#57009,#57010,#57011,#57012,#57013,#57014,#57015,#57016,
#57017,#57018,#57019,#57020,#57021,#57022,#57023,#57024,#57025,#57026,#57027,
#57028,#57029,#57030,#57031,#57032,#57033,#57034,#57035,#57036,#57037,#57038,
#57039,#57040,#57041,#57042,#57043,#57044),.UNSPECIFIED.,.F.,.F.,(4,3,3,
3,3,3,3,3,3,3,3,3,3,3,3,3,3,3,4),(0.,0.0654580192943895,0.124936971683619,
0.19521642709056,0.250000000000039,0.306913925251286,0.384160992342502,
0.437500000000067,0.468750000000071,0.484375000000072,0.492187500000071,
0.498304651669469,0.50000000000007,0.531997336482634,0.633294429777801,
0.713452211844485,0.819820113326127,0.902138636668165,1.),.UNSPECIFIED.);
#304=B_SPLINE_CURVE_WITH_KNOTS('',3,(#57086,#57087,#57088,#57089,#57090,
#57091,#57092,#57093,#57094,#57095,#57096,#57097,#57098,#57099,#57100,#57101,
#57102,#57103,#57104,#57105,#57106,#57107,#57108,#57109,#57110,#57111,#57112,
#57113,#57114,#57115,#57116,#57117,#57118,#57119,#57120,#57121,#57122,#57123,
#57124,#57125,#57126,#57127,#57128,#57129,#57130,#57131,#57132,#57133,#57134,
#57135,#57136,#57137,#57138,#57139,#57140,#57141,#57142,#57143,#57144,#57145,
#57146,#57147,#57148,#57149,#57150,#57151,#57152,#57153,#57154,#57155,#57156,
#57157,#57158,#57159,#57160,#57161,#57162,#57163,#57164,#57165,#57166,#57167,
#57168,#57169,#57170,#57171,#57172,#57173),.UNSPECIFIED.,.F.,.F.,(4,3,3,
3,3,3,3,3,3,3,3,3,3,3,3,3,3,3,3,3,3,3,3,3,3,3,3,3,3,4),(1.09807446774891E-11,
0.0527820137222502,0.0818213359279545,0.138473123221553,0.195945223360734,
0.235750033133544,0.293012182826601,0.35119340202972,0.399875450857417,
0.437499999999998,0.468749999999998,0.484374999999998,0.492187499999998,
0.496093749999998,0.499508594759178,0.499999999999998,0.565860735503257,
0.629574778776911,0.693958686436161,0.725750994255272,0.781250000000002,
0.790730855827748,0.796875000000002,0.812500000000002,0.8690433465425,0.875000000000002,
0.884835785766576,0.938700830850611,0.993360696887802,0.999999777750431),
 .UNSPECIFIED.);
#305=B_SPLINE_CURVE_WITH_KNOTS('',3,(#57176,#57177,#57178,#57179,#57180,
#57181,#57182,#57183,#57184,#57185,#57186,#57187,#57188,#57189,#57190,#57191,
#57192,#57193,#57194,#57195,#57196,#57197,#57198,#57199,#57200,#57201,#57202,
#57203,#57204,#57205,#57206,#57207,#57208,#57209,#57210,#57211,#57212,#57213,
#57214,#57215,#57216,#57217,#57218,#57219,#57220,#57221,#57222,#57223,#57224,
#57225,#57226,#57227,#57228,#57229,#57230,#57231,#57232,#57233),
 .UNSPECIFIED.,.F.,.F.,(4,3,3,3,3,3,3,3,3,3,3,3,3,3,3,3,3,3,3,4),(1.3581547160307E-11,
0.0585628517632844,0.117996194021253,0.168707832741241,0.228541288466462,
0.25,0.3125,0.375,0.421054296540944,0.467108593081889,0.5,0.563532895370386,
0.62639952166682,0.68822323587103,0.75,0.771768878138407,0.832605908968213,
0.892881465150608,0.952307015390897,0.999999961863706),.UNSPECIFIED.);
#306=B_SPLINE_CURVE_WITH_KNOTS('',3,(#57284,#57285,#57286,#57287,#57288,
#57289,#57290,#57291,#57292,#57293,#57294,#57295,#57296,#57297,#57298,#57299,
#57300,#57301,#57302,#57303,#57304,#57305,#57306,#57307,#57308,#57309,#57310,
#57311,#57312,#57313,#57314,#57315,#57316,#57317,#57318,#57319,#57320,#57321,
#57322,#57323,#57324,#57325,#57326,#57327,#57328,#57329,#57330,#57331,#57332,
#57333,#57334,#57335,#57336,#57337,#57338,#57339,#57340,#57341,#57342,#57343,
#57344,#57345,#57346,#57347,#57348,#57349,#57350,#57351,#57352,#57353,#57354,
#57355,#57356,#57357,#57358,#57359,#57360,#57361,#57362,#57363,#57364,#57365,
#57366,#57367,#57368,#57369,#57370,#57371,#57372,#57373,#57374,#57375,#57376,
#57377,#57378,#57379,#57380,#57381,#57382,#57383,#57384,#57385,#57386,#57387,
#57388,#57389,#57390,#57391,#57392,#57393,#57394,#57395,#57396,#57397,#57398,
#57399,#57400,#57401,#57402,#57403,#57404,#57405,#57406,#57407,#57408,#57409,
#57410,#57411,#57412,#57413,#57414,#57415,#57416,#57417,#57418,#57419,#57420,
#57421,#57422,#57423,#57424,#57425,#57426,#57427,#57428,#57429,#57430,#57431,
#57432,#57433,#57434,#57435,#57436,#57437,#57438,#57439,#57440,#57441,#57442,
#57443,#57444,#57445,#57446,#57447,#57448,#57449,#57450,#57451,#57452,#57453,
#57454,#57455,#57456,#57457,#57458,#57459,#57460,#57461,#57462,#57463,#57464,
#57465,#57466,#57467,#57468,#57469,#57470,#57471,#57472,#57473,#57474,#57475,
#57476,#57477,#57478,#57479,#57480,#57481,#57482,#57483,#57484,#57485,#57486,
#57487,#57488,#57489,#57490,#57491,#57492,#57493,#57494,#57495,#57496,#57497,
#57498,#57499,#57500,#57501,#57502,#57503,#57504,#57505,#57506,#57507,#57508,
#57509,#57510,#57511,#57512,#57513,#57514,#57515,#57516,#57517,#57518,#57519,
#57520,#57521,#57522,#57523,#57524),.UNSPECIFIED.,.F.,.F.,(4,3,3,3,3,3,
3,3,3,3,3,3,3,3,3,3,3,3,3,3,3,3,3,3,3,3,3,3,3,3,3,3,3,3,3,3,3,3,3,3,3,3,
3,3,3,3,3,3,3,3,3,3,3,3,3,3,3,3,3,3,3,3,3,3,3,3,3,3,3,3,3,3,3,3,3,3,3,3,
3,3,4),(9.74886797225189E-8,0.0159200057310286,0.0312500000000033,0.0468750000000049,
0.0546875000000058,0.0585937500000062,0.0625000000000067,0.0648608916794454,
0.0837424285003968,0.10256194479458,0.109375000000012,0.117187500000013,
0.121093750000014,0.123046875000014,0.124023437500014,0.124511718750014,
0.125000000000014,0.130881132752826,0.145623337610177,0.160279740114716,
0.171875000000021,0.179687500000022,0.183593750000023,0.185546875000023,
0.186523437500023,0.187500000000023,0.198322293156087,0.209103042320687,
0.21345235022535,0.224198983639946,0.234874955076149,0.242187500000008,
0.246093750000007,0.248046875000007,0.249023437500007,0.249755859375006,
0.250000000000006,0.286128141198425,0.331147428259678,0.373117414469576,
0.413937461021449,0.442038759456119,0.468750000000021,0.484375000000022,
0.492187500000022,0.496093750000022,0.498046875000023,0.498807395625069,
0.499023437500023,0.499511718750023,0.500000000000023,0.527809509355821,
0.555636888410823,0.580222747550704,0.608292500146189,0.634707899498602,
0.64062500000002,0.645734467803367,0.64843750000002,0.665746267512998,0.677886461833895,
0.695389012135111,0.712977524146475,0.730654944749156,0.734375000000017,
0.742187500000017,0.746093750000017,0.748046875000017,0.749023437500017,
0.749511718750016,0.750000000000016,0.752487431440223,0.79797765669168,
0.804136709872947,0.850539441899368,0.858789252586812,0.906288883068206,
0.920205788951179,0.968988610235553,0.993036230319091,1.),.UNSPECIFIED.);
#307=B_SPLINE_CURVE_WITH_KNOTS('',3,(#57607,#57608,#57609,#57610,#57611,
#57612,#57613,#57614,#57615,#57616,#57617,#57618,#57619,#57620,#57621,#57622,
#57623,#57624,#57625,#57626,#57627,#57628,#57629,#57630,#57631,#57632,#57633,
#57634,#57635,#57636,#57637,#57638,#57639,#57640,#57641,#57642,#57643,#57644,
#57645,#57646,#57647,#57648,#57649,#57650,#57651,#57652,#57653,#57654,#57655,
#57656,#57657,#57658,#57659,#57660,#57661,#57662,#57663,#57664,#57665,#57666,
#57667,#57668,#57669,#57670,#57671,#57672,#57673,#57674,#57675,#57676,#57677,
#57678,#57679,#57680,#57681,#57682,#57683,#57684,#57685,#57686,#57687,#57688,
#57689,#57690,#57691,#57692,#57693,#57694,#57695,#57696,#57697,#57698,#57699,
#57700,#57701,#57702,#57703,#57704,#57705,#57706,#57707,#57708,#57709,#57710,
#57711,#57712,#57713,#57714,#57715,#57716,#57717,#57718,#57719,#57720,#57721,
#57722,#57723,#57724,#57725,#57726,#57727,#57728,#57729,#57730,#57731,#57732,
#57733,#57734,#57735,#57736,#57737,#57738,#57739,#57740,#57741,#57742,#57743,
#57744,#57745,#57746,#57747,#57748,#57749,#57750,#57751,#57752,#57753,#57754,
#57755,#57756,#57757,#57758,#57759,#57760,#57761,#57762,#57763),
 .UNSPECIFIED.,.F.,.F.,(4,3,3,3,3,3,3,3,3,3,3,3,3,3,3,3,3,3,3,3,3,3,3,3,
3,3,3,3,3,3,3,3,3,3,3,3,3,3,3,3,3,3,3,3,3,3,3,3,3,3,3,3,4),(1.72726420505883E-7,
0.0434573133218831,0.0863338476385245,0.0932165176868182,0.124999999999984,
0.165840010671867,0.177272924281379,0.187499999999975,0.218749999999971,
0.234374999999969,0.242187499999968,0.246093749999968,0.249511718749968,
0.249999999999968,0.260112843085009,0.284904274190472,0.309601369212814,
0.312499999999972,0.336932313817438,0.343749999999975,0.359374999999976,
0.359741422647275,0.367187499999977,0.371093749999977,0.373046874999977,
0.374023437499977,0.374999999999977,0.427161994615482,0.43749999999998,
0.446539510208758,0.468749999999981,0.484374999999982,0.492187499999982,
0.499058230973304,0.499999999999982,0.529373135558788,0.59548946583794,
0.601625599175875,0.624999999999987,0.666787835011863,0.687499999999989,
0.718749999999991,0.726755886335713,0.734374999999991,0.746093749999992,
0.749999999999992,0.777566191087922,0.821931417049227,0.864144998003108,
0.906142061190345,0.949726796235432,0.99591887464429,0.99999995601045),
 .UNSPECIFIED.);
#308=B_SPLINE_CURVE_WITH_KNOTS('',3,(#57808,#57809,#57810,#57811,#57812,
#57813,#57814,#57815,#57816,#57817,#57818,#57819,#57820,#57821,#57822,#57823,
#57824,#57825,#57826,#57827,#57828,#57829,#57830,#57831,#57832,#57833,#57834,
#57835,#57836,#57837,#57838),.UNSPECIFIED.,.F.,.F.,(4,3,3,3,3,3,3,3,3,3,
4),(0.,0.12500000000001,0.187500000000016,0.218750000000019,0.23437500000002,
0.24218750000002,0.250000000000019,0.375000000000015,0.500000000000012,
0.750000000000006,1.),.UNSPECIFIED.);
#309=B_SPLINE_CURVE_WITH_KNOTS('',3,(#57840,#57841,#57842,#57843,#57844,
#57845,#57846,#57847,#57848,#57849,#57850,#57851,#57852,#57853,#57854,#57855,
#57856,#57857,#57858,#57859,#57860,#57861),.UNSPECIFIED.,.F.,.F.,(4,3,3,
3,3,3,3,4),(0.,0.177097147826628,0.275749264676803,0.455644332730437,0.5,
0.682209113428456,0.858274289412511,0.999997472817192),.UNSPECIFIED.);
#310=B_SPLINE_CURVE_WITH_KNOTS('',3,(#57864,#57865,#57866,#57867,#57868,
#57869,#57870,#57871,#57872,#57873,#57874,#57875,#57876,#57877,#57878,#57879,
#57880,#57881,#57882,#57883,#57884,#57885,#57886,#57887,#57888,#57889,#57890,
#57891,#57892,#57893,#57894,#57895,#57896,#57897,#57898,#57899,#57900,#57901,
#57902,#57903,#57904,#57905,#57906,#57907,#57908,#57909,#57910,#57911,#57912,
#57913,#57914,#57915,#57916,#57917,#57918,#57919,#57920,#57921,#57922,#57923,
#57924),.UNSPECIFIED.,.F.,.F.,(4,3,3,3,3,3,3,3,3,3,3,3,3,3,3,3,3,3,3,3,
4),(4.66155616960519E-11,0.0921586796163419,0.199885250793164,0.250000000000005,
0.280572529806289,0.383374079103984,0.437500000000011,0.462355616577624,
0.468750000000013,0.484375000000013,0.492187500000013,0.497992587906964,
0.500000000000012,0.580654371451503,0.656974867867654,0.686606159361902,
0.750000000000006,0.819755880055471,0.86988546566209,0.934942732831045,
1.),.UNSPECIFIED.);
#311=B_SPLINE_CURVE_WITH_KNOTS('',3,(#57969,#57970,#57971,#57972,#57973,
#57974,#57975,#57976,#57977,#57978,#57979,#57980,#57981,#57982,#57983,#57984,
#57985,#57986,#57987,#57988,#57989,#57990,#57991,#57992,#57993,#57994,#57995,
#57996,#57997,#57998,#57999,#58000,#58001,#58002,#58003,#58004,#58005,#58006,
#58007,#58008,#58009,#58010,#58011,#58012,#58013,#58014,#58015,#58016,#58017,
#58018,#58019,#58020,#58021,#58022,#58023,#58024,#58025,#58026,#58027,#58028,
#58029,#58030,#58031,#58032,#58033,#58034,#58035,#58036,#58037,#58038),
 .UNSPECIFIED.,.F.,.F.,(4,3,3,3,3,3,3,3,3,3,3,3,3,3,3,3,3,3,3,3,3,3,3,4),
(0.,0.0436825095638117,0.0764111191893734,0.120245151483468,0.125,0.179962620917879,
0.223835356219091,0.25,0.320059900246058,0.371520369880292,0.375,0.470560244901238,
0.5,0.519394870044145,0.625,0.667284556549449,0.741667232712626,0.75,0.808039637089994,
0.814941565966665,0.875,0.919746518961679,0.962447676468616,0.999999720259698),
 .UNSPECIFIED.);
#312=B_SPLINE_CURVE_WITH_KNOTS('',3,(#58039,#58040,#58041,#58042,#58043,
#58044,#58045,#58046,#58047,#58048,#58049,#58050,#58051,#58052,#58053,#58054,
#58055,#58056,#58057,#58058,#58059,#58060,#58061,#58062,#58063,#58064,#58065,
#58066,#58067,#58068,#58069,#58070,#58071,#58072,#58073,#58074,#58075,#58076,
#58077,#58078,#58079,#58080,#58081,#58082,#58083,#58084,#58085,#58086,#58087,
#58088,#58089,#58090,#58091,#58092,#58093,#58094,#58095,#58096,#58097,#58098,
#58099,#58100,#58101,#58102,#58103,#58104,#58105,#58106,#58107,#58108),
 .UNSPECIFIED.,.F.,.F.,(4,3,3,3,3,3,3,3,3,3,3,3,3,3,3,3,3,3,3,3,3,3,3,4),
(0.,0.0642447928422595,0.129222307761572,0.139648855540338,0.203363599061252,
0.250000000000004,0.300656405338484,0.369078202669245,0.437500000000007,
0.468750000000007,0.469712015730873,0.484375000000006,0.495155221973674,
0.500000000000006,0.563334839048207,0.625631000054916,0.644015069360023,
0.704247356561986,0.750000000000003,0.80787939926093,0.868482237357585,
0.928163376395018,0.961961767983911,0.999999992445097),.UNSPECIFIED.);
#313=B_SPLINE_CURVE_WITH_KNOTS('',3,(#58144,#58145,#58146,#58147,#58148,
#58149,#58150,#58151,#58152,#58153,#58154,#58155,#58156,#58157,#58158,#58159,
#58160,#58161,#58162,#58163,#58164,#58165,#58166,#58167,#58168,#58169,#58170,
#58171,#58172,#58173,#58174,#58175,#58176,#58177,#58178,#58179,#58180,#58181,
#58182,#58183,#58184,#58185,#58186,#58187,#58188,#58189,#58190,#58191,#58192,
#58193,#58194,#58195,#58196,#58197,#58198,#58199,#58200,#58201),
 .UNSPECIFIED.,.F.,.F.,(4,3,3,3,3,3,3,3,3,3,3,3,3,3,3,3,3,3,3,4),(6.48487790812236E-12,
0.0708156629893494,0.137202248264932,0.198838711004642,0.25,0.306727758080084,
0.362644355852727,0.418198532410901,0.473365958253842,0.5,0.500000490542878,
0.555648115907319,0.611778291583337,0.668285949116982,0.725508796212218,
0.75,0.8125,0.877120927925331,0.947966479212715,1.),.UNSPECIFIED.);
#314=B_SPLINE_CURVE_WITH_KNOTS('',3,(#58238,#58239,#58240,#58241,#58242,
#58243,#58244,#58245,#58246,#58247,#58248,#58249,#58250,#58251,#58252,#58253,
#58254,#58255,#58256,#58257,#58258,#58259,#58260,#58261,#58262,#58263,#58264,
#58265,#58266,#58267,#58268,#58269,#58270,#58271,#58272,#58273,#58274,#58275,
#58276,#58277,#58278,#58279,#58280,#58281,#58282,#58283,#58284,#58285,#58286,
#58287,#58288,#58289,#58290,#58291,#58292,#58293,#58294,#58295,#58296,#58297,
#58298,#58299,#58300,#58301,#58302,#58303,#58304,#58305,#58306,#58307,#58308,
#58309,#58310,#58311,#58312,#58313),.UNSPECIFIED.,.F.,.F.,(4,3,3,3,3,3,
3,3,3,3,3,3,3,3,3,3,3,3,3,3,3,3,3,3,3,4),(0.,0.081446458091042,0.125,0.125095970230205,
0.1875,0.21875,0.234375,0.244468168526415,0.25,0.312288980304435,0.384238156676023,
0.456663011015709,0.5,0.500013819131351,0.570973042205914,0.625,0.6875,
0.687743582276575,0.71875,0.734375,0.74450304915607,0.75,0.825461747691051,
0.874925048178083,0.950952013946258,1.),.UNSPECIFIED.);
#315=B_SPLINE_CURVE_WITH_KNOTS('',3,(#58360,#58361,#58362,#58363,#58364,
#58365,#58366,#58367,#58368,#58369,#58370,#58371,#58372,#58373,#58374,#58375,
#58376,#58377,#58378,#58379,#58380,#58381,#58382,#58383,#58384,#58385,#58386,
#58387,#58388,#58389,#58390,#58391,#58392,#58393,#58394,#58395,#58396,#58397,
#58398,#58399,#58400,#58401,#58402,#58403,#58404,#58405,#58406,#58407,#58408,
#58409,#58410,#58411,#58412,#58413,#58414,#58415,#58416,#58417,#58418,#58419,
#58420,#58421,#58422,#58423,#58424,#58425,#58426,#58427,#58428,#58429,#58430,
#58431,#58432),.UNSPECIFIED.,.F.,.F.,(4,3,3,3,3,3,3,3,3,3,3,3,3,3,3,3,3,
3,3,3,3,3,3,3,4),(1.45289839851345E-9,0.0431123229967307,0.0863131612725165,
0.129361940334382,0.1428571428571,0.153622117526577,0.204599112173322,0.255683858334241,
0.2857142857143,0.306349830038087,0.370801333218286,0.4285714285714,0.45934656340666,
0.52650199371959,0.5714285714286,0.612403301821111,0.676566210914991,0.7142857142857,
0.765276968910288,0.818291465317779,0.8571428571429,0.900814068173372,0.918051237057175,
0.961570018597272,1.),.UNSPECIFIED.);
#316=B_SPLINE_CURVE_WITH_KNOTS('',3,(#58436,#58437,#58438,#58439,#58440,
#58441,#58442,#58443,#58444,#58445,#58446,#58447,#58448,#58449,#58450,#58451,
#58452,#58453,#58454,#58455,#58456,#58457,#58458,#58459,#58460,#58461,#58462,
#58463,#58464,#58465,#58466,#58467,#58468,#58469,#58470,#58471,#58472,#58473,
#58474,#58475,#58476,#58477,#58478,#58479,#58480,#58481,#58482,#58483,#58484,
#58485,#58486,#58487,#58488,#58489,#58490,#58491,#58492,#58493,#58494,#58495,
#58496,#58497,#58498,#58499,#58500,#58501,#58502,#58503,#58504,#58505,#58506,
#58507,#58508),.UNSPECIFIED.,.F.,.F.,(4,3,3,3,3,3,3,3,3,3,3,3,3,3,3,3,3,
3,3,3,3,3,3,3,4),(0.,0.0558892464250319,0.112669224042606,0.15695313080606,
0.215051924639428,0.250000000000001,0.309316237904606,0.324310163867534,
0.385390337781192,0.437500000000002,0.468750000000002,0.484375000000003,
0.492187500000003,0.498949343333879,0.500000000000003,0.504582992891419,
0.573408026528877,0.641343139401869,0.680145623339031,0.750000000000002,
0.815926508015868,0.847891709112523,0.914669427968693,0.980716642894602,
1.),.UNSPECIFIED.);
#317=B_SPLINE_CURVE_WITH_KNOTS('',3,(#58509,#58510,#58511,#58512,#58513,
#58514,#58515,#58516,#58517,#58518,#58519,#58520,#58521,#58522,#58523,#58524,
#58525,#58526,#58527,#58528,#58529,#58530,#58531,#58532,#58533,#58534,#58535,
#58536,#58537,#58538,#58539,#58540,#58541,#58542,#58543,#58544,#58545,#58546,
#58547,#58548,#58549,#58550,#58551,#58552,#58553,#58554,#58555,#58556,#58557,
#58558,#58559,#58560,#58561,#58562,#58563,#58564,#58565,#58566),
 .UNSPECIFIED.,.F.,.F.,(4,3,3,3,3,3,3,3,3,3,3,3,3,3,3,3,3,3,3,4),(2.0837214114929E-13,
0.0546995064401617,0.111292609133422,0.169067321533811,0.228833933582854,
0.249999999999952,0.315860528667816,0.374999999999929,0.437499999999917,
0.468749999999912,0.48437499999991,0.49218749999991,0.498919423983201,0.49999999999991,
0.594327222529717,0.691604111918216,0.793562197925487,0.87730889011914,
0.981274245474638,1.),.UNSPECIFIED.);
#318=B_SPLINE_CURVE_WITH_KNOTS('',3,(#58604,#58605,#58606,#58607,#58608,
#58609,#58610,#58611,#58612,#58613,#58614,#58615,#58616,#58617,#58618,#58619,
#58620,#58621,#58622,#58623,#58624,#58625,#58626,#58627,#58628,#58629,#58630,
#58631,#58632,#58633,#58634,#58635,#58636,#58637,#58638,#58639,#58640,#58641,
#58642,#58643,#58644,#58645,#58646,#58647,#58648,#58649,#58650,#58651,#58652,
#58653,#58654,#58655,#58656,#58657,#58658,#58659,#58660,#58661),
 .UNSPECIFIED.,.F.,.F.,(4,3,3,3,3,3,3,3,3,3,3,3,3,3,3,3,3,3,3,4),(0.,0.0625,
0.123435565785335,0.183431668501261,0.242373265682533,0.25,0.30803982181753,
0.365336089158461,0.42229589810465,0.479062430264781,0.535777853356141,
0.59276962932548,0.649981899303138,0.707851544831901,0.75,0.808902168984071,
0.869151867693713,0.930294043556206,0.992902673504759,1.),.UNSPECIFIED.);
#319=B_SPLINE_CURVE_WITH_KNOTS('',3,(#58663,#58664,#58665,#58666,#58667,
#58668,#58669,#58670,#58671,#58672,#58673,#58674,#58675,#58676,#58677,#58678,
#58679,#58680,#58681,#58682,#58683,#58684,#58685,#58686,#58687),
 .UNSPECIFIED.,.F.,.F.,(4,3,3,3,3,3,3,3,4),(1.09119041741671E-6,0.173330994215996,
0.218339178824648,0.3333333333333,0.61546897963696,0.6666666666667,0.781166266027237,
0.949153050471761,1.),.UNSPECIFIED.);
#320=B_SPLINE_CURVE_WITH_KNOTS('',3,(#58688,#58689,#58690,#58691,#58692,
#58693,#58694,#58695,#58696,#58697,#58698,#58699,#58700),.UNSPECIFIED.,
 .F.,.F.,(4,3,3,3,4),(0.,0.1875,0.25,0.500000000000001,1.),
 .UNSPECIFIED.);
#321=B_SPLINE_CURVE_WITH_KNOTS('',3,(#58747,#58748,#58749,#58750,#58751,
#58752,#58753,#58754,#58755,#58756,#58757,#58758,#58759,#58760,#58761,#58762,
#58763,#58764,#58765,#58766,#58767,#58768,#58769,#58770,#58771,#58772,#58773,
#58774,#58775,#58776,#58777,#58778,#58779,#58780,#58781,#58782,#58783,#58784,
#58785,#58786,#58787,#58788,#58789,#58790,#58791,#58792,#58793,#58794,#58795,
#58796,#58797,#58798,#58799,#58800,#58801,#58802,#58803,#58804),
 .UNSPECIFIED.,.F.,.F.,(4,3,3,3,3,3,3,3,3,3,3,3,3,3,3,3,3,3,3,4),(0.,0.0625,
0.123429189990172,0.183419216265491,0.24235517342882,0.25,0.308040963404769,
0.365338364834653,0.422299317831246,0.479067015070969,0.53578363144022,
0.592776635003554,0.649990153248546,0.70786102805877,0.75,0.808903163413945,
0.869153777952148,0.930296804862004,0.992906138380765,1.),.UNSPECIFIED.);
#322=B_SPLINE_CURVE_WITH_KNOTS('',3,(#58805,#58806,#58807,#58808,#58809,
#58810,#58811,#58812,#58813,#58814,#58815,#58816,#58817,#58818,#58819,#58820,
#58821,#58822,#58823,#58824,#58825,#58826,#58827,#58828,#58829,#58830,#58831,
#58832,#58833,#58834,#58835,#58836,#58837,#58838,#58839,#58840,#58841,#58842,
#58843,#58844,#58845,#58846,#58847,#58848,#58849,#58850,#58851,#58852,#58853,
#58854,#58855,#58856,#58857,#58858,#58859,#58860,#58861,#58862,#58863,#58864,
#58865,#58866,#58867,#58868,#58869,#58870,#58871,#58872,#58873,#58874,#58875,
#58876,#58877,#58878,#58879,#58880,#58881,#58882,#58883,#58884,#58885,#58886,
#58887,#58888,#58889,#58890,#58891,#58892,#58893,#58894,#58895,#58896,#58897,
#58898),.UNSPECIFIED.,.F.,.F.,(4,3,3,3,3,3,3,3,3,3,3,3,3,3,3,3,3,3,3,3,
3,3,3,3,3,3,3,3,3,3,3,4),(0.,0.00359421609921195,0.0901499213363355,0.124999999999999,
0.163074003856875,0.187499999999999,0.218749999999998,0.234374999999998,
0.242187499999998,0.246093749999998,0.248046874999998,0.249999999999998,
0.315877948487601,0.331449187946985,0.3964014492295,0.461540192267028,0.499908689841259,
0.499999999999999,0.564252115945543,0.625,0.668380810462763,0.6875,0.71875,
0.734375000000001,0.742187500000001,0.746093750000001,0.748046875000001,
0.750000000000001,0.836745522375066,0.920992550643248,0.99624855591021,
1.),.UNSPECIFIED.);
#323=B_SPLINE_CURVE_WITH_KNOTS('',3,(#58899,#58900,#58901,#58902,#58903,
#58904,#58905,#58906,#58907,#58908,#58909,#58910,#58911,#58912,#58913,#58914,
#58915,#58916,#58917,#58918,#58919,#58920,#58921,#58922,#58923,#58924,#58925,
#58926,#58927,#58928,#58929,#58930,#58931,#58932,#58933,#58934,#58935,#58936,
#58937,#58938,#58939,#58940,#58941,#58942,#58943,#58944,#58945,#58946,#58947,
#58948,#58949,#58950,#58951,#58952,#58953,#58954,#58955,#58956),
 .UNSPECIFIED.,.F.,.F.,(4,3,3,3,3,3,3,3,3,3,3,3,3,3,3,3,3,3,3,4),(0.,0.0701503128262514,
0.136056545864733,0.197350793223507,0.25,0.307839026190954,0.364828669625009,
0.421434874490469,0.477635358311654,0.5,0.500034575059412,0.555642599320633,
0.611688567793988,0.668085517949893,0.725157605455238,0.75,0.8125,0.876726864335634,
0.946985567133671,1.),.UNSPECIFIED.);
#324=B_SPLINE_CURVE_WITH_KNOTS('',3,(#58993,#58994,#58995,#58996,#58997,
#58998,#58999,#59000,#59001,#59002,#59003,#59004,#59005,#59006,#59007,#59008,
#59009,#59010,#59011,#59012,#59013,#59014,#59015,#59016,#59017,#59018,#59019,
#59020,#59021,#59022,#59023,#59024,#59025,#59026,#59027,#59028,#59029,#59030,
#59031,#59032,#59033,#59034,#59035,#59036,#59037,#59038,#59039,#59040,#59041,
#59042,#59043,#59044,#59045,#59046,#59047,#59048,#59049,#59050,#59051,#59052,
#59053,#59054,#59055,#59056,#59057,#59058,#59059,#59060,#59061,#59062,#59063,
#59064,#59065,#59066,#59067,#59068,#59069,#59070,#59071,#59072,#59073,#59074,
#59075,#59076,#59077,#59078,#59079,#59080,#59081,#59082,#59083,#59084,#59085,
#59086,#59087,#59088,#59089,#59090,#59091,#59092,#59093,#59094,#59095,#59096,
#59097,#59098,#59099,#59100,#59101,#59102,#59103,#59104,#59105,#59106,#59107,
#59108,#59109,#59110,#59111,#59112,#59113,#59114,#59115,#59116),
 .UNSPECIFIED.,.F.,.F.,(4,3,3,3,3,3,3,3,3,3,3,3,3,3,3,3,3,3,3,3,3,3,3,3,
3,3,3,3,3,3,3,3,3,3,3,3,3,3,3,3,3,4),(2.34638652342419E-7,0.0312501759789898,
0.0620856368219447,0.0935428184109735,0.125000000000002,0.156250000000003,
0.187500000000003,0.218750000000004,0.234375000000004,0.242187500000004,
0.246093750000004,0.248046875000004,0.250000000000004,0.298059640401285,
0.343846953199899,0.375000000000004,0.41630338916026,0.437500000000004,
0.468750000000004,0.484375000000004,0.496666652157399,0.499736069550179,
0.500000000000004,0.542051437923008,0.584507507123047,0.625000000000003,
0.671672548344778,0.687500000000003,0.718750000000003,0.734375000000003,
0.742187500000003,0.746093750000003,0.748046875000003,0.750000000000003,
0.781250000000003,0.811342334720831,0.843171167360416,0.875000000000002,
0.906250000000001,0.937257522432499,0.968641912191417,1.),.UNSPECIFIED.);
#325=B_SPLINE_CURVE_WITH_KNOTS('',3,(#59117,#59118,#59119,#59120,#59121,
#59122,#59123,#59124,#59125,#59126,#59127,#59128,#59129,#59130,#59131,#59132,
#59133,#59134,#59135,#59136,#59137,#59138,#59139,#59140,#59141,#59142,#59143,
#59144,#59145,#59146,#59147,#59148,#59149,#59150,#59151,#59152,#59153,#59154,
#59155,#59156,#59157,#59158,#59159,#59160,#59161,#59162,#59163,#59164,#59165,
#59166,#59167,#59168,#59169,#59170,#59171,#59172,#59173,#59174,#59175,#59176,
#59177),.UNSPECIFIED.,.F.,.F.,(4,3,3,3,3,3,3,3,3,3,3,3,3,3,3,3,3,3,3,3,
4),(3.81433860989148E-8,0.0594692343242972,0.119461353578183,0.180335258041045,
0.228233351338028,0.25,0.3125,0.375,0.420629587711987,0.46648057363459,
0.5,0.532982690390264,0.595584385518065,0.657507313747222,0.718468618098683,
0.75,0.809830728585965,0.831293935547951,0.890887163314741,0.94959436212385,
1.),.UNSPECIFIED.);
#326=B_SPLINE_CURVE_WITH_KNOTS('',3,(#59245,#59246,#59247,#59248,#59249,
#59250,#59251,#59252,#59253,#59254,#59255,#59256,#59257,#59258,#59259,#59260,
#59261,#59262,#59263,#59264,#59265,#59266,#59267,#59268,#59269,#59270,#59271,
#59272,#59273,#59274,#59275,#59276,#59277,#59278,#59279,#59280,#59281,#59282,
#59283,#59284,#59285,#59286,#59287,#59288,#59289,#59290,#59291,#59292,#59293,
#59294,#59295,#59296,#59297,#59298,#59299,#59300,#59301,#59302,#59303,#59304,
#59305,#59306,#59307,#59308,#59309,#59310,#59311,#59312,#59313,#59314,#59315,
#59316,#59317,#59318,#59319,#59320,#59321,#59322,#59323,#59324,#59325,#59326,
#59327,#59328,#59329,#59330,#59331,#59332,#59333,#59334,#59335,#59336,#59337,
#59338,#59339,#59340,#59341,#59342,#59343,#59344,#59345,#59346,#59347,#59348,
#59349,#59350,#59351,#59352,#59353,#59354,#59355,#59356,#59357,#59358,#59359,
#59360,#59361,#59362,#59363,#59364,#59365,#59366,#59367,#59368,#59369,#59370,
#59371,#59372,#59373,#59374,#59375,#59376,#59377,#59378,#59379,#59380,#59381,
#59382,#59383,#59384,#59385,#59386,#59387,#59388,#59389,#59390,#59391,#59392,
#59393,#59394,#59395,#59396,#59397,#59398,#59399,#59400,#59401,#59402,#59403,
#59404,#59405,#59406,#59407,#59408,#59409,#59410),.UNSPECIFIED.,.F.,.F.,
(4,3,3,3,3,3,3,3,3,3,3,3,3,3,3,3,3,3,3,3,3,3,3,3,3,3,3,3,3,3,3,3,3,3,3,
3,3,3,3,3,3,3,3,3,3,3,3,3,3,3,3,3,3,3,3,4),(8.92126295307914E-8,0.0341935387179955,
0.0625000000000023,0.0800482297466476,0.0937500000000034,0.109375000000004,
0.117187500000004,0.121093750000004,0.123046875000004,0.125000000000004,
0.156938379731607,0.187500000000001,0.21875,0.234374999999999,0.237595027422283,
0.242187499999999,0.246093749999998,0.248046874999998,0.249999999999998,
0.290857013627676,0.312499999999998,0.328976223561752,0.343749999999998,
0.359374999999998,0.367187499999998,0.371093749999998,0.373046874999998,
0.374999999999998,0.425244790370268,0.437499999999998,0.468749999999998,
0.484374999999998,0.492187499999998,0.496093749999998,0.499999999999998,
0.520144459031146,0.572559628884996,0.616875406841374,0.624999999999999,
0.65137052874562,0.678310089621322,0.687499999999999,0.709129374678632,
0.749999999999999,0.781249999999999,0.789062499999999,0.796875,0.799044011249208,
0.8125,0.858407509871286,0.875,0.885476739305792,0.932673117967918,0.980788676053958,
0.985729040830903,1.),.UNSPECIFIED.);
#327=B_SPLINE_CURVE_WITH_KNOTS('',3,(#59464,#59465,#59466,#59467,#59468,
#59469,#59470,#59471,#59472,#59473,#59474,#59475,#59476,#59477,#59478,#59479,
#59480,#59481,#59482,#59483,#59484,#59485,#59486,#59487,#59488,#59489,#59490,
#59491,#59492,#59493,#59494,#59495,#59496,#59497,#59498,#59499,#59500,#59501,
#59502,#59503,#59504,#59505,#59506,#59507,#59508,#59509,#59510,#59511,#59512,
#59513,#59514,#59515,#59516,#59517,#59518,#59519,#59520,#59521,#59522,#59523,
#59524,#59525,#59526,#59527,#59528,#59529,#59530,#59531,#59532,#59533,#59534,
#59535,#59536,#59537,#59538,#59539,#59540,#59541,#59542,#59543,#59544,#59545,
#59546,#59547,#59548,#59549,#59550,#59551,#59552,#59553,#59554,#59555,#59556,
#59557,#59558,#59559,#59560,#59561,#59562,#59563,#59564,#59565,#59566,#59567,
#59568,#59569,#59570,#59571,#59572,#59573,#59574,#59575,#59576,#59577,#59578,
#59579,#59580,#59581,#59582,#59583,#59584,#59585,#59586,#59587,#59588,#59589,
#59590,#59591,#59592,#59593,#59594,#59595,#59596,#59597,#59598,#59599,#59600,
#59601,#59602,#59603,#59604,#59605,#59606,#59607,#59608,#59609,#59610,#59611,
#59612,#59613,#59614,#59615,#59616,#59617,#59618,#59619,#59620,#59621,#59622,
#59623,#59624,#59625,#59626,#59627,#59628,#59629,#59630,#59631,#59632,#59633,
#59634,#59635,#59636,#59637,#59638,#59639,#59640,#59641,#59642,#59643,#59644,
#59645,#59646,#59647,#59648,#59649,#59650,#59651,#59652,#59653,#59654,#59655,
#59656,#59657,#59658,#59659,#59660,#59661,#59662,#59663,#59664,#59665,#59666,
#59667,#59668,#59669,#59670,#59671,#59672,#59673,#59674,#59675,#59676,#59677),
 .UNSPECIFIED.,.F.,.F.,(4,3,3,3,3,3,3,3,3,3,3,3,3,3,3,3,3,3,3,3,3,3,3,3,
3,3,3,3,3,3,3,3,3,3,3,3,3,3,3,3,3,3,3,3,3,3,3,3,3,3,3,3,3,3,3,3,3,3,3,3,
3,3,3,3,3,3,3,3,3,3,3,4),(1.24252210392226E-7,0.0158962995490016,0.0300344810503092,
0.0432269198228004,0.0555827596438185,0.0625000000000163,0.0703125000000184,
0.0712890625000187,0.0722656250000189,0.0742187500000193,0.0781250000000199,
0.0927960918760498,0.093750000000022,0.10750217113599,0.109375000000024,
0.117187500000025,0.121093750000026,0.123046875000026,0.124023437500026,
0.125000000000026,0.145668040803103,0.156250000000028,0.171875000000029,
0.17968750000003,0.186599973254188,0.18750000000003,0.218750000000033,0.234375000000035,
0.242187500000036,0.249023437500036,0.250000000000036,0.273948923410479,
0.297787299536743,0.312500000000037,0.336691512690665,0.343750000000037,
0.359375000000037,0.367187500000037,0.371093750000037,0.373046875000037,
0.374023437500037,0.375000000000037,0.402438386449995,0.437500000000038,
0.468750000000039,0.484375000000039,0.492187500000039,0.496093750000039,
0.498046875000039,0.499023437500039,0.499511718750039,0.500000000000039,
0.531454858450231,0.563785493779374,0.598875571442389,0.625000000000031,
0.661168477061904,0.687500000000027,0.712237630428612,0.718750000000025,
0.734375000000024,0.742187500000023,0.746093750000023,0.748046875000023,
0.749023437500023,0.750000000000023,0.79575267113575,0.84060489234686,0.884625373990666,
0.928360534765868,0.971893735048001,1.),.UNSPECIFIED.);
#328=B_SPLINE_CURVE_WITH_KNOTS('',3,(#59762,#59763,#59764,#59765,#59766,
#59767,#59768,#59769,#59770,#59771,#59772,#59773,#59774,#59775,#59776,#59777,
#59778,#59779,#59780,#59781,#59782,#59783,#59784,#59785,#59786,#59787,#59788,
#59789,#59790,#59791,#59792,#59793,#59794,#59795,#59796,#59797,#59798,#59799,
#59800,#59801,#59802,#59803,#59804,#59805,#59806,#59807,#59808,#59809,#59810,
#59811,#59812,#59813,#59814,#59815,#59816,#59817,#59818,#59819,#59820,#59821,
#59822,#59823,#59824,#59825,#59826,#59827,#59828,#59829,#59830,#59831,#59832,
#59833,#59834,#59835,#59836,#59837,#59838,#59839,#59840,#59841,#59842,#59843,
#59844,#59845,#59846,#59847,#59848,#59849,#59850,#59851,#59852,#59853,#59854,
#59855,#59856,#59857,#59858,#59859,#59860,#59861,#59862,#59863,#59864,#59865,
#59866,#59867,#59868,#59869,#59870,#59871,#59872,#59873,#59874,#59875,#59876,
#59877,#59878,#59879,#59880,#59881,#59882,#59883,#59884,#59885,#59886,#59887,
#59888,#59889,#59890,#59891,#59892,#59893,#59894,#59895,#59896,#59897,#59898,
#59899,#59900,#59901,#59902,#59903,#59904,#59905,#59906,#59907,#59908,#59909,
#59910,#59911,#59912,#59913,#59914,#59915,#59916,#59917,#59918),
 .UNSPECIFIED.,.F.,.F.,(4,3,3,3,3,3,3,3,3,3,3,3,3,3,3,3,3,3,3,3,3,3,3,3,
3,3,3,3,3,3,3,3,3,3,3,3,3,3,3,3,3,3,3,3,3,3,3,3,3,3,3,3,4),(1.72726524224126E-7,
0.0434573043788212,0.0863338267586707,0.0932171693142727,0.124999999999993,
0.165840000814769,0.177273799940387,0.187499999999989,0.218749999999987,
0.234374999999986,0.242187499999986,0.246093749999986,0.249511718749986,
0.249999999999986,0.260114116099238,0.284905555310815,0.309602658376984,
0.312499999999988,0.33693232554173,0.343749999999989,0.35937499999999,0.359741581816558,
0.36718749999999,0.37109374999999,0.373046874999991,0.374023437499991,0.374999999999991,
0.4271620062675,0.437499999999993,0.446538820825428,0.468749999999994,0.484374999999994,
0.492187499999994,0.499058232171587,0.499999999999994,0.529371777930485,
0.59548810882445,0.601623732066306,0.624999999999998,0.666785566987401,
0.6875,0.718750000000001,0.726753344238875,0.734375000000002,0.746093750000002,
0.750000000000002,0.777563968254758,0.821929376370596,0.864143232885838,
0.906140596325827,0.949725635816364,0.995918047404073,0.999999956001043),
 .UNSPECIFIED.);
#329=B_SPLINE_CURVE_WITH_KNOTS('',3,(#59960,#59961,#59962,#59963,#59964,
#59965,#59966,#59967,#59968,#59969,#59970,#59971,#59972,#59973,#59974,#59975,
#59976,#59977,#59978,#59979,#59980,#59981,#59982,#59983,#59984,#59985,#59986,
#59987,#59988,#59989,#59990),.UNSPECIFIED.,.F.,.F.,(4,3,3,3,3,3,3,3,3,3,
4),(0.,0.125000000000012,0.187500000000019,0.21875000000002,0.234375000000022,
0.242187500000021,0.25000000000002,0.375000000000017,0.500000000000013,
0.750000000000007,1.),.UNSPECIFIED.);
#330=B_SPLINE_CURVE_WITH_KNOTS('',3,(#59992,#59993,#59994,#59995,#59996,
#59997,#59998,#59999,#60000,#60001,#60002,#60003,#60004,#60005,#60006,#60007,
#60008,#60009,#60010,#60011,#60012,#60013),.UNSPECIFIED.,.F.,.F.,(4,3,3,
3,3,3,3,4),(6.12536510437413E-13,0.177079554736073,0.285234641299018,0.46505528483709,
0.5,0.685616239441862,0.871232478883723,0.999997383318307),
 .UNSPECIFIED.);
#331=B_SPLINE_CURVE_WITH_KNOTS('',3,(#60016,#60017,#60018,#60019,#60020,
#60021,#60022,#60023,#60024,#60025,#60026,#60027,#60028,#60029,#60030,#60031,
#60032,#60033,#60034,#60035,#60036,#60037,#60038,#60039,#60040,#60041,#60042,
#60043,#60044,#60045,#60046,#60047,#60048,#60049,#60050,#60051,#60052,#60053,
#60054,#60055,#60056,#60057,#60058,#60059,#60060,#60061,#60062,#60063,#60064,
#60065,#60066,#60067,#60068,#60069,#60070,#60071,#60072,#60073,#60074,#60075,
#60076),.UNSPECIFIED.,.F.,.F.,(4,3,3,3,3,3,3,3,3,3,3,3,3,3,3,3,3,3,3,3,
4),(3.08984601557555E-11,0.101977911095453,0.216247452367153,0.250000000000008,
0.304568311352161,0.375000000000011,0.437500000000014,0.468750000000016,
0.484375000000017,0.49416989406617,0.500000000000017,0.502028002520118,
0.58458238428531,0.662800125303651,0.723699269222825,0.750000000000009,
0.823969575829282,0.894343004279093,0.916583809267426,0.983994210266332,
0.999999999983593),.UNSPECIFIED.);
#332=B_SPLINE_CURVE_WITH_KNOTS('',3,(#60121,#60122,#60123,#60124,#60125,
#60126,#60127,#60128,#60129,#60130,#60131,#60132,#60133,#60134,#60135,#60136,
#60137,#60138,#60139,#60140,#60141,#60142,#60143,#60144,#60145,#60146,#60147,
#60148,#60149,#60150,#60151,#60152,#60153,#60154,#60155,#60156,#60157,#60158,
#60159,#60160,#60161,#60162,#60163,#60164,#60165,#60166,#60167,#60168,#60169,
#60170,#60171,#60172,#60173,#60174,#60175,#60176,#60177,#60178,#60179,#60180,
#60181,#60182,#60183,#60184,#60185,#60186,#60187,#60188,#60189,#60190),
 .UNSPECIFIED.,.F.,.F.,(4,3,3,3,3,3,3,3,3,3,3,3,3,3,3,3,3,3,3,3,3,3,3,4),
(0.,0.043555149686333,0.0764703251628506,0.120151057814094,0.125,0.178532566021585,
0.223906425134656,0.25,0.318743687382601,0.371576027078518,0.375,0.469091463337279,
0.5,0.519437204606587,0.625,0.667313790479252,0.741710622422343,0.75,0.808035613360659,
0.814958103135643,0.875,0.919742715260402,0.962451522902248,0.999999720292486),
 .UNSPECIFIED.);
#333=B_SPLINE_CURVE_WITH_KNOTS('',3,(#60191,#60192,#60193,#60194,#60195,
#60196,#60197,#60198,#60199,#60200,#60201,#60202,#60203,#60204,#60205,#60206,
#60207,#60208,#60209,#60210,#60211,#60212,#60213,#60214,#60215,#60216,#60217,
#60218,#60219,#60220,#60221,#60222,#60223,#60224,#60225,#60226,#60227,#60228,
#60229,#60230,#60231,#60232,#60233,#60234,#60235,#60236,#60237,#60238,#60239,
#60240,#60241,#60242,#60243,#60244,#60245,#60246,#60247,#60248,#60249,#60250,
#60251,#60252,#60253,#60254,#60255,#60256,#60257,#60258,#60259,#60260),
 .UNSPECIFIED.,.F.,.F.,(4,3,3,3,3,3,3,3,3,3,3,3,3,3,3,3,3,3,3,3,3,3,3,4),
(0.,0.0642450128226209,0.129222728498677,0.139648736860595,0.203363671729352,
0.250000000000001,0.300656432205033,0.369078216102518,0.437500000000002,
0.468750000000002,0.46971171597224,0.484375000000001,0.495154978438866,
0.500000000000001,0.563334744373279,0.625630806355903,0.644014764731035,
0.704246943422557,0.750000000000001,0.807879654393242,0.868482353955307,
0.928163350063891,0.961962300095513,0.999999992441419),.UNSPECIFIED.);
#334=B_SPLINE_CURVE_WITH_KNOTS('',3,(#60297,#60298,#60299,#60300,#60301,
#60302,#60303,#60304,#60305,#60306,#60307,#60308,#60309,#60310,#60311,#60312,
#60313,#60314,#60315,#60316,#60317,#60318,#60319,#60320,#60321,#60322,#60323,
#60324,#60325,#60326,#60327,#60328,#60329,#60330,#60331,#60332,#60333,#60334,
#60335,#60336,#60337,#60338,#60339,#60340,#60341,#60342,#60343,#60344,#60345,
#60346,#60347,#60348,#60349,#60350,#60351,#60352,#60353,#60354),
 .UNSPECIFIED.,.F.,.F.,(4,3,3,3,3,3,3,3,3,3,3,3,3,3,3,3,3,3,3,4),(6.60011716677258E-12,
0.0585629947700057,0.117996459937316,0.168707856042748,0.228541438031087,
0.25,0.3125,0.375000000000001,0.421054220391796,0.467108440783592,0.500000000000001,
0.563532899306448,0.626399529031098,0.688223245939294,0.75,0.771768815670398,
0.83260584940954,0.892881408073043,0.952306960013565,0.999999961863675),
 .UNSPECIFIED.);
#335=B_SPLINE_CURVE_WITH_KNOTS('',3,(#60355,#60356,#60357,#60358,#60359,
#60360,#60361,#60362,#60363,#60364,#60365,#60366,#60367,#60368,#60369,#60370,
#60371,#60372,#60373,#60374,#60375,#60376,#60377,#60378,#60379,#60380,#60381,
#60382,#60383,#60384,#60385,#60386,#60387,#60388,#60389,#60390,#60391,#60392,
#60393,#60394,#60395,#60396,#60397,#60398,#60399,#60400,#60401,#60402,#60403,
#60404,#60405,#60406,#60407,#60408,#60409,#60410,#60411,#60412),
 .UNSPECIFIED.,.F.,.F.,(4,3,3,3,3,3,3,3,3,3,3,3,3,3,3,3,3,3,3,4),(0.,0.0823874715591667,
0.156266197944322,0.223011563441643,0.25,0.307989093614892,0.364543396570697,
0.420407336747116,0.475427758760885,0.5,0.500020658777188,0.554932458503316,
0.610826173270344,0.667398897766358,0.725169989432572,0.75,0.817894591813742,
0.890404386237424,0.974097661819355,1.),.UNSPECIFIED.);
#336=B_SPLINE_CURVE_WITH_KNOTS('',3,(#60450,#60451,#60452,#60453,#60454,
#60455,#60456,#60457,#60458,#60459,#60460,#60461,#60462,#60463,#60464,#60465,
#60466,#60467,#60468,#60469,#60470,#60471,#60472,#60473,#60474,#60475,#60476,
#60477,#60478,#60479,#60480,#60481,#60482,#60483,#60484,#60485,#60486,#60487,
#60488,#60489,#60490,#60491,#60492,#60493,#60494,#60495,#60496,#60497,#60498,
#60499,#60500,#60501,#60502,#60503,#60504,#60505,#60506,#60507,#60508,#60509,
#60510,#60511,#60512,#60513,#60514,#60515,#60516,#60517,#60518,#60519,#60520,
#60521,#60522,#60523,#60524,#60525,#60526,#60527,#60528,#60529,#60530,#60531),
 .UNSPECIFIED.,.F.,.F.,(4,3,3,3,3,3,3,3,3,3,3,3,3,3,3,3,3,3,3,3,3,3,3,3,
3,3,3,4),(0.,0.075415314847338,0.125000000000002,0.138683869187328,0.187500000000003,
0.218750000000003,0.234375000000004,0.242187500000004,0.246093750000004,
0.250000000000004,0.321477738395407,0.389912144118573,0.457885661220333,
0.500000000000004,0.500062330010128,0.566092728183435,0.625000000000004,
0.678656853856775,0.687500000000004,0.718750000000004,0.734375000000004,
0.742187500000004,0.746093750000004,0.750000000000004,0.822132808280447,
0.861437880157647,0.936459487512057,0.999999999999982),.UNSPECIFIED.);
#337=B_SPLINE_CURVE_WITH_KNOTS('',3,(#60570,#60571,#60572,#60573,#60574,
#60575,#60576,#60577,#60578,#60579,#60580,#60581,#60582,#60583,#60584,#60585,
#60586,#60587,#60588,#60589,#60590,#60591),.UNSPECIFIED.,.F.,.F.,(4,3,3,
3,3,3,3,4),(4.23912252164219E-6,0.121979217178925,0.310989608589463,0.5,
0.679777216446932,0.707646284458543,0.884704706825873,0.99999999999933),
 .UNSPECIFIED.);
#338=B_SPLINE_CURVE_WITH_KNOTS('',3,(#60593,#60594,#60595,#60596,#60597,
#60598,#60599,#60600,#60601,#60602,#60603,#60604),.UNSPECIFIED.,.F.,.F.,
(4,2,2,2,2,4),(-0.133419885800988,-0.128305363731286,-0.107742733446663,
-0.0932105788792922,-0.0630589864485123,-1.03237217784953E-6),
 .UNSPECIFIED.);
#339=B_SPLINE_CURVE_WITH_KNOTS('',3,(#60605,#60606,#60607,#60608,#60609,
#60610,#60611,#60612,#60613,#60614,#60615,#60616,#60617,#60618,#60619,#60620,
#60621,#60622,#60623,#60624,#60625,#60626,#60627,#60628,#60629,#60630,#60631,
#60632,#60633,#60634,#60635,#60636,#60637,#60638,#60639,#60640,#60641,#60642,
#60643,#60644,#60645,#60646,#60647,#60648,#60649,#60650,#60651,#60652,#60653,
#60654,#60655,#60656,#60657,#60658,#60659,#60660,#60661,#60662),
 .UNSPECIFIED.,.F.,.F.,(4,3,3,3,3,3,3,3,3,3,3,3,3,3,3,3,3,3,3,4),(2.61381413586043E-6,
0.0670473710053725,0.0814149118918829,0.151202322002298,0.224512436629058,
0.24999999999998,0.273781868251335,0.350340974656353,0.430500053925807,
0.437499999999966,0.468749999999964,0.484374999999964,0.494602270260102,
0.495837805863796,0.499999999999964,0.607491325586912,0.693045153608403,
0.80555739922953,0.895474625281069,1.),.UNSPECIFIED.);
#340=B_SPLINE_CURVE_WITH_KNOTS('',3,(#60704,#60705,#60706,#60707,#60708,
#60709,#60710,#60711,#60712,#60713,#60714,#60715,#60716,#60717,#60718,#60719,
#60720,#60721,#60722,#60723,#60724,#60725,#60726,#60727,#60728,#60729,#60730,
#60731,#60732,#60733,#60734,#60735,#60736,#60737,#60738,#60739,#60740,#60741,
#60742,#60743,#60744,#60745,#60746,#60747,#60748,#60749,#60750,#60751,#60752,
#60753,#60754,#60755,#60756,#60757,#60758,#60759,#60760,#60761,#60762,#60763,
#60764,#60765,#60766,#60767,#60768,#60769,#60770,#60771,#60772,#60773,#60774,
#60775,#60776,#60777,#60778,#60779,#60780,#60781,#60782,#60783,#60784,#60785,
#60786,#60787,#60788,#60789,#60790,#60791),.UNSPECIFIED.,.F.,.F.,(4,3,3,
3,3,3,3,3,3,3,3,3,3,3,3,3,3,3,3,3,3,3,3,3,3,3,3,3,3,4),(3.50091154771304E-7,
0.0527824144532673,0.0818205493840706,0.138472328687778,0.195944420947396,
0.235749554746624,0.293011713332015,0.351192964442254,0.399875422218759,
0.437499999999992,0.468749999999991,0.484374999999991,0.49218749999999,
0.496093749999991,0.499508598803165,0.499999999999991,0.565860965729536,
0.629575211034318,0.693959315536848,0.725751294512647,0.781249999999995,
0.790730946026802,0.796874999999996,0.812499999999996,0.869044143359368,
0.874999999999997,0.884835921693697,0.938701676345939,0.993362228153319,
0.999999777713792),.UNSPECIFIED.);
#341=B_SPLINE_CURVE_WITH_KNOTS('',3,(#60865,#60866,#60867,#60868,#60869,
#60870,#60871,#60872,#60873,#60874,#60875,#60876,#60877,#60878,#60879,#60880,
#60881,#60882,#60883,#60884,#60885,#60886,#60887,#60888,#60889,#60890,#60891,
#60892,#60893,#60894,#60895,#60896,#60897,#60898,#60899,#60900,#60901,#60902,
#60903,#60904,#60905,#60906,#60907,#60908,#60909,#60910,#60911,#60912,#60913,
#60914,#60915,#60916,#60917,#60918,#60919,#60920,#60921,#60922,#60923,#60924,
#60925,#60926,#60927,#60928,#60929,#60930,#60931,#60932,#60933,#60934,#60935,
#60936,#60937,#60938,#60939,#60940,#60941,#60942,#60943,#60944,#60945,#60946,
#60947,#60948,#60949,#60950,#60951,#60952,#60953,#60954,#60955),
 .UNSPECIFIED.,.F.,.F.,(4,3,3,3,3,3,3,3,3,3,3,3,3,3,3,3,3,3,3,3,3,3,3,3,
3,3,3,3,3,3,4),(1.9887216213797E-7,0.0470902988611094,0.0950885656755635,
0.109526529164859,0.124999999999995,0.176685441702215,0.187499999999992,
0.195574874079998,0.203124999999992,0.218749999999991,0.249999999999991,
0.27062136400391,0.334103646587719,0.398264704624234,0.430414449322694,
0.437499999999987,0.468749999999987,0.484374999999987,0.492187499999987,
0.498034136225503,0.499999999999987,0.559924712613938,0.600124996010047,
0.658475318160386,0.715889407223646,0.764251057126962,0.821850440010763,
0.878616575074156,0.918179752465716,0.970963259453568,1.),.UNSPECIFIED.);
#342=B_SPLINE_CURVE_WITH_KNOTS('',3,(#60956,#60957,#60958,#60959,#60960,
#60961,#60962,#60963,#60964,#60965,#60966,#60967,#60968,#60969,#60970,#60971,
#60972,#60973,#60974,#60975,#60976,#60977,#60978,#60979,#60980,#60981,#60982,
#60983,#60984,#60985,#60986,#60987,#60988,#60989,#60990,#60991,#60992,#60993,
#60994,#60995,#60996,#60997,#60998,#60999,#61000,#61001,#61002,#61003,#61004,
#61005,#61006,#61007,#61008,#61009,#61010,#61011,#61012,#61013,#61014,#61015,
#61016,#61017,#61018,#61019),.UNSPECIFIED.,.F.,.F.,(4,3,3,3,3,3,3,3,3,3,
3,3,3,3,3,3,3,3,3,3,3,4),(0.,0.0259412938399118,0.127853460989982,0.228784505870627,
0.250000000000025,0.349135504880914,0.375000000000038,0.437500000000044,
0.468750000000048,0.48437500000005,0.492187500000051,0.498686700960381,
0.500000000000052,0.570456477027826,0.639131807094066,0.705384248701921,
0.750000000000026,0.812499999984393,0.870266491265459,0.926774908096166,
0.981742412633779,0.999999999937496),.UNSPECIFIED.);
#343=B_SPLINE_CURVE_WITH_KNOTS('',3,(#61057,#61058,#61059,#61060,#61061,
#61062,#61063,#61064,#61065,#61066,#61067,#61068,#61069,#61070,#61071,#61072,
#61073,#61074,#61075,#61076,#61077,#61078,#61079,#61080,#61081,#61082,#61083,
#61084,#61085,#61086,#61087),.UNSPECIFIED.,.F.,.F.,(4,3,3,3,3,3,3,3,3,3,
4),(0.,0.124999999999989,0.187499999999983,0.21874999999998,0.234374999999979,
0.242187499999979,0.249999999999979,0.374999999999983,0.499999999999987,
0.749999999999993,1.),.UNSPECIFIED.);
#344=B_SPLINE_CURVE_WITH_KNOTS('',3,(#61088,#61089,#61090,#61091,#61092,
#61093,#61094,#61095,#61096,#61097,#61098,#61099,#61100,#61101,#61102,#61103,
#61104,#61105,#61106,#61107,#61108,#61109,#61110,#61111,#61112),
 .UNSPECIFIED.,.F.,.F.,(4,3,3,3,3,3,3,3,4),(0.,0.167965175142067,0.230725444345264,
0.3333333333333,0.614592509477533,0.6666666666667,0.794930443258819,0.968172652596159,
0.999998645723269),.UNSPECIFIED.);
#345=B_SPLINE_CURVE_WITH_KNOTS('',3,(#61157,#61158,#61159,#61160,#61161,
#61162,#61163,#61164,#61165,#61166,#61167,#61168,#61169,#61170,#61171,#61172),
 .UNSPECIFIED.,.F.,.F.,(4,3,3,3,3,4),(0.,0.298197738937631,0.3333333333333,
0.6666666666667,0.972390787491876,0.999897516477361),.UNSPECIFIED.);
#346=B_SPLINE_CURVE_WITH_KNOTS('',3,(#61174,#61175,#61176,#61177,#61178,
#61179,#61180,#61181,#61182,#61183,#61184),.UNSPECIFIED.,.F.,.F.,(4,1,2,
2,2,4),(0.,0.124999999999994,0.218749999999991,0.24999999999999,0.499999999999994,
1.),.UNSPECIFIED.);
#347=B_SPLINE_CURVE_WITH_KNOTS('',3,(#61185,#61186,#61187,#61188,#61189,
#61190,#61191,#61192,#61193,#61194,#61195,#61196,#61197,#61198,#61199,#61200,
#61201,#61202,#61203,#61204,#61205,#61206,#61207,#61208,#61209,#61210,#61211,
#61212,#61213,#61214,#61215,#61216,#61217,#61218,#61219,#61220,#61221,#61222,
#61223,#61224,#61225,#61226,#61227,#61228,#61229,#61230,#61231,#61232,#61233,
#61234,#61235,#61236,#61237,#61238,#61239),.UNSPECIFIED.,.F.,.F.,(4,3,3,
3,3,3,3,3,3,3,3,3,3,3,3,3,3,3,4),(3.73125075129679E-10,0.0423471383370935,
0.110572976501087,0.182336544287981,0.210116916270959,0.249999999999991,
0.327328028218992,0.39972985545195,0.437499999999982,0.46874999999998,0.484374999999979,
0.494232017699017,0.499999999999978,0.591939017264748,0.696116117517602,
0.771382726348881,0.878464369045677,0.957256551971924,0.99995529208901),
 .UNSPECIFIED.);
#348=B_SPLINE_CURVE_WITH_KNOTS('',3,(#61285,#61286,#61287,#61288,#61289,
#61290,#61291,#61292,#61293,#61294,#61295,#61296,#61297,#61298,#61299,#61300,
#61301,#61302,#61303,#61304,#61305,#61306,#61307,#61308,#61309,#61310,#61311,
#61312,#61313,#61314,#61315,#61316,#61317,#61318,#61319,#61320,#61321,#61322,
#61323,#61324,#61325,#61326,#61327,#61328,#61329,#61330,#61331,#61332,#61333,
#61334,#61335,#61336,#61337,#61338,#61339,#61340,#61341,#61342,#61343,#61344,
#61345,#61346,#61347,#61348,#61349,#61350,#61351,#61352,#61353,#61354,#61355,
#61356,#61357),.UNSPECIFIED.,.F.,.F.,(4,3,3,3,3,3,3,3,3,3,3,3,3,3,3,3,3,
3,3,3,3,3,3,3,4),(1.45421596525061E-9,0.0431191253444328,0.0863267720282816,
0.129382358809736,0.1428571428571,0.153643952165499,0.204633581309079,0.255730997990358,
0.2857142857143,0.306393509483645,0.370923699621223,0.4285714285714,0.459412018039415,
0.526893093159749,0.5714285714286,0.612488429098831,0.677675308967365,0.7142857142857,
0.765391329883615,0.819870817141971,0.8571428571429,0.900979337073171,0.91813936937327,
0.961788839319927,0.999999999954867),.UNSPECIFIED.);
#349=B_SPLINE_CURVE_WITH_KNOTS('',3,(#61360,#61361,#61362,#61363,#61364,
#61365,#61366,#61367,#61368,#61369,#61370,#61371,#61372,#61373,#61374,#61375,
#61376,#61377,#61378,#61379,#61380,#61381,#61382,#61383,#61384,#61385,#61386,
#61387,#61388,#61389,#61390,#61391,#61392,#61393,#61394,#61395,#61396,#61397,
#61398,#61399,#61400,#61401,#61402,#61403,#61404,#61405,#61406,#61407,#61408,
#61409,#61410,#61411,#61412,#61413,#61414,#61415,#61416,#61417,#61418,#61419,
#61420,#61421,#61422,#61423,#61424,#61425,#61426,#61427,#61428,#61429,#61430,
#61431,#61432),.UNSPECIFIED.,.F.,.F.,(4,3,3,3,3,3,3,3,3,3,3,3,3,3,3,3,3,
3,3,3,3,3,3,3,4),(0.,0.0558892627811302,0.112669257545258,0.156953426523706,
0.215052236389246,0.25000000000002,0.309316256229949,0.324310867755753,
0.385391063272203,0.437500000000035,0.468750000000038,0.484375000000039,
0.492187500000039,0.498949324581199,0.500000000000039,0.504583614223561,
0.573408717889413,0.64134390510184,0.68014577642823,0.75000000000002,0.81592675256462,
0.847891248873937,0.914669189750963,0.980716833035571,1.),.UNSPECIFIED.);
#350=B_SPLINE_CURVE_WITH_KNOTS('',3,(#61531,#61532,#61533,#61534,#61535,
#61536,#61537,#61538,#61539,#61540,#61541,#61542,#61543,#61544,#61545,#61546,
#61547,#61548,#61549,#61550,#61551,#61552,#61553,#61554,#61555,#61556,#61557,
#61558,#61559,#61560,#61561,#61562,#61563,#61564,#61565,#61566,#61567,#61568,
#61569,#61570,#61571,#61572,#61573,#61574,#61575,#61576,#61577,#61578,#61579,
#61580,#61581,#61582,#61583,#61584,#61585,#61586,#61587,#61588,#61589,#61590,
#61591,#61592,#61593,#61594,#61595,#61596,#61597,#61598,#61599,#61600,#61601,
#61602,#61603,#61604,#61605,#61606,#61607,#61608,#61609,#61610,#61611,#61612,
#61613,#61614,#61615,#61616,#61617,#61618,#61619,#61620,#61621,#61622,#61623,
#61624,#61625,#61626,#61627,#61628,#61629,#61630,#61631,#61632,#61633,#61634,
#61635,#61636,#61637,#61638,#61639,#61640,#61641,#61642,#61643,#61644,#61645,
#61646,#61647,#61648,#61649,#61650,#61651,#61652,#61653,#61654,#61655,#61656,
#61657,#61658,#61659,#61660,#61661,#61662,#61663,#61664,#61665,#61666,#61667,
#61668,#61669,#61670,#61671,#61672,#61673,#61674,#61675,#61676,#61677,#61678,
#61679,#61680,#61681,#61682,#61683,#61684,#61685,#61686,#61687,#61688,#61689,
#61690,#61691,#61692,#61693,#61694,#61695,#61696),.UNSPECIFIED.,.F.,.F.,
(4,3,3,3,3,3,3,3,3,3,3,3,3,3,3,3,3,3,3,3,3,3,3,3,3,3,3,3,3,3,3,3,3,3,3,
3,3,3,3,3,3,3,3,3,3,3,3,3,3,3,3,3,3,3,3,4),(8.91470519372192E-8,0.0341843291030202,
0.0624999999999999,0.0799991073633813,0.0937499999999998,0.109375,0.1171875,
0.12109375,0.123046875,0.125,0.156854101554739,0.1875,0.21875,0.234375,
0.237493486952361,0.2421875,0.24609375,0.248046875,0.25,0.290848999557458,
0.312500000000001,0.328904221360791,0.343750000000002,0.359375000000002,
0.367187500000002,0.371093750000002,0.373046875000002,0.375000000000002,
0.425200709948369,0.437500000000002,0.468750000000002,0.484375000000002,
0.492187500000002,0.496093750000002,0.500000000000002,0.520161000661623,
0.57260995086379,0.616925907134883,0.625000000000001,0.651314116776,0.678193288479241,
0.687500000000001,0.709191597556237,0.750000000000001,0.781250000000001,
0.789062500000001,0.796875000000001,0.799101080805048,0.812500000000001,
0.858392460401059,0.875000000000001,0.885508810391372,0.932690672165831,
0.980791435666233,0.985732819345807,1.),.UNSPECIFIED.);
#351=B_SPLINE_CURVE_WITH_KNOTS('',3,(#61699,#61700,#61701,#61702,#61703,
#61704,#61705,#61706,#61707,#61708,#61709,#61710,#61711,#61712,#61713,#61714,
#61715,#61716,#61717,#61718,#61719,#61720,#61721,#61722,#61723,#61724,#61725,
#61726,#61727,#61728,#61729,#61730,#61731,#61732,#61733,#61734,#61735,#61736,
#61737,#61738,#61739,#61740,#61741,#61742,#61743,#61744,#61745,#61746,#61747,
#61748,#61749,#61750,#61751,#61752,#61753,#61754,#61755,#61756,#61757,#61758,
#61759,#61760,#61761,#61762,#61763,#61764,#61765,#61766,#61767,#61768,#61769,
#61770,#61771,#61772,#61773,#61774,#61775,#61776,#61777,#61778,#61779,#61780,
#61781,#61782,#61783,#61784,#61785,#61786,#61787,#61788,#61789,#61790,#61791,
#61792,#61793,#61794,#61795,#61796,#61797,#61798,#61799,#61800,#61801,#61802,
#61803,#61804,#61805,#61806,#61807,#61808,#61809,#61810,#61811,#61812,#61813,
#61814,#61815,#61816,#61817,#61818,#61819,#61820,#61821,#61822,#61823,#61824,
#61825,#61826,#61827,#61828,#61829,#61830,#61831,#61832,#61833,#61834,#61835,
#61836,#61837,#61838,#61839,#61840),.UNSPECIFIED.,.F.,.F.,(4,3,3,3,3,3,
3,3,3,3,3,3,3,3,3,3,3,3,3,3,3,3,3,3,3,3,3,3,3,3,3,3,3,3,3,3,3,3,3,3,3,3,
3,3,3,3,3,4),(2.34637985974789E-7,0.031595826091221,0.062896465800433,0.0937122471496095,
0.104172266518684,0.124999999999998,0.154837351378791,0.184674702757584,
0.213176019980234,0.218749999999996,0.234374999999996,0.242187499999996,
0.246093749999995,0.248046874999995,0.249999999999996,0.257790681019999,
0.295642689870312,0.334483658793269,0.354334778645037,0.39268306807659,
0.431398782256473,0.470481835057029,0.48237572788559,0.484374999999997,
0.496585735733692,0.499999999999997,0.540377615423201,0.580372331065526,
0.609453985246043,0.649164804655767,0.687499999999999,0.700831465154267,
0.718749999999999,0.734374999999999,0.742187499999999,0.746093749999999,
0.748046874999999,0.749999999999999,0.769091486017791,0.798966759489123,
0.828842032960455,0.858576939735652,0.874999999999999,0.896782274077063,
0.927914209698524,0.959582410600718,0.985641670858647,1.),.UNSPECIFIED.);
#352=B_SPLINE_CURVE_WITH_KNOTS('',3,(#61877,#61878,#61879,#61880,#61881,
#61882,#61883,#61884,#61885,#61886,#61887,#61888,#61889,#61890,#61891,#61892,
#61893,#61894,#61895,#61896,#61897,#61898,#61899,#61900,#61901,#61902,#61903,
#61904,#61905,#61906,#61907,#61908,#61909,#61910,#61911,#61912,#61913,#61914,
#61915,#61916,#61917,#61918,#61919,#61920,#61921,#61922,#61923,#61924,#61925,
#61926,#61927,#61928,#61929,#61930,#61931,#61932,#61933,#61934,#61935,#61936,
#61937),.UNSPECIFIED.,.F.,.F.,(4,3,3,3,3,3,3,3,3,3,3,3,3,3,3,3,3,3,3,3,
4),(3.81436972404066E-8,0.0594692341193173,0.119461353288053,0.180335257934325,
0.228233369909761,0.250000000000001,0.312500000000001,0.375000000000001,
0.420630665240657,0.466482701433567,0.5,0.532982727135479,0.595584458307783,
0.657507423778217,0.718468767547966,0.75,0.80983093432658,0.831293916785482,
0.890887278795621,0.949594741146851,1.),.UNSPECIFIED.);
#353=B_SPLINE_CURVE_WITH_KNOTS('',3,(#61938,#61939,#61940,#61941,#61942,
#61943,#61944,#61945,#61946,#61947,#61948,#61949,#61950,#61951,#61952,#61953,
#61954,#61955,#61956,#61957,#61958,#61959,#61960,#61961,#61962,#61963,#61964,
#61965,#61966,#61967,#61968,#61969,#61970,#61971,#61972,#61973,#61974,#61975,
#61976,#61977,#61978,#61979,#61980,#61981,#61982,#61983,#61984,#61985,#61986,
#61987,#61988,#61989,#61990,#61991,#61992,#61993,#61994,#61995),
 .UNSPECIFIED.,.F.,.F.,(4,3,3,3,3,3,3,3,3,3,3,3,3,3,3,3,3,3,3,4),(0.,0.0706357924192512,
0.136905894358846,0.198469767880529,0.25,0.307239195840158,0.363641873526663,
0.419667860479303,0.475290932764254,0.49995510889698,0.5,0.555615247434432,
0.61170547306681,0.668168214199068,0.725338437553129,0.75,0.8125,0.877100936211395,
0.947886389184427,1.),.UNSPECIFIED.);
#354=B_SPLINE_CURVE_WITH_KNOTS('',3,(#62038,#62039,#62040,#62041,#62042,
#62043,#62044,#62045,#62046,#62047,#62048,#62049,#62050,#62051,#62052,#62053,
#62054,#62055,#62056,#62057,#62058,#62059,#62060,#62061,#62062,#62063,#62064,
#62065,#62066,#62067,#62068,#62069,#62070,#62071,#62072,#62073,#62074,#62075,
#62076,#62077,#62078,#62079,#62080,#62081,#62082,#62083,#62084,#62085,#62086,
#62087,#62088,#62089,#62090,#62091,#62092,#62093,#62094,#62095,#62096,#62097,
#62098,#62099,#62100,#62101,#62102,#62103,#62104,#62105,#62106,#62107,#62108,
#62109,#62110,#62111,#62112,#62113,#62114,#62115,#62116,#62117,#62118,#62119,
#62120,#62121,#62122),.UNSPECIFIED.,.F.,.F.,(4,3,3,3,3,3,3,3,3,3,3,3,3,
3,3,3,3,3,3,3,3,3,3,3,3,3,3,3,4),(0.,0.070984038243982,0.124999999999996,
0.187499999999995,0.218749999999994,0.234374999999994,0.242187499999994,
0.244541813992091,0.246093749999993,0.249999999999993,0.318695715793694,
0.386222190629079,0.414616854789881,0.482181913540056,0.499999999999994,
0.565353689470601,0.585548104938381,0.624999999999995,0.687499999999995,
0.718749999999995,0.734374999999995,0.742187499999995,0.746093749999995,
0.749999999999995,0.755626562870562,0.823511777763023,0.893068528416106,
0.929166670310745,1.),.UNSPECIFIED.);
#355=B_SPLINE_CURVE_WITH_KNOTS('',3,(#62165,#62166,#62167,#62168,#62169,
#62170,#62171,#62172,#62173,#62174,#62175,#62176,#62177,#62178,#62179,#62180,
#62181,#62182,#62183,#62184,#62185,#62186,#62187,#62188,#62189,#62190,#62191,
#62192,#62193,#62194,#62195),.UNSPECIFIED.,.F.,.F.,(4,3,3,3,3,3,3,3,3,3,
4),(0.,0.125000000000036,0.187500000000053,0.21875000000006,0.234375000000062,
0.242187500000063,0.250000000000064,0.375000000000053,0.500000000000043,
0.750000000000021,1.),.UNSPECIFIED.);
#356=B_SPLINE_CURVE_WITH_KNOTS('',3,(#62196,#62197,#62198,#62199,#62200,
#62201,#62202,#62203,#62204,#62205,#62206,#62207,#62208,#62209,#62210,#62211),
 .UNSPECIFIED.,.F.,.F.,(4,3,3,3,3,4),(0.,0.305738962927125,0.3333333333333,
0.6666666666667,0.964886280950195,1.),.UNSPECIFIED.);
#357=B_SPLINE_CURVE_WITH_KNOTS('',3,(#62212,#62213,#62214,#62215,#62216,
#62217,#62218,#62219,#62220,#62221,#62222,#62223,#62224,#62225,#62226,#62227,
#62228,#62229,#62230,#62231,#62232,#62233,#62234,#62235,#62236,#62237,#62238,
#62239,#62240,#62241,#62242,#62243,#62244,#62245,#62246,#62247,#62248,#62249,
#62250,#62251,#62252,#62253,#62254,#62255,#62256,#62257,#62258,#62259,#62260,
#62261,#62262,#62263,#62264,#62265,#62266,#62267,#62268,#62269,#62270,#62271,
#62272,#62273,#62274,#62275),.UNSPECIFIED.,.F.,.F.,(4,3,3,3,3,3,3,3,3,3,
3,3,3,3,3,3,3,3,3,3,3,4),(0.,0.0446614606293701,0.151711825344438,0.230164819186069,
0.25,0.354548286934243,0.375000000000001,0.409260647438796,0.437500000000001,
0.46875,0.484375,0.493953369682669,0.500000000000001,0.580864109044975,
0.601341896293497,0.678602986469359,0.75,0.790540546335742,0.862585242307717,
0.931006462747741,0.957944183693305,1.),.UNSPECIFIED.);
#358=B_SPLINE_CURVE_WITH_KNOTS('',3,(#62318,#62319,#62320,#62321,#62322,
#62323,#62324,#62325,#62326,#62327,#62328,#62329,#62330,#62331,#62332,#62333,
#62334,#62335,#62336,#62337,#62338,#62339,#62340,#62341,#62342,#62343,#62344,
#62345,#62346,#62347,#62348,#62349,#62350,#62351,#62352,#62353,#62354,#62355,
#62356,#62357,#62358,#62359,#62360,#62361,#62362,#62363,#62364,#62365,#62366,
#62367,#62368,#62369,#62370,#62371,#62372,#62373,#62374,#62375,#62376,#62377,
#62378,#62379,#62380,#62381,#62382,#62383,#62384,#62385,#62386,#62387,#62388,
#62389,#62390,#62391,#62392,#62393,#62394,#62395,#62396,#62397,#62398,#62399,
#62400,#62401,#62402,#62403,#62404,#62405,#62406,#62407,#62408),
 .UNSPECIFIED.,.F.,.F.,(4,3,3,3,3,3,3,3,3,3,3,3,3,3,3,3,3,3,3,3,3,3,3,3,
3,3,3,3,3,3,4),(1.98906486742311E-7,0.0470898534984864,0.0950876880993247,
0.10952642980478,0.125000000000006,0.17668496847957,0.18750000000001,0.195574841561927,
0.20312500000001,0.21875000000001,0.250000000000011,0.270621656389179,0.334104136527559,
0.398265387134923,0.430414690770554,0.437500000000015,0.468750000000015,
0.484375000000015,0.492187500000015,0.498034130470392,0.500000000000015,
0.559924746618581,0.600124931584257,0.658475281491341,0.715889390715269,
0.7642505253901,0.821849983871512,0.878616196067142,0.918178937043819,0.970962456769612,
1.),.UNSPECIFIED.);
#359=B_SPLINE_CURVE_WITH_KNOTS('',3,(#62453,#62454,#62455,#62456,#62457,
#62458,#62459,#62460,#62461,#62462,#62463,#62464,#62465,#62466,#62467,#62468,
#62469,#62470,#62471,#62472,#62473,#62474,#62475,#62476,#62477,#62478,#62479,
#62480,#62481,#62482,#62483,#62484,#62485,#62486,#62487,#62488,#62489,#62490,
#62491,#62492,#62493,#62494,#62495,#62496,#62497,#62498,#62499,#62500,#62501,
#62502,#62503,#62504,#62505,#62506,#62507,#62508,#62509,#62510),
 .UNSPECIFIED.,.F.,.F.,(4,3,3,3,3,3,3,3,3,3,3,3,3,3,3,3,3,3,3,4),(0.,0.0625,
0.123433376418121,0.183427620822819,0.242367644898908,0.25,0.308040515079698,
0.365337471650276,0.42229797384171,0.479065208678401,0.535781347576013,
0.592773854696921,0.649986866374424,0.707857241876389,0.75,0.808902570121928,
0.869152639395624,0.930295239220506,0.992904488662291,1.),.UNSPECIFIED.);
#360=B_SPLINE_CURVE_WITH_KNOTS('',3,(#62512,#62513,#62514,#62515,#62516,
#62517,#62518,#62519,#62520,#62521,#62522,#62523,#62524,#62525,#62526,#62527),
 .UNSPECIFIED.,.F.,.F.,(4,3,3,3,3,4),(0.,0.298778860875572,0.3333333333333,
0.6666666666667,0.972465952980625,1.),.UNSPECIFIED.);
#361=B_SPLINE_CURVE_WITH_KNOTS('',3,(#62529,#62530,#62531,#62532,#62533,
#62534,#62535,#62536,#62537,#62538,#62539),.UNSPECIFIED.,.F.,.F.,(4,1,2,
2,2,4),(0.,0.125000000000002,0.218750000000005,0.250000000000005,0.500000000000003,
1.),.UNSPECIFIED.);
#362=B_SPLINE_CURVE_WITH_KNOTS('',3,(#62540,#62541,#62542,#62543,#62544,
#62545,#62546,#62547,#62548,#62549,#62550,#62551,#62552,#62553,#62554,#62555,
#62556,#62557,#62558,#62559,#62560,#62561,#62562,#62563,#62564,#62565,#62566,
#62567,#62568,#62569,#62570,#62571,#62572,#62573,#62574,#62575,#62576,#62577,
#62578,#62579,#62580,#62581,#62582,#62583,#62584,#62585,#62586,#62587,#62588,
#62589,#62590,#62591,#62592,#62593,#62594,#62595,#62596,#62597),
 .UNSPECIFIED.,.F.,.F.,(4,3,3,3,3,3,3,3,3,3,3,3,3,3,3,3,3,3,3,4),(6.11814853262804E-10,
0.0417521477615177,0.109880939803693,0.181543350593602,0.209151847901313,
0.250000000000004,0.32674556824041,0.375000000000005,0.39835952915245,0.437500000000006,
0.468750000000008,0.484375000000009,0.494227622931881,0.500000000000011,
0.590539736464595,0.694718942696452,0.769679430141417,0.876793017787304,
0.95521013021045,0.99999999997903),.UNSPECIFIED.);
#363=B_SPLINE_CURVE_WITH_KNOTS('',3,(#62639,#62640,#62641,#62642,#62643,
#62644,#62645,#62646,#62647,#62648,#62649,#62650,#62651,#62652,#62653,#62654,
#62655,#62656,#62657,#62658,#62659,#62660,#62661,#62662,#62663,#62664,#62665,
#62666,#62667,#62668,#62669,#62670,#62671,#62672,#62673,#62674,#62675,#62676,
#62677,#62678,#62679,#62680,#62681,#62682,#62683,#62684,#62685,#62686,#62687,
#62688,#62689,#62690,#62691,#62692,#62693,#62694,#62695,#62696,#62697,#62698,
#62699,#62700,#62701,#62702,#62703,#62704,#62705,#62706,#62707,#62708,#62709,
#62710,#62711,#62712,#62713,#62714,#62715,#62716,#62717,#62718,#62719,#62720,
#62721,#62722,#62723,#62724,#62725,#62726),.UNSPECIFIED.,.F.,.F.,(4,3,3,
3,3,3,3,3,3,3,3,3,3,3,3,3,3,3,3,3,3,3,3,3,3,3,3,3,3,4),(3.70263034175187E-11,
0.0527820564885111,0.081821354966552,0.138473187136047,0.195945331196402,
0.235750067891708,0.29301224024971,0.351193499636413,0.399875474066281,
0.437499999999966,0.468749999999963,0.484374999999962,0.492187499999962,
0.496093749999963,0.499508596624892,0.499999999999963,0.565860737136916,
0.629574800820601,0.69395872836067,0.725750995729374,0.781249999999981,
0.790730859889013,0.796874999999982,0.812499999999984,0.869043375183258,
0.874999999999989,0.884835790315371,0.938700861559312,0.993360752892644,
0.99999977775045),.UNSPECIFIED.);
#364=B_SPLINE_CURVE_WITH_KNOTS('',3,(#62729,#62730,#62731,#62732,#62733,
#62734,#62735,#62736,#62737,#62738,#62739,#62740,#62741,#62742,#62743,#62744,
#62745,#62746,#62747,#62748,#62749,#62750,#62751,#62752,#62753,#62754,#62755,
#62756,#62757,#62758,#62759,#62760,#62761,#62762,#62763,#62764,#62765,#62766,
#62767,#62768,#62769,#62770,#62771,#62772,#62773,#62774,#62775,#62776,#62777,
#62778,#62779,#62780,#62781,#62782,#62783,#62784,#62785,#62786),
 .UNSPECIFIED.,.F.,.F.,(4,3,3,3,3,3,3,3,3,3,3,3,3,3,3,3,3,3,3,4),(0.,0.0585633378234075,
0.117996984449599,0.168707880043306,0.228541703309256,0.250000000000001,
0.312500000000001,0.375000000000001,0.421054217354142,0.467108434708283,
0.500000000000001,0.563532905575853,0.626399541702303,0.688223265291581,
0.750000000000001,0.771768807379113,0.83260584823571,0.892881414097024,
0.952306973405338,0.999999961863691),.UNSPECIFIED.);
#365=B_SPLINE_CURVE_WITH_KNOTS('',3,(#62837,#62838,#62839,#62840,#62841,
#62842,#62843,#62844,#62845,#62846,#62847,#62848,#62849,#62850,#62851,#62852,
#62853,#62854,#62855,#62856,#62857,#62858,#62859,#62860,#62861,#62862,#62863,
#62864,#62865,#62866,#62867,#62868,#62869,#62870,#62871,#62872,#62873,#62874,
#62875,#62876,#62877,#62878,#62879,#62880,#62881,#62882,#62883,#62884,#62885,
#62886,#62887,#62888,#62889,#62890,#62891,#62892,#62893,#62894,#62895,#62896,
#62897,#62898,#62899,#62900,#62901,#62902,#62903,#62904,#62905,#62906,#62907,
#62908,#62909,#62910,#62911,#62912,#62913,#62914,#62915,#62916,#62917,#62918,
#62919,#62920,#62921,#62922,#62923,#62924,#62925,#62926,#62927,#62928,#62929,
#62930,#62931,#62932,#62933,#62934,#62935,#62936,#62937,#62938,#62939,#62940,
#62941,#62942,#62943,#62944,#62945,#62946,#62947,#62948,#62949,#62950,#62951,
#62952,#62953,#62954,#62955,#62956,#62957,#62958,#62959,#62960,#62961,#62962,
#62963,#62964,#62965,#62966,#62967,#62968,#62969,#62970,#62971,#62972,#62973,
#62974,#62975,#62976,#62977,#62978,#62979,#62980,#62981,#62982,#62983,#62984,
#62985,#62986,#62987,#62988,#62989,#62990,#62991,#62992,#62993,#62994,#62995,
#62996,#62997,#62998,#62999,#63000,#63001,#63002,#63003,#63004,#63005,#63006,
#63007,#63008,#63009,#63010,#63011,#63012,#63013,#63014,#63015,#63016,#63017,
#63018,#63019,#63020,#63021,#63022,#63023,#63024,#63025,#63026,#63027,#63028,
#63029,#63030,#63031,#63032,#63033,#63034,#63035,#63036,#63037,#63038,#63039,
#63040,#63041,#63042,#63043,#63044,#63045,#63046,#63047,#63048,#63049,#63050,
#63051,#63052,#63053,#63054,#63055,#63056,#63057,#63058,#63059,#63060,#63061,
#63062,#63063,#63064,#63065,#63066,#63067,#63068,#63069,#63070,#63071,#63072,
#63073,#63074,#63075,#63076,#63077,#63078,#63079,#63080),.UNSPECIFIED.,
 .F.,.F.,(4,3,3,3,3,3,3,3,3,3,3,3,3,3,3,3,3,3,3,3,3,3,3,3,3,3,3,3,3,3,3,
3,3,3,3,3,3,3,3,3,3,3,3,3,3,3,3,3,3,3,3,3,3,3,3,3,3,3,3,3,3,3,3,3,3,3,3,
3,3,3,3,3,3,3,3,3,3,3,3,3,3,4),(9.73806164256783E-8,0.0159281142913431,
0.0312500000000213,0.046875000000032,0.0546875000000373,0.0585937500000399,
0.0625000000000424,0.0648418039613322,0.0836785664054461,0.102452808361369,
0.109375000000073,0.117187500000078,0.121093750000081,0.123046875000082,
0.124023437500082,0.124511718750083,0.125000000000083,0.130859030271114,
0.14559909038106,0.160253323380513,0.17187500000009,0.179687500000091,0.183593750000092,
0.185546875000092,0.186523437500093,0.187500000000093,0.198325694518741,
0.209109868210274,0.213418238445796,0.224168357782371,0.234847785721346,
0.242187500000105,0.246093750000106,0.248046875000107,0.249023437500107,
0.249755859375107,0.250000000000107,0.286107610092526,0.331138076209162,
0.373109057199251,0.413997211211172,0.437500000000133,0.442041901806469,
0.468750000000137,0.484375000000139,0.49218750000014,0.496093750000141,
0.498046875000141,0.498820943136186,0.499023437500141,0.499511718750141,
0.500000000000141,0.527811010006352,0.555639881747458,0.580242634713494,
0.608313865295241,0.634725967382553,0.640625000000156,0.645735141626808,
0.648437500000157,0.665748936028716,0.677911470409284,0.695416726989991,
0.713007949879031,0.730688053588786,0.734375000000167,0.742187500000168,
0.746093750000168,0.748046875000168,0.749023437500168,0.749511718750168,
0.750000000000167,0.752509339484753,0.797992313705749,0.804152672765917,
0.850548065526046,0.858799535654424,0.906291712294993,0.920210727170671,
0.968985942526481,0.993036925597939,1.),.UNSPECIFIED.);
#366=B_SPLINE_CURVE_WITH_KNOTS('',3,(#63163,#63164,#63165,#63166,#63167,
#63168,#63169,#63170,#63171,#63172,#63173,#63174,#63175,#63176,#63177,#63178,
#63179,#63180,#63181,#63182,#63183,#63184,#63185,#63186,#63187,#63188,#63189,
#63190,#63191,#63192,#63193,#63194,#63195,#63196,#63197,#63198,#63199,#63200,
#63201,#63202,#63203,#63204,#63205,#63206,#63207,#63208,#63209,#63210,#63211,
#63212,#63213,#63214,#63215,#63216,#63217,#63218,#63219,#63220,#63221,#63222,
#63223,#63224,#63225,#63226,#63227,#63228,#63229,#63230,#63231,#63232,#63233,
#63234,#63235,#63236,#63237,#63238,#63239,#63240,#63241,#63242,#63243,#63244,
#63245,#63246,#63247,#63248,#63249,#63250,#63251,#63252,#63253,#63254,#63255,
#63256,#63257,#63258,#63259,#63260,#63261,#63262,#63263,#63264,#63265,#63266,
#63267,#63268,#63269,#63270,#63271,#63272,#63273,#63274,#63275,#63276,#63277,
#63278,#63279,#63280,#63281,#63282,#63283,#63284,#63285,#63286,#63287,#63288,
#63289,#63290,#63291,#63292,#63293,#63294,#63295,#63296,#63297,#63298,#63299,
#63300,#63301,#63302,#63303,#63304,#63305,#63306,#63307,#63308,#63309,#63310,
#63311,#63312,#63313,#63314,#63315,#63316,#63317,#63318,#63319),
 .UNSPECIFIED.,.F.,.F.,(4,3,3,3,3,3,3,3,3,3,3,3,3,3,3,3,3,3,3,3,3,3,3,3,
3,3,3,3,3,3,3,3,3,3,3,3,3,3,3,3,3,3,3,3,3,3,3,3,3,3,3,3,4),(1.72726438405786E-7,
0.0434573164719052,0.086333854898234,0.0932163022794985,0.124999999999983,
0.165840014184437,0.177272634924799,0.187499999999974,0.218749999999969,
0.234374999999967,0.242187499999966,0.246093749999966,0.249511718749965,
0.249999999999965,0.260112422138339,0.284903851802453,0.309600945382747,
0.312499999999968,0.336932311116222,0.343749999999969,0.359374999999969,
0.35974136967626,0.36718749999997,0.37109374999997,0.37304687499997,0.37402343749997,
0.37499999999997,0.42716199723274,0.437499999999972,0.446539738539256,0.468749999999974,
0.484374999999974,0.492187499999975,0.499058231412271,0.499999999999975,
0.529373583917037,0.595489913988851,0.601626215812586,0.62499999999998,
0.666788584072113,0.687499999999983,0.718749999999984,0.726756725922575,
0.734374999999985,0.746093749999985,0.749999999999985,0.777566925552718,
0.821932091724188,0.864145581838811,0.906142545834475,0.94972718006945,
0.995919147870662,0.999999956000501),.UNSPECIFIED.);
#367=B_SPLINE_CURVE_WITH_KNOTS('',3,(#63364,#63365,#63366,#63367,#63368,
#63369,#63370,#63371,#63372,#63373,#63374,#63375,#63376,#63377,#63378,#63379,
#63380,#63381,#63382,#63383,#63384,#63385,#63386,#63387,#63388,#63389,#63390,
#63391,#63392,#63393,#63394),.UNSPECIFIED.,.F.,.F.,(4,3,3,3,3,3,3,3,3,3,
4),(0.,0.125,0.187500000000001,0.218750000000001,0.234375000000002,0.242187500000001,
0.25,0.375,0.500000000000001,0.75,1.),.UNSPECIFIED.);
#368=B_SPLINE_CURVE_WITH_KNOTS('',3,(#63396,#63397,#63398,#63399,#63400,
#63401,#63402,#63403,#63404,#63405,#63406,#63407,#63408,#63409,#63410,#63411),
 .UNSPECIFIED.,.F.,.F.,(4,3,3,3,3,4),(0.000149798704371109,0.305896512638586,
0.3333333333333,0.6666666666667,0.965406965005641,1.),.UNSPECIFIED.);
#369=B_SPLINE_CURVE_WITH_KNOTS('',3,(#63414,#63415,#63416,#63417,#63418,
#63419,#63420,#63421,#63422,#63423,#63424,#63425,#63426,#63427,#63428,#63429,
#63430,#63431,#63432,#63433,#63434,#63435,#63436,#63437,#63438,#63439,#63440,
#63441,#63442,#63443,#63444,#63445,#63446,#63447,#63448,#63449,#63450,#63451,
#63452,#63453,#63454,#63455,#63456,#63457,#63458,#63459,#63460,#63461,#63462,
#63463,#63464,#63465,#63466,#63467,#63468,#63469,#63470,#63471,#63472,#63473,
#63474),.UNSPECIFIED.,.F.,.F.,(4,3,3,3,3,3,3,3,3,3,3,3,3,3,3,3,3,3,3,3,
4),(3.35491904938007E-5,0.0428738058325973,0.149949773961846,0.228787916593128,
0.249999999999993,0.353669955295993,0.408269673424094,0.437499999999988,
0.468749999999987,0.484374999999986,0.493967232192623,0.499999999999985,
0.580997102510811,0.600490344305326,0.677895850195905,0.749999999999992,
0.790086401711803,0.862285218947932,0.930853411259674,0.957922464653335,
1.),.UNSPECIFIED.);
#370=B_SPLINE_CURVE_WITH_KNOTS('',3,(#63519,#63520,#63521,#63522,#63523,
#63524,#63525,#63526,#63527,#63528,#63529,#63530,#63531,#63532,#63533,#63534,
#63535,#63536,#63537,#63538,#63539,#63540,#63541,#63542,#63543,#63544,#63545,
#63546,#63547,#63548,#63549,#63550,#63551,#63552,#63553,#63554,#63555,#63556,
#63557,#63558,#63559,#63560,#63561,#63562,#63563,#63564,#63565,#63566,#63567,
#63568,#63569,#63570,#63571,#63572,#63573,#63574,#63575,#63576,#63577,#63578,
#63579,#63580,#63581,#63582,#63583,#63584,#63585,#63586,#63587,#63588),
 .UNSPECIFIED.,.F.,.F.,(4,3,3,3,3,3,3,3,3,3,3,3,3,3,3,3,3,3,3,3,3,3,3,4),
(0.,0.0436825089787147,0.0764111191074181,0.120245150899802,0.125,0.179962620954868,
0.223835356148353,0.25,0.320059899745086,0.371520369824615,0.375,0.470560242042003,
0.5,0.519394870001365,0.625,0.667284556518977,0.74166723255934,0.75,0.808039637084786,
0.814941565949557,0.875,0.919746518923496,0.962447676465487,0.999999720259695),
 .UNSPECIFIED.);
#371=B_SPLINE_CURVE_WITH_KNOTS('',3,(#63589,#63590,#63591,#63592,#63593,
#63594,#63595,#63596,#63597,#63598,#63599,#63600,#63601,#63602,#63603,#63604,
#63605,#63606,#63607,#63608,#63609,#63610,#63611,#63612,#63613,#63614,#63615,
#63616,#63617,#63618,#63619,#63620,#63621,#63622,#63623,#63624,#63625,#63626,
#63627,#63628,#63629,#63630,#63631,#63632,#63633,#63634,#63635,#63636,#63637,
#63638,#63639,#63640,#63641,#63642,#63643,#63644,#63645,#63646,#63647,#63648,
#63649,#63650,#63651,#63652,#63653,#63654,#63655,#63656,#63657,#63658),
 .UNSPECIFIED.,.F.,.F.,(4,3,3,3,3,3,3,3,3,3,3,3,3,3,3,3,3,3,3,3,3,3,3,4),
(0.,0.0642455417156636,0.12922356065871,0.13964895033816,0.203364207353361,
0.250000000000001,0.300656467909375,0.369078233954689,0.437500000000003,
0.468750000000003,0.469711899594866,0.484375000000003,0.495154873957857,
0.500000000000003,0.56333468259713,0.625630678898964,0.644015076010612,
0.704247191865364,0.750000000000002,0.807879472775742,0.868482121788547,
0.928163066010689,0.961961794088669,0.999999992441328),.UNSPECIFIED.);
#372=B_SPLINE_CURVE_WITH_KNOTS('',3,(#63694,#63695,#63696,#63697,#63698,
#63699,#63700,#63701,#63702,#63703,#63704,#63705,#63706,#63707,#63708,#63709,
#63710,#63711,#63712,#63713,#63714,#63715,#63716,#63717,#63718,#63719,#63720,
#63721,#63722,#63723,#63724,#63725,#63726,#63727,#63728,#63729,#63730,#63731,
#63732,#63733,#63734,#63735,#63736,#63737,#63738,#63739,#63740,#63741,#63742,
#63743,#63744,#63745,#63746,#63747,#63748,#63749,#63750,#63751),
 .UNSPECIFIED.,.F.,.F.,(4,3,3,3,3,3,3,3,3,3,3,3,3,3,3,3,3,3,3,4),(0.,0.0706905706112055,
0.137002900415584,0.198600023213015,0.25,0.306961952173985,0.36310537274714,
0.418882023364704,0.474267462741273,0.5,0.500045996220446,0.555660447642905,
0.611744482007949,0.668197862686385,0.725353764962349,0.75,0.8125,0.877037176849364,
0.947733158289997,1.),.UNSPECIFIED.);
#373=B_SPLINE_CURVE_WITH_KNOTS('',3,(#63792,#63793,#63794,#63795,#63796,
#63797,#63798,#63799,#63800,#63801,#63802,#63803,#63804,#63805,#63806,#63807,
#63808,#63809,#63810,#63811,#63812,#63813,#63814,#63815,#63816,#63817,#63818,
#63819,#63820,#63821,#63822,#63823,#63824,#63825,#63826,#63827,#63828,#63829,
#63830,#63831,#63832,#63833,#63834,#63835,#63836,#63837,#63838,#63839,#63840,
#63841,#63842,#63843,#63844,#63845,#63846,#63847,#63848,#63849,#63850,#63851,
#63852,#63853,#63854,#63855,#63856,#63857,#63858,#63859,#63860,#63861,#63862,
#63863,#63864,#63865,#63866,#63867,#63868,#63869,#63870,#63871,#63872,#63873,
#63874,#63875,#63876),.UNSPECIFIED.,.F.,.F.,(4,3,3,3,3,3,3,3,3,3,3,3,3,
3,3,3,3,3,3,3,3,3,3,3,3,3,3,3,4),(0.,0.0706625665957282,0.124999999999996,
0.187499999999994,0.218749999999993,0.234374999999993,0.242187499999993,
0.244252489601095,0.246093749999993,0.249999999999993,0.317448736797841,
0.383780163038669,0.414395823559992,0.480730288139021,0.499999999999993,
0.565325738265915,0.585446949397997,0.624999999999993,0.687499999999993,
0.718749999999993,0.734374999999993,0.742187499999993,0.746093749999993,
0.749999999999993,0.755577493927536,0.823473673311783,0.893041632226348,
0.929181432390663,1.),.UNSPECIFIED.);
#404=(
BOUNDED_SURFACE()
B_SPLINE_SURFACE(3,3,((#41245,#41246,#41247,#41248,#41249,#41250,#41251,
#41252,#41253,#41254),(#41255,#41256,#41257,#41258,#41259,#41260,#41261,
#41262,#41263,#41264),(#41265,#41266,#41267,#41268,#41269,#41270,#41271,
#41272,#41273,#41274),(#41275,#41276,#41277,#41278,#41279,#41280,#41281,
#41282,#41283,#41284)),.UNSPECIFIED.,.F.,.F.,.F.)
B_SPLINE_SURFACE_WITH_KNOTS((4,4),(4,1,1,1,1,1,1,4),(0.0528476000136677,
0.947690598086684),(0.244373136783768,0.2805071298931,0.3579201174355,0.444129632276,
0.5371346267334,0.6323291307028,0.7265386296373,0.765696187608126),
 .UNSPECIFIED.)
GEOMETRIC_REPRESENTATION_ITEM()
RATIONAL_B_SPLINE_SURFACE(((1.20375116505837,1.20375116505837,1.20375116505837,
1.20375116505837,1.20375116505837,1.20375116505837,1.20375116505837,1.20375116505837,
1.20375116505837,1.20375116505837),(0.93191945338362,0.93191945338362,0.93191945338362,
0.93191945338362,0.93191945338362,0.93191945338362,0.93191945338362,0.93191945338362,
0.93191945338362,0.93191945338362),(0.932083043370885,0.932083043370885,
0.932083043370885,0.932083043370885,0.932083043370885,0.932083043370885,
0.932083043370885,0.932083043370885,0.932083043370885,0.932083043370885),
(1.20424193502017,1.20424193502017,1.20424193502017,1.20424193502017,1.20424193502017,
1.20424193502017,1.20424193502017,1.20424193502017,1.20424193502017,1.20424193502017)))
REPRESENTATION_ITEM('')
SURFACE()
);
#405=(
BOUNDED_SURFACE()
B_SPLINE_SURFACE(3,3,((#41381,#41382,#41383,#41384,#41385,#41386,#41387,
#41388,#41389,#41390,#41391),(#41392,#41393,#41394,#41395,#41396,#41397,
#41398,#41399,#41400,#41401,#41402),(#41403,#41404,#41405,#41406,#41407,
#41408,#41409,#41410,#41411,#41412,#41413),(#41414,#41415,#41416,#41417,
#41418,#41419,#41420,#41421,#41422,#41423,#41424)),.UNSPECIFIED.,.F.,.F.,
 .F.)
B_SPLINE_SURFACE_WITH_KNOTS((4,4),(4,1,1,1,1,1,1,1,4),(0.0434902459051769,
0.938286205395966),(-0.009351371223931,0.,0.1428542653358,0.2856978653279,
0.4287777392072,0.5720428464823,0.7151350525691,0.8578442953538,0.9437353734563),
 .UNSPECIFIED.)
GEOMETRIC_REPRESENTATION_ITEM()
RATIONAL_B_SPLINE_SURFACE(((1.1284425403519,1.1284425403519,1.1284425403519,
1.1284425403519,1.1284425403519,1.1284425403519,1.1284425403519,1.1284425403519,
1.1284425403519,1.1284425403519,1.1284425403519),(0.960604043871938,0.960604043871938,
0.960604043871938,0.960604043871938,0.960604043871938,0.960604043871938,
0.960604043871938,0.960604043871938,0.960604043871938,0.960604043871938,
0.960604043871938),(0.957254046432989,0.957254046432989,0.957254046432989,
0.957254046432989,0.957254046432989,0.957254046432989,0.957254046432989,
0.957254046432989,0.957254046432989,0.957254046432989,0.957254046432989),
(1.11839254803506,1.11839254803506,1.11839254803506,1.11839254803506,1.11839254803506,
1.11839254803506,1.11839254803506,1.11839254803506,1.11839254803506,1.11839254803506,
1.11839254803506)))
REPRESENTATION_ITEM('')
SURFACE()
);
#406=(
BOUNDED_SURFACE()
B_SPLINE_SURFACE(3,3,((#41574,#41575,#41576,#41577,#41578,#41579),(#41580,
#41581,#41582,#41583,#41584,#41585),(#41586,#41587,#41588,#41589,#41590,
#41591),(#41592,#41593,#41594,#41595,#41596,#41597)),.UNSPECIFIED.,.F.,
 .F.,.F.)
B_SPLINE_SURFACE_WITH_KNOTS((4,4),(4,1,1,4),(0.0606720802216265,0.938680242176544),
(-1.E-5,0.,0.333611620483,0.663356363542809),.UNSPECIFIED.)
GEOMETRIC_REPRESENTATION_ITEM()
RATIONAL_B_SPLINE_SURFACE(((1.17463054346692,1.17463054346692,1.17463054346692,
1.17463054346692,1.17463054346692,1.17463054346692),(0.941961451143934,
0.941961451143934,0.941961451143934,0.941961451143934,0.941961451143934,
0.941961451143934),(0.941789945358675,0.941789945358675,0.941789945358675,
0.941789945358675,0.941789945358675,0.941789945358675),(1.17411602611115,
1.17411602611115,1.17411602611115,1.17411602611115,1.17411602611115,1.17411602611115)))
REPRESENTATION_ITEM('')
SURFACE()
);
#407=(
BOUNDED_SURFACE()
B_SPLINE_SURFACE(3,3,((#41607,#41608,#41609,#41610,#41611,#41612,#41613,
#41614,#41615,#41616,#41617,#41618,#41619,#41620,#41621,#41622),(#41623,
#41624,#41625,#41626,#41627,#41628,#41629,#41630,#41631,#41632,#41633,#41634,
#41635,#41636,#41637,#41638),(#41639,#41640,#41641,#41642,#41643,#41644,
#41645,#41646,#41647,#41648,#41649,#41650,#41651,#41652,#41653,#41654),
(#41655,#41656,#41657,#41658,#41659,#41660,#41661,#41662,#41663,#41664,
#41665,#41666,#41667,#41668,#41669,#41670)),.UNSPECIFIED.,.F.,.F.,.F.)
B_SPLINE_SURFACE_WITH_KNOTS((4,4),(4,1,1,1,1,1,1,1,1,1,1,1,1,4),(0.0593643638306098,
0.933020867605329),(-0.009395290949116,0.,0.07535321742101,0.1579192703631,
0.2496876536101,0.3528405416605,0.4595218951032,0.5578812194224,0.6478328330201,
0.7283139538965,0.8001426333254,0.8679421244813,0.9343337877222,0.9520744430181),
 .UNSPECIFIED.)
GEOMETRIC_REPRESENTATION_ITEM()
RATIONAL_B_SPLINE_SURFACE(((1.07784072066994,1.07784072066994,1.07784072066994,
1.07784072066994,1.07784072066994,1.07784072066994,1.07784072066994,1.07784072066994,
1.07784072066994,1.07784072066994,1.07784072066994,1.07784072066994,1.07784072066994,
1.07784072066994,1.07784072066994,1.07784072066994),(0.97494988708073,0.97494988708073,
0.97494988708073,0.97494988708073,0.97494988708073,0.97494988708073,0.97494988708073,
0.97494988708073,0.97494988708073,0.97494988708073,0.97494988708073,0.97494988708073,
0.97494988708073,0.97494988708073,0.97494988708073,0.97494988708073),(0.974060842004898,
0.974060842004898,0.974060842004898,0.974060842004898,0.974060842004898,
0.974060842004898,0.974060842004898,0.974060842004898,0.974060842004898,
0.974060842004898,0.974060842004898,0.974060842004898,0.974060842004898,
0.974060842004898,0.974060842004898,0.974060842004898),(1.07517358544245,
1.07517358544245,1.07517358544245,1.07517358544245,1.07517358544245,1.07517358544245,
1.07517358544245,1.07517358544245,1.07517358544245,1.07517358544245,1.07517358544245,
1.07517358544245,1.07517358544245,1.07517358544245,1.07517358544245,1.07517358544245)))
REPRESENTATION_ITEM('')
SURFACE()
);
#408=(
BOUNDED_SURFACE()
B_SPLINE_SURFACE(3,3,((#42137,#42138,#42139,#42140,#42141,#42142,#42143,
#42144,#42145,#42146,#42147),(#42148,#42149,#42150,#42151,#42152,#42153,
#42154,#42155,#42156,#42157,#42158),(#42159,#42160,#42161,#42162,#42163,
#42164,#42165,#42166,#42167,#42168,#42169),(#42170,#42171,#42172,#42173,
#42174,#42175,#42176,#42177,#42178,#42179,#42180)),.UNSPECIFIED.,.F.,.F.,
 .F.)
B_SPLINE_SURFACE_WITH_KNOTS((4,4),(4,1,1,1,1,1,1,1,4),(0.0575625808515044,
0.953111018999273),(0.2692265737876,0.2759902041141,0.3429705801967,0.4189932324171,
0.4999148778522,0.5808546987381,0.6569197472851,0.7239409538869,0.730783171096),
 .UNSPECIFIED.)
GEOMETRIC_REPRESENTATION_ITEM()
RATIONAL_B_SPLINE_SURFACE(((1.19946799478327,1.19946799478327,1.19946799478327,
1.19946799478327,1.19946799478327,1.19946799478327,1.19946799478327,1.19946799478327,
1.19946799478327,1.19946799478327,1.19946799478327),(0.930302619135532,
0.930302619135532,0.930302619135532,0.930302619135532,0.930302619135532,
0.930302619135532,0.930302619135532,0.930302619135532,0.930302619135532,
0.930302619135532,0.930302619135532),(0.933549364764414,0.933549364764414,
0.933549364764414,0.933549364764414,0.933549364764414,0.933549364764414,
0.933549364764414,0.933549364764414,0.933549364764414,0.933549364764414,
0.933549364764414),(1.20920823166992,1.20920823166992,1.20920823166992,
1.20920823166992,1.20920823166992,1.20920823166992,1.20920823166992,1.20920823166992,
1.20920823166992,1.20920823166992,1.20920823166992)))
REPRESENTATION_ITEM('')
SURFACE()
);
#409=(
BOUNDED_SURFACE()
B_SPLINE_SURFACE(3,3,((#42337,#42338,#42339,#42340,#42341,#42342,#42343,
#42344,#42345,#42346),(#42347,#42348,#42349,#42350,#42351,#42352,#42353,
#42354,#42355,#42356),(#42357,#42358,#42359,#42360,#42361,#42362,#42363,
#42364,#42365,#42366),(#42367,#42368,#42369,#42370,#42371,#42372,#42373,
#42374,#42375,#42376)),.UNSPECIFIED.,.F.,.F.,.F.)
B_SPLINE_SURFACE_WITH_KNOTS((4,4),(4,1,1,1,1,1,1,4),(0.0524700928528923,
0.946598976508213),(0.233280457741109,0.275500869742,0.3703985451353,0.466098394046,
0.5590144004915,0.6447566117018,0.7216147879488,0.755011631638526),
 .UNSPECIFIED.)
GEOMETRIC_REPRESENTATION_ITEM()
RATIONAL_B_SPLINE_SURFACE(((1.20409350814067,1.20409350814067,1.20409350814067,
1.20409350814067,1.20409350814067,1.20409350814067,1.20409350814067,1.20409350814067,
1.20409350814067,1.20409350814067),(0.932251861089728,0.932251861089728,
0.932251861089728,0.932251861089728,0.932251861089728,0.932251861089728,
0.932251861089728,0.932251861089728,0.932251861089728,0.932251861089728),
(0.931969124993072,0.931969124993072,0.931969124993072,0.931969124993072,
0.931969124993072,0.931969124993072,0.931969124993072,0.931969124993072,
0.931969124993072,0.931969124993072),(1.2032452998507,1.2032452998507,1.2032452998507,
1.2032452998507,1.2032452998507,1.2032452998507,1.2032452998507,1.2032452998507,
1.2032452998507,1.2032452998507)))
REPRESENTATION_ITEM('')
SURFACE()
);
#410=(
BOUNDED_SURFACE()
B_SPLINE_SURFACE(3,3,((#42496,#42497,#42498,#42499,#42500,#42501,#42502,
#42503,#42504,#42505),(#42506,#42507,#42508,#42509,#42510,#42511,#42512,
#42513,#42514,#42515),(#42516,#42517,#42518,#42519,#42520,#42521,#42522,
#42523,#42524,#42525),(#42526,#42527,#42528,#42529,#42530,#42531,#42532,
#42533,#42534,#42535)),.UNSPECIFIED.,.F.,.F.,.F.)
B_SPLINE_SURFACE_WITH_KNOTS((4,4),(4,1,1,1,1,1,1,4),(0.0418821802266755,
0.963270218260783),(0.03308221537298,0.1426814328896,0.2856167511242,0.4287842354877,
0.5720769404683,0.7151870379729,0.857915162902,0.9460833465879),
 .UNSPECIFIED.)
GEOMETRIC_REPRESENTATION_ITEM()
RATIONAL_B_SPLINE_SURFACE(((1.13002895600752,1.13002895600752,1.13002895600752,
1.13002895600752,1.13002895600752,1.13002895600752,1.13002895600752,1.13002895600752,
1.13002895600752,1.13002895600752),(0.955682067510927,0.955682067510927,
0.955682067510927,0.955682067510927,0.955682067510927,0.955682067510927,
0.955682067510927,0.955682067510927,0.955682067510927,0.955682067510927),
(0.956662497223339,0.956662497223339,0.956662497223339,0.956662497223339,
0.956662497223339,0.956662497223339,0.956662497223339,0.956662497223339,
0.956662497223339,0.956662497223339),(1.13297024514475,1.13297024514475,
1.13297024514475,1.13297024514475,1.13297024514475,1.13297024514475,1.13297024514475,
1.13297024514475,1.13297024514475,1.13297024514475)))
REPRESENTATION_ITEM('')
SURFACE()
);
#411=(
BOUNDED_SURFACE()
B_SPLINE_SURFACE(3,3,((#42631,#42632,#42633,#42634,#42635,#42636,#42637,
#42638,#42639),(#42640,#42641,#42642,#42643,#42644,#42645,#42646,#42647,
#42648),(#42649,#42650,#42651,#42652,#42653,#42654,#42655,#42656,#42657),
(#42658,#42659,#42660,#42661,#42662,#42663,#42664,#42665,#42666)),
 .UNSPECIFIED.,.F.,.F.,.F.)
B_SPLINE_SURFACE_WITH_KNOTS((4,4),(4,1,1,1,1,1,4),(0.0492017316995449,0.946591168401197),
(0.241730229047189,0.3218312100746,0.4122894827558,0.509878641653,0.6104690130364,
0.7106140327391,0.769990672175726),.UNSPECIFIED.)
GEOMETRIC_REPRESENTATION_ITEM()
RATIONAL_B_SPLINE_SURFACE(((1.20708757459828,1.20708757459828,1.20708757459828,
1.20708757459828,1.20708757459828,1.20708757459828,1.20708757459828,1.20708757459828,
1.20708757459828),(0.93225924600194,0.93225924600194,0.93225924600194,0.93225924600194,
0.93225924600194,0.93225924600194,0.93225924600194,0.93225924600194,0.93225924600194),
(0.930976820674631,0.930976820674631,0.930976820674631,0.930976820674631,
0.930976820674631,0.930976820674631,0.930976820674631,0.930976820674631,
0.930976820674631),(1.20324029861636,1.20324029861636,1.20324029861636,
1.20324029861636,1.20324029861636,1.20324029861636,1.20324029861636,1.20324029861636,
1.20324029861636)))
REPRESENTATION_ITEM('')
SURFACE()
);
#412=(
BOUNDED_SURFACE()
B_SPLINE_SURFACE(3,3,((#42817,#42818,#42819,#42820,#42821,#42822,#42823,
#42824,#42825,#42826),(#42827,#42828,#42829,#42830,#42831,#42832,#42833,
#42834,#42835,#42836),(#42837,#42838,#42839,#42840,#42841,#42842,#42843,
#42844,#42845,#42846),(#42847,#42848,#42849,#42850,#42851,#42852,#42853,
#42854,#42855,#42856)),.UNSPECIFIED.,.F.,.F.,.F.)
B_SPLINE_SURFACE_WITH_KNOTS((4,4),(4,1,1,1,1,1,1,4),(0.0418840519216512,
0.963268772425882),(0.05391635149789,0.1420848326441,0.2848129595133,0.427923059503,
0.5712157657557,0.7143832503701,0.8573185672175,0.9669169090855),
 .UNSPECIFIED.)
GEOMETRIC_REPRESENTATION_ITEM()
RATIONAL_B_SPLINE_SURFACE(((1.13002789794623,1.13002789794623,1.13002789794623,
1.13002789794623,1.13002789794623,1.13002789794623,1.13002789794623,1.13002789794623,
1.13002789794623,1.13002789794623),(0.955682343566337,0.955682343566337,
0.955682343566337,0.955682343566337,0.955682343566337,0.955682343566337,
0.955682343566337,0.955682343566337,0.955682343566337,0.955682343566337),
(0.956662850817025,0.956662850817025,0.956662850817025,0.956662850817025,
0.956662850817025,0.956662850817025,0.956662850817025,0.956662850817025,
0.956662850817025,0.956662850817025),(1.13296941969829,1.13296941969829,
1.13296941969829,1.13296941969829,1.13296941969829,1.13296941969829,1.13296941969829,
1.13296941969829,1.13296941969829,1.13296941969829)))
REPRESENTATION_ITEM('')
SURFACE()
);
#413=(
BOUNDED_SURFACE()
B_SPLINE_SURFACE(3,3,((#43010,#43011,#43012,#43013,#43014,#43015),(#43016,
#43017,#43018,#43019,#43020,#43021),(#43022,#43023,#43024,#43025,#43026,
#43027),(#43028,#43029,#43030,#43031,#43032,#43033)),.UNSPECIFIED.,.F.,
 .F.,.F.)
B_SPLINE_SURFACE_WITH_KNOTS((4,4),(4,1,1,4),(0.0606070590319605,0.939489995881052),
(0.199119631240235,0.3331969354622,0.6668030645378,0.800880373959484),
 .UNSPECIFIED.)
GEOMETRIC_REPRESENTATION_ITEM()
RATIONAL_B_SPLINE_SURFACE(((1.17469014875841,1.17469014875841,1.17469014875841,
1.17469014875841,1.17469014875841,1.17469014875841),(0.94174422623015,0.94174422623015,
0.94174422623015,0.94174422623015,0.94174422623015,0.94174422623015),(0.941769953255028,
0.941769953255028,0.941769953255028,0.941769953255028,0.941769953255028,
0.941769953255028),(1.17476732983304,1.17476732983304,1.17476732983304,
1.17476732983304,1.17476732983304,1.17476732983304)))
REPRESENTATION_ITEM('')
SURFACE()
);
#414=(
BOUNDED_SURFACE()
B_SPLINE_SURFACE(3,3,((#43270,#43271,#43272,#43273,#43274,#43275,#43276,
#43277,#43278,#43279,#43280,#43281,#43282,#43283,#43284,#43285,#43286,#43287,
#43288,#43289),(#43290,#43291,#43292,#43293,#43294,#43295,#43296,#43297,
#43298,#43299,#43300,#43301,#43302,#43303,#43304,#43305,#43306,#43307,#43308,
#43309),(#43310,#43311,#43312,#43313,#43314,#43315,#43316,#43317,#43318,
#43319,#43320,#43321,#43322,#43323,#43324,#43325,#43326,#43327,#43328,#43329),
(#43330,#43331,#43332,#43333,#43334,#43335,#43336,#43337,#43338,#43339,
#43340,#43341,#43342,#43343,#43344,#43345,#43346,#43347,#43348,#43349)),
 .UNSPECIFIED.,.F.,.F.,.F.)
B_SPLINE_SURFACE_WITH_KNOTS((4,4),(4,1,1,1,1,1,1,1,1,1,1,1,1,1,1,1,1,4),
(0.0633076807246293,0.940122691260961),(-0.009153831274742,0.,0.07546678292497,
0.1557183846407,0.2404004052355,0.3291524428378,0.4125156378631,0.4856754559561,
0.5506573173948,0.6094478462087,0.663816257157,0.7128070375475,0.7565080779544,
0.796844405971,0.8357673160271,0.8748875859849,0.9149298599826,0.9275319405944),
 .UNSPECIFIED.)
GEOMETRIC_REPRESENTATION_ITEM()
RATIONAL_B_SPLINE_SURFACE(((1.07645082325527,1.07645082325527,1.07645082325527,
1.07645082325527,1.07645082325527,1.07645082325527,1.07645082325527,1.07645082325527,
1.07645082325527,1.07645082325527,1.07645082325527,1.07645082325527,1.07645082325527,
1.07645082325527,1.07645082325527,1.07645082325527,1.07645082325527,1.07645082325527,
1.07645082325527,1.07645082325527),(0.974116026818099,0.974116026818099,
0.974116026818099,0.974116026818099,0.974116026818099,0.974116026818099,
0.974116026818099,0.974116026818099,0.974116026818099,0.974116026818099,
0.974116026818099,0.974116026818099,0.974116026818099,0.974116026818099,
0.974116026818099,0.974116026818099,0.974116026818099,0.974116026818099,
0.974116026818099,0.974116026818099),(0.97451796475398,0.97451796475398,
0.97451796475398,0.97451796475398,0.97451796475398,0.97451796475398,0.97451796475398,
0.97451796475398,0.97451796475398,0.97451796475398,0.97451796475398,0.97451796475398,
0.97451796475398,0.97451796475398,0.97451796475398,0.97451796475398,0.97451796475398,
0.97451796475398,0.97451796475398,0.97451796475398),(1.07765663706292,1.07765663706292,
1.07765663706292,1.07765663706292,1.07765663706292,1.07765663706292,1.07765663706292,
1.07765663706292,1.07765663706292,1.07765663706292,1.07765663706292,1.07765663706292,
1.07765663706292,1.07765663706292,1.07765663706292,1.07765663706292,1.07765663706292,
1.07765663706292,1.07765663706292,1.07765663706292)))
REPRESENTATION_ITEM('')
SURFACE()
);
#415=(
BOUNDED_SURFACE()
B_SPLINE_SURFACE(3,3,((#43511,#43512,#43513,#43514,#43515,#43516,#43517,
#43518,#43519,#43520),(#43521,#43522,#43523,#43524,#43525,#43526,#43527,
#43528,#43529,#43530),(#43531,#43532,#43533,#43534,#43535,#43536,#43537,
#43538,#43539,#43540),(#43541,#43542,#43543,#43544,#43545,#43546,#43547,
#43548,#43549,#43550)),.UNSPECIFIED.,.F.,.F.,.F.)
B_SPLINE_SURFACE_WITH_KNOTS((4,4),(4,1,1,1,1,1,1,4),(0.0487270144504504,
0.946595210845177),(0.230696742769469,0.2874600436204,0.3870132096883,0.4873166151045,
0.5850151613027,0.6759386432829,0.7570631359977,0.759743251677477),
 .UNSPECIFIED.)
GEOMETRIC_REPRESENTATION_ITEM()
RATIONAL_B_SPLINE_SURFACE(((1.20752815540325,1.20752815540325,1.20752815540325,
1.20752815540325,1.20752815540325,1.20752815540325,1.20752815540325,1.20752815540325,
1.20752815540325,1.20752815540325),(0.932258068988716,0.932258068988716,
0.932258068988716,0.932258068988716,0.932258068988716,0.932258068988716,
0.932258068988716,0.932258068988716,0.932258068988716,0.932258068988716),
(0.930831381054436,0.930831381054436,0.930831381054436,0.930831381054436,
0.930831381054436,0.930831381054436,0.930831381054436,0.930831381054436,
0.930831381054436,0.930831381054436),(1.20324809160041,1.20324809160041,
1.20324809160041,1.20324809160041,1.20324809160041,1.20324809160041,1.20324809160041,
1.20324809160041,1.20324809160041,1.20324809160041)))
REPRESENTATION_ITEM('')
SURFACE()
);
#416=(
BOUNDED_SURFACE()
B_SPLINE_SURFACE(3,3,((#43670,#43671,#43672,#43673,#43674,#43675,#43676,
#43677,#43678,#43679,#43680),(#43681,#43682,#43683,#43684,#43685,#43686,
#43687,#43688,#43689,#43690,#43691),(#43692,#43693,#43694,#43695,#43696,
#43697,#43698,#43699,#43700,#43701,#43702),(#43703,#43704,#43705,#43706,
#43707,#43708,#43709,#43710,#43711,#43712,#43713)),.UNSPECIFIED.,.F.,.F.,
 .F.)
B_SPLINE_SURFACE_WITH_KNOTS((4,4),(4,1,1,1,1,1,1,1,4),(0.0595203655455625,
0.937477016075647),(0.05105962744621,0.1243082719354,0.2492351900332,0.374483525782,
0.4998948479171,0.6253218237211,0.750616579156,0.8756124488067,0.9160299520784),
 .UNSPECIFIED.)
GEOMETRIC_REPRESENTATION_ITEM()
RATIONAL_B_SPLINE_SURFACE(((1.1195805667017,1.1195805667017,1.1195805667017,
1.1195805667017,1.1195805667017,1.1195805667017,1.1195805667017,1.1195805667017,
1.1195805667017,1.1195805667017,1.1195805667017),(0.960683241153594,0.960683241153594,
0.960683241153594,0.960683241153594,0.960683241153594,0.960683241153594,
0.960683241153594,0.960683241153594,0.960683241153594,0.960683241153594,
0.960683241153594),(0.960141663299918,0.960141663299918,0.960141663299918,
0.960141663299918,0.960141663299918,0.960141663299918,0.960141663299918,
0.960141663299918,0.960141663299918,0.960141663299918,0.960141663299918),
(1.11795583314067,1.11795583314067,1.11795583314067,1.11795583314067,1.11795583314067,
1.11795583314067,1.11795583314067,1.11795583314067,1.11795583314067,1.11795583314067,
1.11795583314067)))
REPRESENTATION_ITEM('')
SURFACE()
);
#417=(
BOUNDED_SURFACE()
B_SPLINE_SURFACE(3,3,((#43947,#43948,#43949,#43950,#43951,#43952,#43953,
#43954,#43955,#43956,#43957),(#43958,#43959,#43960,#43961,#43962,#43963,
#43964,#43965,#43966,#43967,#43968),(#43969,#43970,#43971,#43972,#43973,
#43974,#43975,#43976,#43977,#43978,#43979),(#43980,#43981,#43982,#43983,
#43984,#43985,#43986,#43987,#43988,#43989,#43990)),.UNSPECIFIED.,.F.,.F.,
 .F.)
B_SPLINE_SURFACE_WITH_KNOTS((4,4),(4,1,1,1,1,1,1,1,4),(0.0574729628393945,
0.952962452837741),(0.269222366519,0.2762332346986,0.3429031113093,0.4188966873867,
0.4999818942308,0.5810709354785,0.657074202193,0.7237529548095,0.7307669759034),
 .UNSPECIFIED.)
GEOMETRIC_REPRESENTATION_ITEM()
RATIONAL_B_SPLINE_SURFACE(((1.19955084132791,1.19955084132791,1.19955084132791,
1.19955084132791,1.19955084132791,1.19955084132791,1.19955084132791,1.19955084132791,
1.19955084132791,1.19955084132791,1.19955084132791),(0.930345924831433,
0.930345924831433,0.930345924831433,0.930345924831433,0.930345924831433,
0.930345924831433,0.930345924831433,0.930345924831433,0.930345924831433,
0.930345924831433,0.930345924831433),(0.933520041857134,0.933520041857134,
0.933520041857134,0.933520041857134,0.933520041857134,0.933520041857134,
0.933520041857134,0.933520041857134,0.933520041857134,0.933520041857134,
0.933520041857134),(1.20907319240501,1.20907319240501,1.20907319240501,
1.20907319240501,1.20907319240501,1.20907319240501,1.20907319240501,1.20907319240501,
1.20907319240501,1.20907319240501,1.20907319240501)))
REPRESENTATION_ITEM('')
SURFACE()
);
#418=(
BOUNDED_SURFACE()
B_SPLINE_SURFACE(3,3,((#44088,#44089,#44090,#44091,#44092,#44093,#44094,
#44095,#44096,#44097),(#44098,#44099,#44100,#44101,#44102,#44103,#44104,
#44105,#44106,#44107),(#44108,#44109,#44110,#44111,#44112,#44113,#44114,
#44115,#44116,#44117),(#44118,#44119,#44120,#44121,#44122,#44123,#44124,
#44125,#44126,#44127)),.UNSPECIFIED.,.F.,.F.,.F.)
B_SPLINE_SURFACE_WITH_KNOTS((4,4),(4,1,1,1,1,1,1,4),(0.0479830632576071,
0.946593353952545),(0.239518392653729,0.2430457985497,0.3242077675677,0.4151597485037,
0.5128629249771,0.6131453793564,0.7126591925481,0.77004587812324),
 .UNSPECIFIED.)
GEOMETRIC_REPRESENTATION_ITEM()
RATIONAL_B_SPLINE_SURFACE(((1.20821093244647,1.20821093244647,1.20821093244647,
1.20821093244647,1.20821093244647,1.20821093244647,1.20821093244647,1.20821093244647,
1.20821093244647,1.20821093244647),(0.932261852779893,0.932261852779893,
0.932261852779893,0.932261852779893,0.932261852779893,0.932261852779893,
0.932261852779893,0.932261852779893,0.932261852779893,0.932261852779893),
(0.930606347689597,0.930606347689597,0.930606347689597,0.930606347689597,
0.930606347689597,0.930606347689597,0.930606347689597,0.930606347689597,
0.930606347689597,0.930606347689597),(1.20324441717558,1.20324441717558,
1.20324441717558,1.20324441717558,1.20324441717558,1.20324441717558,1.20324441717558,
1.20324441717558,1.20324441717558,1.20324441717558)))
REPRESENTATION_ITEM('')
SURFACE()
);
#419=(
BOUNDED_SURFACE()
B_SPLINE_SURFACE(3,3,((#44278,#44279,#44280,#44281,#44282,#44283,#44284,
#44285,#44286,#44287,#44288),(#44289,#44290,#44291,#44292,#44293,#44294,
#44295,#44296,#44297,#44298,#44299),(#44300,#44301,#44302,#44303,#44304,
#44305,#44306,#44307,#44308,#44309,#44310),(#44311,#44312,#44313,#44314,
#44315,#44316,#44317,#44318,#44319,#44320,#44321)),.UNSPECIFIED.,.F.,.F.,
 .F.)
B_SPLINE_SURFACE_WITH_KNOTS((4,4),(4,1,1,1,1,1,1,1,4),(0.0434902455975137,
0.937490443114784),(-0.009351371223931,0.,0.1428542653358,0.2856978653279,
0.4287777392072,0.5720428464823,0.7151350525691,0.8578442953538,0.9437353734563),
 .UNSPECIFIED.)
GEOMETRIC_REPRESENTATION_ITEM()
RATIONAL_B_SPLINE_SURFACE(((1.1284425406159,1.1284425406159,1.1284425406159,
1.1284425406159,1.1284425406159,1.1284425406159,1.1284425406159,1.1284425406159,
1.1284425406159,1.1284425406159,1.1284425406159),(0.960753306416933,0.960753306416933,
0.960753306416933,0.960753306416933,0.960753306416933,0.960753306416933,
0.960753306416933,0.960753306416933,0.960753306416933,0.960753306416933,
0.960753306416933),(0.95726013489752,0.95726013489752,0.95726013489752,
0.95726013489752,0.95726013489752,0.95726013489752,0.95726013489752,0.95726013489752,
0.95726013489752,0.95726013489752,0.95726013489752),(1.11796302605766,1.11796302605766,
1.11796302605766,1.11796302605766,1.11796302605766,1.11796302605766,1.11796302605766,
1.11796302605766,1.11796302605766,1.11796302605766,1.11796302605766)))
REPRESENTATION_ITEM('')
SURFACE()
);
#420=(
BOUNDED_SURFACE()
B_SPLINE_SURFACE(3,3,((#44471,#44472,#44473,#44474,#44475,#44476),(#44477,
#44478,#44479,#44480,#44481,#44482),(#44483,#44484,#44485,#44486,#44487,
#44488),(#44489,#44490,#44491,#44492,#44493,#44494)),.UNSPECIFIED.,.F.,
 .F.,.F.)
B_SPLINE_SURFACE_WITH_KNOTS((4,4),(4,1,1,4),(0.0606720802291994,0.938680242177155),
(-1.E-5,0.,0.333611620483,0.663356363538714),.UNSPECIFIED.)
GEOMETRIC_REPRESENTATION_ITEM()
RATIONAL_B_SPLINE_SURFACE(((1.1746305434609,1.1746305434609,1.1746305434609,
1.1746305434609,1.1746305434609,1.1746305434609),(0.941961451143769,0.941961451143769,
0.941961451143769,0.941961451143769,0.941961451143769,0.941961451143769),
(0.941789945360679,0.941789945360679,0.941789945360679,0.941789945360679,
0.941789945360679,0.941789945360679),(1.17411602611163,1.17411602611163,
1.17411602611163,1.17411602611163,1.17411602611163,1.17411602611163)))
REPRESENTATION_ITEM('')
SURFACE()
);
#421=(
BOUNDED_SURFACE()
B_SPLINE_SURFACE(3,3,((#44504,#44505,#44506,#44507,#44508,#44509,#44510,
#44511,#44512,#44513,#44514,#44515,#44516,#44517,#44518,#44519),(#44520,
#44521,#44522,#44523,#44524,#44525,#44526,#44527,#44528,#44529,#44530,#44531,
#44532,#44533,#44534,#44535),(#44536,#44537,#44538,#44539,#44540,#44541,
#44542,#44543,#44544,#44545,#44546,#44547,#44548,#44549,#44550,#44551),
(#44552,#44553,#44554,#44555,#44556,#44557,#44558,#44559,#44560,#44561,
#44562,#44563,#44564,#44565,#44566,#44567)),.UNSPECIFIED.,.F.,.F.,.F.)
B_SPLINE_SURFACE_WITH_KNOTS((4,4),(4,1,1,1,1,1,1,1,1,1,1,1,1,4),(0.0593643652551394,
0.933020867259932),(-0.009395290949111,0.,0.07535321742145,0.157919270364,
0.2496876536115,0.3528405416624,0.4595218951051,0.5578812194241,0.6478328330216,
0.7283139538977,0.8001426333264,0.867942124482,0.9343337877226,0.9520744430181),
 .UNSPECIFIED.)
GEOMETRIC_REPRESENTATION_ITEM()
RATIONAL_B_SPLINE_SURFACE(((1.07784072016664,1.07784072016664,1.07784072016664,
1.07784072016664,1.07784072016664,1.07784072016664,1.07784072016664,1.07784072016664,
1.07784072016664,1.07784072016664,1.07784072016664,1.07784072016664,1.07784072016664,
1.07784072016664,1.07784072016664,1.07784072016664),(0.974949887118508,
0.974949887118508,0.974949887118508,0.974949887118508,0.974949887118508,
0.974949887118508,0.974949887118508,0.974949887118508,0.974949887118508,
0.974949887118508,0.974949887118508,0.974949887118508,0.974949887118508,
0.974949887118508,0.974949887118508,0.974949887118508),(0.974060842170469,
0.974060842170469,0.974060842170469,0.974060842170469,0.974060842170469,
0.974060842170469,0.974060842170469,0.974060842170469,0.974060842170469,
0.974060842170469,0.974060842170469,0.974060842170469,0.974060842170469,
0.974060842170469,0.974060842170469,0.974060842170469),(1.07517358532252,
1.07517358532252,1.07517358532252,1.07517358532252,1.07517358532252,1.07517358532252,
1.07517358532252,1.07517358532252,1.07517358532252,1.07517358532252,1.07517358532252,
1.07517358532252,1.07517358532252,1.07517358532252,1.07517358532252,1.07517358532252)))
REPRESENTATION_ITEM('')
SURFACE()
);
#422=(
BOUNDED_SURFACE()
B_SPLINE_SURFACE(3,3,((#45034,#45035,#45036,#45037,#45038,#45039,#45040,
#45041,#45042),(#45043,#45044,#45045,#45046,#45047,#45048,#45049,#45050,
#45051),(#45052,#45053,#45054,#45055,#45056,#45057,#45058,#45059,#45060),
(#45061,#45062,#45063,#45064,#45065,#45066,#45067,#45068,#45069)),
 .UNSPECIFIED.,.F.,.F.,.F.)
B_SPLINE_SURFACE_WITH_KNOTS((4,4),(4,1,1,1,1,1,4),(0.0580455558123085,0.958568124373128),
(0.2691839650007,0.3316562569637,0.4169046927584,0.4999998690309,0.5830948871324,
0.6683429718279,0.7308256938231),.UNSPECIFIED.)
GEOMETRIC_REPRESENTATION_ITEM()
RATIONAL_B_SPLINE_SURFACE(((1.19903368770339,1.19903368770339,1.19903368770339,
1.19903368770339,1.19903368770339,1.19903368770339,1.19903368770339,1.19903368770339,
1.19903368770339),(0.928667469287341,0.928667469287341,0.928667469287341,
0.928667469287341,0.928667469287341,0.928667469287341,0.928667469287341,
0.928667469287341,0.928667469287341),(0.933749189750596,0.933749189750596,
0.933749189750596,0.933749189750596,0.933749189750596,0.933749189750596,
0.933749189750596,0.933749189750596,0.933749189750596),(1.21427884909316,
1.21427884909316,1.21427884909316,1.21427884909316,1.21427884909316,1.21427884909316,
1.21427884909316,1.21427884909316,1.21427884909316)))
REPRESENTATION_ITEM('')
SURFACE()
);
#423=(
BOUNDED_SURFACE()
B_SPLINE_SURFACE(3,3,((#45154,#45155,#45156,#45157,#45158,#45159,#45160,
#45161,#45162),(#45163,#45164,#45165,#45166,#45167,#45168,#45169,#45170,
#45171),(#45172,#45173,#45174,#45175,#45176,#45177,#45178,#45179,#45180),
(#45181,#45182,#45183,#45184,#45185,#45186,#45187,#45188,#45189)),
 .UNSPECIFIED.,.F.,.F.,.F.)
B_SPLINE_SURFACE_WITH_KNOTS((4,4),(4,1,1,1,1,1,4),(0.0491576309218551,0.946591024024462),
(0.229965585781331,0.2892821336432,0.3893944751953,0.4899684739877,0.5875628745582,
0.6780458172145,0.758314174711455),.UNSPECIFIED.)
GEOMETRIC_REPRESENTATION_ITEM()
RATIONAL_B_SPLINE_SURFACE(((1.20712810422792,1.20712810422792,1.20712810422792,
1.20712810422792,1.20712810422792,1.20712810422792,1.20712810422792,1.20712810422792,
1.20712810422792),(0.932259413774452,0.932259413774452,0.932259413774453,
0.932259413774452,0.932259413774452,0.932259413774452,0.932259413774452,
0.932259413774452,0.932259413774452),(0.930963437921561,0.930963437921561,
0.930963437921561,0.930963437921561,0.930963437921561,0.930963437921561,
0.930963437921561,0.930963437921561,0.930963437921561),(1.20324017666925,
1.20324017666925,1.20324017666925,1.20324017666925,1.20324017666925,1.20324017666925,
1.20324017666925,1.20324017666925,1.20324017666925)))
REPRESENTATION_ITEM('')
SURFACE()
);
#424=(
BOUNDED_SURFACE()
B_SPLINE_SURFACE(3,3,((#45306,#45307,#45308,#45309,#45310,#45311,#45312,
#45313,#45314,#45315),(#45316,#45317,#45318,#45319,#45320,#45321,#45322,
#45323,#45324,#45325),(#45326,#45327,#45328,#45329,#45330,#45331,#45332,
#45333,#45334,#45335),(#45336,#45337,#45338,#45339,#45340,#45341,#45342,
#45343,#45344,#45345)),.UNSPECIFIED.,.F.,.F.,.F.)
B_SPLINE_SURFACE_WITH_KNOTS((4,4),(4,1,1,1,1,1,1,4),(0.0418802231131534,
0.963270149250729),(0.03308221537293,0.1426814329309,0.2856167516997,0.4287842359667,
0.5720769404573,0.7151870370047,0.8579151611867,0.9460833465934),
 .UNSPECIFIED.)
GEOMETRIC_REPRESENTATION_ITEM()
RATIONAL_B_SPLINE_SURFACE(((1.13003006699672,1.13003006699672,1.13003006699672,
1.13003006699672,1.13003006699672,1.13003006699672,1.13003006699672,1.13003006699672,
1.13003006699672,1.13003006699672),(0.95568207640514,0.95568207640514,0.95568207640514,
0.95568207640514,0.95568207640514,0.95568207640514,0.95568207640514,0.95568207640514,
0.95568207640514,0.95568207640514),(0.956662122582739,0.956662122582739,
0.956662122582739,0.956662122582739,0.956662122582739,0.956662122582739,
0.956662122582739,0.956662122582739,0.956662122582739,0.956662122582739),
(1.13297020552952,1.13297020552952,1.13297020552952,1.13297020552952,1.13297020552952,
1.13297020552952,1.13297020552952,1.13297020552952,1.13297020552952,1.13297020552952)))
REPRESENTATION_ITEM('')
SURFACE()
);
#425=(
BOUNDED_SURFACE()
B_SPLINE_SURFACE(3,3,((#45441,#45442,#45443,#45444,#45445,#45446,#45447,
#45448,#45449),(#45450,#45451,#45452,#45453,#45454,#45455,#45456,#45457,
#45458),(#45459,#45460,#45461,#45462,#45463,#45464,#45465,#45466,#45467),
(#45468,#45469,#45470,#45471,#45472,#45473,#45474,#45475,#45476)),
 .UNSPECIFIED.,.F.,.F.,.F.)
B_SPLINE_SURFACE_WITH_KNOTS((4,4),(4,1,1,1,1,1,4),(0.0540934813622643,0.946591460873296),
(0.245865408070653,0.3024523093122,0.4027483393081,0.5068291243807,0.6089769737371,
0.7095485234591,0.76504862578338),.UNSPECIFIED.)
GEOMETRIC_REPRESENTATION_ITEM()
RATIONAL_B_SPLINE_SURFACE(((1.20261761447037,1.20261761447037,1.20261761447037,
1.20261761447037,1.20261761447037,1.20261761447037,1.20261761447037,1.20261761447037,
1.20261761447037),(0.932253305705167,0.932253305705168,0.932253305705168,
0.932253305705168,0.932253305705168,0.932253305705168,0.932253305705168,
0.932253305705168,0.932253305705168),(0.932460954535495,0.932460954535495,
0.932460954535495,0.932460954535495,0.932460954535495,0.932460954535495,
0.932460954535495,0.932460954535495,0.932460954535495),(1.20324056096136,
1.20324056096136,1.20324056096136,1.20324056096136,1.20324056096136,1.20324056096136,
1.20324056096136,1.20324056096136,1.20324056096136)))
REPRESENTATION_ITEM('')
SURFACE()
);
#426=(
BOUNDED_SURFACE()
B_SPLINE_SURFACE(3,3,((#45633,#45634,#45635,#45636,#45637,#45638,#45639,
#45640,#45641,#45642),(#45643,#45644,#45645,#45646,#45647,#45648,#45649,
#45650,#45651,#45652),(#45653,#45654,#45655,#45656,#45657,#45658,#45659,
#45660,#45661,#45662),(#45663,#45664,#45665,#45666,#45667,#45668,#45669,
#45670,#45671,#45672)),.UNSPECIFIED.,.F.,.F.,.F.)
B_SPLINE_SURFACE_WITH_KNOTS((4,4),(4,1,1,1,1,1,1,4),(0.0418829371158205,
0.963268707799286),(0.05391635148624,0.1420848319079,0.2848129590977,0.4279230594983,
0.5712157659613,0.7143832506171,0.8573185672352,0.9669169090856),
 .UNSPECIFIED.)
GEOMETRIC_REPRESENTATION_ITEM()
RATIONAL_B_SPLINE_SURFACE(((1.1300285307818,1.1300285307818,1.1300285307818,
1.1300285307818,1.1300285307818,1.1300285307818,1.1300285307818,1.1300285307818,
1.1300285307818,1.1300285307818),(0.955682353422669,0.955682353422669,0.955682353422669,
0.955682353422669,0.955682353422669,0.955682353422669,0.955682353422669,
0.955682353422669,0.955682353422669,0.955682353422669),(0.956662637361894,
0.956662637361894,0.956662637361894,0.956662637361894,0.956662637361894,
0.956662637361894,0.956662637361894,0.956662637361894,0.956662637361894,
0.956662637361894),(1.13296938259948,1.13296938259948,1.13296938259948,
1.13296938259948,1.13296938259948,1.13296938259948,1.13296938259948,1.13296938259948,
1.13296938259948,1.13296938259948)))
REPRESENTATION_ITEM('')
SURFACE()
);
#427=(
BOUNDED_SURFACE()
B_SPLINE_SURFACE(3,3,((#45826,#45827,#45828,#45829,#45830,#45831),(#45832,
#45833,#45834,#45835,#45836,#45837),(#45838,#45839,#45840,#45841,#45842,
#45843),(#45844,#45845,#45846,#45847,#45848,#45849)),.UNSPECIFIED.,.F.,
 .F.,.F.)
B_SPLINE_SURFACE_WITH_KNOTS((4,4),(4,1,1,4),(0.0606070590317961,0.939490000441598),
(0.199119625235361,0.3331969354622,0.6668030645378,0.800880379918004),
 .UNSPECIFIED.)
GEOMETRIC_REPRESENTATION_ITEM()
RATIONAL_B_SPLINE_SURFACE(((1.17469014875854,1.17469014875854,1.17469014875854,
1.17469014875854,1.17469014875854,1.17469014875854),(0.941744225021387,
0.941744225021387,0.941744225021387,0.941744225021387,0.941744225021387,
0.941744225021387),(0.941769953255252,0.941769953255252,0.941769953255252,
0.941769953255252,0.941769953255252,0.941769953255252),(1.17476733346014,
1.17476733346014,1.17476733346014,1.17476733346014,1.17476733346014,1.17476733346014)))
REPRESENTATION_ITEM('')
SURFACE()
);
#428=(
BOUNDED_SURFACE()
B_SPLINE_SURFACE(3,3,((#46086,#46087,#46088,#46089,#46090,#46091,#46092,
#46093,#46094,#46095,#46096,#46097,#46098,#46099,#46100,#46101,#46102,#46103,
#46104,#46105),(#46106,#46107,#46108,#46109,#46110,#46111,#46112,#46113,
#46114,#46115,#46116,#46117,#46118,#46119,#46120,#46121,#46122,#46123,#46124,
#46125),(#46126,#46127,#46128,#46129,#46130,#46131,#46132,#46133,#46134,
#46135,#46136,#46137,#46138,#46139,#46140,#46141,#46142,#46143,#46144,#46145),
(#46146,#46147,#46148,#46149,#46150,#46151,#46152,#46153,#46154,#46155,
#46156,#46157,#46158,#46159,#46160,#46161,#46162,#46163,#46164,#46165)),
 .UNSPECIFIED.,.F.,.F.,.F.)
B_SPLINE_SURFACE_WITH_KNOTS((4,4),(4,1,1,1,1,1,1,1,1,1,1,1,1,1,1,1,1,4),
(0.0633076755623825,0.940122691277643),(-0.009153831274746,0.,0.07546678292519,
0.1557183846411,0.2404004052361,0.3291524428384,0.4125156378636,0.4856754559566,
0.5506573173952,0.6094478462092,0.6638162571575,0.7128070375479,0.7565080779548,
0.7968444059713,0.8357673160275,0.8748875859852,0.9149298599828,0.9275319405944),
 .UNSPECIFIED.)
GEOMETRIC_REPRESENTATION_ITEM()
RATIONAL_B_SPLINE_SURFACE(((1.07645082506276,1.07645082506276,1.07645082506276,
1.07645082506276,1.07645082506276,1.07645082506276,1.07645082506276,1.07645082506276,
1.07645082506276,1.07645082506276,1.07645082506276,1.07645082506276,1.07645082506276,
1.07645082506276,1.07645082506276,1.07645082506276,1.07645082506276,1.07645082506276,
1.07645082506276,1.07645082506276),(0.974116026811419,0.974116026811419,
0.974116026811419,0.974116026811419,0.974116026811419,0.974116026811419,
0.974116026811419,0.974116026811419,0.974116026811419,0.974116026811419,
0.974116026811419,0.974116026811419,0.974116026811419,0.974116026811419,
0.974116026811419,0.974116026811419,0.974116026811419,0.974116026811419,
0.974116026811419,0.974116026811419),(0.974517964146766,0.974517964146766,
0.974517964146766,0.974517964146766,0.974517964146766,0.974517964146766,
0.974517964146766,0.974517964146766,0.974517964146766,0.974517964146766,
0.974517964146766,0.974517964146766,0.974517964146766,0.974517964146766,
0.974517964146766,0.974517964146766,0.974517964146766,0.974517964146766,
0.974517964146766,0.974517964146766),(1.0776566370688,1.0776566370688,1.0776566370688,
1.0776566370688,1.0776566370688,1.0776566370688,1.0776566370688,1.0776566370688,
1.0776566370688,1.0776566370688,1.0776566370688,1.0776566370688,1.0776566370688,
1.0776566370688,1.0776566370688,1.0776566370688,1.0776566370688,1.0776566370688,
1.0776566370688,1.0776566370688)))
REPRESENTATION_ITEM('')
SURFACE()
);
#429=(
BOUNDED_SURFACE()
B_SPLINE_SURFACE(3,3,((#46327,#46328,#46329,#46330,#46331,#46332,#46333,
#46334,#46335),(#46336,#46337,#46338,#46339,#46340,#46341,#46342,#46343,
#46344),(#46345,#46346,#46347,#46348,#46349,#46350,#46351,#46352,#46353),
(#46354,#46355,#46356,#46357,#46358,#46359,#46360,#46361,#46362)),
 .UNSPECIFIED.,.F.,.F.,.F.)
B_SPLINE_SURFACE_WITH_KNOTS((4,4),(4,1,1,1,1,1,4),(0.0550234586932618,0.946595623648369),
(0.237043609063762,0.2885350173546,0.3884487037489,0.4899228139079,0.5932141819403,
0.693729972196,0.754343676236394),.UNSPECIFIED.)
GEOMETRIC_REPRESENTATION_ITEM()
RATIONAL_B_SPLINE_SURFACE(((1.20177749083624,1.20177749083624,1.20177749083624,
1.20177749083624,1.20177749083624,1.20177749083624,1.20177749083624,1.20177749083624,
1.20177749083624),(0.932251380814184,0.932251380814184,0.932251380814185,
0.932251380814185,0.932251380814185,0.932251380814185,0.932251380814185,
0.932251380814185,0.932251380814185),(0.932741726849128,0.932741726849128,
0.932741726849128,0.932741726849128,0.932741726849128,0.932741726849128,
0.932741726849128,0.932741726849128,0.932741726849128),(1.20324852894107,
1.20324852894107,1.20324852894107,1.20324852894107,1.20324852894107,1.20324852894107,
1.20324852894107,1.20324852894107,1.20324852894107)))
REPRESENTATION_ITEM('')
SURFACE()
);
#430=(
BOUNDED_SURFACE()
B_SPLINE_SURFACE(3,3,((#46488,#46489,#46490,#46491,#46492,#46493,#46494,
#46495,#46496,#46497,#46498),(#46499,#46500,#46501,#46502,#46503,#46504,
#46505,#46506,#46507,#46508,#46509),(#46510,#46511,#46512,#46513,#46514,
#46515,#46516,#46517,#46518,#46519,#46520),(#46521,#46522,#46523,#46524,
#46525,#46526,#46527,#46528,#46529,#46530,#46531)),.UNSPECIFIED.,.F.,.F.,
 .F.)
B_SPLINE_SURFACE_WITH_KNOTS((4,4),(4,1,1,1,1,1,1,1,4),(0.0595061205631346,
0.935560325927021),(0.05105962744621,0.1243082719354,0.2492351900332,0.374483525782,
0.4998948479171,0.6253218237211,0.750616579156,0.8756124488067,0.9160299520784),
 .UNSPECIFIED.)
GEOMETRIC_REPRESENTATION_ITEM()
RATIONAL_B_SPLINE_SURFACE(((1.11958830128056,1.11958830128056,1.11958830128056,
1.11958830128056,1.11958830128056,1.11958830128056,1.11958830128056,1.11958830128056,
1.11958830128056,1.11958830128056,1.11958830128056),(0.961030162882069,
0.961030162882069,0.961030162882069,0.961030162882069,0.961030162882069,
0.961030162882069,0.961030162882069,0.961030162882069,0.961030162882069,
0.961030162882069,0.961030162882069),(0.960142233336703,0.960142233336703,
0.960142233336703,0.960142233336703,0.960142233336703,0.960142233336703,
0.960142233336703,0.960142233336703,0.960142233336703,0.960142233336703,
0.960142233336703),(1.11692451264446,1.11692451264446,1.11692451264446,
1.11692451264446,1.11692451264446,1.11692451264446,1.11692451264446,1.11692451264446,
1.11692451264446,1.11692451264446,1.11692451264446)))
REPRESENTATION_ITEM('')
SURFACE()
);
#431=(
BOUNDED_SURFACE()
B_SPLINE_SURFACE(3,3,((#46765,#46766,#46767,#46768,#46769,#46770,#46771,
#46772,#46773),(#46774,#46775,#46776,#46777,#46778,#46779,#46780,#46781,
#46782),(#46783,#46784,#46785,#46786,#46787,#46788,#46789,#46790,#46791),
(#46792,#46793,#46794,#46795,#46796,#46797,#46798,#46799,#46800)),
 .UNSPECIFIED.,.F.,.F.,.F.)
B_SPLINE_SURFACE_WITH_KNOTS((4,4),(4,1,1,1,1,1,4),(0.055545193241446,0.960521967825338),
(0.2692083078063,0.3340264203125,0.4179413584375,0.5000270643821,0.5821139624052,
0.6660288146751,0.730780783099),.UNSPECIFIED.)
GEOMETRIC_REPRESENTATION_ITEM()
RATIONAL_B_SPLINE_SURFACE(((1.20129409867085,1.20129409867085,1.20129409867085,
1.20129409867085,1.20129409867085,1.20129409867085,1.20129409867085,1.20129409867085,
1.20129409867085),(0.928050743159333,0.928050743159333,0.928050743159333,
0.928050743159333,0.928050743159333,0.928050743159333,0.928050743159333,
0.928050743159333,0.928050743159333),(0.932989653636476,0.932989653636476,
0.932989653636476,0.932989653636476,0.932989653636476,0.932989653636476,
0.932989653636476,0.932989653636476,0.932989653636476),(1.21611083010228,
1.21611083010228,1.21611083010228,1.21611083010228,1.21611083010228,1.21611083010228,
1.21611083010228,1.21611083010228,1.21611083010228)))
REPRESENTATION_ITEM('')
SURFACE()
);
#432=(
BOUNDED_SURFACE()
B_SPLINE_SURFACE(3,3,((#46871,#46872,#46873,#46874,#46875,#46876,#46877,
#46878,#46879),(#46880,#46881,#46882,#46883,#46884,#46885,#46886,#46887,
#46888),(#46889,#46890,#46891,#46892,#46893,#46894,#46895,#46896,#46897),
(#46898,#46899,#46900,#46901,#46902,#46903,#46904,#46905,#46906)),
 .UNSPECIFIED.,.F.,.F.,.F.)
B_SPLINE_SURFACE_WITH_KNOTS((4,4),(4,1,1,1,1,1,4),(0.0527983372245638,0.946599001588779),
(0.244210271093049,0.3259550556335,0.4264563043828,0.5263661020306,0.6246508850818,
0.7212192975236,0.765147692445861),.UNSPECIFIED.)
GEOMETRIC_REPRESENTATION_ITEM()
RATIONAL_B_SPLINE_SURFACE(((1.20379704514701,1.20379704514701,1.20379704514701,
1.20379704514701,1.20379704514701,1.20379704514701,1.20379704514701,1.20379704514701,
1.20379704514701),(0.93225074659745,0.93225074659745,0.93225074659745,0.93225074659745,
0.93225074659745,0.93225074659745,0.93225074659745,0.93225074659745,0.93225074659745),
(0.932067774989629,0.932067774989629,0.932067774989629,0.932067774989629,
0.932067774989629,0.932067774989629,0.932067774989629,0.932067774989629,
0.932067774989629),(1.20324813032355,1.20324813032355,1.20324813032355,
1.20324813032355,1.20324813032355,1.20324813032355,1.20324813032355,1.20324813032355,
1.20324813032355)))
REPRESENTATION_ITEM('')
SURFACE()
);
#433=(
BOUNDED_SURFACE()
B_SPLINE_SURFACE(3,3,((#47062,#47063,#47064,#47065,#47066,#47067,#47068,
#47069,#47070,#47071,#47072),(#47073,#47074,#47075,#47076,#47077,#47078,
#47079,#47080,#47081,#47082,#47083),(#47084,#47085,#47086,#47087,#47088,
#47089,#47090,#47091,#47092,#47093,#47094),(#47095,#47096,#47097,#47098,
#47099,#47100,#47101,#47102,#47103,#47104,#47105)),.UNSPECIFIED.,.F.,.F.,
 .F.)
B_SPLINE_SURFACE_WITH_KNOTS((4,4),(4,1,1,1,1,1,1,1,4),(0.0422658727921174,
0.937259435667498),(-0.009351371223903,0.,0.1428542653358,0.2856978653279,
0.4287777392072,0.5720428464823,0.7151350525691,0.8578442953538,0.9437353734563),
 .UNSPECIFIED.)
GEOMETRIC_REPRESENTATION_ITEM()
RATIONAL_B_SPLINE_SURFACE(((1.12913243791303,1.12913243791303,1.12913243791303,
1.12913243791303,1.12913243791303,1.12913243791303,1.12913243791303,1.12913243791303,
1.12913243791303,1.12913243791303,1.12913243791303),(0.960806629223671,
0.960806629223671,0.960806629223671,0.960806629223671,0.960806629223671,
0.960806629223671,0.960806629223671,0.960806629223671,0.960806629223671,
0.960806629223671,0.960806629223671),(0.957041977642826,0.957041977642826,
0.957041977642826,0.957041977642826,0.957041977642826,0.957041977642826,
0.957041977642826,0.957041977642826,0.957041977642826,0.957041977642826,
0.957041977642826),(1.11783848317049,1.11783848317049,1.11783848317049,
1.11783848317049,1.11783848317049,1.11783848317049,1.11783848317049,1.11783848317049,
1.11783848317049,1.11783848317049,1.11783848317049)))
REPRESENTATION_ITEM('')
SURFACE()
);
#434=(
BOUNDED_SURFACE()
B_SPLINE_SURFACE(3,3,((#47255,#47256,#47257,#47258,#47259,#47260),(#47261,
#47262,#47263,#47264,#47265,#47266),(#47267,#47268,#47269,#47270,#47271,
#47272),(#47273,#47274,#47275,#47276,#47277,#47278)),.UNSPECIFIED.,.F.,
 .F.,.F.)
B_SPLINE_SURFACE_WITH_KNOTS((4,4),(4,1,1,4),(0.0606720802170434,0.938680239730501),
(-1.E-5,0.,0.333614254626,0.663356363343292),.UNSPECIFIED.)
GEOMETRIC_REPRESENTATION_ITEM()
RATIONAL_B_SPLINE_SURFACE(((1.17463054347057,1.17463054347057,1.17463054347057,
1.17463054347057,1.17463054347057,1.17463054347057),(0.941961451792129,
0.941961451792129,0.941961451792129,0.941961451792129,0.941961451792129,
0.941961451792129),(0.941789945358418,0.941789945358418,0.941789945358418,
0.941789945358418,0.941789945358418,0.941789945358418),(1.17411602416943,
1.17411602416943,1.17411602416943,1.17411602416943,1.17411602416943,1.17411602416943)))
REPRESENTATION_ITEM('')
SURFACE()
);
#435=(
BOUNDED_SURFACE()
B_SPLINE_SURFACE(3,3,((#47288,#47289,#47290,#47291,#47292,#47293,#47294,
#47295,#47296,#47297,#47298,#47299,#47300,#47301,#47302,#47303),(#47304,
#47305,#47306,#47307,#47308,#47309,#47310,#47311,#47312,#47313,#47314,#47315,
#47316,#47317,#47318,#47319),(#47320,#47321,#47322,#47323,#47324,#47325,
#47326,#47327,#47328,#47329,#47330,#47331,#47332,#47333,#47334,#47335),
(#47336,#47337,#47338,#47339,#47340,#47341,#47342,#47343,#47344,#47345,
#47346,#47347,#47348,#47349,#47350,#47351)),.UNSPECIFIED.,.F.,.F.,.F.)
B_SPLINE_SURFACE_WITH_KNOTS((4,4),(4,1,1,1,1,1,1,1,1,1,1,1,1,4),(0.0600759826757179,
0.933027467697898),(-0.009395290946096,0.,0.0753532717085,0.1579194084299,
0.2496878347785,0.3528404724376,0.4595208130976,0.5578799794626,0.6478320754114,
0.7283136662239,0.8001425287391,0.8679420769042,0.9343337648423,0.9520744430431),
 .UNSPECIFIED.)
GEOMETRIC_REPRESENTATION_ITEM()
RATIONAL_B_SPLINE_SURFACE(((1.07758950148,1.07758950148,1.07758950148,1.07758950148,
1.07758950148,1.07758950148,1.07758950148,1.07758950148,1.07758950148,1.07758950148,
1.07758950148,1.07758950148,1.07758950148,1.07758950148,1.07758950148,1.07758950148),
(0.974947730216909,0.974947730216909,0.974947730216909,0.974947730216909,
0.974947730216909,0.974947730216909,0.974947730216909,0.974947730216909,
0.974947730216909,0.974947730216909,0.974947730216909,0.974947730216909,
0.974947730216909,0.974947730216909,0.974947730216909,0.974947730216909),
(0.974143188930937,0.974143188930937,0.974143188930937,0.974143188930937,
0.974143188930937,0.974143188930937,0.974143188930937,0.974143188930937,
0.974143188930937,0.974143188930937,0.974143188930937,0.974143188930937,
0.974143188930937,0.974143188930937,0.974143188930937,0.974143188930937),
(1.07517587762208,1.07517587762208,1.07517587762208,1.07517587762208,1.07517587762208,
1.07517587762208,1.07517587762208,1.07517587762208,1.07517587762208,1.07517587762208,
1.07517587762208,1.07517587762208,1.07517587762208,1.07517587762208,1.07517587762208,
1.07517587762208)))
REPRESENTATION_ITEM('')
SURFACE()
);
#436=(
BOUNDED_SURFACE()
B_SPLINE_SURFACE(3,3,((#47818,#47819,#47820,#47821,#47822,#47823,#47824,
#47825,#47826,#47827,#47828),(#47829,#47830,#47831,#47832,#47833,#47834,
#47835,#47836,#47837,#47838,#47839),(#47840,#47841,#47842,#47843,#47844,
#47845,#47846,#47847,#47848,#47849,#47850),(#47851,#47852,#47853,#47854,
#47855,#47856,#47857,#47858,#47859,#47860,#47861)),.UNSPECIFIED.,.F.,.F.,
 .F.)
B_SPLINE_SURFACE_WITH_KNOTS((4,4),(4,1,1,1,1,1,1,1,4),(0.0572310664754211,
0.950572798231042),(0.2692300395995,0.2751075328761,0.3418387429095,0.417931198782,
0.4999456991685,0.5819697696493,0.6580841324447,0.7248361845443,0.7307799588033),
 .UNSPECIFIED.)
GEOMETRIC_REPRESENTATION_ITEM()
RATIONAL_B_SPLINE_SURFACE(((1.19976708046968,1.19976708046968,1.19976708046968,
1.19976708046968,1.19976708046968,1.19976708046968,1.19976708046968,1.19976708046968,
1.19976708046968,1.19976708046968,1.19976708046968),(0.931063691256385,
0.931063691256385,0.931063691256385,0.931063691256385,0.931063691256385,
0.931063691256385,0.931063691256385,0.931063691256385,0.931063691256385,
0.931063691256385,0.931063691256385),(0.933431658763609,0.933431658763609,
0.933431658763609,0.933431658763609,0.933431658763609,0.933431658763609,
0.933431658763609,0.933431658763609,0.933431658763609,0.933431658763609,
0.933431658763609),(1.20687098299135,1.20687098299135,1.20687098299135,
1.20687098299135,1.20687098299135,1.20687098299135,1.20687098299135,1.20687098299135,
1.20687098299135,1.20687098299135,1.20687098299135)))
REPRESENTATION_ITEM('')
SURFACE()
);
#437=(
BOUNDED_SURFACE()
B_SPLINE_SURFACE(3,3,((#48021,#48022,#48023,#48024,#48025,#48026,#48027,
#48028,#48029),(#48030,#48031,#48032,#48033,#48034,#48035,#48036,#48037,
#48038),(#48039,#48040,#48041,#48042,#48043,#48044,#48045,#48046,#48047),
(#48048,#48049,#48050,#48051,#48052,#48053,#48054,#48055,#48056)),
 .UNSPECIFIED.,.F.,.F.,.F.)
B_SPLINE_SURFACE_WITH_KNOTS((4,4),(4,1,1,1,1,1,4),(0.0524039687756051,0.946596210479273),
(0.233297759115741,0.279643029582,0.3765118146602,0.4751376597475,0.5753331138272,
0.6758913779353,0.755181913864713),.UNSPECIFIED.)
GEOMETRIC_REPRESENTATION_ITEM()
RATIONAL_B_SPLINE_SURFACE(((1.2041545053254,1.2041545053254,1.2041545053254,
1.2041545053254,1.2041545053254,1.2041545053254,1.2041545053254,1.2041545053254,
1.2041545053254),(0.932252519254702,0.932252519254703,0.932252519254703,
0.932252519254703,0.932252519254703,0.932252519254703,0.932252519254703,
0.932252519254703,0.932252519254703),(0.931948837779277,0.931948837779277,
0.931948837779277,0.931948837779277,0.931948837779277,0.931948837779277,
0.931948837779277,0.931948837779277,0.931948837779277),(1.20324346089913,
1.20324346089913,1.20324346089913,1.20324346089913,1.20324346089913,1.20324346089913,
1.20324346089913,1.20324346089913,1.20324346089913)))
REPRESENTATION_ITEM('')
SURFACE()
);
#438=(
BOUNDED_SURFACE()
B_SPLINE_SURFACE(3,3,((#48157,#48158,#48159,#48160,#48161,#48162,#48163,
#48164,#48165,#48166),(#48167,#48168,#48169,#48170,#48171,#48172,#48173,
#48174,#48175,#48176),(#48177,#48178,#48179,#48180,#48181,#48182,#48183,
#48184,#48185,#48186),(#48187,#48188,#48189,#48190,#48191,#48192,#48193,
#48194,#48195,#48196)),.UNSPECIFIED.,.F.,.F.,.F.)
B_SPLINE_SURFACE_WITH_KNOTS((4,4),(4,1,1,1,1,1,1,4),(0.0418820588917568,
0.963270218620141),(0.03308221537277,0.1426814329706,0.285616752253,0.4287842364271,
0.5720769404467,0.7151870360741,0.8579151595379,0.9460833466108),
 .UNSPECIFIED.)
GEOMETRIC_REPRESENTATION_ITEM()
RATIONAL_B_SPLINE_SURFACE(((1.13002902488611,1.13002902488611,1.13002902488611,
1.13002902488611,1.13002902488611,1.13002902488611,1.13002902488611,1.13002902488611,
1.13002902488611,1.13002902488611),(0.955682067184747,0.955682067184747,
0.955682067184747,0.955682067184747,0.955682067184747,0.955682067184747,
0.955682067184747,0.955682067184747,0.955682067184747,0.955682067184747),
(0.956662474006688,0.956662474006688,0.956662474006688,0.956662474006688,
0.956662474006688,0.956662474006688,0.956662474006688,0.956662474006688,
0.956662474006688,0.956662474006688),(1.13297024535194,1.13297024535194,
1.13297024535194,1.13297024535194,1.13297024535194,1.13297024535194,1.13297024535194,
1.13297024535194,1.13297024535194,1.13297024535194)))
REPRESENTATION_ITEM('')
SURFACE()
);
#439=(
BOUNDED_SURFACE()
B_SPLINE_SURFACE(3,3,((#48292,#48293,#48294,#48295,#48296,#48297,#48298,
#48299,#48300),(#48301,#48302,#48303,#48304,#48305,#48306,#48307,#48308,
#48309),(#48310,#48311,#48312,#48313,#48314,#48315,#48316,#48317,#48318),
(#48319,#48320,#48321,#48322,#48323,#48324,#48325,#48326,#48327)),
 .UNSPECIFIED.,.F.,.F.,.F.)
B_SPLINE_SURFACE_WITH_KNOTS((4,4),(4,1,1,1,1,1,4),(0.0550113442417672,0.946590905096635),
(0.245672692603397,0.293915687091,0.3999811782267,0.5047555052941,0.607503035598,
0.7085304952283,0.764913517676986),.UNSPECIFIED.)
GEOMETRIC_REPRESENTATION_ITEM()
RATIONAL_B_SPLINE_SURFACE(((1.20178444363563,1.20178444363563,1.20178444363563,
1.20178444363563,1.20178444363563,1.20178444363563,1.20178444363563,1.20178444363563,
1.20178444363563),(0.932254148400803,0.932254148400803,0.932254148400803,
0.932254148400803,0.932254148400803,0.932254148400803,0.932254148400803,
0.932254148400803,0.932254148400803),(0.932739390812751,0.932739390812751,
0.932739390812751,0.932739390812751,0.932739390812751,0.932739390812751,
0.932739390812751,0.932739390812751,0.932739390812751),(1.20324017087147,
1.20324017087147,1.20324017087147,1.20324017087147,1.20324017087147,1.20324017087147,
1.20324017087147,1.20324017087147,1.20324017087147)))
REPRESENTATION_ITEM('')
SURFACE()
);
#440=(
BOUNDED_SURFACE()
B_SPLINE_SURFACE(3,3,((#48486,#48487,#48488,#48489,#48490,#48491,#48492,
#48493,#48494,#48495),(#48496,#48497,#48498,#48499,#48500,#48501,#48502,
#48503,#48504,#48505),(#48506,#48507,#48508,#48509,#48510,#48511,#48512,
#48513,#48514,#48515),(#48516,#48517,#48518,#48519,#48520,#48521,#48522,
#48523,#48524,#48525)),.UNSPECIFIED.,.F.,.F.,.F.)
B_SPLINE_SURFACE_WITH_KNOTS((4,4),(4,1,1,1,1,1,1,4),(0.0418824149398342,
0.963268707201785),(0.05391635144762,0.142084832232,0.2848129592807,0.4279230595004,
0.5712157658708,0.7143832505083,0.8573185672274,0.966916909086),
 .UNSPECIFIED.)
GEOMETRIC_REPRESENTATION_ITEM()
RATIONAL_B_SPLINE_SURFACE(((1.13002882720305,1.13002882720305,1.13002882720305,
1.13002882720305,1.13002882720305,1.13002882720305,1.13002882720305,1.13002882720305,
1.13002882720305,1.13002882720305),(0.955682352424675,0.955682352424675,
0.955682352424675,0.955682352424675,0.955682352424675,0.955682352424675,
0.955682352424675,0.955682352424675,0.955682352424675,0.955682352424675),
(0.956662537442487,0.956662537442487,0.956662537442487,0.956662537442487,
0.956662537442487,0.956662537442487,0.956662537442487,0.956662537442487,
0.956662537442487,0.956662537442487),(1.13296938225648,1.13296938225648,
1.13296938225648,1.13296938225648,1.13296938225648,1.13296938225648,1.13296938225648,
1.13296938225648,1.13296938225648,1.13296938225648)))
REPRESENTATION_ITEM('')
SURFACE()
);
#441=(
BOUNDED_SURFACE()
B_SPLINE_SURFACE(3,3,((#48679,#48680,#48681,#48682,#48683,#48684),(#48685,
#48686,#48687,#48688,#48689,#48690),(#48691,#48692,#48693,#48694,#48695,
#48696),(#48697,#48698,#48699,#48700,#48701,#48702)),.UNSPECIFIED.,.F.,
 .F.,.F.)
B_SPLINE_SURFACE_WITH_KNOTS((4,4),(4,1,1,4),(0.0606070589585487,0.939489994809047),
(0.199119633361316,0.3331969354622,0.6668030645378,0.800880372533487),
 .UNSPECIFIED.)
GEOMETRIC_REPRESENTATION_ITEM()
RATIONAL_B_SPLINE_SURFACE(((1.17469014881678,1.17469014881678,1.17469014881678,
1.17469014881678,1.17469014881678,1.17469014881678),(0.941744226514278,
0.941744226514278,0.941744226514278,0.941744226514278,0.941744226514278,
0.941744226514278),(0.941769953235504,0.941769953235505,0.941769953235504,
0.941769953235504,0.941769953235504,0.941769953235504),(1.17476732898046,
1.17476732898046,1.17476732898046,1.17476732898046,1.17476732898046,1.17476732898046)))
REPRESENTATION_ITEM('')
SURFACE()
);
#442=(
BOUNDED_SURFACE()
B_SPLINE_SURFACE(3,3,((#48972,#48973,#48974,#48975,#48976,#48977,#48978,
#48979,#48980,#48981,#48982,#48983,#48984,#48985,#48986,#48987,#48988,#48989,
#48990,#48991),(#48992,#48993,#48994,#48995,#48996,#48997,#48998,#48999,
#49000,#49001,#49002,#49003,#49004,#49005,#49006,#49007,#49008,#49009,#49010,
#49011),(#49012,#49013,#49014,#49015,#49016,#49017,#49018,#49019,#49020,
#49021,#49022,#49023,#49024,#49025,#49026,#49027,#49028,#49029,#49030,#49031),
(#49032,#49033,#49034,#49035,#49036,#49037,#49038,#49039,#49040,#49041,
#49042,#49043,#49044,#49045,#49046,#49047,#49048,#49049,#49050,#49051)),
 .UNSPECIFIED.,.F.,.F.,.F.)
B_SPLINE_SURFACE_WITH_KNOTS((4,4),(4,1,1,1,1,1,1,1,1,1,1,1,1,1,1,1,1,4),
(0.0633076715126945,0.939196073757282),(-0.009153831276904,0.,0.07546659124057,
0.1557180876065,0.2404001363499,0.3291523816843,0.4125158427863,0.4856758619718,
0.550657876718,0.6094485282688,0.6638170257842,0.7128077767047,0.7565087359809,
0.7968449582087,0.83576776035,0.8748879264935,0.9149300941035,0.92753194056),
 .UNSPECIFIED.)
GEOMETRIC_REPRESENTATION_ITEM()
RATIONAL_B_SPLINE_SURFACE(((1.07645082698873,1.07645082698873,1.07645082698873,
1.07645082698873,1.07645082698873,1.07645082698873,1.07645082698873,1.07645082698873,
1.07645082698873,1.07645082698873,1.07645082698873,1.07645082698873,1.07645082698873,
1.07645082698873,1.07645082698873,1.07645082698873,1.07645082698873,1.07645082698873,
1.07645082698873,1.07645082698873),(0.974224173983562,0.974224173983562,
0.974224173983562,0.974224173983562,0.974224173983562,0.974224173983562,
0.974224173983562,0.974224173983562,0.974224173983562,0.974224173983562,
0.974224173983562,0.974224173983562,0.974224173983562,0.974224173983562,
0.974224173983562,0.974224173983562,0.974224173983562,0.974224173983562,
0.974224173983562,0.974224173983562),(0.974517228706797,0.974517228706797,
0.974517228706797,0.974517228706797,0.974517228706797,0.974517228706797,
0.974517228706797,0.974517228706797,0.974517228706797,0.974517228706797,
0.974517228706797,0.974517228706797,0.974517228706797,0.974517228706797,
0.974517228706797,0.974517228706797,0.974517228706797,0.974517228706797,
0.974517228706797,0.974517228706797),(1.07732999115843,1.07732999115843,
1.07732999115843,1.07732999115843,1.07732999115843,1.07732999115843,1.07732999115843,
1.07732999115843,1.07732999115843,1.07732999115843,1.07732999115843,1.07732999115843,
1.07732999115843,1.07732999115843,1.07732999115843,1.07732999115843,1.07732999115843,
1.07732999115843,1.07732999115843,1.07732999115843)))
REPRESENTATION_ITEM('')
SURFACE()
);
#443=(
BOUNDED_SURFACE()
B_SPLINE_SURFACE(3,3,((#49213,#49214,#49215,#49216,#49217,#49218,#49219,
#49220,#49221),(#49222,#49223,#49224,#49225,#49226,#49227,#49228,#49229,
#49230),(#49231,#49232,#49233,#49234,#49235,#49236,#49237,#49238,#49239),
(#49240,#49241,#49242,#49243,#49244,#49245,#49246,#49247,#49248)),
 .UNSPECIFIED.,.F.,.F.,.F.)
B_SPLINE_SURFACE_WITH_KNOTS((4,4),(4,1,1,1,1,1,4),(0.055506584836218,0.946593944947033),
(0.236411568203208,0.2913697515911,0.3923800891028,0.4951121067649,0.5998777813914,
0.7059484945911,0.755322160627775),.UNSPECIFIED.)
GEOMETRIC_REPRESENTATION_ITEM()
RATIONAL_B_SPLINE_SURFACE(((1.2013399063862,1.2013399063862,1.2013399063862,
1.2013399063862,1.2013399063862,1.2013399063862,1.2013399063862,1.2013399063862,
1.2013399063862),(0.93225238705743,0.93225238705743,0.93225238705743,0.93225238705743,
0.93225238705743,0.93225238705743,0.93225238705743,0.93225238705743,0.93225238705743),
(0.932888196643544,0.932888196643544,0.932888196643544,0.932888196643544,
0.932888196643544,0.932888196643544,0.932888196643544,0.932888196643544,
0.932888196643544),(1.20324733514454,1.20324733514454,1.20324733514454,
1.20324733514454,1.20324733514454,1.20324733514454,1.20324733514454,1.20324733514454,
1.20324733514454)))
REPRESENTATION_ITEM('')
SURFACE()
);
#444=(
BOUNDED_SURFACE()
B_SPLINE_SURFACE(3,3,((#49371,#49372,#49373,#49374,#49375,#49376,#49377,
#49378,#49379,#49380,#49381),(#49382,#49383,#49384,#49385,#49386,#49387,
#49388,#49389,#49390,#49391,#49392),(#49393,#49394,#49395,#49396,#49397,
#49398,#49399,#49400,#49401,#49402,#49403),(#49404,#49405,#49406,#49407,
#49408,#49409,#49410,#49411,#49412,#49413,#49414)),.UNSPECIFIED.,.F.,.F.,
 .F.)
B_SPLINE_SURFACE_WITH_KNOTS((4,4),(4,1,1,1,1,1,1,1,4),(0.0595080337692124,
0.938373838344971),(0.05105962744621,0.1243082719354,0.2492351900332,0.374483525782,
0.4998948479171,0.6253218237211,0.750616579156,0.8756124488067,0.9160299520784),
 .UNSPECIFIED.)
GEOMETRIC_REPRESENTATION_ITEM()
RATIONAL_B_SPLINE_SURFACE(((1.11958726248623,1.11958726248623,1.11958726248623,
1.11958726248623,1.11958726248623,1.11958726248623,1.11958726248623,1.11958726248623,
1.11958726248623,1.11958726248623,1.11958726248623),(0.960520940102268,
0.960520940102268,0.960520940102268,0.960520940102268,0.960520940102268,
0.960520940102268,0.960520940102268,0.960520940102268,0.960520940102268,
0.960520940102268,0.960520940102268),(0.960138500876397,0.960138500876397,
0.960138500876397,0.960138500876397,0.960138500876397,0.960138500876397,
0.960138500876397,0.960138500876397,0.960138500876397,0.960138500876397,
0.960138500876397),(1.11843994480862,1.11843994480862,1.11843994480862,
1.11843994480862,1.11843994480862,1.11843994480862,1.11843994480862,1.11843994480862,
1.11843994480862,1.11843994480862,1.11843994480862)))
REPRESENTATION_ITEM('')
SURFACE()
);
#445=(
BOUNDED_SURFACE()
B_SPLINE_SURFACE(3,3,((#49648,#49649,#49650,#49651,#49652,#49653,#49654,
#49655,#49656),(#49657,#49658,#49659,#49660,#49661,#49662,#49663,#49664,
#49665),(#49666,#49667,#49668,#49669,#49670,#49671,#49672,#49673,#49674),
(#49675,#49676,#49677,#49678,#49679,#49680,#49681,#49682,#49683)),
 .UNSPECIFIED.,.F.,.F.,.F.)
B_SPLINE_SURFACE_WITH_KNOTS((4,4),(4,1,1,1,1,1,4),(0.0580450064981613,0.95970901530257),
(0.2691730573356,0.3323186552644,0.4172250302096,0.5000005102551,0.5827761716977,
0.6676829731686,0.7308158292446),.UNSPECIFIED.)
GEOMETRIC_REPRESENTATION_ITEM()
RATIONAL_B_SPLINE_SURFACE(((1.1990364284185,1.1990364284185,1.1990364284185,
1.1990364284185,1.1990364284185,1.1990364284185,1.1990364284185,1.1990364284185,
1.1990364284185),(0.928324121230913,0.928324121230913,0.928324121230913,
0.928324121230913,0.928324121230913,0.928324121230913,0.928324121230913,
0.928324121230913,0.928324121230913),(0.933761589156609,0.933761589156609,
0.933761589156609,0.933761589156609,0.933761589156609,0.933761589156609,
0.933761589156609,0.933761589156609,0.933761589156609),(1.21534883219559,
1.21534883219559,1.21534883219559,1.21534883219559,1.21534883219559,1.21534883219559,
1.21534883219559,1.21534883219559,1.21534883219559)))
REPRESENTATION_ITEM('')
SURFACE()
);
#446=(
BOUNDED_SURFACE()
B_SPLINE_SURFACE(3,3,((#49766,#49767,#49768,#49769,#49770,#49771,#49772,
#49773,#49774,#49775),(#49776,#49777,#49778,#49779,#49780,#49781,#49782,
#49783,#49784,#49785),(#49786,#49787,#49788,#49789,#49790,#49791,#49792,
#49793,#49794,#49795),(#49796,#49797,#49798,#49799,#49800,#49801,#49802,
#49803,#49804,#49805)),.UNSPECIFIED.,.F.,.F.,.F.)
B_SPLINE_SURFACE_WITH_KNOTS((4,4),(4,1,1,1,1,1,1,4),(0.0528241875078419,
0.947906039093121),(0.244350846833031,0.2800690513799,0.3573786635911,0.443483668411,
0.5364412743718,0.6317122802247,0.7260664139081,0.765913579734812),
 .UNSPECIFIED.)
GEOMETRIC_REPRESENTATION_ITEM()
RATIONAL_B_SPLINE_SURFACE(((1.20377260436513,1.20377260436513,1.20377260436513,
1.20377260436513,1.20377260436513,1.20377260436513,1.20377260436513,1.20377260436513,
1.20377260436513,1.20377260436513),(0.931853961596766,0.931853961596766,
0.931853961596766,0.931853961596766,0.931853961596766,0.931853961596766,
0.931853961596766,0.931853961596766,0.931853961596766,0.931853961596766),
(0.932075979671873,0.932075979671873,0.932075979671873,0.932075979671873,
0.932075979671873,0.932075979671873,0.932075979671873,0.932075979671873,
0.932075979671873,0.932075979671873),(1.20443865859045,1.20443865859045,
1.20443865859045,1.20443865859045,1.20443865859045,1.20443865859045,1.20443865859045,
1.20443865859045,1.20443865859045,1.20443865859045)))
REPRESENTATION_ITEM('')
SURFACE()
);
#447=(
BOUNDED_SURFACE()
B_SPLINE_SURFACE(3,3,((#49902,#49903,#49904,#49905,#49906,#49907,#49908,
#49909,#49910,#49911,#49912),(#49913,#49914,#49915,#49916,#49917,#49918,
#49919,#49920,#49921,#49922,#49923),(#49924,#49925,#49926,#49927,#49928,
#49929,#49930,#49931,#49932,#49933,#49934),(#49935,#49936,#49937,#49938,
#49939,#49940,#49941,#49942,#49943,#49944,#49945)),.UNSPECIFIED.,.F.,.F.,
 .F.)
B_SPLINE_SURFACE_WITH_KNOTS((4,4),(4,1,1,1,1,1,1,1,4),(0.0434902476857429,
0.938303096471174),(-0.009351371213968,0.,0.1428545029,0.2856984060337,
0.4287781897902,0.5720429752755,0.7151346717899,0.857843506892,0.9437353739471),
 .UNSPECIFIED.)
GEOMETRIC_REPRESENTATION_ITEM()
RATIONAL_B_SPLINE_SURFACE(((1.12844253935412,1.12844253935412,1.12844253935412,
1.12844253935412,1.12844253935412,1.12844253935412,1.12844253935412,1.12844253935412,
1.12844253935412,1.12844253935412,1.12844253935412),(0.960600875567781,
0.960600875567781,0.960600875567781,0.960600875567781,0.960600875567781,
0.960600875567781,0.960600875567781,0.960600875567781,0.960600875567781,
0.960600875567781,0.960600875567781),(0.957253920334955,0.957253920334955,
0.957253920334955,0.957253920334955,0.957253920334955,0.957253920334955,
0.957253920334955,0.957253920334955,0.957253920334955,0.957253920334955,
0.957253920334955),(1.11840167365564,1.11840167365564,1.11840167365564,
1.11840167365564,1.11840167365564,1.11840167365564,1.11840167365564,1.11840167365564,
1.11840167365564,1.11840167365564,1.11840167365564)))
REPRESENTATION_ITEM('')
SURFACE()
);
#448=(
BOUNDED_SURFACE()
B_SPLINE_SURFACE(3,3,((#50095,#50096,#50097,#50098,#50099,#50100),(#50101,
#50102,#50103,#50104,#50105,#50106),(#50107,#50108,#50109,#50110,#50111,
#50112),(#50113,#50114,#50115,#50116,#50117,#50118)),.UNSPECIFIED.,.F.,
 .F.,.F.)
B_SPLINE_SURFACE_WITH_KNOTS((4,4),(4,1,1,4),(0.0606720801613996,0.938680242177229),
(-1.E-5,0.,0.3336142546261,0.6633563633615),.UNSPECIFIED.)
GEOMETRIC_REPRESENTATION_ITEM()
RATIONAL_B_SPLINE_SURFACE(((1.1746305435148,1.1746305435148,1.1746305435148,
1.1746305435148,1.1746305435148,1.1746305435148),(0.941961451143776,0.941961451143776,
0.941961451143776,0.941961451143776,0.941961451143776,0.941961451143776),
(0.941789945342739,0.941789945342739,0.941789945342739,0.941789945342739,
0.941789945342739,0.941789945342739),(1.17411602611169,1.17411602611169,
1.17411602611169,1.17411602611169,1.17411602611169,1.17411602611169)))
REPRESENTATION_ITEM('')
SURFACE()
);
#449=(
BOUNDED_SURFACE()
B_SPLINE_SURFACE(3,3,((#50128,#50129,#50130,#50131,#50132,#50133,#50134,
#50135,#50136,#50137,#50138,#50139,#50140,#50141,#50142,#50143),(#50144,
#50145,#50146,#50147,#50148,#50149,#50150,#50151,#50152,#50153,#50154,#50155,
#50156,#50157,#50158,#50159),(#50160,#50161,#50162,#50163,#50164,#50165,
#50166,#50167,#50168,#50169,#50170,#50171,#50172,#50173,#50174,#50175),
(#50176,#50177,#50178,#50179,#50180,#50181,#50182,#50183,#50184,#50185,
#50186,#50187,#50188,#50189,#50190,#50191)),.UNSPECIFIED.,.F.,.F.,.F.)
B_SPLINE_SURFACE_WITH_KNOTS((4,4),(4,1,1,1,1,1,1,1,1,1,1,1,1,4),(0.0600759832204326,
0.9330208779252),(-0.009395290945745,0.,0.07535327170826,0.1579194084293,
0.2496878347776,0.3528404724363,0.4595208130962,0.5578799794614,0.6478320754105,
0.7283136662232,0.8001425287387,0.867942076904,0.9343337648423,0.9520744430431),
 .UNSPECIFIED.)
GEOMETRIC_REPRESENTATION_ITEM()
RATIONAL_B_SPLINE_SURFACE(((1.07758950128785,1.07758950128785,1.07758950128785,
1.07758950128785,1.07758950128785,1.07758950128785,1.07758950128785,1.07758950128785,
1.07758950128785,1.07758950128785,1.07758950128785,1.07758950128785,1.07758950128785,
1.07758950128785,1.07758950128785,1.07758950128785),(0.974948505042402,
0.974948505042402,0.974948505042402,0.974948505042402,0.974948505042402,
0.974948505042402,0.974948505042402,0.974948505042402,0.974948505042402,
0.974948505042402,0.974948505042402,0.974948505042402,0.974948505042402,
0.974948505042402,0.974948505042402,0.974948505042402),(0.974143201146493,
0.974143201146493,0.974143201146493,0.974143201146493,0.974143201146493,
0.974143201146493,0.974143201146493,0.974143201146493,0.974143201146493,
0.974143201146493,0.974143201146493,0.974143201146493,0.974143201146493,
0.974143201146493,0.974143201146493,0.974143201146493),(1.07517358960013,
1.07517358960013,1.07517358960013,1.07517358960013,1.07517358960013,1.07517358960013,
1.07517358960013,1.07517358960013,1.07517358960013,1.07517358960013,1.07517358960013,
1.07517358960013,1.07517358960013,1.07517358960013,1.07517358960013,1.07517358960013)))
REPRESENTATION_ITEM('')
SURFACE()
);
#450=(
BOUNDED_SURFACE()
B_SPLINE_SURFACE(3,3,((#50658,#50659,#50660,#50661,#50662,#50663,#50664,
#50665,#50666,#50667,#50668),(#50669,#50670,#50671,#50672,#50673,#50674,
#50675,#50676,#50677,#50678,#50679),(#50680,#50681,#50682,#50683,#50684,
#50685,#50686,#50687,#50688,#50689,#50690),(#50691,#50692,#50693,#50694,
#50695,#50696,#50697,#50698,#50699,#50700,#50701)),.UNSPECIFIED.,.F.,.F.,
 .F.)
B_SPLINE_SURFACE_WITH_KNOTS((4,4),(4,1,1,1,1,1,1,1,4),(0.0575632716498308,
0.953112794434742),(0.2692267298686,0.2759856699154,0.3429685143453,0.4189932536889,
0.4999153618947,0.580855541603,0.656922437546,0.7239458783794,0.7307829892477),
 .UNSPECIFIED.)
GEOMETRIC_REPRESENTATION_ITEM()
RATIONAL_B_SPLINE_SURFACE(((1.19946737217014,1.19946737217014,1.19946737217014,
1.19946737217014,1.19946737217014,1.19946737217014,1.19946737217014,1.19946737217014,
1.19946737217014,1.19946737217014,1.19946737217014),(0.930302090429665,
0.930302090429665,0.930302090429665,0.930302090429665,0.930302090429665,
0.930302090429665,0.930302090429665,0.930302090429665,0.930302090429665,
0.930302090429665,0.930302090429665),(0.933549590186578,0.933549590186578,
0.933549590186578,0.933549590186578,0.933549590186578,0.933549590186578,
0.933549590186578,0.933549590186578,0.933549590186578,0.933549590186578,
0.933549590186578),(1.20920987144088,1.20920987144088,1.20920987144088,
1.20920987144088,1.20920987144088,1.20920987144088,1.20920987144088,1.20920987144088,
1.20920987144088,1.20920987144088,1.20920987144088)))
REPRESENTATION_ITEM('')
SURFACE()
);
#451=(
BOUNDED_SURFACE()
B_SPLINE_SURFACE(3,3,((#50855,#50856,#50857,#50858,#50859,#50860,#50861,
#50862,#50863,#50864),(#50865,#50866,#50867,#50868,#50869,#50870,#50871,
#50872,#50873,#50874),(#50875,#50876,#50877,#50878,#50879,#50880,#50881,
#50882,#50883,#50884),(#50885,#50886,#50887,#50888,#50889,#50890,#50891,
#50892,#50893,#50894)),.UNSPECIFIED.,.F.,.F.,.F.)
B_SPLINE_SURFACE_WITH_KNOTS((4,4),(4,1,1,1,1,1,1,4),(0.0524368674708791,
0.9465986338923),(0.233245719424266,0.2759694154114,0.371008392869,0.4667717162199,
0.5596326028965,0.6452726458233,0.7220332580943,0.755043759390866),
 .UNSPECIFIED.)
GEOMETRIC_REPRESENTATION_ITEM()
RATIONAL_B_SPLINE_SURFACE(((1.20412390665185,1.20412390665185,1.20412390665185,
1.20412390665185,1.20412390665185,1.20412390665185,1.20412390665185,1.20412390665185,
1.20412390665185,1.20412390665185),(0.932251955821422,0.932251955821422,
0.932251955821421,0.932251955821422,0.932251955821422,0.932251955821422,
0.932251955821422,0.932251955821422,0.932251955821422,0.932251955821422),
(0.931959013768214,0.931959013768214,0.931959013768214,0.931959013768214,
0.931959013768214,0.931959013768214,0.931959013768214,0.931959013768214,
0.931959013768214,0.931959013768214),(1.20324508049223,1.20324508049223,
1.20324508049223,1.20324508049223,1.20324508049223,1.20324508049223,1.20324508049223,
1.20324508049223,1.20324508049223,1.20324508049223)))
REPRESENTATION_ITEM('')
SURFACE()
);
#452=(
BOUNDED_SURFACE()
B_SPLINE_SURFACE(3,3,((#51014,#51015,#51016,#51017,#51018,#51019,#51020,
#51021,#51022,#51023),(#51024,#51025,#51026,#51027,#51028,#51029,#51030,
#51031,#51032,#51033),(#51034,#51035,#51036,#51037,#51038,#51039,#51040,
#51041,#51042,#51043),(#51044,#51045,#51046,#51047,#51048,#51049,#51050,
#51051,#51052,#51053)),.UNSPECIFIED.,.F.,.F.,.F.)
B_SPLINE_SURFACE_WITH_KNOTS((4,4),(4,1,1,1,1,1,1,4),(0.0376044687776927,
0.9632701597044),(0.03308221537891,0.1426814398896,0.2856169915253,0.4287844228248,
0.5720769018248,0.7151865898555,0.857914409195,0.9460833470288),
 .UNSPECIFIED.)
GEOMETRIC_REPRESENTATION_ITEM()
RATIONAL_B_SPLINE_SURFACE(((1.13246860461612,1.13246860461612,1.13246860461612,
1.13246860461612,1.13246860461612,1.13246860461612,1.13246860461612,1.13246860461612,
1.13246860461612,1.13246860461612),(0.955676754150111,0.955676754150111,
0.955676754150111,0.955676754150111,0.955676754150111,0.955676754150111,
0.955676754150111,0.955676754150111,0.955676754150111,0.955676754150111),
(0.955843956444876,0.955843956444876,0.955843956444876,0.955843956444876,
0.955843956444876,0.955843956444876,0.955843956444876,0.955843956444876,
0.955843956444876,0.955843956444876),(1.13297021150041,1.13297021150041,
1.13297021150041,1.13297021150041,1.13297021150041,1.13297021150041,1.13297021150041,
1.13297021150041,1.13297021150041,1.13297021150041)))
REPRESENTATION_ITEM('')
SURFACE()
);
#453=(
BOUNDED_SURFACE()
B_SPLINE_SURFACE(3,3,((#51149,#51150,#51151,#51152,#51153,#51154,#51155,
#51156,#51157,#51158,#51159),(#51160,#51161,#51162,#51163,#51164,#51165,
#51166,#51167,#51168,#51169,#51170),(#51171,#51172,#51173,#51174,#51175,
#51176,#51177,#51178,#51179,#51180,#51181),(#51182,#51183,#51184,#51185,
#51186,#51187,#51188,#51189,#51190,#51191,#51192)),.UNSPECIFIED.,.F.,.F.,
 .F.)
B_SPLINE_SURFACE_WITH_KNOTS((4,4),(4,1,1,1,1,1,1,1,4),(0.0522071605228554,
0.949229841408476),(0.244546321466786,0.2921614493104,0.3746006374515,0.4619240874495,
0.5486822225607,0.6295887174107,0.7017044698897,0.765848500065,0.768100603477379),
 .UNSPECIFIED.)
GEOMETRIC_REPRESENTATION_ITEM()
RATIONAL_B_SPLINE_SURFACE(((1.20432661363983,1.20432661363983,1.20432661363983,
1.20432661363983,1.20432661363983,1.20432661363983,1.20432661363983,1.20432661363983,
1.20432661363983,1.20432661363983,1.20432661363983),(0.931453995492728,
0.931453995492728,0.931453995492728,0.931453995492728,0.931453995492728,
0.931453995492728,0.931453995492728,0.931453995492728,0.931453995492728,
0.931453995492728,0.931453995492728),(0.931891830184036,0.931891830184036,
0.931891830184036,0.931891830184036,0.931891830184036,0.931891830184036,
0.931891830184036,0.931891830184036,0.931891830184036,0.931891830184036,
0.931891830184036),(1.20564011771375,1.20564011771375,1.20564011771375,
1.20564011771375,1.20564011771375,1.20564011771375,1.20564011771375,1.20564011771375,
1.20564011771375,1.20564011771375,1.20564011771375)))
REPRESENTATION_ITEM('')
SURFACE()
);
#454=(
BOUNDED_SURFACE()
B_SPLINE_SURFACE(3,3,((#51289,#51290,#51291,#51292,#51293,#51294,#51295,
#51296,#51297,#51298),(#51299,#51300,#51301,#51302,#51303,#51304,#51305,
#51306,#51307,#51308),(#51309,#51310,#51311,#51312,#51313,#51314,#51315,
#51316,#51317,#51318),(#51319,#51320,#51321,#51322,#51323,#51324,#51325,
#51326,#51327,#51328)),.UNSPECIFIED.,.F.,.F.,.F.)
B_SPLINE_SURFACE_WITH_KNOTS((4,4),(4,1,1,1,1,1,1,4),(0.0418851650492697,
0.963268717220642),(0.05391635099551,0.1420855915678,0.2848134105773,0.4279230981834,
0.5712155769628,0.7143830082179,0.8573185600922,0.9669169090932),
 .UNSPECIFIED.)
GEOMETRIC_REPRESENTATION_ITEM()
RATIONAL_B_SPLINE_SURFACE(((1.13002726603044,1.13002726603044,1.13002726603044,
1.13002726603044,1.13002726603044,1.13002726603044,1.13002726603044,1.13002726603044,
1.13002726603044,1.13002726603044),(0.955682356393539,0.955682356393539,
0.955682356393539,0.955682356393539,0.955682356393539,0.955682356393539,
0.955682356393539,0.955682356393539,0.955682356393539,0.955682356393539),
(0.956663063707594,0.956663063707594,0.956663063707594,0.956663063707594,
0.956663063707594,0.956663063707594,0.956663063707594,0.956663063707594,
0.956663063707594,0.956663063707594),(1.13296938797261,1.13296938797261,
1.13296938797261,1.13296938797261,1.13296938797261,1.13296938797261,1.13296938797261,
1.13296938797261,1.13296938797261,1.13296938797261)))
REPRESENTATION_ITEM('')
SURFACE()
);
#455=(
BOUNDED_SURFACE()
B_SPLINE_SURFACE(3,3,((#51482,#51483,#51484,#51485,#51486,#51487),(#51488,
#51489,#51490,#51491,#51492,#51493),(#51494,#51495,#51496,#51497,#51498,
#51499),(#51500,#51501,#51502,#51503,#51504,#51505)),.UNSPECIFIED.,.F.,
 .F.,.F.)
B_SPLINE_SURFACE_WITH_KNOTS((4,4),(4,1,1,4),(0.0606070589527452,0.939490000441276),
(0.199119625235957,0.3331969354622,0.6668030645378,0.800880379917306),
 .UNSPECIFIED.)
GEOMETRIC_REPRESENTATION_ITEM()
RATIONAL_B_SPLINE_SURFACE(((1.1746901488214,1.1746901488214,1.1746901488214,
1.1746901488214,1.1746901488214,1.1746901488214),(0.941744225021468,0.941744225021468,
0.941744225021468,0.941744225021468,0.941744225021468,0.941744225021468),
(0.941769953234294,0.941769953234295,0.941769953234294,0.941769953234294,
0.941769953234294,0.941769953234294),(1.17476733345988,1.17476733345988,
1.17476733345988,1.17476733345988,1.17476733345988,1.17476733345988)))
REPRESENTATION_ITEM('')
SURFACE()
);
#456=(
BOUNDED_SURFACE()
B_SPLINE_SURFACE(3,3,((#51772,#51773,#51774,#51775,#51776,#51777,#51778,
#51779,#51780,#51781,#51782,#51783,#51784,#51785,#51786,#51787,#51788,#51789,
#51790,#51791),(#51792,#51793,#51794,#51795,#51796,#51797,#51798,#51799,
#51800,#51801,#51802,#51803,#51804,#51805,#51806,#51807,#51808,#51809,#51810,
#51811),(#51812,#51813,#51814,#51815,#51816,#51817,#51818,#51819,#51820,
#51821,#51822,#51823,#51824,#51825,#51826,#51827,#51828,#51829,#51830,#51831),
(#51832,#51833,#51834,#51835,#51836,#51837,#51838,#51839,#51840,#51841,
#51842,#51843,#51844,#51845,#51846,#51847,#51848,#51849,#51850,#51851)),
 .UNSPECIFIED.,.F.,.F.,.F.)
B_SPLINE_SURFACE_WITH_KNOTS((4,4),(4,1,1,1,1,1,1,1,1,1,1,1,1,1,1,1,1,4),
(0.0633076699555623,0.939196073758018),(-0.00915383127714,0.,0.07546659123987,
0.1557180876053,0.2404001363484,0.3291523816828,0.4125158427852,0.485675861971,
0.5506578767173,0.6094485282683,0.6638170257839,0.7128077767044,0.7565087359807,
0.7968449582086,0.8357677603499,0.8748879264935,0.9149300941034,0.92753194056),
 .UNSPECIFIED.)
GEOMETRIC_REPRESENTATION_ITEM()
RATIONAL_B_SPLINE_SURFACE(((1.07645082753394,1.07645082753394,1.07645082753394,
1.07645082753394,1.07645082753394,1.07645082753394,1.07645082753394,1.07645082753394,
1.07645082753394,1.07645082753394,1.07645082753394,1.07645082753394,1.07645082753394,
1.07645082753394,1.07645082753394,1.07645082753394,1.07645082753394,1.07645082753394,
1.07645082753394,1.07645082753394),(0.974224173982434,0.974224173982434,
0.974224173982434,0.974224173982434,0.974224173982434,0.974224173982434,
0.974224173982434,0.974224173982434,0.974224173982434,0.974224173982434,
0.974224173982434,0.974224173982434,0.974224173982434,0.974224173982434,
0.974224173982434,0.974224173982434,0.974224173982434,0.974224173982434,
0.974224173982434,0.974224173982434),(0.97451722852402,0.97451722852402,
0.97451722852402,0.97451722852402,0.97451722852402,0.97451722852402,0.97451722852402,
0.97451722852402,0.97451722852402,0.97451722852402,0.97451722852402,0.97451722852402,
0.97451722852402,0.97451722852402,0.97451722852402,0.97451722852402,0.97451722852402,
0.97451722852402,0.97451722852402,0.97451722852402),(1.07732999115869,1.07732999115869,
1.07732999115869,1.07732999115869,1.07732999115869,1.07732999115869,1.07732999115869,
1.07732999115869,1.07732999115869,1.07732999115869,1.07732999115869,1.07732999115869,
1.07732999115869,1.07732999115869,1.07732999115869,1.07732999115869,1.07732999115869,
1.07732999115869,1.07732999115869,1.07732999115869)))
REPRESENTATION_ITEM('')
SURFACE()
);
#457=(
BOUNDED_SURFACE()
B_SPLINE_SURFACE(3,3,((#52013,#52014,#52015,#52016,#52017,#52018,#52019,
#52020,#52021,#52022),(#52023,#52024,#52025,#52026,#52027,#52028,#52029,
#52030,#52031,#52032),(#52033,#52034,#52035,#52036,#52037,#52038,#52039,
#52040,#52041,#52042),(#52043,#52044,#52045,#52046,#52047,#52048,#52049,
#52050,#52051,#52052)),.UNSPECIFIED.,.F.,.F.,.F.)
B_SPLINE_SURFACE_WITH_KNOTS((4,4),(4,1,1,1,1,1,1,4),(0.0534066136803702,
0.94724602026267),(0.235043827368409,0.2946028323238,0.3657508320856,0.445876802538,
0.5324642225534,0.6203243693421,0.7038886951953,0.755256380853433),
 .UNSPECIFIED.)
GEOMETRIC_REPRESENTATION_ITEM()
RATIONAL_B_SPLINE_SURFACE(((1.20323901910316,1.20323901910316,1.20323901910316,
1.20323901910316,1.20323901910316,1.20323901910316,1.20323901910316,1.20323901910316,
1.20323901910316,1.20323901910316),(0.932055656646419,0.932055656646419,
0.932055656646419,0.932055656646419,0.932055656646419,0.932055656646419,
0.932055656646419,0.932055656646419,0.932055656646419,0.932055656646419),
(0.932253804976139,0.932253804976139,0.932253804976139,0.932253804976139,
0.932253804976139,0.932253804976139,0.932253804976139,0.932253804976139,
0.932253804976139,0.932253804976139),(1.20383346409232,1.20383346409232,
1.20383346409232,1.20383346409232,1.20383346409232,1.20383346409232,1.20383346409232,
1.20383346409232,1.20383346409232,1.20383346409232)))
REPRESENTATION_ITEM('')
SURFACE()
);
#458=(
BOUNDED_SURFACE()
B_SPLINE_SURFACE(3,3,((#52172,#52173,#52174,#52175,#52176,#52177,#52178,
#52179,#52180,#52181,#52182),(#52183,#52184,#52185,#52186,#52187,#52188,
#52189,#52190,#52191,#52192,#52193),(#52194,#52195,#52196,#52197,#52198,
#52199,#52200,#52201,#52202,#52203,#52204),(#52205,#52206,#52207,#52208,
#52209,#52210,#52211,#52212,#52213,#52214,#52215)),.UNSPECIFIED.,.F.,.F.,
 .F.)
B_SPLINE_SURFACE_WITH_KNOTS((4,4),(4,1,1,1,1,1,1,1,4),(0.0595062761581278,
0.935433221282967),(0.05105962729005,0.1243084941807,0.2492353165502,0.3744835129416,
0.4998949769261,0.6253220276845,0.7506164023093,0.8756120170229,0.9160299525995),
 .UNSPECIFIED.)
GEOMETRIC_REPRESENTATION_ITEM()
RATIONAL_B_SPLINE_SURFACE(((1.11958821674223,1.11958821674223,1.11958821674223,
1.11958821674223,1.11958821674223,1.11958821674223,1.11958821674223,1.11958821674223,
1.11958821674223,1.11958821674223,1.11958821674223),(0.961053167403458,
0.961053167403458,0.961053167403458,0.961053167403458,0.961053167403458,
0.961053167403458,0.961053167403458,0.961053167403458,0.961053167403458,
0.961053167403458,0.961053167403458),(0.960142522166725,0.960142522166725,
0.960142522166725,0.960142522166725,0.960142522166725,0.960142522166725,
0.960142522166725,0.960142522166725,0.960142522166725,0.960142522166725,
0.960142522166725),(1.11685628103203,1.11685628103203,1.11685628103203,
1.11685628103203,1.11685628103203,1.11685628103203,1.11685628103203,1.11685628103203,
1.11685628103203,1.11685628103203,1.11685628103203)))
REPRESENTATION_ITEM('')
SURFACE()
);
#459=(
BOUNDED_SURFACE()
B_SPLINE_SURFACE(3,3,((#52449,#52450,#52451,#52452,#52453,#52454,#52455,
#52456,#52457,#52458,#52459),(#52460,#52461,#52462,#52463,#52464,#52465,
#52466,#52467,#52468,#52469,#52470),(#52471,#52472,#52473,#52474,#52475,
#52476,#52477,#52478,#52479,#52480,#52481),(#52482,#52483,#52484,#52485,
#52486,#52487,#52488,#52489,#52490,#52491,#52492)),.UNSPECIFIED.,.F.,.F.,
 .F.)
B_SPLINE_SURFACE_WITH_KNOTS((4,4),(4,1,1,1,1,1,1,1,4),(0.0575588785903921,
0.953164053882501),(0.2692226783974,0.2757404474013,0.3428253937552,0.4189611174942,
0.4999467364448,0.5809436838552,0.6571062155613,0.7242167269719,0.7307666831887),
 .UNSPECIFIED.)
GEOMETRIC_REPRESENTATION_ITEM()
RATIONAL_B_SPLINE_SURFACE(((1.19947338866439,1.19947338866439,1.19947338866439,
1.19947338866439,1.19947338866439,1.19947338866439,1.19947338866439,1.19947338866439,
1.19947338866439,1.19947338866439,1.19947338866439),(0.93028593361712,0.93028593361712,
0.93028593361712,0.93028593361712,0.93028593361712,0.93028593361712,0.93028593361712,
0.93028593361712,0.93028593361712,0.93028593361712,0.93028593361712),(0.933547925736913,
0.933547925736913,0.933547925736913,0.933547925736913,0.933547925736913,
0.933547925736913,0.933547925736913,0.933547925736913,0.933547925736913,
0.933547925736913,0.933547925736913),(1.20925936502377,1.20925936502377,
1.20925936502377,1.20925936502377,1.20925936502377,1.20925936502377,1.20925936502377,
1.20925936502377,1.20925936502377,1.20925936502377,1.20925936502377)))
REPRESENTATION_ITEM('')
SURFACE()
);
#460=(
BOUNDED_SURFACE()
B_SPLINE_SURFACE(3,3,((#52578,#52579,#52580,#52581,#52582,#52583,#52584,
#52585,#52586,#52587),(#52588,#52589,#52590,#52591,#52592,#52593,#52594,
#52595,#52596,#52597),(#52598,#52599,#52600,#52601,#52602,#52603,#52604,
#52605,#52606,#52607),(#52608,#52609,#52610,#52611,#52612,#52613,#52614,
#52615,#52616,#52617)),.UNSPECIFIED.,.F.,.F.,.F.)
B_SPLINE_SURFACE_WITH_KNOTS((4,4),(4,1,1,1,1,1,1,4),(0.0479830627277209,
0.946593353629165),(0.239518392063012,0.2430457920758,0.3242077589869,0.4151597383417,
0.5128629145943,0.6131453701819,0.7126591855993,0.770045878654716),
 .UNSPECIFIED.)
GEOMETRIC_REPRESENTATION_ITEM()
RATIONAL_B_SPLINE_SURFACE(((1.20821093302208,1.20821093302208,1.20821093302208,
1.20821093302208,1.20821093302208,1.20821093302208,1.20821093302208,1.20821093302208,
1.20821093302208,1.20821093302208),(0.932261852852764,0.932261852852764,
0.932261852852764,0.932261852852764,0.932261852852764,0.932261852852764,
0.932261852852764,0.932261852852764,0.932261852852764,0.932261852852764),
(0.93060634750094,0.93060634750094,0.93060634750094,0.93060634750094,0.93060634750094,
0.93060634750094,0.93060634750094,0.93060634750094,0.93060634750094,0.93060634750094),
(1.20324441696661,1.20324441696661,1.20324441696661,1.20324441696661,1.20324441696661,
1.20324441696661,1.20324441696661,1.20324441696661,1.20324441696661,1.20324441696661)))
REPRESENTATION_ITEM('')
SURFACE()
);
#461=(
BOUNDED_SURFACE()
B_SPLINE_SURFACE(3,3,((#52768,#52769,#52770,#52771,#52772,#52773,#52774,
#52775,#52776,#52777,#52778),(#52779,#52780,#52781,#52782,#52783,#52784,
#52785,#52786,#52787,#52788,#52789),(#52790,#52791,#52792,#52793,#52794,
#52795,#52796,#52797,#52798,#52799,#52800),(#52801,#52802,#52803,#52804,
#52805,#52806,#52807,#52808,#52809,#52810,#52811)),.UNSPECIFIED.,.F.,.F.,
 .F.)
B_SPLINE_SURFACE_WITH_KNOTS((4,4),(4,1,1,1,1,1,1,1,4),(0.0434902481459629,
0.937490443608701),(-0.009351371213944,0.,0.1428545029,0.2856984060337,
0.4287781897902,0.5720429752755,0.7151346717899,0.857843506892,0.9437353739471),
 .UNSPECIFIED.)
GEOMETRIC_REPRESENTATION_ITEM()
RATIONAL_B_SPLINE_SURFACE(((1.128442539186,1.128442539186,1.128442539186,
1.128442539186,1.128442539186,1.128442539186,1.128442539186,1.128442539186,
1.128442539186,1.128442539186,1.128442539186),(0.960753306302974,0.960753306302974,
0.960753306302974,0.960753306302974,0.960753306302974,0.960753306302974,
0.960753306302974,0.960753306302974,0.960753306302974,0.960753306302974,
0.960753306302974),(0.957260135350247,0.957260135350247,0.957260135350247,
0.957260135350247,0.957260135350247,0.957260135350247,0.957260135350247,
0.957260135350247,0.957260135350247,0.957260135350247,0.957260135350247),
(1.11796302632782,1.11796302632782,1.11796302632782,1.11796302632782,1.11796302632782,
1.11796302632782,1.11796302632782,1.11796302632782,1.11796302632782,1.11796302632782,
1.11796302632782)))
REPRESENTATION_ITEM('')
SURFACE()
);
#462=(
BOUNDED_SURFACE()
B_SPLINE_SURFACE(3,3,((#52961,#52962,#52963,#52964,#52965,#52966),(#52967,
#52968,#52969,#52970,#52971,#52972),(#52973,#52974,#52975,#52976,#52977,
#52978),(#52979,#52980,#52981,#52982,#52983,#52984)),.UNSPECIFIED.,.F.,
 .F.,.F.)
B_SPLINE_SURFACE_WITH_KNOTS((4,4),(4,1,1,4),(0.0606720801571754,0.938680242177121),
(-1.E-5,0.,0.3336142546261,0.663356363362649),.UNSPECIFIED.)
GEOMETRIC_REPRESENTATION_ITEM()
RATIONAL_B_SPLINE_SURFACE(((1.17463054351816,1.17463054351816,1.17463054351816,
1.17463054351816,1.17463054351816,1.17463054351816),(0.941961451143807,
0.941961451143807,0.941961451143807,0.941961451143807,0.941961451143807,
0.941961451143807),(0.941789945341621,0.941789945341621,0.941789945341621,
0.941789945341621,0.941789945341621,0.941789945341621),(1.1741160261116,
1.1741160261116,1.1741160261116,1.1741160261116,1.1741160261116,1.1741160261116)))
REPRESENTATION_ITEM('')
SURFACE()
);
#463=(
BOUNDED_SURFACE()
B_SPLINE_SURFACE(3,3,((#52994,#52995,#52996,#52997,#52998,#52999,#53000,
#53001,#53002,#53003,#53004,#53005,#53006,#53007,#53008,#53009),(#53010,
#53011,#53012,#53013,#53014,#53015,#53016,#53017,#53018,#53019,#53020,#53021,
#53022,#53023,#53024,#53025),(#53026,#53027,#53028,#53029,#53030,#53031,
#53032,#53033,#53034,#53035,#53036,#53037,#53038,#53039,#53040,#53041),
(#53042,#53043,#53044,#53045,#53046,#53047,#53048,#53049,#53050,#53051,
#53052,#53053,#53054,#53055,#53056,#53057)),.UNSPECIFIED.,.F.,.F.,.F.)
B_SPLINE_SURFACE_WITH_KNOTS((4,4),(4,1,1,1,1,1,1,1,1,1,1,1,1,4),(0.0607615083810939,
0.93302086581287),(-0.009395290942738,0.,0.0753533259589,0.1579195464055,
0.2496880158193,0.352840403202,0.4595197316146,0.5578787401128,0.6478313181872,
0.7283133787206,0.8001424242299,0.867942029368,0.9343337419824,0.9520744430681),
 .UNSPECIFIED.)
GEOMETRIC_REPRESENTATION_ITEM()
RATIONAL_B_SPLINE_SURFACE(((1.07734787781885,1.07734787781885,1.07734787781885,
1.07734787781885,1.07734787781885,1.07734787781885,1.07734787781885,1.07734787781885,
1.07734787781885,1.07734787781885,1.07734787781885,1.07734787781885,1.07734787781885,
1.07734787781885,1.07734787781885,1.07734787781885),(0.974947304262177,
0.974947304262177,0.974947304262177,0.974947304262177,0.974947304262177,
0.974947304262177,0.974947304262177,0.974947304262177,0.974947304262177,
0.974947304262177,0.974947304262177,0.974947304262177,0.974947304262177,
0.974947304262177,0.974947304262177,0.974947304262177),(0.974222540311786,
0.974222540311786,0.974222540311786,0.974222540311786,0.974222540311786,
0.974222540311786,0.974222540311786,0.974222540311786,0.974222540311786,
0.974222540311786,0.974222540311786,0.974222540311786,0.974222540311786,
0.974222540311786,0.974222540311786,0.974222540311786),(1.07517358596768,
1.07517358596768,1.07517358596768,1.07517358596768,1.07517358596768,1.07517358596768,
1.07517358596768,1.07517358596768,1.07517358596768,1.07517358596768,1.07517358596768,
1.07517358596768,1.07517358596768,1.07517358596768,1.07517358596768,1.07517358596768)))
REPRESENTATION_ITEM('')
SURFACE()
);
#464=(
BOUNDED_SURFACE()
B_SPLINE_SURFACE(3,3,((#53524,#53525,#53526,#53527,#53528,#53529,#53530,
#53531,#53532),(#53533,#53534,#53535,#53536,#53537,#53538,#53539,#53540,
#53541),(#53542,#53543,#53544,#53545,#53546,#53547,#53548,#53549,#53550),
(#53551,#53552,#53553,#53554,#53555,#53556,#53557,#53558,#53559)),
 .UNSPECIFIED.,.F.,.F.,.F.)
B_SPLINE_SURFACE_WITH_KNOTS((4,4),(4,1,1,1,1,1,4),(0.0580455652775177,0.958569362546839),
(0.2691839560331,0.3316611066132,0.4169070356234,0.499999867704,0.5830925415824,
0.6683381194025,0.7308257034814),.UNSPECIFIED.)
GEOMETRIC_REPRESENTATION_ITEM()
RATIONAL_B_SPLINE_SURFACE(((1.19903368051256,1.19903368051256,1.19903368051256,
1.19903368051256,1.19903368051256,1.19903368051256,1.19903368051256,1.19903368051256,
1.19903368051256),(0.928667097175851,0.928667097175851,0.928667097175851,
0.928667097175851,0.928667097175851,0.928667097175851,0.928667097175851,
0.928667097175851,0.928667097175851),(0.933749206229783,0.933749206229783,
0.933749206229783,0.933749206229783,0.933749206229783,0.933749206229783,
0.933749206229783,0.933749206229783,0.933749206229783),(1.21428000767435,
1.21428000767435,1.21428000767435,1.21428000767435,1.21428000767435,1.21428000767435,
1.21428000767435,1.21428000767435,1.21428000767435)))
REPRESENTATION_ITEM('')
SURFACE()
);
#465=(
BOUNDED_SURFACE()
B_SPLINE_SURFACE(3,3,((#53644,#53645,#53646,#53647,#53648,#53649,#53650,
#53651,#53652),(#53653,#53654,#53655,#53656,#53657,#53658,#53659,#53660,
#53661),(#53662,#53663,#53664,#53665,#53666,#53667,#53668,#53669,#53670),
(#53671,#53672,#53673,#53674,#53675,#53676,#53677,#53678,#53679)),
 .UNSPECIFIED.,.F.,.F.,.F.)
B_SPLINE_SURFACE_WITH_KNOTS((4,4),(4,1,1,1,1,1,4),(0.0491576255108182,0.946591020356229),
(0.22996558030876,0.2892821395991,0.3893944830893,0.4899684829189,0.5875628832777,
0.6780458245647,0.758314180295999),.UNSPECIFIED.)
GEOMETRIC_REPRESENTATION_ITEM()
RATIONAL_B_SPLINE_SURFACE(((1.20712810928682,1.20712810928682,1.20712810928682,
1.20712810928682,1.20712810928682,1.20712810928682,1.20712810928682,1.20712810928682,
1.20712810928682),(0.932259414885021,0.932259414885021,0.932259414885021,
0.932259414885021,0.932259414885021,0.932259414885021,0.932259414885021,
0.932259414885021,0.932259414885021),(0.930963436261351,0.930963436261351,
0.930963436261351,0.930963436261351,0.930963436261351,0.930963436261351,
0.930963436261351,0.930963436261351,0.930963436261351),(1.20324017341582,
1.20324017341582,1.20324017341582,1.20324017341582,1.20324017341582,1.20324017341582,
1.20324017341582,1.20324017341582,1.20324017341582)))
REPRESENTATION_ITEM('')
SURFACE()
);
#466=(
BOUNDED_SURFACE()
B_SPLINE_SURFACE(3,3,((#53796,#53797,#53798,#53799,#53800,#53801,#53802,
#53803,#53804,#53805),(#53806,#53807,#53808,#53809,#53810,#53811,#53812,
#53813,#53814,#53815),(#53816,#53817,#53818,#53819,#53820,#53821,#53822,
#53823,#53824,#53825),(#53826,#53827,#53828,#53829,#53830,#53831,#53832,
#53833,#53834,#53835)),.UNSPECIFIED.,.F.,.F.,.F.)
B_SPLINE_SURFACE_WITH_KNOTS((4,4),(4,1,1,1,1,1,1,4),(0.0418800048973985,
0.963270228783426),(0.03308221537886,0.1426814397772,0.2856169899415,0.4287844215146,
0.5720769018753,0.7151865925248,0.8579144138988,0.9460833470307),
 .UNSPECIFIED.)
GEOMETRIC_REPRESENTATION_ITEM()
RATIONAL_B_SPLINE_SURFACE(((1.1300301908407,1.1300301908407,1.1300301908407,
1.1300301908407,1.1300301908407,1.1300301908407,1.1300301908407,1.1300301908407,
1.1300301908407,1.1300301908407),(0.955682060901635,0.955682060901635,0.955682060901635,
0.955682060901635,0.955682060901635,0.955682060901635,0.955682060901635,
0.955682060901635,0.955682060901635,0.955682060901635),(0.956662081006193,
0.956662081006193,0.956662081006193,0.956662081006193,0.956662081006193,
0.956662081006193,0.956662081006193,0.956662081006193,0.956662081006193,
0.956662081006193),(1.13297025115438,1.13297025115438,1.13297025115438,
1.13297025115438,1.13297025115438,1.13297025115438,1.13297025115438,1.13297025115438,
1.13297025115438,1.13297025115438)))
REPRESENTATION_ITEM('')
SURFACE()
);
#467=(
BOUNDED_SURFACE()
B_SPLINE_SURFACE(3,3,((#53931,#53932,#53933,#53934,#53935,#53936,#53937,
#53938,#53939,#53940),(#53941,#53942,#53943,#53944,#53945,#53946,#53947,
#53948,#53949,#53950),(#53951,#53952,#53953,#53954,#53955,#53956,#53957,
#53958,#53959,#53960),(#53961,#53962,#53963,#53964,#53965,#53966,#53967,
#53968,#53969,#53970)),.UNSPECIFIED.,.F.,.F.,.F.)
B_SPLINE_SURFACE_WITH_KNOTS((4,4),(4,1,1,1,1,1,1,4),(0.0438856011091739,
0.946597267382723),(0.236379435895912,0.2520150267493,0.335933433698,0.4293648728823,
0.5272993584536,0.6257010423672,0.7220735755741,0.775269513209664),
 .UNSPECIFIED.)
GEOMETRIC_REPRESENTATION_ITEM()
RATIONAL_B_SPLINE_SURFACE(((1.21199876592565,1.21199876592565,1.21199876592565,
1.21199876592565,1.21199876592565,1.21199876592565,1.21199876592565,1.21199876592565,
1.21199876592565,1.21199876592565),(0.932282741901863,0.932282741901864,
0.932282741901864,0.932282741901864,0.932282741901864,0.932282741901864,
0.932282741901864,0.932282741901864,0.932282741901864,0.932282741901864),
(0.929364511089559,0.929364511089559,0.929364511089559,0.929364511089559,
0.929364511089559,0.929364511089559,0.929364511089559,0.929364511089559,
0.929364511089559,0.929364511089559),(1.20324407348874,1.20324407348874,
1.20324407348874,1.20324407348874,1.20324407348874,1.20324407348874,1.20324407348874,
1.20324407348874,1.20324407348874,1.20324407348874)))
REPRESENTATION_ITEM('')
SURFACE()
);
#468=(
BOUNDED_SURFACE()
B_SPLINE_SURFACE(3,3,((#54150,#54151,#54152,#54153,#54154,#54155,#54156,
#54157,#54158,#54159),(#54160,#54161,#54162,#54163,#54164,#54165,#54166,
#54167,#54168,#54169),(#54170,#54171,#54172,#54173,#54174,#54175,#54176,
#54177,#54178,#54179),(#54180,#54181,#54182,#54183,#54184,#54185,#54186,
#54187,#54188,#54189)),.UNSPECIFIED.,.F.,.F.,.F.)
B_SPLINE_SURFACE_WITH_KNOTS((4,4),(4,1,1,1,1,1,1,4),(0.0418844974680166,
0.963268781581434),(0.05391635099617,0.1420855946084,0.2848134123028,0.427923098216,
0.5712155761158,0.714383007194,0.8573185600195,0.9669169090932),
 .UNSPECIFIED.)
GEOMETRIC_REPRESENTATION_ITEM()
RATIONAL_B_SPLINE_SURFACE(((1.13002764499145,1.13002764499145,1.13002764499145,
1.13002764499145,1.13002764499145,1.13002764499145,1.13002764499145,1.13002764499145,
1.13002764499145,1.13002764499145),(0.955682342794086,0.955682342794086,
0.955682342794086,0.955682342794086,0.955682342794086,0.955682342794086,
0.955682342794086,0.955682342794086,0.955682342794086,0.955682342794086),
(0.956662936103217,0.956662936103217,0.956662936103217,0.956662936103217,
0.956662936103217,0.956662936103217,0.956662936103217,0.956662936103217,
0.956662936103217,0.956662936103217),(1.13296942491884,1.13296942491884,
1.13296942491884,1.13296942491884,1.13296942491884,1.13296942491884,1.13296942491884,
1.13296942491884,1.13296942491884,1.13296942491884)))
REPRESENTATION_ITEM('')
SURFACE()
);
#469=(
BOUNDED_SURFACE()
B_SPLINE_SURFACE(3,3,((#54343,#54344,#54345,#54346,#54347,#54348),(#54349,
#54350,#54351,#54352,#54353,#54354),(#54355,#54356,#54357,#54358,#54359,
#54360),(#54361,#54362,#54363,#54364,#54365,#54366)),.UNSPECIFIED.,.F.,
 .F.,.F.)
B_SPLINE_SURFACE_WITH_KNOTS((4,4),(4,1,1,4),(0.060607058952475,0.939489995743308),
(0.199119631433838,0.3331969354622,0.6668030645378,0.800880373770273),
 .UNSPECIFIED.)
GEOMETRIC_REPRESENTATION_ITEM()
RATIONAL_B_SPLINE_SURFACE(((1.17469014882161,1.17469014882161,1.17469014882161,
1.17469014882161,1.17469014882161,1.17469014882161),(0.941744226266654,
0.941744226266654,0.941744226266654,0.941744226266654,0.941744226266654,
0.941744226266654),(0.941769953233949,0.941769953233949,0.941769953233949,
0.941769953233949,0.941769953233949,0.941769953233949),(1.1747673297235,
1.1747673297235,1.1747673297235,1.1747673297235,1.1747673297235,1.1747673297235)))
REPRESENTATION_ITEM('')
SURFACE()
);
#470=(
BOUNDED_SURFACE()
B_SPLINE_SURFACE(3,3,((#54633,#54634,#54635,#54636,#54637,#54638,#54639,
#54640,#54641,#54642,#54643,#54644,#54645,#54646,#54647,#54648,#54649,#54650,
#54651,#54652),(#54653,#54654,#54655,#54656,#54657,#54658,#54659,#54660,
#54661,#54662,#54663,#54664,#54665,#54666,#54667,#54668,#54669,#54670,#54671,
#54672),(#54673,#54674,#54675,#54676,#54677,#54678,#54679,#54680,#54681,
#54682,#54683,#54684,#54685,#54686,#54687,#54688,#54689,#54690,#54691,#54692),
(#54693,#54694,#54695,#54696,#54697,#54698,#54699,#54700,#54701,#54702,
#54703,#54704,#54705,#54706,#54707,#54708,#54709,#54710,#54711,#54712)),
 .UNSPECIFIED.,.F.,.F.,.F.)
B_SPLINE_SURFACE_WITH_KNOTS((4,4),(4,1,1,1,1,1,1,1,1,1,1,1,1,1,1,1,1,4),
(0.0633076649181857,0.9392002877331),(-0.0091538312793,0.,0.07546639963989,
0.1557177906993,0.2403998675743,0.3291523205441,0.4125160476047,0.4856762677964,
0.5506584357867,0.6094492100254,0.6638177940728,0.7128085155366,0.7565093937176,
0.7968455102028,0.8357682044765,0.8748882668515,0.9149303281208,0.9275319405255),
 .UNSPECIFIED.)
GEOMETRIC_REPRESENTATION_ITEM()
RATIONAL_B_SPLINE_SURFACE(((1.07645082929997,1.07645082929997,1.07645082929997,
1.07645082929997,1.07645082929997,1.07645082929997,1.07645082929997,1.07645082929997,
1.07645082929997,1.07645082929997,1.07645082929997,1.07645082929997,1.07645082929997,
1.07645082929997,1.07645082929997,1.07645082929997,1.07645082929997,1.07645082929997,
1.07645082929997,1.07645082929997),(0.974223682156895,0.974223682156895,
0.974223682156895,0.974223682156895,0.974223682156895,0.974223682156895,
0.974223682156895,0.974223682156895,0.974223682156895,0.974223682156895,
0.974223682156895,0.974223682156895,0.974223682156895,0.974223682156895,
0.974223682156895,0.974223682156895,0.974223682156895,0.974223682156895,
0.974223682156895,0.974223682156895),(0.974517230754059,0.974517230754059,
0.974517230754059,0.974517230754059,0.974517230754059,0.974517230754059,
0.974517230754059,0.974517230754059,0.974517230754059,0.974517230754059,
0.974517230754059,0.974517230754059,0.974517230754059,0.974517230754059,
0.974517230754059,0.974517230754059,0.974517230754059,0.974517230754059,
0.974517230754059,0.974517230754059),(1.07733147509147,1.07733147509147,
1.07733147509147,1.07733147509147,1.07733147509147,1.07733147509147,1.07733147509147,
1.07733147509147,1.07733147509147,1.07733147509147,1.07733147509147,1.07733147509147,
1.07733147509147,1.07733147509147,1.07733147509147,1.07733147509147,1.07733147509147,
1.07733147509147,1.07733147509147,1.07733147509147)))
REPRESENTATION_ITEM('')
SURFACE()
);
#471=(
BOUNDED_SURFACE()
B_SPLINE_SURFACE(3,3,((#54874,#54875,#54876,#54877,#54878,#54879,#54880,
#54881,#54882,#54883),(#54884,#54885,#54886,#54887,#54888,#54889,#54890,
#54891,#54892,#54893),(#54894,#54895,#54896,#54897,#54898,#54899,#54900,
#54901,#54902,#54903),(#54904,#54905,#54906,#54907,#54908,#54909,#54910,
#54911,#54912,#54913)),.UNSPECIFIED.,.F.,.F.,.F.)
B_SPLINE_SURFACE_WITH_KNOTS((4,4),(4,1,1,1,1,1,1,4),(0.0471532343849083,
0.946601707615917),(0.229158000328599,0.2767714735063,0.372769960558,0.470949598223,
0.568892608243,0.662583621586,0.7468957137446,0.761354885822289),
 .UNSPECIFIED.)
GEOMETRIC_REPRESENTATION_ITEM()
RATIONAL_B_SPLINE_SURFACE(((1.20897622394021,1.20897622394021,1.20897622394021,
1.20897622394021,1.20897622394021,1.20897622394021,1.20897622394021,1.20897622394021,
1.20897622394021,1.20897622394021),(0.932262539405233,0.932262539405233,
0.932262539405233,0.932262539405233,0.932262539405233,0.932262539405233,
0.932262539405233,0.932262539405233,0.932262539405233,0.932262539405233),
(0.930354506555822,0.930354506555822,0.930354506555822,0.930354506555822,
0.930354506555822,0.930354506555822,0.930354506555822,0.930354506555822,
0.930354506555822,0.930354506555822),(1.20325212539198,1.20325212539198,
1.20325212539198,1.20325212539198,1.20325212539198,1.20325212539198,1.20325212539198,
1.20325212539198,1.20325212539198,1.20325212539198)))
REPRESENTATION_ITEM('')
SURFACE()
);
#472=(
BOUNDED_SURFACE()
B_SPLINE_SURFACE(3,3,((#55105,#55106,#55107,#55108,#55109,#55110,#55111,
#55112,#55113,#55114,#55115),(#55116,#55117,#55118,#55119,#55120,#55121,
#55122,#55123,#55124,#55125,#55126),(#55127,#55128,#55129,#55130,#55131,
#55132,#55133,#55134,#55135,#55136,#55137),(#55138,#55139,#55140,#55141,
#55142,#55143,#55144,#55145,#55146,#55147,#55148)),.UNSPECIFIED.,.F.,.F.,
 .F.)
B_SPLINE_SURFACE_WITH_KNOTS((4,4),(4,1,1,1,1,1,1,1,4),(0.059506601274082,
0.936820242954807),(0.05105962729005,0.1243084941807,0.2492353165502,0.3744835129416,
0.4998949769261,0.6253220276845,0.7506164023093,0.8756120170229,0.9160299525995),
 .UNSPECIFIED.)
GEOMETRIC_REPRESENTATION_ITEM()
RATIONAL_B_SPLINE_SURFACE(((1.11958804019898,1.11958804019898,1.11958804019898,
1.11958804019898,1.11958804019898,1.11958804019898,1.11958804019898,1.11958804019898,
1.11958804019898,1.11958804019898,1.11958804019898),(0.960802128231612,
0.960802128231612,0.960802128231612,0.960802128231612,0.960802128231612,
0.960802128231612,0.960802128231612,0.960802128231612,0.960802128231612,
0.960802128231612,0.960802128231612),(0.960140091762279,0.960140091762279,
0.960140091762279,0.960140091762279,0.960140091762279,0.960140091762279,
0.960140091762279,0.960140091762279,0.960140091762279,0.960140091762279,
0.960140091762279),(1.11760193079098,1.11760193079098,1.11760193079098,
1.11760193079098,1.11760193079098,1.11760193079098,1.11760193079098,1.11760193079098,
1.11760193079098,1.11760193079098,1.11760193079098)))
REPRESENTATION_ITEM('')
SURFACE()
);
#473=(
BOUNDED_SURFACE()
B_SPLINE_SURFACE(3,3,((#55382,#55383,#55384,#55385,#55386,#55387,#55388,
#55389,#55390,#55391,#55392),(#55393,#55394,#55395,#55396,#55397,#55398,
#55399,#55400,#55401,#55402,#55403),(#55404,#55405,#55406,#55407,#55408,
#55409,#55410,#55411,#55412,#55413,#55414),(#55415,#55416,#55417,#55418,
#55419,#55420,#55421,#55422,#55423,#55424,#55425)),.UNSPECIFIED.,.F.,.F.,
 .F.)
B_SPLINE_SURFACE_WITH_KNOTS((4,4),(4,1,1,1,1,1,1,1,4),(0.0556357165437915,
0.955304109070403),(0.2692123318637,0.2896670261853,0.3517274755791,0.422380333238,
0.5000250192074,0.5776669090115,0.6483133938419,0.7103683419862,0.730777134988),
 .UNSPECIFIED.)
GEOMETRIC_REPRESENTATION_ITEM()
RATIONAL_B_SPLINE_SURFACE(((1.20121075267841,1.20121075267841,1.20121075267841,
1.20121075267841,1.20121075267841,1.20121075267841,1.20121075267841,1.20121075267841,
1.20121075267841,1.20121075267841,1.20121075267841),(0.929627337657785,
0.929627337657785,0.929627337657785,0.929627337657785,0.929627337657785,
0.929627337657785,0.929627337657785,0.929627337657785,0.929627337657785,
0.929627337657785,0.929627337657785),(0.93297040022002,0.93297040022002,
0.93297040022002,0.93297040022002,0.93297040022002,0.93297040022002,0.93297040022002,
0.93297040022002,0.93297040022002,0.93297040022002,0.93297040022002),(1.21123994036511,
1.21123994036511,1.21123994036511,1.21123994036511,1.21123994036511,1.21123994036511,
1.21123994036511,1.21123994036511,1.21123994036511,1.21123994036511,1.21123994036511)))
REPRESENTATION_ITEM('')
SURFACE()
);
#474=(
BOUNDED_SURFACE()
B_SPLINE_SURFACE(3,3,((#55517,#55518,#55519,#55520,#55521,#55522,#55523,
#55524,#55525),(#55526,#55527,#55528,#55529,#55530,#55531,#55532,#55533,
#55534),(#55535,#55536,#55537,#55538,#55539,#55540,#55541,#55542,#55543),
(#55544,#55545,#55546,#55547,#55548,#55549,#55550,#55551,#55552)),
 .UNSPECIFIED.,.F.,.F.,.F.)
B_SPLINE_SURFACE_WITH_KNOTS((4,4),(4,1,1,1,1,1,4),(0.053271791488534,0.946598328512929),
(0.244689773436238,0.3238159337994,0.4243565900039,0.5246117495307,0.6233178136293,
0.720247333279,0.764677618064232),.UNSPECIFIED.)
GEOMETRIC_REPRESENTATION_ITEM()
RATIONAL_B_SPLINE_SURFACE(((1.20336592416562,1.20336592416562,1.20336592416562,
1.20336592416562,1.20336592416562,1.20336592416562,1.20336592416562,1.20336592416562,
1.20336592416562),(0.9322507758164,0.932250775816401,0.9322507758164,0.932250775816401,
0.932250775816401,0.932250775816401,0.932250775816401,0.932250775816401,
0.9322507758164),(0.932211364341593,0.932211364341593,0.932211364341593,
0.932211364341593,0.932211364341593,0.932211364341593,0.932211364341593,
0.932211364341593,0.932211364341593),(1.2032476897412,1.2032476897412,1.2032476897412,
1.2032476897412,1.2032476897412,1.2032476897412,1.2032476897412,1.2032476897412,
1.2032476897412)))
REPRESENTATION_ITEM('')
SURFACE()
);
#475=(
BOUNDED_SURFACE()
B_SPLINE_SURFACE(3,3,((#55689,#55690,#55691,#55692,#55693,#55694,#55695,
#55696,#55697,#55698,#55699),(#55700,#55701,#55702,#55703,#55704,#55705,
#55706,#55707,#55708,#55709,#55710),(#55711,#55712,#55713,#55714,#55715,
#55716,#55717,#55718,#55719,#55720,#55721),(#55722,#55723,#55724,#55725,
#55726,#55727,#55728,#55729,#55730,#55731,#55732)),.UNSPECIFIED.,.F.,.F.,
 .F.)
B_SPLINE_SURFACE_WITH_KNOTS((4,4),(4,1,1,1,1,1,1,1,4),(0.0422678684933725,
0.937007437303486),(-0.009351371213946,0.,0.1428545029,0.2856984060337,
0.4287781897902,0.5720429752755,0.7151346717899,0.857843506892,0.9437353739471),
 .UNSPECIFIED.)
GEOMETRIC_REPRESENTATION_ITEM()
RATIONAL_B_SPLINE_SURFACE(((1.12913131189582,1.12913131189582,1.12913131189582,
1.12913131189582,1.12913131189582,1.12913131189582,1.12913131189582,1.12913131189582,
1.12913131189582,1.12913131189582,1.12913131189582),(0.960854006789805,
0.960854006789805,0.960854006789805,0.960854006789805,0.960854006789805,
0.960854006789805,0.960854006789805,0.960854006789805,0.960854006789805,
0.960854006789805,0.960854006789805),(0.957044469016947,0.957044469016947,
0.957044469016947,0.957044469016947,0.957044469016947,0.957044469016947,
0.957044469016947,0.957044469016947,0.957044469016947,0.957044469016947,
0.957044469016947),(1.11770269857725,1.11770269857725,1.11770269857725,
1.11770269857725,1.11770269857725,1.11770269857725,1.11770269857725,1.11770269857725,
1.11770269857725,1.11770269857725,1.11770269857725)))
REPRESENTATION_ITEM('')
SURFACE()
);
#476=(
BOUNDED_SURFACE()
B_SPLINE_SURFACE(3,3,((#55882,#55883,#55884,#55885,#55886,#55887),(#55888,
#55889,#55890,#55891,#55892,#55893),(#55894,#55895,#55896,#55897,#55898,
#55899),(#55900,#55901,#55902,#55903,#55904,#55905)),.UNSPECIFIED.,.F.,
 .F.,.F.)
B_SPLINE_SURFACE_WITH_KNOTS((4,4),(4,1,1,4),(0.0606720801614013,0.938680242176577),
(-1.E-5,0.,0.333614254626,0.663356363361679),.UNSPECIFIED.)
GEOMETRIC_REPRESENTATION_ITEM()
RATIONAL_B_SPLINE_SURFACE(((1.1746305435148,1.1746305435148,1.1746305435148,
1.1746305435148,1.1746305435148,1.1746305435148),(0.941961451143949,0.941961451143949,
0.941961451143949,0.941961451143949,0.941961451143949,0.941961451143949),
(0.941789945342739,0.941789945342739,0.941789945342739,0.941789945342739,
0.941789945342739,0.941789945342739),(1.17411602611117,1.17411602611117,
1.17411602611117,1.17411602611117,1.17411602611117,1.17411602611117)))
REPRESENTATION_ITEM('')
SURFACE()
);
#477=(
BOUNDED_SURFACE()
B_SPLINE_SURFACE(3,3,((#55915,#55916,#55917,#55918,#55919,#55920,#55921,
#55922,#55923,#55924,#55925,#55926,#55927,#55928,#55929,#55930),(#55931,
#55932,#55933,#55934,#55935,#55936,#55937,#55938,#55939,#55940,#55941,#55942,
#55943,#55944,#55945,#55946),(#55947,#55948,#55949,#55950,#55951,#55952,
#55953,#55954,#55955,#55956,#55957,#55958,#55959,#55960,#55961,#55962),
(#55963,#55964,#55965,#55966,#55967,#55968,#55969,#55970,#55971,#55972,
#55973,#55974,#55975,#55976,#55977,#55978)),.UNSPECIFIED.,.F.,.F.,.F.)
B_SPLINE_SURFACE_WITH_KNOTS((4,4),(4,1,1,1,1,1,1,1,1,1,1,1,1,4),(0.060761509047659,
0.933020866626784),(-0.009395290942739,0.,0.07535332595895,0.1579195464056,
0.2496880158195,0.3528404032023,0.4595197316149,0.5578787401132,0.6478313181877,
0.7283133787211,0.8001424242306,0.8679420293686,0.9343337419829,0.9520744430681),
 .UNSPECIFIED.)
GEOMETRIC_REPRESENTATION_ITEM()
RATIONAL_B_SPLINE_SURFACE(((1.07734787758409,1.07734787758409,1.07734787758409,
1.07734787758409,1.07734787758409,1.07734787758409,1.07734787758409,1.07734787758409,
1.07734787758409,1.07734787758409,1.07734787758409,1.07734787758409,1.07734787758409,
1.07734787758409,1.07734787758409,1.07734787758409),(0.974947304165518,
0.974947304165518,0.974947304165518,0.974947304165518,0.974947304165518,
0.974947304165518,0.974947304165518,0.974947304165518,0.974947304165518,
0.974947304165518,0.974947304165518,0.974947304165518,0.974947304165518,
0.974947304165518,0.974947304165518,0.974947304165518),(0.974222540387579,
0.974222540387579,0.974222540387579,0.974222540387579,0.974222540387579,
0.974222540387579,0.974222540387579,0.974222540387579,0.974222540387579,
0.974222540387579,0.974222540387579,0.974222540387579,0.974222540387579,
0.974222540387579,0.974222540387579,0.974222540387579),(1.07517358625027,
1.07517358625027,1.07517358625027,1.07517358625027,1.07517358625027,1.07517358625027,
1.07517358625027,1.07517358625027,1.07517358625027,1.07517358625027,1.07517358625027,
1.07517358625027,1.07517358625027,1.07517358625027,1.07517358625027,1.07517358625027)))
REPRESENTATION_ITEM('')
SURFACE()
);
#478=(
BOUNDED_SURFACE()
B_SPLINE_SURFACE(3,3,((#56445,#56446,#56447,#56448,#56449,#56450,#56451,
#56452,#56453,#56454,#56455),(#56456,#56457,#56458,#56459,#56460,#56461,
#56462,#56463,#56464,#56465,#56466),(#56467,#56468,#56469,#56470,#56471,
#56472,#56473,#56474,#56475,#56476,#56477),(#56478,#56479,#56480,#56481,
#56482,#56483,#56484,#56485,#56486,#56487,#56488)),.UNSPECIFIED.,.F.,.F.,
 .F.)
B_SPLINE_SURFACE_WITH_KNOTS((4,4),(4,1,1,1,1,1,1,1,4),(0.0571956856471758,
0.954452770725331),(0.2692306949416,0.2749419490826,0.3416670598954,0.4177877612555,
0.4999458204015,0.5821135283534,0.658256170395,0.7250020340387,0.7307792782023),
 .UNSPECIFIED.)
GEOMETRIC_REPRESENTATION_ITEM()
RATIONAL_B_SPLINE_SURFACE(((1.19979901822718,1.19979901822718,1.1997990182272,
1.19979901822718,1.19979901822718,1.19979901822718,1.19979901822718,1.19979901822718,
1.19979901822718,1.19979901822718,1.19979901822718),(0.929896371414247,
0.929896371414247,0.929896371414343,0.929896371414247,0.929896371414247,
0.929896371414247,0.929896371414247,0.929896371414247,0.929896371414247,
0.929896371414247,0.929896371414247),(0.933446414971094,0.933446414971094,
0.933446414971189,0.933446414971094,0.933446414971094,0.933446414971094,
0.933446414971094,0.933446414971094,0.933446414971094,0.933446414971094,
0.933446414971094),(1.21044914889772,1.21044914889772,1.21044914889774,
1.21044914889772,1.21044914889772,1.21044914889772,1.21044914889772,1.21044914889772,
1.21044914889772,1.21044914889772,1.21044914889772)))
REPRESENTATION_ITEM('')
SURFACE()
);
#479=(
BOUNDED_SURFACE()
B_SPLINE_SURFACE(3,3,((#56645,#56646,#56647,#56648,#56649,#56650,#56651,
#56652,#56653),(#56654,#56655,#56656,#56657,#56658,#56659,#56660,#56661,
#56662),(#56663,#56664,#56665,#56666,#56667,#56668,#56669,#56670,#56671),
(#56672,#56673,#56674,#56675,#56676,#56677,#56678,#56679,#56680)),
 .UNSPECIFIED.,.F.,.F.,.F.)
B_SPLINE_SURFACE_WITH_KNOTS((4,4),(4,1,1,1,1,1,4),(0.0528061476738938,0.946595630268755),
(0.233696593713312,0.2806158094266,0.377846836066,0.4768946763461,0.5774309799662,
0.6780149464306,0.75477374610499),.UNSPECIFIED.)
GEOMETRIC_REPRESENTATION_ITEM()
RATIONAL_B_SPLINE_SURFACE(((1.20378794912229,1.20378794912229,1.20378794912229,
1.20378794912229,1.20378794912229,1.20378794912229,1.20378794912229,1.20378794912229,
1.20378794912229),(0.932252425012417,0.932252425012417,0.932252425012417,
0.932252425012417,0.932252425012417,0.932252425012417,0.932252425012417,
0.932252425012417,0.932252425012417),(0.932070805185767,0.932070805185767,
0.932070805185767,0.932070805185767,0.932070805185767,0.932070805185767,
0.932070805185767,0.932070805185767,0.932070805185767),(1.20324308964234,
1.20324308964234,1.20324308964234,1.20324308964234,1.20324308964234,1.20324308964234,
1.20324308964234,1.20324308964234,1.20324308964234)))
REPRESENTATION_ITEM('')
SURFACE()
);
#480=(
BOUNDED_SURFACE()
B_SPLINE_SURFACE(3,3,((#56781,#56782,#56783,#56784,#56785,#56786,#56787,
#56788,#56789,#56790),(#56791,#56792,#56793,#56794,#56795,#56796,#56797,
#56798,#56799,#56800),(#56801,#56802,#56803,#56804,#56805,#56806,#56807,
#56808,#56809,#56810),(#56811,#56812,#56813,#56814,#56815,#56816,#56817,
#56818,#56819,#56820)),.UNSPECIFIED.,.F.,.F.,.F.)
B_SPLINE_SURFACE_WITH_KNOTS((4,4),(4,1,1,1,1,1,1,4),(0.0418818139400337,
0.96327015985212),(0.03308221537868,0.1426814397217,0.2856169891585,0.4287844208669,
0.5720769019003,0.7151865938446,0.8579144162245,0.9460833470456),
 .UNSPECIFIED.)
GEOMETRIC_REPRESENTATION_ITEM()
RATIONAL_B_SPLINE_SURFACE(((1.13002916390669,1.13002916390669,1.13002916390669,
1.13002916390669,1.13002916390669,1.13002916390669,1.13002916390669,1.13002916390669,
1.13002916390669,1.13002916390669),(0.955682077793698,0.955682077793698,
0.955682077793698,0.955682077793698,0.955682077793698,0.955682077793698,
0.955682077793698,0.955682077793698,0.955682077793698,0.955682077793698),
(0.956662427019863,0.956662427019863,0.956662427019863,0.956662427019863,
0.956662427019863,0.956662427019863,0.956662427019863,0.956662427019863,
0.956662427019863,0.956662427019863),(1.13297021158519,1.13297021158519,
1.13297021158519,1.13297021158519,1.13297021158519,1.13297021158519,1.13297021158519,
1.13297021158519,1.13297021158519,1.13297021158519)))
REPRESENTATION_ITEM('')
SURFACE()
);
#481=(
BOUNDED_SURFACE()
B_SPLINE_SURFACE(3,3,((#56916,#56917,#56918,#56919,#56920,#56921,#56922,
#56923,#56924),(#56925,#56926,#56927,#56928,#56929,#56930,#56931,#56932,
#56933),(#56934,#56935,#56936,#56937,#56938,#56939,#56940,#56941,#56942),
(#56943,#56944,#56945,#56946,#56947,#56948,#56949,#56950,#56951)),
 .UNSPECIFIED.,.F.,.F.,.F.)
B_SPLINE_SURFACE_WITH_KNOTS((4,4),(4,1,1,1,1,1,4),(0.0492017398553194,0.946591167977457),
(0.241730237030952,0.3218312021396,0.4122894732501,0.5098786318471,0.6104690043264,
0.7106140261538,0.769990664121402),.UNSPECIFIED.)
GEOMETRIC_REPRESENTATION_ITEM()
RATIONAL_B_SPLINE_SURFACE(((1.20708756720507,1.20708756720507,1.20708756720507,
1.20708756720507,1.20708756720507,1.20708756720507,1.20708756720507,1.20708756720507,
1.20708756720507),(0.932259246075696,0.932259246075696,0.932259246075696,
0.932259246075696,0.932259246075696,0.932259246075696,0.932259246075696,
0.932259246075696,0.932259246075696),(0.930976823116939,0.930976823116939,
0.930976823116939,0.930976823116939,0.930976823116939,0.930976823116939,
0.930976823116939,0.930976823116939,0.930976823116939),(1.2032402983288,
1.2032402983288,1.2032402983288,1.2032402983288,1.2032402983288,1.2032402983288,
1.2032402983288,1.2032402983288,1.2032402983288)))
REPRESENTATION_ITEM('')
SURFACE()
);
#482=(
BOUNDED_SURFACE()
B_SPLINE_SURFACE(3,3,((#57045,#57046,#57047,#57048,#57049,#57050,#57051,
#57052,#57053,#57054),(#57055,#57056,#57057,#57058,#57059,#57060,#57061,
#57062,#57063,#57064),(#57065,#57066,#57067,#57068,#57069,#57070,#57071,
#57072,#57073,#57074),(#57075,#57076,#57077,#57078,#57079,#57080,#57081,
#57082,#57083,#57084)),.UNSPECIFIED.,.F.,.F.,.F.)
B_SPLINE_SURFACE_WITH_KNOTS((4,4),(4,1,1,1,1,1,1,4),(0.0418822688619605,
0.96326878165287),(0.05391635099207,0.1420855967788,0.2848134135343,0.4279230982392,
0.5712155755112,0.7143830064632,0.8573185599676,0.9669169090933),
 .UNSPECIFIED.)
GEOMETRIC_REPRESENTATION_ITEM()
RATIONAL_B_SPLINE_SURFACE(((1.1300289100912,1.1300289100912,1.1300289100912,
1.1300289100912,1.1300289100912,1.1300289100912,1.1300289100912,1.1300289100912,
1.1300289100912,1.1300289100912),(0.955682338038116,0.955682338038116,0.955682338038116,
0.955682338038116,0.955682338038116,0.955682338038116,0.955682338038116,
0.955682338038116,0.955682338038116,0.955682338038116),(0.956662509660705,
0.956662509660705,0.956662509660705,0.956662509660705,0.956662509660705,
0.956662509660705,0.956662509660705,0.956662509660705,0.956662509660705,
0.956662509660705),(1.13296942495897,1.13296942495897,1.13296942495897,
1.13296942495897,1.13296942495897,1.13296942495897,1.13296942495897,1.13296942495897,
1.13296942495897,1.13296942495897)))
REPRESENTATION_ITEM('')
SURFACE()
);
#483=(
BOUNDED_SURFACE()
B_SPLINE_SURFACE(3,3,((#57238,#57239,#57240,#57241,#57242,#57243),(#57244,
#57245,#57246,#57247,#57248,#57249),(#57250,#57251,#57252,#57253,#57254,
#57255),(#57256,#57257,#57258,#57259,#57260,#57261)),.UNSPECIFIED.,.F.,
 .F.,.F.)
B_SPLINE_SURFACE_WITH_KNOTS((4,4),(4,1,1,4),(0.0606070589478182,0.939490001387273),
(0.199119623286195,0.3331969354622,0.6668030645378,0.800880381172182),
 .UNSPECIFIED.)
GEOMETRIC_REPRESENTATION_ITEM()
RATIONAL_B_SPLINE_SURFACE(((1.17469014882531,1.17469014882531,1.17469014882531,
1.17469014882531,1.17469014882531,1.17469014882531),(0.941744224770734,
0.941744224770734,0.941744224770734,0.941744224770734,0.941744224770734,
0.941744224770734),(0.941769953233044,0.941769953233044,0.941769953233044,
0.941769953233044,0.941769953233044,0.941769953233044),(1.17476733421225,
1.17476733421225,1.17476733421225,1.17476733421225,1.17476733421225,1.17476733421225)))
REPRESENTATION_ITEM('')
SURFACE()
);
#484=(
BOUNDED_SURFACE()
B_SPLINE_SURFACE(3,3,((#57525,#57526,#57527,#57528,#57529,#57530,#57531,
#57532,#57533,#57534,#57535,#57536,#57537,#57538,#57539,#57540,#57541,#57542,
#57543,#57544),(#57545,#57546,#57547,#57548,#57549,#57550,#57551,#57552,
#57553,#57554,#57555,#57556,#57557,#57558,#57559,#57560,#57561,#57562,#57563,
#57564),(#57565,#57566,#57567,#57568,#57569,#57570,#57571,#57572,#57573,
#57574,#57575,#57576,#57577,#57578,#57579,#57580,#57581,#57582,#57583,#57584),
(#57585,#57586,#57587,#57588,#57589,#57590,#57591,#57592,#57593,#57594,
#57595,#57596,#57597,#57598,#57599,#57600,#57601,#57602,#57603,#57604)),
 .UNSPECIFIED.,.F.,.F.,.F.)
B_SPLINE_SURFACE_WITH_KNOTS((4,4),(4,1,1,1,1,1,1,1,1,1,1,1,1,1,1,1,1,4),
(0.063307662778757,0.939200287735074),(-0.009153831279309,0.,0.07546639963968,
0.155717790699,0.2403998675739,0.3291523205437,0.4125160476044,0.4856762677962,
0.5506584357865,0.6094492100253,0.6638177940728,0.7128085155366,0.7565093937177,
0.7968455102028,0.8357682044765,0.8748882668516,0.9149303281208,0.9275319405256),
 .UNSPECIFIED.)
GEOMETRIC_REPRESENTATION_ITEM()
RATIONAL_B_SPLINE_SURFACE(((1.07645083004906,1.07645083004906,1.07645083004906,
1.07645083004906,1.07645083004906,1.07645083004906,1.07645083004906,1.07645083004906,
1.07645083004906,1.07645083004906,1.07645083004906,1.07645083004906,1.07645083004906,
1.07645083004906,1.07645083004906,1.07645083004906,1.07645083004906,1.07645083004906,
1.07645083004906,1.07645083004906),(0.97422368215523,0.97422368215523,0.97422368215523,
0.97422368215523,0.97422368215523,0.97422368215523,0.97422368215523,0.97422368215523,
0.97422368215523,0.97422368215523,0.97422368215523,0.97422368215523,0.97422368215523,
0.97422368215523,0.97422368215523,0.97422368215523,0.97422368215523,0.97422368215523,
0.97422368215523,0.97422368215523),(0.974517230502929,0.974517230502929,
0.974517230502929,0.974517230502929,0.974517230502929,0.974517230502929,
0.974517230502929,0.974517230502929,0.974517230502929,0.974517230502929,
0.974517230502929,0.974517230502929,0.974517230502929,0.974517230502929,
0.974517230502929,0.974517230502929,0.974517230502929,0.974517230502929,
0.974517230502929,0.974517230502929),(1.07733147509216,1.07733147509216,
1.07733147509216,1.07733147509216,1.07733147509216,1.07733147509216,1.07733147509216,
1.07733147509216,1.07733147509216,1.07733147509216,1.07733147509216,1.07733147509216,
1.07733147509216,1.07733147509216,1.07733147509216,1.07733147509216,1.07733147509216,
1.07733147509216,1.07733147509216,1.07733147509216)))
REPRESENTATION_ITEM('')
SURFACE()
);
#485=(
BOUNDED_SURFACE()
B_SPLINE_SURFACE(3,3,((#57766,#57767,#57768,#57769,#57770,#57771,#57772,
#57773,#57774,#57775),(#57776,#57777,#57778,#57779,#57780,#57781,#57782,
#57783,#57784,#57785),(#57786,#57787,#57788,#57789,#57790,#57791,#57792,
#57793,#57794,#57795),(#57796,#57797,#57798,#57799,#57800,#57801,#57802,
#57803,#57804,#57805)),.UNSPECIFIED.,.F.,.F.,.F.)
B_SPLINE_SURFACE_WITH_KNOTS((4,4),(4,1,1,1,1,1,1,4),(0.0487270299825949,
0.94659521046586),(0.230696758264988,0.2874600458818,0.3870132126609,0.4873166184574,
0.5850151645794,0.675938646053,0.7570631380884,0.759743236107495),
 .UNSPECIFIED.)
GEOMETRIC_REPRESENTATION_ITEM()
RATIONAL_B_SPLINE_SURFACE(((1.20752814113149,1.20752814113149,1.20752814113149,
1.20752814113149,1.20752814113149,1.20752814113149,1.20752814113149,1.20752814113149,
1.20752814113149,1.20752814113149),(0.932258069051191,0.932258069051191,
0.932258069051191,0.932258069051191,0.932258069051191,0.932258069051191,
0.932258069051191,0.932258069051191,0.932258069051191,0.932258069051191),
(0.930831385763603,0.930831385763603,0.930831385763603,0.930831385763603,
0.930831385763603,0.930831385763603,0.930831385763603,0.930831385763603,
0.930831385763603,0.930831385763603),(1.20324809126873,1.20324809126873,
1.20324809126873,1.20324809126873,1.20324809126873,1.20324809126873,1.20324809126873,
1.20324809126873,1.20324809126873,1.20324809126873)))
REPRESENTATION_ITEM('')
SURFACE()
);
#486=(
BOUNDED_SURFACE()
B_SPLINE_SURFACE(3,3,((#57925,#57926,#57927,#57928,#57929,#57930,#57931,
#57932,#57933,#57934,#57935),(#57936,#57937,#57938,#57939,#57940,#57941,
#57942,#57943,#57944,#57945,#57946),(#57947,#57948,#57949,#57950,#57951,
#57952,#57953,#57954,#57955,#57956,#57957),(#57958,#57959,#57960,#57961,
#57962,#57963,#57964,#57965,#57966,#57967,#57968)),.UNSPECIFIED.,.F.,.F.,
 .F.)
B_SPLINE_SURFACE_WITH_KNOTS((4,4),(4,1,1,1,1,1,1,1,4),(0.0595203864762429,
0.937476996026637),(0.05105962729005,0.1243084941807,0.2492353165502,0.3744835129416,
0.4998949769261,0.6253220276845,0.7506164023093,0.8756120170229,0.9160299525995),
 .UNSPECIFIED.)
GEOMETRIC_REPRESENTATION_ITEM()
RATIONAL_B_SPLINE_SURFACE(((1.11958055541173,1.11958055541173,1.11958055541173,
1.11958055541173,1.11958055541173,1.11958055541173,1.11958055541173,1.11958055541173,
1.11958055541173,1.11958055541173,1.11958055541173),(0.960683244731665,
0.960683244731665,0.960683244731665,0.960683244731665,0.960683244731665,
0.960683244731665,0.960683244731665,0.960683244731665,0.960683244731665,
0.960683244731665,0.960683244731665),(0.960141667061955,0.960141667061955,
0.960141667061955,0.960141667061955,0.960141667061955,0.960141667061955,
0.960141667061955,0.960141667061955,0.960141667061955,0.960141667061955,
0.960141667061955),(1.1179558224026,1.1179558224026,1.1179558224026,1.1179558224026,
1.1179558224026,1.1179558224026,1.1179558224026,1.1179558224026,1.1179558224026,
1.1179558224026,1.1179558224026)))
REPRESENTATION_ITEM('')
SURFACE()
);
#487=(
BOUNDED_SURFACE()
B_SPLINE_SURFACE(3,3,((#58202,#58203,#58204,#58205,#58206,#58207,#58208,
#58209,#58210),(#58211,#58212,#58213,#58214,#58215,#58216,#58217,#58218,
#58219),(#58220,#58221,#58222,#58223,#58224,#58225,#58226,#58227,#58228),
(#58229,#58230,#58231,#58232,#58233,#58234,#58235,#58236,#58237)),
 .UNSPECIFIED.,.F.,.F.,.F.)
B_SPLINE_SURFACE_WITH_KNOTS((4,4),(4,1,1,1,1,1,4),(0.0580435500156731,0.958553804869728),
(0.2691745286223,0.3315918821098,0.4168737318583,0.5000003344174,0.583127115061,
0.6684093799117,0.7308143681514),.UNSPECIFIED.)
GEOMETRIC_REPRESENTATION_ITEM()
RATIONAL_B_SPLINE_SURFACE(((1.19903754000942,1.19903754000942,1.19903754000942,
1.19903754000942,1.19903754000942,1.19903754000942,1.19903754000942,1.19903754000942,
1.19903754000942),(0.928671012740672,0.928671012740672,0.928671012740672,
0.928671012740672,0.928671012740672,0.928671012740672,0.928671012740672,
0.928671012740672,0.928671012740672),(0.933747722450839,0.933747722450839,
0.933747722450839,0.933747722450839,0.933747722450839,0.933747722450839,
0.933747722450839,0.933747722450839,0.933747722450839),(1.21426766913992,
1.21426766913992,1.21426766913992,1.21426766913992,1.21426766913992,1.21426766913992,
1.21426766913992,1.21426766913992,1.21426766913992)))
REPRESENTATION_ITEM('')
SURFACE()
);
#488=(
BOUNDED_SURFACE()
B_SPLINE_SURFACE(3,3,((#58314,#58315,#58316,#58317,#58318,#58319,#58320,
#58321,#58322,#58323,#58324),(#58325,#58326,#58327,#58328,#58329,#58330,
#58331,#58332,#58333,#58334,#58335),(#58336,#58337,#58338,#58339,#58340,
#58341,#58342,#58343,#58344,#58345,#58346),(#58347,#58348,#58349,#58350,
#58351,#58352,#58353,#58354,#58355,#58356,#58357)),.UNSPECIFIED.,.F.,.F.,
 .F.)
B_SPLINE_SURFACE_WITH_KNOTS((4,4),(4,1,1,1,1,1,1,1,4),(0.0422653268062964,
0.937533390179831),(-0.009351371223958,0.,0.1428542653358,0.2856978653279,
0.4287777392072,0.5720428464823,0.7151350525691,0.8578442953538,0.9437353734563),
 .UNSPECIFIED.)
GEOMETRIC_REPRESENTATION_ITEM()
RATIONAL_B_SPLINE_SURFACE(((1.12913274597187,1.12913274597187,1.12913274597187,
1.12913274597187,1.12913274597187,1.12913274597187,1.12913274597187,1.12913274597187,
1.12913274597187,1.12913274597187,1.12913274597187),(0.960755109792916,
0.960755109792916,0.960755109792916,0.960755109792916,0.960755109792916,
0.960755109792916,0.960755109792916,0.960755109792916,0.960755109792916,
0.960755109792916,0.960755109792916),(0.957039590212626,0.957039590212626,
0.957039590212626,0.957039590212626,0.957039590212626,0.957039590212626,
0.957039590212626,0.957039590212626,0.957039590212626,0.957039590212626,
0.957039590212626),(1.117986187231,1.117986187231,1.117986187231,1.117986187231,
1.117986187231,1.117986187231,1.117986187231,1.117986187231,1.117986187231,
1.117986187231,1.117986187231)))
REPRESENTATION_ITEM('')
SURFACE()
);
#489=(
BOUNDED_SURFACE()
B_SPLINE_SURFACE(3,3,((#58567,#58568,#58569,#58570,#58571,#58572,#58573,
#58574,#58575),(#58576,#58577,#58578,#58579,#58580,#58581,#58582,#58583,
#58584),(#58585,#58586,#58587,#58588,#58589,#58590,#58591,#58592,#58593),
(#58594,#58595,#58596,#58597,#58598,#58599,#58600,#58601,#58602)),
 .UNSPECIFIED.,.F.,.F.,.F.)
B_SPLINE_SURFACE_WITH_KNOTS((4,4),(4,1,1,1,1,1,4),(0.0522319358346092,0.946599708933178),
(0.243637547330016,0.3281816498601,0.4286250598175,0.5281721425414,0.6260232294075,
0.7222208859256,0.765710581954822),.UNSPECIFIED.)
GEOMETRIC_REPRESENTATION_ITEM()
RATIONAL_B_SPLINE_SURFACE(((1.20431342445013,1.20431342445013,1.20431342445013,
1.20431342445013,1.20431342445013,1.20431342445013,1.20431342445013,1.20431342445013,
1.20431342445013),(0.932250933377241,0.932250933377241,0.932250933377241,
0.932250933377241,0.932250933377241,0.932250933377241,0.932250933377241,
0.932250933377241,0.932250933377241),(0.931895988864253,0.931895988864253,
0.931895988864253,0.931895988864253,0.931895988864253,0.931895988864253,
0.931895988864253,0.931895988864253,0.931895988864253),(1.20324859091116,
1.20324859091116,1.20324859091116,1.20324859091116,1.20324859091116,1.20324859091116,
1.20324859091116,1.20324859091116,1.20324859091116)))
REPRESENTATION_ITEM('')
SURFACE()
);
#490=(
BOUNDED_SURFACE()
B_SPLINE_SURFACE(3,3,((#58701,#58702,#58703,#58704,#58705,#58706,#58707,
#58708,#58709,#58710,#58711),(#58712,#58713,#58714,#58715,#58716,#58717,
#58718,#58719,#58720,#58721,#58722),(#58723,#58724,#58725,#58726,#58727,
#58728,#58729,#58730,#58731,#58732,#58733),(#58734,#58735,#58736,#58737,
#58738,#58739,#58740,#58741,#58742,#58743,#58744)),.UNSPECIFIED.,.F.,.F.,
 .F.)
B_SPLINE_SURFACE_WITH_KNOTS((4,4),(4,1,1,1,1,1,1,1,4),(0.0572670136322689,
0.950748781721039),(0.269229383309,0.2752759889051,0.3420135561061,0.4180771376681,
0.4999456411107,0.5818236269898,0.657909057418,0.7246675349474,0.7307806429001),
 .UNSPECIFIED.)
GEOMETRIC_REPRESENTATION_ITEM()
RATIONAL_B_SPLINE_SURFACE(((1.19973463403615,1.19973463403615,1.19973463403615,
1.19973463403615,1.19973463403615,1.19973463403615,1.19973463403615,1.19973463403615,
1.19973463403615,1.19973463403615,1.19973463403615),(0.931010957144128,
0.931010957144128,0.931010957144128,0.931010957144128,0.931010957144128,
0.931010957144128,0.931010957144128,0.931010957144128,0.931010957144128,
0.931010957144128,0.931010957144128),(0.933443613018979,0.933443613018979,
0.933443613018979,0.933443613018979,0.933443613018979,0.933443613018979,
0.933443613018979,0.933443613018979,0.933443613018979,0.933443613018979,
0.933443613018979),(1.2070326016607,1.2070326016607,1.2070326016607,1.2070326016607,
1.2070326016607,1.2070326016607,1.2070326016607,1.2070326016607,1.2070326016607,
1.2070326016607,1.2070326016607)))
REPRESENTATION_ITEM('')
SURFACE()
);
#491=(
BOUNDED_SURFACE()
B_SPLINE_SURFACE(3,3,((#59178,#59179,#59180,#59181,#59182,#59183,#59184,
#59185,#59186,#59187,#59188,#59189,#59190,#59191,#59192,#59193),(#59194,
#59195,#59196,#59197,#59198,#59199,#59200,#59201,#59202,#59203,#59204,#59205,
#59206,#59207,#59208,#59209),(#59210,#59211,#59212,#59213,#59214,#59215,
#59216,#59217,#59218,#59219,#59220,#59221,#59222,#59223,#59224,#59225),
(#59226,#59227,#59228,#59229,#59230,#59231,#59232,#59233,#59234,#59235,
#59236,#59237,#59238,#59239,#59240,#59241)),.UNSPECIFIED.,.F.,.F.,.F.)
B_SPLINE_SURFACE_WITH_KNOTS((4,4),(4,1,1,1,1,1,1,1,1,1,1,1,1,4),(0.0586203715926453,
0.933020863373606),(-0.009395290952153,0.,0.07535316275351,0.1579191313331,
0.2496874711698,0.3528406113057,0.4595229844577,0.5578824678157,0.6478335957937,
0.7283142435542,0.8001427386493,0.8679421724001,0.9343338107667,0.952074442993),
 .UNSPECIFIED.)
GEOMETRIC_REPRESENTATION_ITEM()
RATIONAL_B_SPLINE_SURFACE(((1.07810380266528,1.07810380266528,1.07810380266528,
1.07810380266528,1.07810380266528,1.07810380266528,1.07810380266528,1.07810380266528,
1.07810380266528,1.07810380266528,1.07810380266528,1.07810380266528,1.07810380266528,
1.07810380266528,1.07810380266528,1.07810380266528),(0.974951475937913,
0.974951475937913,0.974951475937913,0.974951475937913,0.974951475937913,
0.974951475937913,0.974951475937913,0.974951475937913,0.974951475937913,
0.974951475937913,0.974951475937913,0.974951475937913,0.974951475937913,
0.974951475937913,0.974951475937913,0.974951475937913),(0.973974736181131,
0.973974736181131,0.973974736181131,0.973974736181131,0.973974736181131,
0.973974736181131,0.973974736181131,0.973974736181131,0.973974736181131,
0.973974736181131,0.973974736181131,0.973974736181131,0.973974736181131,
0.973974736181131,0.973974736181131,0.973974736181131),(1.07517358339494,
1.07517358339494,1.07517358339494,1.07517358339494,1.07517358339494,1.07517358339494,
1.07517358339494,1.07517358339494,1.07517358339494,1.07517358339494,1.07517358339494,
1.07517358339494,1.07517358339494,1.07517358339494,1.07517358339494,1.07517358339494)))
REPRESENTATION_ITEM('')
SURFACE()
);
#492=(
BOUNDED_SURFACE()
B_SPLINE_SURFACE(3,3,((#59414,#59415,#59416,#59417,#59418,#59419),(#59420,
#59421,#59422,#59423,#59424,#59425),(#59426,#59427,#59428,#59429,#59430,
#59431),(#59432,#59433,#59434,#59435,#59436,#59437)),.UNSPECIFIED.,.F.,
 .F.,.F.)
B_SPLINE_SURFACE_WITH_KNOTS((4,4),(4,1,1,4),(0.0606720802686711,0.938680242175199),
(-1.E-5,0.,0.3335568389414,0.663356367030841),.UNSPECIFIED.)
GEOMETRIC_REPRESENTATION_ITEM()
RATIONAL_B_SPLINE_SURFACE(((1.17463054343028,1.17463054343028,1.17463054343028,
1.17463054343028,1.17463054343028,1.17463054343028),(0.941961451143953,
0.941961451143953,0.941961451143953,0.941961451143953,0.941961451143953,
0.941961451143953),(0.941789945370804,0.941789945370804,0.941789945370804,
0.941789945370804,0.941789945370804,0.941789945370804),(1.17411602611083,
1.17411602611083,1.17411602611083,1.17411602611083,1.17411602611083,1.17411602611083)))
REPRESENTATION_ITEM('')
SURFACE()
);
#493=(
BOUNDED_SURFACE()
B_SPLINE_SURFACE(3,3,((#59679,#59680,#59681,#59682,#59683,#59684,#59685,
#59686,#59687,#59688,#59689,#59690,#59691,#59692,#59693,#59694,#59695,#59696,
#59697,#59698),(#59699,#59700,#59701,#59702,#59703,#59704,#59705,#59706,
#59707,#59708,#59709,#59710,#59711,#59712,#59713,#59714,#59715,#59716,#59717,
#59718),(#59719,#59720,#59721,#59722,#59723,#59724,#59725,#59726,#59727,
#59728,#59729,#59730,#59731,#59732,#59733,#59734,#59735,#59736,#59737,#59738),
(#59739,#59740,#59741,#59742,#59743,#59744,#59745,#59746,#59747,#59748,
#59749,#59750,#59751,#59752,#59753,#59754,#59755,#59756,#59757,#59758)),
 .UNSPECIFIED.,.F.,.F.,.F.)
B_SPLINE_SURFACE_WITH_KNOTS((4,4),(4,1,1,1,1,1,1,1,1,1,1,1,1,1,1,1,1,4),
(0.0633076876987065,0.940112450452113),(-0.009153831272559,0.,0.07546697590282,
0.1557186836765,0.240400675928,0.3291525043907,0.4125154315421,0.4856750471872,
0.5506567542878,0.6094471595415,0.6638154833413,0.7128062934011,0.7565074154861,
0.7968438500049,0.8357668687042,0.874887243177,0.9149296242807,0.9275319406291),
 .UNSPECIFIED.)
GEOMETRIC_REPRESENTATION_ITEM()
RATIONAL_B_SPLINE_SURFACE(((1.07645082081108,1.07645082081108,1.07645082081108,
1.07645082081108,1.07645082081108,1.07645082081108,1.07645082081108,1.07645082081108,
1.07645082081108,1.07645082081108,1.07645082081108,1.07645082081108,1.07645082081108,
1.07645082081108,1.07645082081108,1.07645082081108,1.07645082081108,1.07645082081108,
1.07645082081108,1.07645082081108),(0.974117222049909,0.974117222049909,
0.974117222049909,0.974117222049909,0.974117222049909,0.974117222049909,
0.974117222049909,0.974117222049909,0.974117222049909,0.974117222049909,
0.974117222049909,0.974117222049909,0.974117222049909,0.974117222049909,
0.974117222049909,0.974117222049909,0.974117222049909,0.974117222049909,
0.974117222049909,0.974117222049909),(0.97451795619999,0.97451795619999,
0.97451795619999,0.97451795619999,0.97451795619999,0.97451795619999,0.97451795619999,
0.97451795619999,0.97451795619999,0.97451795619999,0.97451795619999,0.97451795619999,
0.97451795619999,0.97451795619999,0.97451795619999,0.97451795619999,0.97451795619999,
0.97451795619999,0.97451795619999,0.97451795619999),(1.07765302326132,1.07765302326132,
1.07765302326132,1.07765302326132,1.07765302326132,1.07765302326132,1.07765302326132,
1.07765302326132,1.07765302326132,1.07765302326132,1.07765302326132,1.07765302326132,
1.07765302326132,1.07765302326132,1.07765302326132,1.07765302326132,1.07765302326132,
1.07765302326132,1.07765302326132,1.07765302326132)))
REPRESENTATION_ITEM('')
SURFACE()
);
#494=(
BOUNDED_SURFACE()
B_SPLINE_SURFACE(3,3,((#59922,#59923,#59924,#59925,#59926,#59927,#59928,
#59929,#59930),(#59931,#59932,#59933,#59934,#59935,#59936,#59937,#59938,
#59939),(#59940,#59941,#59942,#59943,#59944,#59945,#59946,#59947,#59948),
(#59949,#59950,#59951,#59952,#59953,#59954,#59955,#59956,#59957)),
 .UNSPECIFIED.,.F.,.F.,.F.)
B_SPLINE_SURFACE_WITH_KNOTS((4,4),(4,1,1,1,1,1,4),(0.0556339209179322,0.946594676964208),
(0.23622684912609,0.2892204677235,0.3894748956345,0.4915097291946,0.5954545891223,
0.7006023497823,0.755351077420202),.UNSPECIFIED.)
GEOMETRIC_REPRESENTATION_ITEM()
RATIONAL_B_SPLINE_SURFACE(((1.20122430718483,1.20122430718483,1.20122430718483,
1.20122430718483,1.20122430718483,1.20122430718483,1.20122430718483,1.20122430718483,
1.20122430718483),(0.932252440213298,0.932252440213298,0.932252440213298,
0.932252440213298,0.932252440213298,0.932252440213298,0.932252440213298,
0.932252440213298,0.932252440213298),(0.932926918038345,0.932926918038345,
0.932926918038345,0.932926918038345,0.932926918038345,0.932926918038345,
0.932926918038345,0.932926918038345,0.932926918038345),(1.20324774065997,
1.20324774065997,1.20324774065997,1.20324774065997,1.20324774065997,1.20324774065997,
1.20324774065997,1.20324774065997,1.20324774065997)))
REPRESENTATION_ITEM('')
SURFACE()
);
#495=(
BOUNDED_SURFACE()
B_SPLINE_SURFACE(3,3,((#60077,#60078,#60079,#60080,#60081,#60082,#60083,
#60084,#60085,#60086,#60087),(#60088,#60089,#60090,#60091,#60092,#60093,
#60094,#60095,#60096,#60097,#60098),(#60099,#60100,#60101,#60102,#60103,
#60104,#60105,#60106,#60107,#60108,#60109),(#60110,#60111,#60112,#60113,
#60114,#60115,#60116,#60117,#60118,#60119,#60120)),.UNSPECIFIED.,.F.,.F.,
 .F.)
B_SPLINE_SURFACE_WITH_KNOTS((4,4),(4,1,1,1,1,1,1,1,4),(0.0595078021839535,
0.938342362610477),(0.05105962744621,0.1243082719354,0.2492351900332,0.374483525782,
0.4998948479171,0.6253218237211,0.750616579156,0.8756124488067,0.9160299520784),
 .UNSPECIFIED.)
GEOMETRIC_REPRESENTATION_ITEM()
RATIONAL_B_SPLINE_SURFACE(((1.1195873881288,1.1195873881288,1.1195873881288,
1.1195873881288,1.1195873881288,1.1195873881288,1.1195873881288,1.1195873881288,
1.1195873881288,1.1195873881288,1.1195873881288),(0.96052663714813,0.96052663714813,
0.96052663714813,0.96052663714813,0.96052663714813,0.96052663714813,0.96052663714813,
0.96052663714813,0.96052663714813,0.96052663714813,0.96052663714813),(0.960138486797252,
0.960138486797252,0.960138486797252,0.960138486797252,0.960138486797252,
0.960138486797252,0.960138486797252,0.960138486797252,0.960138486797252,
0.960138486797252,0.960138486797252),(1.11842293707616,1.11842293707616,
1.11842293707616,1.11842293707616,1.11842293707616,1.11842293707616,1.11842293707616,
1.11842293707616,1.11842293707616,1.11842293707616,1.11842293707616)))
REPRESENTATION_ITEM('')
SURFACE()
);
#496=(
BOUNDED_SURFACE()
B_SPLINE_SURFACE(3,3,((#60413,#60414,#60415,#60416,#60417,#60418,#60419,
#60420,#60421),(#60422,#60423,#60424,#60425,#60426,#60427,#60428,#60429,
#60430),(#60431,#60432,#60433,#60434,#60435,#60436,#60437,#60438,#60439),
(#60440,#60441,#60442,#60443,#60444,#60445,#60446,#60447,#60448)),
 .UNSPECIFIED.,.F.,.F.,.F.)
B_SPLINE_SURFACE_WITH_KNOTS((4,4),(4,1,1,1,1,1,4),(0.0549132206529749,0.961333582072497),
(0.269227069858,0.3329416456222,0.4153128648057,0.5000235250822,0.5847341870831,
0.6671012504363,0.7307621725325),.UNSPECIFIED.)
GEOMETRIC_REPRESENTATION_ITEM()
RATIONAL_B_SPLINE_SURFACE(((1.20186626112831,1.20186626112831,1.20186626112831,
1.20186626112831,1.20186626112831,1.20186626112831,1.20186626112831,1.20186626112831,
1.20186626112831),(0.92779882400403,0.92779882400403,0.92779882400403,0.92779882400403,
0.92779882400403,0.92779882400403,0.92779882400403,0.92779882400403,0.92779882400403),
(0.932800904262363,0.932800904262363,0.932800904262363,0.932800904262363,
0.932800904262363,0.932800904262363,0.932800904262363,0.932800904262363,
0.932800904262363),(1.21687250190331,1.21687250190331,1.21687250190331,
1.21687250190331,1.21687250190331,1.21687250190331,1.21687250190331,1.21687250190331,
1.21687250190331)))
REPRESENTATION_ITEM('')
SURFACE()
);
#497=(
BOUNDED_SURFACE()
B_SPLINE_SURFACE(3,3,((#60533,#60534,#60535,#60536,#60537,#60538,#60539,
#60540,#60541),(#60542,#60543,#60544,#60545,#60546,#60547,#60548,#60549,
#60550),(#60551,#60552,#60553,#60554,#60555,#60556,#60557,#60558,#60559),
(#60560,#60561,#60562,#60563,#60564,#60565,#60566,#60567,#60568)),
 .UNSPECIFIED.,.F.,.F.,.F.)
B_SPLINE_SURFACE_WITH_KNOTS((4,4),(4,1,1,1,1,1,4),(0.0551738827458389,0.94659152318391),
(0.245643394324907,0.2993405166024,0.4044749934007,0.5084175034907,0.6104536407677,
0.7107127111402,0.764615799035645),.UNSPECIFIED.)
GEOMETRIC_REPRESENTATION_ITEM()
RATIONAL_B_SPLINE_SURFACE(((1.20163682857439,1.20163682857439,1.20163682857439,
1.20163682857439,1.20163682857439,1.20163682857439,1.20163682857439,1.20163682857439,
1.20163682857439),(0.932254225678232,0.932254225678232,0.932254225678232,
0.932254225678232,0.932254225678232,0.932254225678232,0.932254225678232,
0.932254225678232,0.932254225678232),(0.932788782470288,0.932788782470288,
0.932788782470288,0.932788782470288,0.932788782470288,0.932788782470288,
0.932788782470288,0.932788782470288,0.932788782470288),(1.20324049895056,
1.20324049895056,1.20324049895056,1.20324049895056,1.20324049895056,1.20324049895056,
1.20324049895056,1.20324049895056,1.20324049895056)))
REPRESENTATION_ITEM('')
SURFACE()
);
#498=(
BOUNDED_SURFACE()
B_SPLINE_SURFACE(3,3,((#60663,#60664,#60665,#60666,#60667,#60668,#60669,
#60670,#60671,#60672),(#60673,#60674,#60675,#60676,#60677,#60678,#60679,
#60680,#60681,#60682),(#60683,#60684,#60685,#60686,#60687,#60688,#60689,
#60690,#60691,#60692),(#60693,#60694,#60695,#60696,#60697,#60698,#60699,
#60700,#60701,#60702)),.UNSPECIFIED.,.F.,.F.,.F.)
B_SPLINE_SURFACE_WITH_KNOTS((4,4),(4,1,1,1,1,1,1,4),(0.041884544995783,
0.963268707501492),(0.05391635144467,0.142084834672,0.2848129606579,0.4279230595161,
0.5712157651896,0.7143832496897,0.8573185671688,0.966916909086),
 .UNSPECIFIED.)
GEOMETRIC_REPRESENTATION_ITEM()
RATIONAL_B_SPLINE_SURFACE(((1.13002761804694,1.13002761804694,1.13002761804694,
1.13002761804694,1.13002761804694,1.13002761804694,1.13002761804694,1.13002761804694,
1.13002761804694,1.13002761804694),(0.955682356900717,0.955682356900717,
0.955682356900717,0.955682356900717,0.955682356900717,0.955682356900717,
0.955682356900717,0.955682356900717,0.955682356900717,0.955682356900717),
(0.956662945028202,0.956662945028202,0.956662945028202,0.956662945028202,
0.956662945028202,0.956662945028202,0.956662945028202,0.956662945028202,
0.956662945028202,0.956662945028202),(1.1329693824294,1.1329693824294,1.1329693824294,
1.1329693824294,1.1329693824294,1.1329693824294,1.1329693824294,1.1329693824294,
1.1329693824294,1.1329693824294)))
REPRESENTATION_ITEM('')
SURFACE()
);
#499=(
BOUNDED_SURFACE()
B_SPLINE_SURFACE(3,3,((#60795,#60796,#60797,#60798,#60799,#60800),(#60801,
#60802,#60803,#60804,#60805,#60806),(#60807,#60808,#60809,#60810,#60811,
#60812),(#60813,#60814,#60815,#60816,#60817,#60818)),.UNSPECIFIED.,.F.,
 .F.,.F.)
B_SPLINE_SURFACE_WITH_KNOTS((4,4),(4,1,1,4),(0.0606070674814838,0.939489987503615),
(0.199119642928049,0.3332353956662,0.6667646043338,0.800880362821028),
 .UNSPECIFIED.)
GEOMETRIC_REPRESENTATION_ITEM()
RATIONAL_B_SPLINE_SURFACE(((1.17469014203132,1.17469014203132,1.17469014203132,
1.17469014203132,1.17469014203132,1.17469014203132),(0.941744228453835,
0.941744228453835,0.941744228453835,0.941744228453835,0.941744228453835,
0.941744228453835),(0.941769955497328,0.941769955497328,0.941769955497328,
0.941769955497328,0.941769955497328,0.941769955497328),(1.1747673231618,
1.1747673231618,1.1747673231618,1.1747673231618,1.1747673231618,1.1747673231618)))
REPRESENTATION_ITEM('')
SURFACE()
);
#500=(
BOUNDED_SURFACE()
B_SPLINE_SURFACE(3,3,((#60824,#60825,#60826,#60827,#60828,#60829,#60830,
#60831,#60832,#60833),(#60834,#60835,#60836,#60837,#60838,#60839,#60840,
#60841,#60842,#60843),(#60844,#60845,#60846,#60847,#60848,#60849,#60850,
#60851,#60852,#60853),(#60854,#60855,#60856,#60857,#60858,#60859,#60860,
#60861,#60862,#60863)),.UNSPECIFIED.,.F.,.F.,.F.)
B_SPLINE_SURFACE_WITH_KNOTS((4,4),(4,1,1,1,1,1,1,4),(0.0418820911112758,
0.963270219149611),(0.03308221537276,0.1426814328191,0.2856167501412,0.4287842346698,
0.5720769404872,0.7151870396265,0.8579151658318,0.9460833466072),
 .UNSPECIFIED.)
GEOMETRIC_REPRESENTATION_ITEM()
RATIONAL_B_SPLINE_SURFACE(((1.13002900659617,1.13002900659617,1.13002900659617,
1.13002900659617,1.13002900659617,1.13002900659617,1.13002900659617,1.13002900659617,
1.13002900659617,1.13002900659617),(0.95568206715303,0.95568206715303,0.95568206715303,
0.95568206715303,0.95568206715303,0.95568206715303,0.95568206715303,0.95568206715303,
0.95568206715303,0.95568206715303),(0.956662480172929,0.956662480172929,
0.956662480172929,0.956662480172929,0.956662480172929,0.956662480172929,
0.956662480172929,0.956662480172929,0.956662480172929,0.956662480172929),
(1.13297024565587,1.13297024565587,1.13297024565587,1.13297024565587,1.13297024565587,
1.13297024565587,1.13297024565587,1.13297024565587,1.13297024565587,1.13297024565587)))
REPRESENTATION_ITEM('')
SURFACE()
);
#501=(
BOUNDED_SURFACE()
B_SPLINE_SURFACE(3,3,((#61020,#61021,#61022,#61023,#61024,#61025,#61026,
#61027,#61028),(#61029,#61030,#61031,#61032,#61033,#61034,#61035,#61036,
#61037),(#61038,#61039,#61040,#61041,#61042,#61043,#61044,#61045,#61046),
(#61047,#61048,#61049,#61050,#61051,#61052,#61053,#61054,#61055)),
 .UNSPECIFIED.,.F.,.F.,.F.)
B_SPLINE_SURFACE_WITH_KNOTS((4,4),(4,1,1,1,1,1,4),(0.0519164749251763,0.946596975406882),
(0.23281373816856,0.2786409342623,0.3751379338287,0.4733293945345,0.5731667317773,
0.6736811683426,0.755675667880648),.UNSPECIFIED.)
GEOMETRIC_REPRESENTATION_ITEM()
RATIONAL_B_SPLINE_SURFACE(((1.20459928322244,1.20459928322244,1.20459928322244,
1.20459928322244,1.20459928322244,1.20459928322244,1.20459928322244,1.20459928322244,
1.20459928322244),(0.932252754256132,0.932252754256133,0.932252754256132,
0.932252754256132,0.932252754256132,0.932252754256132,0.932252754256132,
0.932252754256133,0.932252754256132),(0.931800989552072,0.931800989552072,
0.931800989552072,0.931800989552072,0.931800989552072,0.931800989552072,
0.931800989552072,0.931800989552072,0.931800989552072),(1.20324398911026,
1.20324398911026,1.20324398911026,1.20324398911026,1.20324398911026,1.20324398911026,
1.20324398911026,1.20324398911026,1.20324398911026)))
REPRESENTATION_ITEM('')
SURFACE()
);
#502=(
BOUNDED_SURFACE()
B_SPLINE_SURFACE(3,3,((#61113,#61114,#61115,#61116,#61117,#61118,#61119,
#61120,#61121,#61122),(#61123,#61124,#61125,#61126,#61127,#61128,#61129,
#61130,#61131,#61132),(#61133,#61134,#61135,#61136,#61137,#61138,#61139,
#61140,#61141,#61142),(#61143,#61144,#61145,#61146,#61147,#61148,#61149,
#61150,#61151,#61152)),.UNSPECIFIED.,.F.,.F.,.F.)
B_SPLINE_SURFACE_WITH_KNOTS((4,4),(4,1,1,1,1,1,1,4),(0.0506777938854956,
0.94932519705549),(0.077728727808056,0.1141533201323,0.2302983301971,0.3458029403667,
0.4595257213141,0.5713502050872,0.6814413055602,0.713640661394635),
 .UNSPECIFIED.)
GEOMETRIC_REPRESENTATION_ITEM()
RATIONAL_B_SPLINE_SURFACE(((1.20573036432394,1.20573036432394,1.20573036432394,
1.20573036432394,1.20573036432394,1.20573036432394,1.20573036432394,1.20573036432394,
1.20573036432394,1.20573036432394),(0.931422298920844,0.931422298920844,
0.931422298920844,0.931422298920844,0.931422298920844,0.931422298920844,
0.931422298920844,0.931422298920844,0.931422298920844,0.931422298920844),
(0.931423211895124,0.931423211895124,0.931423211895124,0.931423211895124,
0.931423211895124,0.931423211895124,0.931423211895124,0.931423211895124,
0.931423211895124,0.931423211895124),(1.20573310324678,1.20573310324678,
1.20573310324678,1.20573310324678,1.20573310324678,1.20573310324678,1.20573310324678,
1.20573310324678,1.20573310324678,1.20573310324678)))
REPRESENTATION_ITEM('')
SURFACE()
);
#503=(
BOUNDED_SURFACE()
B_SPLINE_SURFACE(3,3,((#61240,#61241,#61242,#61243,#61244,#61245,#61246,
#61247,#61248,#61249,#61250),(#61251,#61252,#61253,#61254,#61255,#61256,
#61257,#61258,#61259,#61260,#61261),(#61262,#61263,#61264,#61265,#61266,
#61267,#61268,#61269,#61270,#61271,#61272),(#61273,#61274,#61275,#61276,
#61277,#61278,#61279,#61280,#61281,#61282,#61283)),.UNSPECIFIED.,.F.,.F.,
 .F.)
B_SPLINE_SURFACE_WITH_KNOTS((4,4),(4,1,1,1,1,1,1,1,4),(0.0434902479384873,
0.93850620438699),(-0.009351371213917,0.,0.1428545029,0.2856984060337,0.4287781897902,
0.5720429752755,0.7151346717899,0.857843506892,0.9437353739471),
 .UNSPECIFIED.)
GEOMETRIC_REPRESENTATION_ITEM()
RATIONAL_B_SPLINE_SURFACE(((1.12844253916938,1.12844253916938,1.12844253916938,
1.12844253916938,1.12844253916938,1.12844253916938,1.12844253916938,1.12844253916938,
1.12844253916938,1.12844253916938,1.12844253916938),(0.960562778259995,
0.960562778259995,0.960562778259995,0.960562778259995,0.960562778259995,
0.960562778259995,0.960562778259995,0.960562778259995,0.960562778259995,
0.960562778259995,0.960562778259995),(0.957252409461222,0.957252409461222,
0.957252409461222,0.957252409461222,0.957252409461222,0.957252409461222,
0.957252409461222,0.957252409461222,0.957252409461222,0.957252409461222,
0.957252409461222),(1.11851143277306,1.11851143277306,1.11851143277306,
1.11851143277306,1.11851143277306,1.11851143277306,1.11851143277306,1.11851143277306,
1.11851143277306,1.11851143277306,1.11851143277306)))
REPRESENTATION_ITEM('')
SURFACE()
);
#504=(
BOUNDED_SURFACE()
B_SPLINE_SURFACE(3,3,((#61433,#61434,#61435,#61436,#61437,#61438),(#61439,
#61440,#61441,#61442,#61443,#61444),(#61445,#61446,#61447,#61448,#61449,
#61450),(#61451,#61452,#61453,#61454,#61455,#61456)),.UNSPECIFIED.,.F.,
 .F.,.F.)
B_SPLINE_SURFACE_WITH_KNOTS((4,4),(4,1,1,4),(0.0606720801571683,0.938680239727398),
(-1.E-5,0.,0.3336142546261,0.663356363362683),.UNSPECIFIED.)
GEOMETRIC_REPRESENTATION_ITEM()
RATIONAL_B_SPLINE_SURFACE(((1.17463054351817,1.17463054351817,1.17463054351817,
1.17463054351817,1.17463054351817,1.17463054351817),(0.941961451792975,
0.941961451792975,0.941961451792975,0.941961451792975,0.941961451792975,
0.941961451792975),(0.941789945342576,0.941789945342576,0.941789945342576,
0.941789945342576,0.941789945342576,0.941789945342576),(1.17411602416697,
1.17411602416697,1.17411602416697,1.17411602416697,1.17411602416697,1.17411602416697)))
REPRESENTATION_ITEM('')
SURFACE()
);
#505=(
BOUNDED_SURFACE()
B_SPLINE_SURFACE(3,3,((#61466,#61467,#61468,#61469,#61470,#61471,#61472,
#61473,#61474,#61475,#61476,#61477,#61478,#61479,#61480,#61481),(#61482,
#61483,#61484,#61485,#61486,#61487,#61488,#61489,#61490,#61491,#61492,#61493,
#61494,#61495,#61496,#61497),(#61498,#61499,#61500,#61501,#61502,#61503,
#61504,#61505,#61506,#61507,#61508,#61509,#61510,#61511,#61512,#61513),
(#61514,#61515,#61516,#61517,#61518,#61519,#61520,#61521,#61522,#61523,
#61524,#61525,#61526,#61527,#61528,#61529)),.UNSPECIFIED.,.F.,.F.,.F.)
B_SPLINE_SURFACE_WITH_KNOTS((4,4),(4,1,1,1,1,1,1,1,1,1,1,1,1,4),(0.0608897632428477,
0.933027487588604),(-0.009395290939728,0.,0.07535337983447,0.1579196834309,
0.2496881956056,0.3528403343846,0.4595186573857,0.5578775090873,0.6478305660607,
0.7283130931759,0.8001423204479,0.8679419821683,0.9343337192845,0.9520744430929),
 .UNSPECIFIED.)
GEOMETRIC_REPRESENTATION_ITEM()
RATIONAL_B_SPLINE_SURFACE(((1.07730271481584,1.07730271481584,1.07730271481584,
1.07730271481584,1.07730271481584,1.07730271481584,1.07730271481584,1.07730271481584,
1.07730271481584,1.07730271481584,1.07730271481584,1.07730271481584,1.07730271481584,
1.07730271481584,1.07730271481584,1.07730271481584),(0.974946315986727,
0.974946315986727,0.974946315986727,0.974946315986727,0.974946315986727,
0.974946315986727,0.974946315986727,0.974946315986727,0.974946315986727,
0.974946315986727,0.974946315986727,0.974946315986727,0.974946315986727,
0.974946315986727,0.974946315986727,0.974946315986727),(0.974237372938085,
0.974237372938085,0.974237372938085,0.974237372938085,0.974237372938085,
0.974237372938085,0.974237372938085,0.974237372938085,0.974237372938085,
0.974237372938085,0.974237372938085,0.974237372938085,0.974237372938085,
0.974237372938085,0.974237372938085,0.974237372938085),(1.07517588566991,
1.07517588566991,1.07517588566991,1.07517588566991,1.07517588566991,1.07517588566991,
1.07517588566991,1.07517588566991,1.07517588566991,1.07517588566991,1.07517588566991,
1.07517588566991,1.07517588566991,1.07517588566991,1.07517588566991,1.07517588566991)))
REPRESENTATION_ITEM('')
SURFACE()
);
#506=(
BOUNDED_SURFACE()
B_SPLINE_SURFACE(3,3,((#61996,#61997,#61998,#61999,#62000,#62001,#62002,
#62003,#62004,#62005),(#62006,#62007,#62008,#62009,#62010,#62011,#62012,
#62013,#62014,#62015),(#62016,#62017,#62018,#62019,#62020,#62021,#62022,
#62023,#62024,#62025),(#62026,#62027,#62028,#62029,#62030,#62031,#62032,
#62033,#62034,#62035)),.UNSPECIFIED.,.F.,.F.,.F.)
B_SPLINE_SURFACE_WITH_KNOTS((4,4),(4,1,1,1,1,1,1,4),(0.0329440013745224,
0.967052315169442),(0.2245728991605,0.2654375946881,0.3544413771844,0.4511118902311,
0.549022999066,0.6456758358933,0.7346467284996,0.775427045264),
 .UNSPECIFIED.)
GEOMETRIC_REPRESENTATION_ITEM()
RATIONAL_B_SPLINE_SURFACE(((1.22228338242005,1.22228338242005,1.22228338242005,
1.22228338242005,1.22228338242005,1.22228338242005,1.22228338242005,1.22228338242005,
1.22228338242005,1.22228338242005),(0.925906707891112,0.925906707891112,
0.925906707891112,0.925906707891112,0.925906707891112,0.925906707891112,
0.925906707891112,0.925906707891112,0.925906707891112,0.925906707891112),
(0.925905539197793,0.925905539197793,0.925905539197793,0.925905539197793,
0.925905539197793,0.925905539197793,0.925905539197793,0.925905539197793,
0.925905539197793,0.925905539197793),(1.22227987634009,1.22227987634009,
1.22227987634009,1.22227987634009,1.22227987634009,1.22227987634009,1.22227987634009,
1.22227987634009,1.22227987634009,1.22227987634009)))
REPRESENTATION_ITEM('')
SURFACE()
);
#507=(
BOUNDED_SURFACE()
B_SPLINE_SURFACE(3,3,((#62123,#62124,#62125,#62126,#62127,#62128,#62129,
#62130,#62131,#62132),(#62133,#62134,#62135,#62136,#62137,#62138,#62139,
#62140,#62141,#62142),(#62143,#62144,#62145,#62146,#62147,#62148,#62149,
#62150,#62151,#62152),(#62153,#62154,#62155,#62156,#62157,#62158,#62159,
#62160,#62161,#62162)),.UNSPECIFIED.,.F.,.F.,.F.)
B_SPLINE_SURFACE_WITH_KNOTS((4,4),(4,1,1,1,1,1,1,4),(0.0311354311261585,
0.968867350391379),(0.2740335216418,0.3186323860176,0.4287267447046,0.5405493543357,
0.6542631421455,0.769753263817,0.8858807480565,0.922150638721103),
 .UNSPECIFIED.)
GEOMETRIC_REPRESENTATION_ITEM()
RATIONAL_B_SPLINE_SURFACE(((1.22401274089182,1.22401274089182,1.22401274089182,
1.22401274089182,1.22401274089182,1.22401274089182,1.22401274089182,1.22401274089182,
1.22401274089182,1.22401274089182),(0.92532820040589,0.92532820040589,0.92532820040589,
0.92532820040589,0.92532820040589,0.92532820040589,0.92532820040589,0.92532820040589,
0.92532820040589,0.92532820040589),(0.925329086372054,0.925329086372054,
0.925329086372054,0.925329086372054,0.925329086372054,0.925329086372054,
0.925329086372054,0.925329086372054,0.925329086372054,0.925329086372054),
(1.22401539879031,1.22401539879031,1.22401539879031,1.22401539879031,1.22401539879031,
1.22401539879031,1.22401539879031,1.22401539879031,1.22401539879031,1.22401539879031)))
REPRESENTATION_ITEM('')
SURFACE()
);
#508=(
BOUNDED_SURFACE()
B_SPLINE_SURFACE(3,3,((#62276,#62277,#62278,#62279,#62280,#62281,#62282,
#62283,#62284,#62285),(#62286,#62287,#62288,#62289,#62290,#62291,#62292,
#62293,#62294,#62295),(#62296,#62297,#62298,#62299,#62300,#62301,#62302,
#62303,#62304,#62305),(#62306,#62307,#62308,#62309,#62310,#62311,#62312,
#62313,#62314,#62315)),.UNSPECIFIED.,.F.,.F.,.F.)
B_SPLINE_SURFACE_WITH_KNOTS((4,4),(4,1,1,1,1,1,1,4),(0.0418834176682723,
0.963270158916865),(0.03308221537874,0.1426814400664,0.2856169940151,0.4287844248845,
0.5720769017456,0.7151865856598,0.857914401801,0.9460833470526),
 .UNSPECIFIED.)
GEOMETRIC_REPRESENTATION_ITEM()
RATIONAL_B_SPLINE_SURFACE(((1.13002825352558,1.13002825352558,1.13002825352558,
1.13002825352558,1.13002825352558,1.13002825352558,1.13002825352558,1.13002825352558,
1.13002825352558,1.13002825352558),(0.955682081384098,0.955682081384098,
0.955682081384098,0.955682081384098,0.955682081384098,0.955682081384098,
0.955682081384098,0.955682081384098,0.955682081384098,0.955682081384098),
(0.95666273389168,0.95666273389168,0.95666273389168,0.95666273389168,0.95666273389168,
0.95666273389168,0.95666273389168,0.95666273389168,0.95666273389168,0.95666273389168),
(1.13297021104833,1.13297021104833,1.13297021104833,1.13297021104833,1.13297021104833,
1.13297021104833,1.13297021104833,1.13297021104833,1.13297021104833,1.13297021104833)))
REPRESENTATION_ITEM('')
SURFACE()
);
#509=(
BOUNDED_SURFACE()
B_SPLINE_SURFACE(3,3,((#62411,#62412,#62413,#62414,#62415,#62416,#62417,
#62418,#62419,#62420),(#62421,#62422,#62423,#62424,#62425,#62426,#62427,
#62428,#62429,#62430),(#62431,#62432,#62433,#62434,#62435,#62436,#62437,
#62438,#62439,#62440),(#62441,#62442,#62443,#62444,#62445,#62446,#62447,
#62448,#62449,#62450)),.UNSPECIFIED.,.F.,.F.,.F.)
B_SPLINE_SURFACE_WITH_KNOTS((4,4),(4,1,1,1,1,1,1,4),(0.0506807378443564,
0.94932028223993),(0.0780685614205442,0.1141112037554,0.2302382189757,0.3457306297879,
0.4594466176023,0.5712706666257,0.681366169875,0.714773732635213),
 .UNSPECIFIED.)
GEOMETRIC_REPRESENTATION_ITEM()
RATIONAL_B_SPLINE_SURFACE(((1.20572543061212,1.20572543061212,1.20572543061212,
1.20572543061212,1.20572543061212,1.20572543061212,1.20572543061212,1.20572543061212,
1.20572543061212,1.20572543061212),(0.931424545091861,0.931424545091861,
0.931424545091861,0.931424545091861,0.931424545091861,0.931424545091861,
0.931424545091861,0.931424545091861,0.931424545091861,0.931424545091861),
(0.931424856462914,0.931424856462914,0.931424856462914,0.931424856462914,
0.931424856462914,0.931424856462914,0.931424856462914,0.931424856462914,
0.931424856462914,0.931424856462914),(1.20572636472528,1.20572636472528,
1.20572636472528,1.20572636472528,1.20572636472528,1.20572636472528,1.20572636472528,
1.20572636472528,1.20572636472528,1.20572636472528)))
REPRESENTATION_ITEM('')
SURFACE()
);
#510=(
BOUNDED_SURFACE()
B_SPLINE_SURFACE(3,3,((#62598,#62599,#62600,#62601,#62602,#62603,#62604,
#62605,#62606,#62607),(#62608,#62609,#62610,#62611,#62612,#62613,#62614,
#62615,#62616,#62617),(#62618,#62619,#62620,#62621,#62622,#62623,#62624,
#62625,#62626,#62627),(#62628,#62629,#62630,#62631,#62632,#62633,#62634,
#62635,#62636,#62637)),.UNSPECIFIED.,.F.,.F.,.F.)
B_SPLINE_SURFACE_WITH_KNOTS((4,4),(4,1,1,1,1,1,1,4),(0.0418856368296952,
0.963268780585969),(0.05391635097625,0.1420855982353,0.2848134143608,0.4279230982548,
0.5712155751054,0.7143830059727,0.8573185599327,0.9669169090934),
 .UNSPECIFIED.)
GEOMETRIC_REPRESENTATION_ITEM()
RATIONAL_B_SPLINE_SURFACE(((1.13002699821861,1.13002699821861,1.13002699821861,
1.13002699821861,1.13002699821861,1.13002699821861,1.13002699821861,1.13002699821861,
1.13002699821861,1.13002699821861),(0.955682345407873,0.955682345407873,
0.955682345407873,0.955682345407873,0.955682345407873,0.955682345407873,
0.955682345407873,0.955682345407873,0.955682345407873,0.955682345407873),
(0.956663154117468,0.956663154117468,0.956663154117468,0.956663154117468,
0.956663154117468,0.956663154117468,0.956663154117468,0.956663154117468,
0.956663154117468,0.956663154117468),(1.13296942434739,1.13296942434739,
1.13296942434739,1.13296942434739,1.13296942434739,1.13296942434739,1.13296942434739,
1.13296942434739,1.13296942434739,1.13296942434739)))
REPRESENTATION_ITEM('')
SURFACE()
);
#511=(
BOUNDED_SURFACE()
B_SPLINE_SURFACE(3,3,((#62791,#62792,#62793,#62794,#62795,#62796),(#62797,
#62798,#62799,#62800,#62801,#62802),(#62803,#62804,#62805,#62806,#62807,
#62808),(#62809,#62810,#62811,#62812,#62813,#62814)),.UNSPECIFIED.,.F.,
 .F.,.F.)
B_SPLINE_SURFACE_WITH_KNOTS((4,4),(4,1,1,4),(0.0606070589512044,0.9394900012978),
(0.199119623412498,0.3331969354622,0.6668030645378,0.800880381046923),
 .UNSPECIFIED.)
GEOMETRIC_REPRESENTATION_ITEM()
RATIONAL_B_SPLINE_SURFACE(((1.17469014882262,1.17469014882262,1.17469014882262,
1.17469014882262,1.17469014882262,1.17469014882262),(0.941744224794448,
0.941744224794448,0.941744224794448,0.941744224794448,0.941744224794448,
0.941744224794448),(0.941769953233938,0.941769953233938,0.941769953233937,
0.941769953233937,0.941769953233937,0.941769953233937),(1.17476733414109,
1.17476733414109,1.17476733414109,1.17476733414109,1.17476733414109,1.17476733414109)))
REPRESENTATION_ITEM('')
SURFACE()
);
#512=(
BOUNDED_SURFACE()
B_SPLINE_SURFACE(3,3,((#63081,#63082,#63083,#63084,#63085,#63086,#63087,
#63088,#63089,#63090,#63091,#63092,#63093,#63094,#63095,#63096,#63097,#63098,
#63099,#63100),(#63101,#63102,#63103,#63104,#63105,#63106,#63107,#63108,
#63109,#63110,#63111,#63112,#63113,#63114,#63115,#63116,#63117,#63118,#63119,
#63120),(#63121,#63122,#63123,#63124,#63125,#63126,#63127,#63128,#63129,
#63130,#63131,#63132,#63133,#63134,#63135,#63136,#63137,#63138,#63139,#63140),
(#63141,#63142,#63143,#63144,#63145,#63146,#63147,#63148,#63149,#63150,
#63151,#63152,#63153,#63154,#63155,#63156,#63157,#63158,#63159,#63160)),
 .UNSPECIFIED.,.F.,.F.,.F.)
B_SPLINE_SURFACE_WITH_KNOTS((4,4),(4,1,1,1,1,1,1,1,1,1,1,1,1,1,1,1,1,4),
(0.0633076409949893,0.939204474105228),(-0.009153831281455,0.,0.07546620931579,
0.1557174957677,0.2403996005821,0.3291522597982,0.4125162510435,0.4856766709034,
0.5506589911205,0.6094498872342,0.6638185572398,0.7128092494438,0.7565100470699,
0.7968460585168,0.8357686456417,0.87488860494,0.9149305605777,0.9275319404913),
 .UNSPECIFIED.)
GEOMETRIC_REPRESENTATION_ITEM()
RATIONAL_B_SPLINE_SURFACE(((1.07645083767944,1.07645083767944,1.07645083767944,
1.07645083767944,1.07645083767944,1.07645083767944,1.07645083767944,1.07645083767944,
1.07645083767944,1.07645083767944,1.07645083767944,1.07645083767944,1.07645083767944,
1.07645083767944,1.07645083767944,1.07645083767944,1.07645083767944,1.07645083767944,
1.07645083767944,1.07645083767944),(0.974223193540317,0.974223193540317,
0.974223193540317,0.974223193540317,0.974223193540317,0.974223193540317,
0.974223193540317,0.974223193540317,0.974223193540317,0.974223193540317,
0.974223193540317,0.974223193540317,0.974223193540317,0.974223193540317,
0.974223193540317,0.974223193540317,0.974223193540317,0.974223193540317,
0.974223193540317,0.974223193540317),(0.974517230753478,0.974517230753478,
0.974517230753478,0.974517230753478,0.974517230753478,0.974517230753478,
0.974517230753478,0.974517230753478,0.974517230753478,0.974517230753478,
0.974517230753478,0.974517230753478,0.974517230753478,0.974517230753478,
0.974517230753478,0.974517230753478,0.974517230753478,0.974517230753478,
0.974517230753478,0.974517230753478),(1.07733294931892,1.07733294931892,
1.07733294931892,1.07733294931892,1.07733294931892,1.07733294931892,1.07733294931892,
1.07733294931892,1.07733294931892,1.07733294931892,1.07733294931892,1.07733294931892,
1.07733294931892,1.07733294931892,1.07733294931892,1.07733294931892,1.07733294931892,
1.07733294931892,1.07733294931892,1.07733294931892)))
REPRESENTATION_ITEM('')
SURFACE()
);
#513=(
BOUNDED_SURFACE()
B_SPLINE_SURFACE(3,3,((#63322,#63323,#63324,#63325,#63326,#63327,#63328,
#63329,#63330,#63331),(#63332,#63333,#63334,#63335,#63336,#63337,#63338,
#63339,#63340,#63341),(#63342,#63343,#63344,#63345,#63346,#63347,#63348,
#63349,#63350,#63351),(#63352,#63353,#63354,#63355,#63356,#63357,#63358,
#63359,#63360,#63361)),.UNSPECIFIED.,.F.,.F.,.F.)
B_SPLINE_SURFACE_WITH_KNOTS((4,4),(4,1,1,1,1,1,1,4),(0.0543118686704758,
0.946617716449823),(0.289640600847592,0.3185583158377,0.428651361796,0.5404783317088,
0.654204063309,0.7697110119304,0.8858550830104,0.922057258249154),
 .UNSPECIFIED.)
GEOMETRIC_REPRESENTATION_ITEM()
RATIONAL_B_SPLINE_SURFACE(((1.20241792264148,1.20241792264148,1.20241792264148,
1.20241792264148,1.20241792264148,1.20241792264148,1.20241792264148,1.20241792264148,
1.20241792264148,1.20241792264148),(0.932245899692698,0.932245899692698,
0.932245899692698,0.932245899692698,0.932245899692698,0.932245899692698,
0.932245899692698,0.932245899692698,0.932245899692698,0.932245899692698),
(0.932527652643697,0.932527652643697,0.932527652643697,0.932527652643697,
0.932527652643697,0.932527652643697,0.932527652643697,0.932527652643697,
0.932527652643697,0.932527652643697),(1.20326318149447,1.20326318149447,
1.20326318149447,1.20326318149447,1.20326318149447,1.20326318149447,1.20326318149447,
1.20326318149447,1.20326318149447,1.20326318149447)))
REPRESENTATION_ITEM('')
SURFACE()
);
#514=(
BOUNDED_SURFACE()
B_SPLINE_SURFACE(3,3,((#63475,#63476,#63477,#63478,#63479,#63480,#63481,
#63482,#63483,#63484,#63485),(#63486,#63487,#63488,#63489,#63490,#63491,
#63492,#63493,#63494,#63495,#63496),(#63497,#63498,#63499,#63500,#63501,
#63502,#63503,#63504,#63505,#63506,#63507),(#63508,#63509,#63510,#63511,
#63512,#63513,#63514,#63515,#63516,#63517,#63518)),.UNSPECIFIED.,.F.,.F.,
 .F.)
B_SPLINE_SURFACE_WITH_KNOTS((4,4),(4,1,1,1,1,1,1,1,4),(0.0595203863462284,
0.938436205671232),(0.05105962729005,0.1243084941807,0.2492353165502,0.3744835129416,
0.4998949769261,0.6253220276845,0.7506164023093,0.8756120170229,0.9160299525996),
 .UNSPECIFIED.)
GEOMETRIC_REPRESENTATION_ITEM()
RATIONAL_B_SPLINE_SURFACE(((1.11958055537369,1.11958055537369,1.11958055537369,
1.11958055537369,1.11958055537369,1.11958055537369,1.11958055537369,1.11958055537369,
1.11958055537369,1.11958055537369,1.11958055537369),(0.96050964184567,0.96050964184567,
0.96050964184567,0.96050964184567,0.96050964184567,0.96050964184567,0.96050964184567,
0.96050964184567,0.96050964184567,0.96050964184567,0.96050964184567),(0.960140672698838,
0.960140672698838,0.960140672698838,0.960140672698838,0.960140672698838,
0.960140672698838,0.960140672698838,0.960140672698838,0.960140672698838,
0.960140672698838,0.960140672698838),(1.1184736479332,1.1184736479332,1.1184736479332,
1.1184736479332,1.1184736479332,1.1184736479332,1.1184736479332,1.1184736479332,
1.1184736479332,1.1184736479332,1.1184736479332)))
REPRESENTATION_ITEM('')
SURFACE()
);
#515=(
BOUNDED_SURFACE()
B_SPLINE_SURFACE(3,3,((#63752,#63753,#63754,#63755,#63756,#63757,#63758,
#63759,#63760,#63761),(#63762,#63763,#63764,#63765,#63766,#63767,#63768,
#63769,#63770,#63771),(#63772,#63773,#63774,#63775,#63776,#63777,#63778,
#63779,#63780,#63781),(#63782,#63783,#63784,#63785,#63786,#63787,#63788,
#63789,#63790,#63791)),.UNSPECIFIED.,.F.,.F.,.F.)
B_SPLINE_SURFACE_WITH_KNOTS((4,4),(4,1,1,1,1,1,1,4),(0.0567016135390075,
0.965170855368738),(0.2246119235744,0.2652891204936,0.3542346581807,0.4509283928036,
0.5489344914255,0.6456463447232,0.7346252853759,0.7753865663254),
 .UNSPECIFIED.)
GEOMETRIC_REPRESENTATION_ITEM()
RATIONAL_B_SPLINE_SURFACE(((1.20024622089112,1.20024622089112,1.20024622089112,
1.20024622089112,1.20024622089112,1.20024622089112,1.20024622089112,1.20024622089112,
1.20024622089112,1.20024622089112),(0.926664455909577,0.926664455909577,
0.926664455909577,0.926664455909577,0.926664455909577,0.926664455909577,
0.926664455909577,0.926664455909577,0.926664455909577,0.926664455909577),
(0.933413757092531,0.933413757092531,0.933413757092531,0.933413757092531,
0.933413757092531,0.933413757092531,0.933413757092531,0.933413757092531,
0.933413757092531,0.933413757092531),(1.22049412443998,1.22049412443998,
1.22049412443998,1.22049412443998,1.22049412443998,1.22049412443998,1.22049412443998,
1.22049412443998,1.22049412443998,1.22049412443998)))
REPRESENTATION_ITEM('')
SURFACE()
);
#516=(
BOUNDED_SURFACE()
B_SPLINE_SURFACE(2,2,((#63877,#63878,#63879),(#63880,#63881,#63882),(#63883,
#63884,#63885)),.UNSPECIFIED.,.F.,.F.,.F.)
B_SPLINE_SURFACE_WITH_KNOTS((3,3),(3,3),(-0.316361998869524,0.316361961333282),
(0.571031091629656,0.999765088357377),.UNSPECIFIED.)
GEOMETRIC_REPRESENTATION_ITEM()
RATIONAL_B_SPLINE_SURFACE(((1.,0.977111247736172,1.),(0.950373533316957,
0.928620668954766,0.950373533316957),(1.,0.977111247736172,1.)))
REPRESENTATION_ITEM('')
SURFACE()
);
#517=(
BOUNDED_SURFACE()
B_SPLINE_SURFACE(2,2,((#63888,#63889,#63890),(#63891,#63892,#63893),(#63894,
#63895,#63896)),.UNSPECIFIED.,.F.,.F.,.F.)
B_SPLINE_SURFACE_WITH_KNOTS((3,3),(3,3),(-0.316362027618547,0.316362033179937),
(1.35642916480867,1.78516363636164),.UNSPECIFIED.)
GEOMETRIC_REPRESENTATION_ITEM()
RATIONAL_B_SPLINE_SURFACE(((1.,0.977111197231604,1.),(0.950373517668733,
0.928620605666507,0.950373517668733),(1.,0.977111197231604,1.)))
REPRESENTATION_ITEM('')
SURFACE()
);
#518=(
BOUNDED_SURFACE()
B_SPLINE_SURFACE(2,2,((#63899,#63900,#63901),(#63902,#63903,#63904),(#63905,
#63906,#63907)),.UNSPECIFIED.,.F.,.F.,.F.)
B_SPLINE_SURFACE_WITH_KNOTS((3,3),(3,3),(-0.31636199673171,0.316361977977988),
(2.14182744740588,2.57056168331331),.UNSPECIFIED.)
GEOMETRIC_REPRESENTATION_ITEM()
RATIONAL_B_SPLINE_SURFACE(((1.,0.97711122229594,1.),(0.950373531060328,
0.928620642572066,0.950373531060328),(1.,0.97711122229594,1.)))
REPRESENTATION_ITEM('')
SURFACE()
);
#519=(
BOUNDED_SURFACE()
B_SPLINE_SURFACE(2,2,((#63910,#63911,#63912),(#63913,#63914,#63915),(#63916,
#63917,#63918)),.UNSPECIFIED.,.F.,.F.,.F.)
B_SPLINE_SURFACE_WITH_KNOTS((3,3),(3,3),(-0.316362001159797,0.316362001025874),
(-0.214366972691254,0.214366972691255),.UNSPECIFIED.)
GEOMETRIC_REPRESENTATION_ITEM()
RATIONAL_B_SPLINE_SURFACE(((1.,0.977111253197478,1.),(0.950373526786289,
0.928620667763857,0.950373526786289),(1.,0.977111253197478,1.)))
REPRESENTATION_ITEM('')
SURFACE()
);
#520=(
BOUNDED_SURFACE()
B_SPLINE_SURFACE(2,2,((#63921,#63922,#63923),(#63924,#63925,#63926),(#63927,
#63928,#63929)),.UNSPECIFIED.,.F.,.F.,.F.)
B_SPLINE_SURFACE_WITH_KNOTS((3,3),(3,3),(-0.316362027572333,0.316361999994803),
(-2.57055983293518,-2.14182718056046),.UNSPECIFIED.)
GEOMETRIC_REPRESENTATION_ITEM()
RATIONAL_B_SPLINE_SURFACE(((1.,0.977111390727357,1.),(0.950373522838055,
0.928620794610749,0.950373522838055),(1.,0.977111390727357,1.)))
REPRESENTATION_ITEM('')
SURFACE()
);
#521=(
BOUNDED_SURFACE()
B_SPLINE_SURFACE(2,2,((#63932,#63933,#63934),(#63935,#63936,#63937),(#63938,
#63939,#63940)),.UNSPECIFIED.,.F.,.F.,.F.)
B_SPLINE_SURFACE_WITH_KNOTS((3,3),(3,3),(-0.316361976307064,0.316361980987301),
(-1.78516344737183,-1.35642909114174),.UNSPECIFIED.)
GEOMETRIC_REPRESENTATION_ITEM()
RATIONAL_B_SPLINE_SURFACE(((1.,0.977111209497874,1.),(0.950373533769378,
0.928620633056165,0.950373533769378),(1.,0.977111209497874,1.)))
REPRESENTATION_ITEM('')
SURFACE()
);
#522=(
BOUNDED_SURFACE()
B_SPLINE_SURFACE(2,2,((#63943,#63944,#63945),(#63946,#63947,#63948),(#63949,
#63950,#63951)),.UNSPECIFIED.,.F.,.F.,.F.)
B_SPLINE_SURFACE_WITH_KNOTS((3,3),(3,3),(-0.316361997381232,0.316362033180092),
(-0.999765325442169,-0.571033470390333),.UNSPECIFIED.)
GEOMETRIC_REPRESENTATION_ITEM()
RATIONAL_B_SPLINE_SURFACE(((1.,0.977111475533851,1.),(0.950373522372293,
0.928620874753495,0.950373522372293),(1.,0.977111475533851,1.)))
REPRESENTATION_ITEM('')
SURFACE()
);
#523=(
BOUNDED_SURFACE()
B_SPLINE_SURFACE(2,2,((#63954,#63955,#63956),(#63957,#63958,#63959),(#63960,
#63961,#63962)),.UNSPECIFIED.,.F.,.F.,.F.)
B_SPLINE_SURFACE_WITH_KNOTS((3,3),(3,3),(-0.316361967725758,0.316361973128478),
(-0.2143652338984,0.214367145981156),.UNSPECIFIED.)
GEOMETRIC_REPRESENTATION_ITEM()
RATIONAL_B_SPLINE_SURFACE(((1.,0.977111419711065,1.),(0.950373536326736,
0.928620835336042,0.950373536326736),(1.,0.977111419711065,1.)))
REPRESENTATION_ITEM('')
SURFACE()
);
#1053=SHAPE_REPRESENTATION_RELATIONSHIP('SRR','None',#66916,#1084);
#1084=ADVANCED_BREP_SHAPE_REPRESENTATION('',(#1150),#66707);
#1115=STYLED_ITEM('',(#67095),#1150);
#1150=MANIFOLD_SOLID_BREP('Body1',#25681);
#1393=FACE_BOUND('',#4974,.T.);
#1394=FACE_BOUND('',#4975,.T.);
#1395=FACE_BOUND('',#4976,.T.);
#1396=FACE_BOUND('',#4977,.T.);
#1397=FACE_BOUND('',#4978,.T.);
#1398=FACE_BOUND('',#4987,.T.);
#1399=FACE_BOUND('',#4988,.T.);
#1400=FACE_BOUND('',#4989,.T.);
#1401=FACE_BOUND('',#4990,.T.);
#1402=FACE_BOUND('',#4991,.T.);
#2016=PLANE('',#27715);
#2017=PLANE('',#27719);
#2018=PLANE('',#27915);
#2019=PLANE('',#27919);
#2020=PLANE('',#27923);
#2021=PLANE('',#27927);
#2022=PLANE('',#27931);
#2023=PLANE('',#27935);
#2024=PLANE('',#27939);
#2025=PLANE('',#27943);
#3120=FACE_OUTER_BOUND('',#4787,.T.);
#3121=FACE_OUTER_BOUND('',#4788,.T.);
#3122=FACE_OUTER_BOUND('',#4789,.T.);
#3123=FACE_OUTER_BOUND('',#4790,.T.);
#3124=FACE_OUTER_BOUND('',#4791,.T.);
#3125=FACE_OUTER_BOUND('',#4792,.T.);
#3126=FACE_OUTER_BOUND('',#4793,.T.);
#3127=FACE_OUTER_BOUND('',#4794,.T.);
#3128=FACE_OUTER_BOUND('',#4795,.T.);
#3129=FACE_OUTER_BOUND('',#4796,.T.);
#3130=FACE_OUTER_BOUND('',#4797,.T.);
#3131=FACE_OUTER_BOUND('',#4798,.T.);
#3132=FACE_OUTER_BOUND('',#4799,.T.);
#3133=FACE_OUTER_BOUND('',#4800,.T.);
#3134=FACE_OUTER_BOUND('',#4801,.T.);
#3135=FACE_OUTER_BOUND('',#4802,.T.);
#3136=FACE_OUTER_BOUND('',#4803,.T.);
#3137=FACE_OUTER_BOUND('',#4804,.T.);
#3138=FACE_OUTER_BOUND('',#4805,.T.);
#3139=FACE_OUTER_BOUND('',#4806,.T.);
#3140=FACE_OUTER_BOUND('',#4807,.T.);
#3141=FACE_OUTER_BOUND('',#4808,.T.);
#3142=FACE_OUTER_BOUND('',#4809,.T.);
#3143=FACE_OUTER_BOUND('',#4810,.T.);
#3144=FACE_OUTER_BOUND('',#4811,.T.);
#3145=FACE_OUTER_BOUND('',#4812,.T.);
#3146=FACE_OUTER_BOUND('',#4813,.T.);
#3147=FACE_OUTER_BOUND('',#4814,.T.);
#3148=FACE_OUTER_BOUND('',#4815,.T.);
#3149=FACE_OUTER_BOUND('',#4816,.T.);
#3150=FACE_OUTER_BOUND('',#4817,.T.);
#3151=FACE_OUTER_BOUND('',#4818,.T.);
#3152=FACE_OUTER_BOUND('',#4819,.T.);
#3153=FACE_OUTER_BOUND('',#4820,.T.);
#3154=FACE_OUTER_BOUND('',#4821,.T.);
#3155=FACE_OUTER_BOUND('',#4822,.T.);
#3156=FACE_OUTER_BOUND('',#4823,.T.);
#3157=FACE_OUTER_BOUND('',#4824,.T.);
#3158=FACE_OUTER_BOUND('',#4825,.T.);
#3159=FACE_OUTER_BOUND('',#4826,.T.);
#3160=FACE_OUTER_BOUND('',#4827,.T.);
#3161=FACE_OUTER_BOUND('',#4828,.T.);
#3162=FACE_OUTER_BOUND('',#4829,.T.);
#3163=FACE_OUTER_BOUND('',#4830,.T.);
#3164=FACE_OUTER_BOUND('',#4831,.T.);
#3165=FACE_OUTER_BOUND('',#4832,.T.);
#3166=FACE_OUTER_BOUND('',#4833,.T.);
#3167=FACE_OUTER_BOUND('',#4834,.T.);
#3168=FACE_OUTER_BOUND('',#4835,.T.);
#3169=FACE_OUTER_BOUND('',#4836,.T.);
#3170=FACE_OUTER_BOUND('',#4837,.T.);
#3171=FACE_OUTER_BOUND('',#4838,.T.);
#3172=FACE_OUTER_BOUND('',#4839,.T.);
#3173=FACE_OUTER_BOUND('',#4840,.T.);
#3174=FACE_OUTER_BOUND('',#4841,.T.);
#3175=FACE_OUTER_BOUND('',#4842,.T.);
#3176=FACE_OUTER_BOUND('',#4843,.T.);
#3177=FACE_OUTER_BOUND('',#4844,.T.);
#3178=FACE_OUTER_BOUND('',#4845,.T.);
#3179=FACE_OUTER_BOUND('',#4846,.T.);
#3180=FACE_OUTER_BOUND('',#4847,.T.);
#3181=FACE_OUTER_BOUND('',#4848,.T.);
#3182=FACE_OUTER_BOUND('',#4849,.T.);
#3183=FACE_OUTER_BOUND('',#4850,.T.);
#3184=FACE_OUTER_BOUND('',#4851,.T.);
#3185=FACE_OUTER_BOUND('',#4852,.T.);
#3186=FACE_OUTER_BOUND('',#4853,.T.);
#3187=FACE_OUTER_BOUND('',#4854,.T.);
#3188=FACE_OUTER_BOUND('',#4855,.T.);
#3189=FACE_OUTER_BOUND('',#4856,.T.);
#3190=FACE_OUTER_BOUND('',#4857,.T.);
#3191=FACE_OUTER_BOUND('',#4858,.T.);
#3192=FACE_OUTER_BOUND('',#4859,.T.);
#3193=FACE_OUTER_BOUND('',#4860,.T.);
#3194=FACE_OUTER_BOUND('',#4861,.T.);
#3195=FACE_OUTER_BOUND('',#4862,.T.);
#3196=FACE_OUTER_BOUND('',#4863,.T.);
#3197=FACE_OUTER_BOUND('',#4864,.T.);
#3198=FACE_OUTER_BOUND('',#4865,.T.);
#3199=FACE_OUTER_BOUND('',#4866,.T.);
#3200=FACE_OUTER_BOUND('',#4867,.T.);
#3201=FACE_OUTER_BOUND('',#4868,.T.);
#3202=FACE_OUTER_BOUND('',#4869,.T.);
#3203=FACE_OUTER_BOUND('',#4870,.T.);
#3204=FACE_OUTER_BOUND('',#4871,.T.);
#3205=FACE_OUTER_BOUND('',#4872,.T.);
#3206=FACE_OUTER_BOUND('',#4873,.T.);
#3207=FACE_OUTER_BOUND('',#4874,.T.);
#3208=FACE_OUTER_BOUND('',#4875,.T.);
#3209=FACE_OUTER_BOUND('',#4876,.T.);
#3210=FACE_OUTER_BOUND('',#4877,.T.);
#3211=FACE_OUTER_BOUND('',#4878,.T.);
#3212=FACE_OUTER_BOUND('',#4879,.T.);
#3213=FACE_OUTER_BOUND('',#4880,.T.);
#3214=FACE_OUTER_BOUND('',#4881,.T.);
#3215=FACE_OUTER_BOUND('',#4882,.T.);
#3216=FACE_OUTER_BOUND('',#4883,.T.);
#3217=FACE_OUTER_BOUND('',#4884,.T.);
#3218=FACE_OUTER_BOUND('',#4885,.T.);
#3219=FACE_OUTER_BOUND('',#4886,.T.);
#3220=FACE_OUTER_BOUND('',#4887,.T.);
#3221=FACE_OUTER_BOUND('',#4888,.T.);
#3222=FACE_OUTER_BOUND('',#4889,.T.);
#3223=FACE_OUTER_BOUND('',#4890,.T.);
#3224=FACE_OUTER_BOUND('',#4891,.T.);
#3225=FACE_OUTER_BOUND('',#4892,.T.);
#3226=FACE_OUTER_BOUND('',#4893,.T.);
#3227=FACE_OUTER_BOUND('',#4894,.T.);
#3228=FACE_OUTER_BOUND('',#4895,.T.);
#3229=FACE_OUTER_BOUND('',#4896,.T.);
#3230=FACE_OUTER_BOUND('',#4897,.T.);
#3231=FACE_OUTER_BOUND('',#4898,.T.);
#3232=FACE_OUTER_BOUND('',#4899,.T.);
#3233=FACE_OUTER_BOUND('',#4900,.T.);
#3234=FACE_OUTER_BOUND('',#4901,.T.);
#3235=FACE_OUTER_BOUND('',#4902,.T.);
#3236=FACE_OUTER_BOUND('',#4903,.T.);
#3237=FACE_OUTER_BOUND('',#4904,.T.);
#3238=FACE_OUTER_BOUND('',#4905,.T.);
#3239=FACE_OUTER_BOUND('',#4906,.T.);
#3240=FACE_OUTER_BOUND('',#4907,.T.);
#3241=FACE_OUTER_BOUND('',#4908,.T.);
#3242=FACE_OUTER_BOUND('',#4909,.T.);
#3243=FACE_OUTER_BOUND('',#4910,.T.);
#3244=FACE_OUTER_BOUND('',#4911,.T.);
#3245=FACE_OUTER_BOUND('',#4912,.T.);
#3246=FACE_OUTER_BOUND('',#4913,.T.);
#3247=FACE_OUTER_BOUND('',#4914,.T.);
#3248=FACE_OUTER_BOUND('',#4915,.T.);
#3249=FACE_OUTER_BOUND('',#4916,.T.);
#3250=FACE_OUTER_BOUND('',#4917,.T.);
#3251=FACE_OUTER_BOUND('',#4918,.T.);
#3252=FACE_OUTER_BOUND('',#4919,.T.);
#3253=FACE_OUTER_BOUND('',#4920,.T.);
#3254=FACE_OUTER_BOUND('',#4921,.T.);
#3255=FACE_OUTER_BOUND('',#4922,.T.);
#3256=FACE_OUTER_BOUND('',#4923,.T.);
#3257=FACE_OUTER_BOUND('',#4924,.T.);
#3258=FACE_OUTER_BOUND('',#4925,.T.);
#3259=FACE_OUTER_BOUND('',#4926,.T.);
#3260=FACE_OUTER_BOUND('',#4927,.T.);
#3261=FACE_OUTER_BOUND('',#4928,.T.);
#3262=FACE_OUTER_BOUND('',#4929,.T.);
#3263=FACE_OUTER_BOUND('',#4930,.T.);
#3264=FACE_OUTER_BOUND('',#4931,.T.);
#3265=FACE_OUTER_BOUND('',#4932,.T.);
#3266=FACE_OUTER_BOUND('',#4933,.T.);
#3267=FACE_OUTER_BOUND('',#4934,.T.);
#3268=FACE_OUTER_BOUND('',#4935,.T.);
#3269=FACE_OUTER_BOUND('',#4936,.T.);
#3270=FACE_OUTER_BOUND('',#4937,.T.);
#3271=FACE_OUTER_BOUND('',#4938,.T.);
#3272=FACE_OUTER_BOUND('',#4939,.T.);
#3273=FACE_OUTER_BOUND('',#4940,.T.);
#3274=FACE_OUTER_BOUND('',#4941,.T.);
#3275=FACE_OUTER_BOUND('',#4942,.T.);
#3276=FACE_OUTER_BOUND('',#4943,.T.);
#3277=FACE_OUTER_BOUND('',#4944,.T.);
#3278=FACE_OUTER_BOUND('',#4945,.T.);
#3279=FACE_OUTER_BOUND('',#4946,.T.);
#3280=FACE_OUTER_BOUND('',#4947,.T.);
#3281=FACE_OUTER_BOUND('',#4948,.T.);
#3282=FACE_OUTER_BOUND('',#4949,.T.);
#3283=FACE_OUTER_BOUND('',#4950,.T.);
#3284=FACE_OUTER_BOUND('',#4951,.T.);
#3285=FACE_OUTER_BOUND('',#4952,.T.);
#3286=FACE_OUTER_BOUND('',#4953,.T.);
#3287=FACE_OUTER_BOUND('',#4954,.T.);
#3288=FACE_OUTER_BOUND('',#4955,.T.);
#3289=FACE_OUTER_BOUND('',#4956,.T.);
#3290=FACE_OUTER_BOUND('',#4957,.T.);
#3291=FACE_OUTER_BOUND('',#4958,.T.);
#3292=FACE_OUTER_BOUND('',#4959,.T.);
#3293=FACE_OUTER_BOUND('',#4960,.T.);
#3294=FACE_OUTER_BOUND('',#4961,.T.);
#3295=FACE_OUTER_BOUND('',#4962,.T.);
#3296=FACE_OUTER_BOUND('',#4963,.T.);
#3297=FACE_OUTER_BOUND('',#4964,.T.);
#3298=FACE_OUTER_BOUND('',#4965,.T.);
#3299=FACE_OUTER_BOUND('',#4966,.T.);
#3300=FACE_OUTER_BOUND('',#4967,.T.);
#3301=FACE_OUTER_BOUND('',#4968,.T.);
#3302=FACE_OUTER_BOUND('',#4969,.T.);
#3303=FACE_OUTER_BOUND('',#4970,.T.);
#3304=FACE_OUTER_BOUND('',#4971,.T.);
#3305=FACE_OUTER_BOUND('',#4972,.T.);
#3306=FACE_OUTER_BOUND('',#4973,.T.);
#3307=FACE_OUTER_BOUND('',#4979,.T.);
#3308=FACE_OUTER_BOUND('',#4980,.T.);
#3309=FACE_OUTER_BOUND('',#4981,.T.);
#3310=FACE_OUTER_BOUND('',#4982,.T.);
#3311=FACE_OUTER_BOUND('',#4983,.T.);
#3312=FACE_OUTER_BOUND('',#4984,.T.);
#3313=FACE_OUTER_BOUND('',#4985,.T.);
#3314=FACE_OUTER_BOUND('',#4986,.T.);
#4787=EDGE_LOOP('',(#21072));
#4788=EDGE_LOOP('',(#21073,#21074,#21075,#21076));
#4789=EDGE_LOOP('',(#21077));
#4790=EDGE_LOOP('',(#21078,#21079,#21080,#21081));
#4791=EDGE_LOOP('',(#21082,#21083,#21084,#21085));
#4792=EDGE_LOOP('',(#21086,#21087,#21088,#21089));
#4793=EDGE_LOOP('',(#21090,#21091,#21092,#21093));
#4794=EDGE_LOOP('',(#21094,#21095,#21096));
#4795=EDGE_LOOP('',(#21097,#21098,#21099,#21100));
#4796=EDGE_LOOP('',(#21101,#21102,#21103,#21104));
#4797=EDGE_LOOP('',(#21105,#21106,#21107,#21108));
#4798=EDGE_LOOP('',(#21109,#21110,#21111,#21112));
#4799=EDGE_LOOP('',(#21113,#21114,#21115,#21116));
#4800=EDGE_LOOP('',(#21117,#21118,#21119));
#4801=EDGE_LOOP('',(#21120,#21121,#21122,#21123));
#4802=EDGE_LOOP('',(#21124,#21125,#21126,#21127));
#4803=EDGE_LOOP('',(#21128,#21129,#21130));
#4804=EDGE_LOOP('',(#21131,#21132,#21133,#21134));
#4805=EDGE_LOOP('',(#21135,#21136,#21137,#21138));
#4806=EDGE_LOOP('',(#21139,#21140,#21141,#21142));
#4807=EDGE_LOOP('',(#21143,#21144,#21145));
#4808=EDGE_LOOP('',(#21146,#21147,#21148,#21149));
#4809=EDGE_LOOP('',(#21150,#21151,#21152,#21153));
#4810=EDGE_LOOP('',(#21154,#21155,#21156,#21157));
#4811=EDGE_LOOP('',(#21158,#21159,#21160,#21161));
#4812=EDGE_LOOP('',(#21162,#21163,#21164,#21165));
#4813=EDGE_LOOP('',(#21166,#21167,#21168,#21169));
#4814=EDGE_LOOP('',(#21170,#21171,#21172,#21173));
#4815=EDGE_LOOP('',(#21174,#21175,#21176));
#4816=EDGE_LOOP('',(#21177,#21178,#21179,#21180));
#4817=EDGE_LOOP('',(#21181,#21182,#21183,#21184));
#4818=EDGE_LOOP('',(#21185,#21186,#21187,#21188));
#4819=EDGE_LOOP('',(#21189,#21190,#21191,#21192));
#4820=EDGE_LOOP('',(#21193,#21194,#21195,#21196));
#4821=EDGE_LOOP('',(#21197,#21198,#21199));
#4822=EDGE_LOOP('',(#21200,#21201,#21202,#21203));
#4823=EDGE_LOOP('',(#21204,#21205,#21206,#21207));
#4824=EDGE_LOOP('',(#21208,#21209,#21210));
#4825=EDGE_LOOP('',(#21211,#21212,#21213,#21214));
#4826=EDGE_LOOP('',(#21215,#21216,#21217,#21218));
#4827=EDGE_LOOP('',(#21219,#21220,#21221,#21222));
#4828=EDGE_LOOP('',(#21223,#21224,#21225));
#4829=EDGE_LOOP('',(#21226,#21227,#21228,#21229));
#4830=EDGE_LOOP('',(#21230,#21231,#21232,#21233));
#4831=EDGE_LOOP('',(#21234,#21235,#21236,#21237));
#4832=EDGE_LOOP('',(#21238,#21239,#21240,#21241));
#4833=EDGE_LOOP('',(#21242,#21243,#21244,#21245));
#4834=EDGE_LOOP('',(#21246,#21247,#21248,#21249));
#4835=EDGE_LOOP('',(#21250,#21251,#21252,#21253));
#4836=EDGE_LOOP('',(#21254,#21255,#21256));
#4837=EDGE_LOOP('',(#21257,#21258,#21259,#21260));
#4838=EDGE_LOOP('',(#21261,#21262,#21263,#21264));
#4839=EDGE_LOOP('',(#21265,#21266,#21267,#21268));
#4840=EDGE_LOOP('',(#21269,#21270,#21271,#21272));
#4841=EDGE_LOOP('',(#21273,#21274,#21275,#21276));
#4842=EDGE_LOOP('',(#21277,#21278,#21279));
#4843=EDGE_LOOP('',(#21280,#21281,#21282,#21283));
#4844=EDGE_LOOP('',(#21284,#21285,#21286,#21287));
#4845=EDGE_LOOP('',(#21288,#21289,#21290));
#4846=EDGE_LOOP('',(#21291,#21292,#21293,#21294));
#4847=EDGE_LOOP('',(#21295,#21296,#21297,#21298));
#4848=EDGE_LOOP('',(#21299,#21300,#21301,#21302));
#4849=EDGE_LOOP('',(#21303,#21304,#21305));
#4850=EDGE_LOOP('',(#21306,#21307,#21308,#21309));
#4851=EDGE_LOOP('',(#21310,#21311,#21312,#21313));
#4852=EDGE_LOOP('',(#21314,#21315,#21316,#21317));
#4853=EDGE_LOOP('',(#21318,#21319,#21320,#21321));
#4854=EDGE_LOOP('',(#21322,#21323,#21324,#21325));
#4855=EDGE_LOOP('',(#21326,#21327,#21328,#21329));
#4856=EDGE_LOOP('',(#21330,#21331,#21332,#21333));
#4857=EDGE_LOOP('',(#21334,#21335,#21336));
#4858=EDGE_LOOP('',(#21337,#21338,#21339,#21340));
#4859=EDGE_LOOP('',(#21341,#21342,#21343,#21344));
#4860=EDGE_LOOP('',(#21345,#21346,#21347,#21348));
#4861=EDGE_LOOP('',(#21349,#21350,#21351,#21352));
#4862=EDGE_LOOP('',(#21353,#21354,#21355,#21356));
#4863=EDGE_LOOP('',(#21357,#21358,#21359));
#4864=EDGE_LOOP('',(#21360,#21361,#21362,#21363));
#4865=EDGE_LOOP('',(#21364,#21365,#21366,#21367));
#4866=EDGE_LOOP('',(#21368,#21369,#21370));
#4867=EDGE_LOOP('',(#21371,#21372,#21373,#21374));
#4868=EDGE_LOOP('',(#21375,#21376,#21377,#21378));
#4869=EDGE_LOOP('',(#21379,#21380,#21381,#21382));
#4870=EDGE_LOOP('',(#21383,#21384,#21385));
#4871=EDGE_LOOP('',(#21386,#21387,#21388,#21389));
#4872=EDGE_LOOP('',(#21390,#21391,#21392,#21393));
#4873=EDGE_LOOP('',(#21394,#21395,#21396,#21397));
#4874=EDGE_LOOP('',(#21398,#21399,#21400,#21401));
#4875=EDGE_LOOP('',(#21402,#21403,#21404,#21405));
#4876=EDGE_LOOP('',(#21406,#21407,#21408,#21409));
#4877=EDGE_LOOP('',(#21410,#21411,#21412,#21413));
#4878=EDGE_LOOP('',(#21414,#21415,#21416));
#4879=EDGE_LOOP('',(#21417,#21418,#21419,#21420));
#4880=EDGE_LOOP('',(#21421,#21422,#21423,#21424));
#4881=EDGE_LOOP('',(#21425,#21426,#21427,#21428));
#4882=EDGE_LOOP('',(#21429,#21430,#21431,#21432));
#4883=EDGE_LOOP('',(#21433,#21434,#21435,#21436));
#4884=EDGE_LOOP('',(#21437,#21438,#21439));
#4885=EDGE_LOOP('',(#21440,#21441,#21442,#21443));
#4886=EDGE_LOOP('',(#21444,#21445,#21446,#21447));
#4887=EDGE_LOOP('',(#21448,#21449,#21450));
#4888=EDGE_LOOP('',(#21451,#21452,#21453,#21454));
#4889=EDGE_LOOP('',(#21455,#21456,#21457,#21458));
#4890=EDGE_LOOP('',(#21459,#21460,#21461,#21462));
#4891=EDGE_LOOP('',(#21463,#21464,#21465));
#4892=EDGE_LOOP('',(#21466,#21467,#21468,#21469));
#4893=EDGE_LOOP('',(#21470,#21471,#21472,#21473));
#4894=EDGE_LOOP('',(#21474,#21475,#21476,#21477));
#4895=EDGE_LOOP('',(#21478,#21479,#21480,#21481));
#4896=EDGE_LOOP('',(#21482,#21483,#21484,#21485));
#4897=EDGE_LOOP('',(#21486,#21487,#21488,#21489));
#4898=EDGE_LOOP('',(#21490,#21491,#21492,#21493));
#4899=EDGE_LOOP('',(#21494,#21495,#21496));
#4900=EDGE_LOOP('',(#21497,#21498,#21499,#21500));
#4901=EDGE_LOOP('',(#21501,#21502,#21503,#21504));
#4902=EDGE_LOOP('',(#21505,#21506,#21507,#21508));
#4903=EDGE_LOOP('',(#21509,#21510,#21511,#21512));
#4904=EDGE_LOOP('',(#21513,#21514,#21515,#21516));
#4905=EDGE_LOOP('',(#21517,#21518,#21519));
#4906=EDGE_LOOP('',(#21520,#21521,#21522,#21523));
#4907=EDGE_LOOP('',(#21524,#21525,#21526,#21527));
#4908=EDGE_LOOP('',(#21528,#21529,#21530));
#4909=EDGE_LOOP('',(#21531,#21532,#21533,#21534));
#4910=EDGE_LOOP('',(#21535,#21536,#21537,#21538));
#4911=EDGE_LOOP('',(#21539,#21540,#21541,#21542));
#4912=EDGE_LOOP('',(#21543,#21544,#21545));
#4913=EDGE_LOOP('',(#21546,#21547,#21548,#21549));
#4914=EDGE_LOOP('',(#21550,#21551,#21552,#21553));
#4915=EDGE_LOOP('',(#21554,#21555,#21556,#21557));
#4916=EDGE_LOOP('',(#21558,#21559,#21560,#21561));
#4917=EDGE_LOOP('',(#21562,#21563,#21564,#21565));
#4918=EDGE_LOOP('',(#21566,#21567,#21568,#21569));
#4919=EDGE_LOOP('',(#21570,#21571,#21572,#21573));
#4920=EDGE_LOOP('',(#21574,#21575,#21576,#21577));
#4921=EDGE_LOOP('',(#21578,#21579,#21580,#21581));
#4922=EDGE_LOOP('',(#21582,#21583,#21584));
#4923=EDGE_LOOP('',(#21585,#21586,#21587,#21588));
#4924=EDGE_LOOP('',(#21589,#21590,#21591,#21592));
#4925=EDGE_LOOP('',(#21593,#21594,#21595,#21596));
#4926=EDGE_LOOP('',(#21597,#21598,#21599));
#4927=EDGE_LOOP('',(#21600,#21601,#21602,#21603));
#4928=EDGE_LOOP('',(#21604,#21605,#21606,#21607));
#4929=EDGE_LOOP('',(#21608,#21609,#21610,#21611));
#4930=EDGE_LOOP('',(#21612,#21613,#21614,#21615));
#4931=EDGE_LOOP('',(#21616,#21617,#21618,#21619));
#4932=EDGE_LOOP('',(#21620,#21621,#21622,#21623));
#4933=EDGE_LOOP('',(#21624,#21625,#21626));
#4934=EDGE_LOOP('',(#21627,#21628,#21629,#21630));
#4935=EDGE_LOOP('',(#21631,#21632,#21633));
#4936=EDGE_LOOP('',(#21634,#21635,#21636,#21637));
#4937=EDGE_LOOP('',(#21638,#21639,#21640,#21641));
#4938=EDGE_LOOP('',(#21642,#21643,#21644,#21645));
#4939=EDGE_LOOP('',(#21646,#21647,#21648,#21649));
#4940=EDGE_LOOP('',(#21650,#21651,#21652,#21653));
#4941=EDGE_LOOP('',(#21654,#21655,#21656));
#4942=EDGE_LOOP('',(#21657,#21658,#21659,#21660));
#4943=EDGE_LOOP('',(#21661,#21662,#21663,#21664));
#4944=EDGE_LOOP('',(#21665,#21666,#21667,#21668));
#4945=EDGE_LOOP('',(#21669,#21670,#21671,#21672));
#4946=EDGE_LOOP('',(#21673,#21674,#21675,#21676));
#4947=EDGE_LOOP('',(#21677,#21678,#21679));
#4948=EDGE_LOOP('',(#21680,#21681,#21682,#21683));
#4949=EDGE_LOOP('',(#21684,#21685,#21686,#21687));
#4950=EDGE_LOOP('',(#21688,#21689,#21690));
#4951=EDGE_LOOP('',(#21691,#21692,#21693,#21694));
#4952=EDGE_LOOP('',(#21695,#21696,#21697,#21698));
#4953=EDGE_LOOP('',(#21699,#21700,#21701,#21702));
#4954=EDGE_LOOP('',(#21703,#21704,#21705));
#4955=EDGE_LOOP('',(#21706,#21707,#21708,#21709));
#4956=EDGE_LOOP('',(#21710,#21711,#21712,#21713));
#4957=EDGE_LOOP('',(#21714,#21715,#21716,#21717));
#4958=EDGE_LOOP('',(#21718,#21719,#21720,#21721));
#4959=EDGE_LOOP('',(#21722,#21723,#21724,#21725,#21726,#21727,#21728,#21729));
#4960=EDGE_LOOP('',(#21730,#21731,#21732,#21733,#21734,#21735,#21736,#21737));
#4961=EDGE_LOOP('',(#21738,#21739,#21740,#21741,#21742,#21743,#21744,#21745));
#4962=EDGE_LOOP('',(#21746,#21747,#21748,#21749,#21750,#21751,#21752,#21753));
#4963=EDGE_LOOP('',(#21754,#21755,#21756,#21757,#21758,#21759,#21760,#21761));
#4964=EDGE_LOOP('',(#21762,#21763,#21764,#21765,#21766,#21767,#21768,#21769));
#4965=EDGE_LOOP('',(#21770,#21771,#21772,#21773,#21774,#21775,#21776,#21777));
#4966=EDGE_LOOP('',(#21778,#21779,#21780,#21781,#21782,#21783,#21784,#21785));
#4967=EDGE_LOOP('',(#21786));
#4968=EDGE_LOOP('',(#21787,#21788,#21789,#21790));
#4969=EDGE_LOOP('',(#21791));
#4970=EDGE_LOOP('',(#21792,#21793,#21794,#21795));
#4971=EDGE_LOOP('',(#21796));
#4972=EDGE_LOOP('',(#21797,#21798,#21799,#21800));
#4973=EDGE_LOOP('',(#21801,#21802,#21803,#21804,#21805,#21806,#21807,#21808,
#21809,#21810,#21811,#21812,#21813,#21814,#21815,#21816,#21817,#21818,#21819,
#21820,#21821,#21822,#21823,#21824,#21825,#21826,#21827,#21828,#21829,#21830,
#21831,#21832,#21833,#21834,#21835,#21836,#21837,#21838,#21839,#21840,#21841,
#21842,#21843,#21844,#21845,#21846,#21847,#21848));
#4974=EDGE_LOOP('',(#21849));
#4975=EDGE_LOOP('',(#21850));
#4976=EDGE_LOOP('',(#21851));
#4977=EDGE_LOOP('',(#21852));
#4978=EDGE_LOOP('',(#21853));
#4979=EDGE_LOOP('',(#21854,#21855,#21856,#21857));
#4980=EDGE_LOOP('',(#21858));
#4981=EDGE_LOOP('',(#21859,#21860,#21861,#21862));
#4982=EDGE_LOOP('',(#21863));
#4983=EDGE_LOOP('',(#21864,#21865,#21866,#21867));
#4984=EDGE_LOOP('',(#21868));
#4985=EDGE_LOOP('',(#21869,#21870,#21871,#21872));
#4986=EDGE_LOOP('',(#21873,#21874,#21875,#21876,#21877,#21878,#21879,#21880,
#21881,#21882,#21883,#21884,#21885,#21886,#21887,#21888,#21889,#21890,#21891,
#21892,#21893,#21894,#21895,#21896,#21897,#21898,#21899,#21900,#21901,#21902,
#21903,#21904,#21905,#21906,#21907,#21908,#21909,#21910,#21911,#21912,#21913,
#21914,#21915,#21916,#21917,#21918,#21919,#21920));
#4987=EDGE_LOOP('',(#21921));
#4988=EDGE_LOOP('',(#21922));
#4989=EDGE_LOOP('',(#21923));
#4990=EDGE_LOOP('',(#21924));
#4991=EDGE_LOOP('',(#21925));
#6892=LINE('',#41236,#8881);
#6893=LINE('',#41244,#8882);
#6894=LINE('',#63971,#8883);
#6895=LINE('',#63978,#8884);
#6896=LINE('',#63985,#8885);
#6897=LINE('',#63992,#8886);
#6898=LINE('',#63998,#8887);
#6899=LINE('',#64005,#8888);
#6900=LINE('',#64012,#8889);
#8881=VECTOR('',#33519,2.);
#8882=VECTOR('',#33530,2.);
#8883=VECTOR('',#33923,2.);
#8884=VECTOR('',#33932,2.);
#8885=VECTOR('',#33941,2.);
#8886=VECTOR('',#33950,13.5);
#8887=VECTOR('',#33957,2.);
#8888=VECTOR('',#33966,2.);
#8889=VECTOR('',#33975,2.);
#10163=CIRCLE('',#27716,2.);
#10164=CIRCLE('',#27718,2.);
#10165=CIRCLE('',#27720,2.);
#10166=CIRCLE('',#27722,2.);
#10167=CIRCLE('',#27723,1.000000009999);
#10168=CIRCLE('',#27724,1.000000122615);
#10169=CIRCLE('',#27725,1.000000000939);
#10170=CIRCLE('',#27726,39.901435785627);
#10171=CIRCLE('',#27727,0.999999999999998);
#10172=CIRCLE('',#27728,38.8921101653477);
#10173=CIRCLE('',#27730,1.00000197298164);
#10174=CIRCLE('',#27731,1.000005019194);
#10175=CIRCLE('',#27732,1.00001938568424);
#10176=CIRCLE('',#27734,1.000000068316);
#10177=CIRCLE('',#27735,1.00001946091789);
#10178=CIRCLE('',#27737,1.000005006638);
#10179=CIRCLE('',#27738,1.000000068317);
#10180=CIRCLE('',#27739,39.8991935477595);
#10181=CIRCLE('',#27740,38.874817547618);
#10182=CIRCLE('',#27741,1.000000000939);
#10183=CIRCLE('',#27743,1.00003031349091);
#10184=CIRCLE('',#27744,0.999996385196527);
#10185=CIRCLE('',#27745,1.000000122615);
#10186=CIRCLE('',#27746,1.000000000939);
#10187=CIRCLE('',#27747,39.9014357641817);
#10188=CIRCLE('',#27748,0.999999999999999);
#10189=CIRCLE('',#27749,38.8921101994134);
#10190=CIRCLE('',#27751,1.00000197297109);
#10191=CIRCLE('',#27752,1.000005019194);
#10192=CIRCLE('',#27753,1.00000191452219);
#10193=CIRCLE('',#27754,1.00001938569039);
#10194=CIRCLE('',#27756,1.000000068316);
#10195=CIRCLE('',#27757,1.00001946091372);
#10196=CIRCLE('',#27759,1.000005006638);
#10197=CIRCLE('',#27760,1.000000068317);
#10198=CIRCLE('',#27761,39.8991935573533);
#10199=CIRCLE('',#27762,38.8748146429027);
#10200=CIRCLE('',#27763,1.000000000939);
#10201=CIRCLE('',#27765,1.00003031350209);
#10202=CIRCLE('',#27766,0.999996390589362);
#10203=CIRCLE('',#27767,1.000000122615);
#10204=CIRCLE('',#27768,1.000000000939);
#10205=CIRCLE('',#27769,39.9014357932221);
#10206=CIRCLE('',#27770,1.);
#10207=CIRCLE('',#27771,38.8921101598015);
#10208=CIRCLE('',#27773,1.00000197298478);
#10209=CIRCLE('',#27774,1.000005019194);
#10210=CIRCLE('',#27775,1.00001938568406);
#10211=CIRCLE('',#27777,1.000000068316);
#10212=CIRCLE('',#27778,1.00001946091692);
#10213=CIRCLE('',#27780,1.000005006638);
#10214=CIRCLE('',#27781,1.000000068317);
#10215=CIRCLE('',#27782,39.899193552042);
#10216=CIRCLE('',#27783,38.8748161532142);
#10217=CIRCLE('',#27784,1.000000000939);
#10218=CIRCLE('',#27786,1.00003031349466);
#10219=CIRCLE('',#27787,0.999996305682662);
#10220=CIRCLE('',#27788,1.000000009973);
#10221=CIRCLE('',#27789,1.000000122615);
#10222=CIRCLE('',#27790,1.000000000939);
#10223=CIRCLE('',#27791,39.9014357779458);
#10224=CIRCLE('',#27792,0.999999999999999);
#10225=CIRCLE('',#27793,38.8921099760719);
#10226=CIRCLE('',#27795,1.00000197298803);
#10227=CIRCLE('',#27796,1.0000050192);
#10228=CIRCLE('',#27797,1.00001938562544);
#10229=CIRCLE('',#27799,1.000000068316);
#10230=CIRCLE('',#27800,1.0000000086);
#10231=CIRCLE('',#27801,1.00001946091164);
#10232=CIRCLE('',#27803,1.000005006635);
#10233=CIRCLE('',#27804,1.000000068317);
#10234=CIRCLE('',#27805,39.8991935595103);
#10235=CIRCLE('',#27806,38.8748146565752);
#10236=CIRCLE('',#27807,1.000000000939);
#10237=CIRCLE('',#27809,1.00003031414254);
#10238=CIRCLE('',#27810,1.000000004171);
#10239=CIRCLE('',#27811,1.000000122616);
#10240=CIRCLE('',#27812,1.000000000939);
#10241=CIRCLE('',#27813,39.9014357924868);
#10242=CIRCLE('',#27814,1.);
#10243=CIRCLE('',#27815,38.8921099732382);
#10244=CIRCLE('',#27817,1.00000197301089);
#10245=CIRCLE('',#27818,1.0000050192);
#10246=CIRCLE('',#27819,1.00000191098175);
#10247=CIRCLE('',#27820,1.00001938561266);
#10248=CIRCLE('',#27822,1.000000068316);
#10249=CIRCLE('',#27823,1.00001946090666);
#10250=CIRCLE('',#27825,1.000005006635);
#10251=CIRCLE('',#27826,1.000000068317);
#10252=CIRCLE('',#27827,39.8991935511885);
#10253=CIRCLE('',#27828,38.8748175664677);
#10254=CIRCLE('',#27829,1.000000000939);
#10255=CIRCLE('',#27831,1.00003031414535);
#10256=CIRCLE('',#27832,1.000000122616);
#10257=CIRCLE('',#27833,1.000000000939);
#10258=CIRCLE('',#27834,39.9014357636129);
#10259=CIRCLE('',#27835,1.);
#10260=CIRCLE('',#27836,38.8921099760377);
#10261=CIRCLE('',#27838,1.0000019729999);
#10262=CIRCLE('',#27839,1.0000050192);
#10263=CIRCLE('',#27840,1.00001938562086);
#10264=CIRCLE('',#27842,1.000000068316);
#10265=CIRCLE('',#27843,0.999996375475787);
#10266=CIRCLE('',#27844,1.0000194609088);
#10267=CIRCLE('',#27846,1.000005006635);
#10268=CIRCLE('',#27847,1.000000068317);
#10269=CIRCLE('',#27848,39.8991935494084);
#10270=CIRCLE('',#27849,38.874816056833);
#10271=CIRCLE('',#27850,1.000000000939);
#10272=CIRCLE('',#27852,1.00003031413779);
#10273=CIRCLE('',#27853,0.999996384223477);
#10274=CIRCLE('',#27854,1.000000122614);
#10275=CIRCLE('',#27855,1.00000197292957);
#10276=CIRCLE('',#27856,1.000005019194);
#10277=CIRCLE('',#27858,1.);
#10278=CIRCLE('',#27859,1.00000000094);
#10279=CIRCLE('',#27860,39.9014356027643);
#10280=CIRCLE('',#27861,38.8921102040137);
#10281=CIRCLE('',#27862,39.8991935568584);
#10282=CIRCLE('',#27863,1.00000000094);
#10283=CIRCLE('',#27864,1.000005006638);
#10284=CIRCLE('',#27866,1.0000303135037);
#10285=CIRCLE('',#27867,0.999996369425503);
#10286=CIRCLE('',#27868,0.999976684049138);
#10287=CIRCLE('',#27869,1.00001946095475);
#10288=CIRCLE('',#27871,1.000000068378);
#10289=CIRCLE('',#27872,1.000000068377);
#10290=CIRCLE('',#27873,38.8748167422972);
#10291=CIRCLE('',#27875,1.00001938573349);
#10292=CIRCLE('',#27876,1.000000251468);
#10293=CIRCLE('',#27877,1.000000122616);
#10294=CIRCLE('',#27878,1.000000000939);
#10295=CIRCLE('',#27879,39.9014357922065);
#10296=CIRCLE('',#27880,0.999999999999998);
#10297=CIRCLE('',#27881,38.8921099729939);
#10298=CIRCLE('',#27883,1.00000197301321);
#10299=CIRCLE('',#27884,1.0000050192);
#10300=CIRCLE('',#27885,1.00000650505067);
#10301=CIRCLE('',#27886,1.00001938561205);
#10302=CIRCLE('',#27888,1.000000068316);
#10303=CIRCLE('',#27889,1.0000194609075);
#10304=CIRCLE('',#27891,1.000005006635);
#10305=CIRCLE('',#27892,1.000000068317);
#10306=CIRCLE('',#27893,39.8991935508386);
#10307=CIRCLE('',#27894,38.8748160719392);
#10308=CIRCLE('',#27895,1.000000000939);
#10309=CIRCLE('',#27897,1.00003031415272);
#10310=CIRCLE('',#27898,1.000000046838);
#10311=CIRCLE('',#27899,14.88340478034);
#10312=CIRCLE('',#27900,14.88340478034);
#10313=CIRCLE('',#27901,14.88340478034);
#10314=CIRCLE('',#27902,14.88340478034);
#10315=CIRCLE('',#27903,14.88340478034);
#10316=CIRCLE('',#27904,14.88340478034);
#10317=CIRCLE('',#27905,14.88340478034);
#10318=CIRCLE('',#27906,14.88340478034);
#10319=CIRCLE('',#27907,14.88340478034);
#10320=CIRCLE('',#27908,14.88340478034);
#10321=CIRCLE('',#27909,14.88340478034);
#10322=CIRCLE('',#27910,14.88340478034);
#10323=CIRCLE('',#27911,14.88340478034);
#10324=CIRCLE('',#27912,14.88340478034);
#10325=CIRCLE('',#27913,14.88340478034);
#10326=CIRCLE('',#27914,14.88340478034);
#10327=CIRCLE('',#27916,2.);
#10328=CIRCLE('',#27918,2.);
#10329=CIRCLE('',#27920,2.);
#10330=CIRCLE('',#27922,2.);
#10331=CIRCLE('',#27924,2.);
#10332=CIRCLE('',#27926,2.);
#10333=CIRCLE('',#27928,13.5);
#10334=CIRCLE('',#27930,13.5);
#10335=CIRCLE('',#27932,2.);
#10336=CIRCLE('',#27934,2.);
#10337=CIRCLE('',#27936,2.);
#10338=CIRCLE('',#27938,2.);
#10339=CIRCLE('',#27940,2.);
#10340=CIRCLE('',#27942,2.);
#12119=VERTEX_POINT('',#41232);
#12120=VERTEX_POINT('',#41235);
#12121=VERTEX_POINT('',#41239);
#12122=VERTEX_POINT('',#41242);
#12123=VERTEX_POINT('',#41285);
#12124=VERTEX_POINT('',#41286);
#12125=VERTEX_POINT('',#41288);
#12126=VERTEX_POINT('',#41314);
#12127=VERTEX_POINT('',#41425);
#12128=VERTEX_POINT('',#41499);
#12129=VERTEX_POINT('',#41598);
#12130=VERTEX_POINT('',#41599);
#12131=VERTEX_POINT('',#41601);
#12132=VERTEX_POINT('',#41671);
#12133=VERTEX_POINT('',#41838);
#12134=VERTEX_POINT('',#42017);
#12135=VERTEX_POINT('',#42181);
#12136=VERTEX_POINT('',#42377);
#12137=VERTEX_POINT('',#42378);
#12138=VERTEX_POINT('',#42536);
#12139=VERTEX_POINT('',#42667);
#12140=VERTEX_POINT('',#42668);
#12141=VERTEX_POINT('',#42727);
#12142=VERTEX_POINT('',#42750);
#12143=VERTEX_POINT('',#42857);
#12144=VERTEX_POINT('',#42946);
#12145=VERTEX_POINT('',#43007);
#12146=VERTEX_POINT('',#43350);
#12147=VERTEX_POINT('',#43551);
#12148=VERTEX_POINT('',#43552);
#12149=VERTEX_POINT('',#43584);
#12150=VERTEX_POINT('',#43607);
#12151=VERTEX_POINT('',#44128);
#12152=VERTEX_POINT('',#44129);
#12153=VERTEX_POINT('',#44188);
#12154=VERTEX_POINT('',#44211);
#12155=VERTEX_POINT('',#44322);
#12156=VERTEX_POINT('',#44396);
#12157=VERTEX_POINT('',#44495);
#12158=VERTEX_POINT('',#44496);
#12159=VERTEX_POINT('',#44498);
#12160=VERTEX_POINT('',#44568);
#12161=VERTEX_POINT('',#44735);
#12162=VERTEX_POINT('',#44914);
#12163=VERTEX_POINT('',#45070);
#12164=VERTEX_POINT('',#45190);
#12165=VERTEX_POINT('',#45191);
#12166=VERTEX_POINT('',#45346);
#12167=VERTEX_POINT('',#45477);
#12168=VERTEX_POINT('',#45478);
#12169=VERTEX_POINT('',#45537);
#12170=VERTEX_POINT('',#45563);
#12171=VERTEX_POINT('',#45673);
#12172=VERTEX_POINT('',#45762);
#12173=VERTEX_POINT('',#45823);
#12174=VERTEX_POINT('',#46166);
#12175=VERTEX_POINT('',#46363);
#12176=VERTEX_POINT('',#46364);
#12177=VERTEX_POINT('',#46396);
#12178=VERTEX_POINT('',#46422);
#12179=VERTEX_POINT('',#46907);
#12180=VERTEX_POINT('',#46908);
#12181=VERTEX_POINT('',#46967);
#12182=VERTEX_POINT('',#46993);
#12183=VERTEX_POINT('',#47106);
#12184=VERTEX_POINT('',#47180);
#12185=VERTEX_POINT('',#47279);
#12186=VERTEX_POINT('',#47280);
#12187=VERTEX_POINT('',#47282);
#12188=VERTEX_POINT('',#47352);
#12189=VERTEX_POINT('',#47519);
#12190=VERTEX_POINT('',#47698);
#12191=VERTEX_POINT('',#47862);
#12192=VERTEX_POINT('',#48057);
#12193=VERTEX_POINT('',#48058);
#12194=VERTEX_POINT('',#48197);
#12195=VERTEX_POINT('',#48328);
#12196=VERTEX_POINT('',#48329);
#12197=VERTEX_POINT('',#48388);
#12198=VERTEX_POINT('',#48414);
#12199=VERTEX_POINT('',#48526);
#12200=VERTEX_POINT('',#48615);
#12201=VERTEX_POINT('',#48676);
#12202=VERTEX_POINT('',#49052);
#12203=VERTEX_POINT('',#49249);
#12204=VERTEX_POINT('',#49250);
#12205=VERTEX_POINT('',#49282);
#12206=VERTEX_POINT('',#49308);
#12207=VERTEX_POINT('',#49806);
#12208=VERTEX_POINT('',#49807);
#12209=VERTEX_POINT('',#49809);
#12210=VERTEX_POINT('',#49835);
#12211=VERTEX_POINT('',#49946);
#12212=VERTEX_POINT('',#50020);
#12213=VERTEX_POINT('',#50119);
#12214=VERTEX_POINT('',#50120);
#12215=VERTEX_POINT('',#50122);
#12216=VERTEX_POINT('',#50192);
#12217=VERTEX_POINT('',#50359);
#12218=VERTEX_POINT('',#50538);
#12219=VERTEX_POINT('',#50702);
#12220=VERTEX_POINT('',#50895);
#12221=VERTEX_POINT('',#50896);
#12222=VERTEX_POINT('',#51054);
#12223=VERTEX_POINT('',#51193);
#12224=VERTEX_POINT('',#51194);
#12225=VERTEX_POINT('',#51196);
#12226=VERTEX_POINT('',#51222);
#12227=VERTEX_POINT('',#51329);
#12228=VERTEX_POINT('',#51418);
#12229=VERTEX_POINT('',#51479);
#12230=VERTEX_POINT('',#51852);
#12231=VERTEX_POINT('',#52053);
#12232=VERTEX_POINT('',#52054);
#12233=VERTEX_POINT('',#52086);
#12234=VERTEX_POINT('',#52112);
#12235=VERTEX_POINT('',#52618);
#12236=VERTEX_POINT('',#52619);
#12237=VERTEX_POINT('',#52678);
#12238=VERTEX_POINT('',#52701);
#12239=VERTEX_POINT('',#52812);
#12240=VERTEX_POINT('',#52886);
#12241=VERTEX_POINT('',#52985);
#12242=VERTEX_POINT('',#52986);
#12243=VERTEX_POINT('',#52988);
#12244=VERTEX_POINT('',#53058);
#12245=VERTEX_POINT('',#53225);
#12246=VERTEX_POINT('',#53404);
#12247=VERTEX_POINT('',#53560);
#12248=VERTEX_POINT('',#53680);
#12249=VERTEX_POINT('',#53681);
#12250=VERTEX_POINT('',#53836);
#12251=VERTEX_POINT('',#53971);
#12252=VERTEX_POINT('',#53972);
#12253=VERTEX_POINT('',#54031);
#12254=VERTEX_POINT('',#54057);
#12255=VERTEX_POINT('',#54190);
#12256=VERTEX_POINT('',#54279);
#12257=VERTEX_POINT('',#54340);
#12258=VERTEX_POINT('',#54713);
#12259=VERTEX_POINT('',#54914);
#12260=VERTEX_POINT('',#54915);
#12261=VERTEX_POINT('',#54947);
#12262=VERTEX_POINT('',#54973);
#12263=VERTEX_POINT('',#55553);
#12264=VERTEX_POINT('',#55554);
#12265=VERTEX_POINT('',#55613);
#12266=VERTEX_POINT('',#55620);
#12267=VERTEX_POINT('',#55733);
#12268=VERTEX_POINT('',#55807);
#12269=VERTEX_POINT('',#55906);
#12270=VERTEX_POINT('',#55907);
#12271=VERTEX_POINT('',#55909);
#12272=VERTEX_POINT('',#55979);
#12273=VERTEX_POINT('',#56146);
#12274=VERTEX_POINT('',#56325);
#12275=VERTEX_POINT('',#56489);
#12276=VERTEX_POINT('',#56681);
#12277=VERTEX_POINT('',#56682);
#12278=VERTEX_POINT('',#56821);
#12279=VERTEX_POINT('',#56952);
#12280=VERTEX_POINT('',#56953);
#12281=VERTEX_POINT('',#56955);
#12282=VERTEX_POINT('',#56978);
#12283=VERTEX_POINT('',#57085);
#12284=VERTEX_POINT('',#57174);
#12285=VERTEX_POINT('',#57235);
#12286=VERTEX_POINT('',#57605);
#12287=VERTEX_POINT('',#57806);
#12288=VERTEX_POINT('',#57807);
#12289=VERTEX_POINT('',#57839);
#12290=VERTEX_POINT('',#57862);
#12291=VERTEX_POINT('',#58358);
#12292=VERTEX_POINT('',#58359);
#12293=VERTEX_POINT('',#58433);
#12294=VERTEX_POINT('',#58435);
#12295=VERTEX_POINT('',#58603);
#12296=VERTEX_POINT('',#58662);
#12297=VERTEX_POINT('',#58745);
#12298=VERTEX_POINT('',#58746);
#12299=VERTEX_POINT('',#58992);
#12300=VERTEX_POINT('',#59242);
#12301=VERTEX_POINT('',#59244);
#12302=VERTEX_POINT('',#59438);
#12303=VERTEX_POINT('',#59439);
#12304=VERTEX_POINT('',#59463);
#12305=VERTEX_POINT('',#59759);
#12306=VERTEX_POINT('',#59761);
#12307=VERTEX_POINT('',#59958);
#12308=VERTEX_POINT('',#59959);
#12309=VERTEX_POINT('',#59991);
#12310=VERTEX_POINT('',#60014);
#12311=VERTEX_POINT('',#60296);
#12312=VERTEX_POINT('',#60449);
#12313=VERTEX_POINT('',#60569);
#12314=VERTEX_POINT('',#60592);
#12315=VERTEX_POINT('',#60703);
#12316=VERTEX_POINT('',#60819);
#12317=VERTEX_POINT('',#60864);
#12318=VERTEX_POINT('',#61056);
#12319=VERTEX_POINT('',#61153);
#12320=VERTEX_POINT('',#61154);
#12321=VERTEX_POINT('',#61156);
#12322=VERTEX_POINT('',#61173);
#12323=VERTEX_POINT('',#61284);
#12324=VERTEX_POINT('',#61358);
#12325=VERTEX_POINT('',#61457);
#12326=VERTEX_POINT('',#61458);
#12327=VERTEX_POINT('',#61460);
#12328=VERTEX_POINT('',#61530);
#12329=VERTEX_POINT('',#61697);
#12330=VERTEX_POINT('',#61876);
#12331=VERTEX_POINT('',#62036);
#12332=VERTEX_POINT('',#62163);
#12333=VERTEX_POINT('',#62164);
#12334=VERTEX_POINT('',#62316);
#12335=VERTEX_POINT('',#62451);
#12336=VERTEX_POINT('',#62452);
#12337=VERTEX_POINT('',#62511);
#12338=VERTEX_POINT('',#62528);
#12339=VERTEX_POINT('',#62638);
#12340=VERTEX_POINT('',#62727);
#12341=VERTEX_POINT('',#62788);
#12342=VERTEX_POINT('',#63161);
#12343=VERTEX_POINT('',#63362);
#12344=VERTEX_POINT('',#63363);
#12345=VERTEX_POINT('',#63395);
#12346=VERTEX_POINT('',#63412);
#12347=VERTEX_POINT('',#63966);
#12348=VERTEX_POINT('',#63969);
#12349=VERTEX_POINT('',#63973);
#12350=VERTEX_POINT('',#63976);
#12351=VERTEX_POINT('',#63980);
#12352=VERTEX_POINT('',#63983);
#12353=VERTEX_POINT('',#63987);
#12354=VERTEX_POINT('',#63990);
#12355=VERTEX_POINT('',#63994);
#12356=VERTEX_POINT('',#63997);
#12357=VERTEX_POINT('',#64001);
#12358=VERTEX_POINT('',#64004);
#12359=VERTEX_POINT('',#64008);
#12360=VERTEX_POINT('',#64011);
#15229=EDGE_CURVE('',#12119,#12119,#10163,.T.);
#15230=EDGE_CURVE('',#12119,#12120,#6892,.T.);
#15231=EDGE_CURVE('',#12120,#12120,#10164,.T.);
#15232=EDGE_CURVE('',#12121,#12121,#10165,.T.);
#15233=EDGE_CURVE('',#12122,#12122,#10166,.T.);
#15234=EDGE_CURVE('',#12122,#12121,#6893,.T.);
#15235=EDGE_CURVE('',#12123,#12124,#10167,.T.);
#15236=EDGE_CURVE('',#12125,#12124,#134,.T.);
#15237=EDGE_CURVE('',#12126,#12125,#135,.T.);
#15238=EDGE_CURVE('',#12126,#12123,#136,.T.);
#15239=EDGE_CURVE('',#12127,#12126,#137,.T.);
#15240=EDGE_CURVE('',#12127,#12128,#10168,.T.);
#15241=EDGE_CURVE('',#12128,#12123,#138,.T.);
#15242=EDGE_CURVE('',#12129,#12130,#10169,.T.);
#15243=EDGE_CURVE('',#12130,#12131,#10170,.T.);
#15244=EDGE_CURVE('',#12131,#12127,#10171,.T.);
#15245=EDGE_CURVE('',#12129,#12127,#10172,.T.);
#15246=EDGE_CURVE('',#12128,#12131,#10173,.T.);
#15247=EDGE_CURVE('',#12132,#12131,#139,.T.);
#15248=EDGE_CURVE('',#12132,#12133,#10174,.T.);
#15249=EDGE_CURVE('',#12133,#12128,#140,.T.);
#15250=EDGE_CURVE('',#12133,#12134,#141,.T.);
#15251=EDGE_CURVE('',#12123,#12134,#142,.T.);
#15252=EDGE_CURVE('',#12134,#12135,#143,.T.);
#15253=EDGE_CURVE('',#12124,#12135,#144,.T.);
#15254=EDGE_CURVE('',#12136,#12137,#145,.T.);
#15255=EDGE_CURVE('',#12135,#12137,#146,.T.);
#15256=EDGE_CURVE('',#12134,#12136,#147,.T.);
#15257=EDGE_CURVE('',#12133,#12138,#10175,.T.);
#15258=EDGE_CURVE('',#12138,#12136,#148,.T.);
#15259=EDGE_CURVE('',#12138,#12132,#10176,.T.);
#15260=EDGE_CURVE('',#12139,#12140,#149,.T.);
#15261=EDGE_CURVE('',#12141,#12140,#150,.T.);
#15262=EDGE_CURVE('',#12142,#12141,#151,.T.);
#15263=EDGE_CURVE('',#12142,#12139,#152,.T.);
#15264=EDGE_CURVE('',#12142,#12143,#153,.T.);
#15265=EDGE_CURVE('',#12143,#12144,#10177,.T.);
#15266=EDGE_CURVE('',#12139,#12144,#154,.T.);
#15267=EDGE_CURVE('',#12144,#12145,#10178,.T.);
#15268=EDGE_CURVE('',#12145,#12143,#10179,.T.);
#15269=EDGE_CURVE('',#12145,#12132,#10180,.T.);
#15270=EDGE_CURVE('',#12143,#12138,#10181,.T.);
#15271=EDGE_CURVE('',#12145,#12130,#155,.T.);
#15272=EDGE_CURVE('',#12130,#12146,#10182,.T.);
#15273=EDGE_CURVE('',#12144,#12146,#156,.T.);
#15274=EDGE_CURVE('',#12146,#12129,#10183,.T.);
#15275=EDGE_CURVE('',#12147,#12148,#157,.T.);
#15276=EDGE_CURVE('',#12149,#12148,#158,.T.);
#15277=EDGE_CURVE('',#12150,#12149,#10184,.T.);
#15278=EDGE_CURVE('',#12150,#12147,#159,.T.);
#15279=EDGE_CURVE('',#12147,#12129,#160,.T.);
#15280=EDGE_CURVE('',#12150,#12146,#161,.T.);
#15281=EDGE_CURVE('',#12139,#12150,#162,.T.);
#15282=EDGE_CURVE('',#12140,#12149,#163,.T.);
#15283=EDGE_CURVE('',#12151,#12152,#164,.T.);
#15284=EDGE_CURVE('',#12153,#12152,#165,.T.);
#15285=EDGE_CURVE('',#12154,#12153,#166,.T.);
#15286=EDGE_CURVE('',#12154,#12151,#167,.T.);
#15287=EDGE_CURVE('',#12155,#12154,#168,.T.);
#15288=EDGE_CURVE('',#12155,#12156,#10185,.T.);
#15289=EDGE_CURVE('',#12156,#12151,#169,.T.);
#15290=EDGE_CURVE('',#12157,#12158,#10186,.T.);
#15291=EDGE_CURVE('',#12158,#12159,#10187,.T.);
#15292=EDGE_CURVE('',#12159,#12155,#10188,.T.);
#15293=EDGE_CURVE('',#12157,#12155,#10189,.T.);
#15294=EDGE_CURVE('',#12156,#12159,#10190,.T.);
#15295=EDGE_CURVE('',#12160,#12159,#170,.T.);
#15296=EDGE_CURVE('',#12160,#12161,#10191,.T.);
#15297=EDGE_CURVE('',#12161,#12156,#171,.T.);
#15298=EDGE_CURVE('',#12161,#12162,#172,.T.);
#15299=EDGE_CURVE('',#12151,#12162,#173,.T.);
#15300=EDGE_CURVE('',#12162,#12163,#10192,.T.);
#15301=EDGE_CURVE('',#12152,#12163,#174,.T.);
#15302=EDGE_CURVE('',#12164,#12165,#175,.T.);
#15303=EDGE_CURVE('',#12163,#12165,#176,.T.);
#15304=EDGE_CURVE('',#12162,#12164,#177,.T.);
#15305=EDGE_CURVE('',#12161,#12166,#10193,.T.);
#15306=EDGE_CURVE('',#12166,#12164,#178,.T.);
#15307=EDGE_CURVE('',#12166,#12160,#10194,.T.);
#15308=EDGE_CURVE('',#12167,#12168,#179,.T.);
#15309=EDGE_CURVE('',#12169,#12168,#180,.T.);
#15310=EDGE_CURVE('',#12170,#12169,#181,.T.);
#15311=EDGE_CURVE('',#12170,#12167,#182,.T.);
#15312=EDGE_CURVE('',#12170,#12171,#183,.T.);
#15313=EDGE_CURVE('',#12171,#12172,#10195,.T.);
#15314=EDGE_CURVE('',#12167,#12172,#184,.T.);
#15315=EDGE_CURVE('',#12172,#12173,#10196,.T.);
#15316=EDGE_CURVE('',#12173,#12171,#10197,.T.);
#15317=EDGE_CURVE('',#12173,#12160,#10198,.T.);
#15318=EDGE_CURVE('',#12171,#12166,#10199,.T.);
#15319=EDGE_CURVE('',#12173,#12158,#185,.T.);
#15320=EDGE_CURVE('',#12158,#12174,#10200,.T.);
#15321=EDGE_CURVE('',#12172,#12174,#186,.T.);
#15322=EDGE_CURVE('',#12174,#12157,#10201,.T.);
#15323=EDGE_CURVE('',#12175,#12176,#187,.T.);
#15324=EDGE_CURVE('',#12177,#12176,#188,.T.);
#15325=EDGE_CURVE('',#12178,#12177,#10202,.T.);
#15326=EDGE_CURVE('',#12178,#12175,#189,.T.);
#15327=EDGE_CURVE('',#12175,#12157,#190,.T.);
#15328=EDGE_CURVE('',#12178,#12174,#191,.T.);
#15329=EDGE_CURVE('',#12167,#12178,#192,.T.);
#15330=EDGE_CURVE('',#12168,#12177,#193,.T.);
#15331=EDGE_CURVE('',#12179,#12180,#194,.T.);
#15332=EDGE_CURVE('',#12181,#12180,#195,.T.);
#15333=EDGE_CURVE('',#12182,#12181,#196,.T.);
#15334=EDGE_CURVE('',#12182,#12179,#197,.T.);
#15335=EDGE_CURVE('',#12183,#12182,#198,.T.);
#15336=EDGE_CURVE('',#12183,#12184,#10203,.T.);
#15337=EDGE_CURVE('',#12184,#12179,#199,.T.);
#15338=EDGE_CURVE('',#12185,#12186,#10204,.T.);
#15339=EDGE_CURVE('',#12186,#12187,#10205,.T.);
#15340=EDGE_CURVE('',#12187,#12183,#10206,.T.);
#15341=EDGE_CURVE('',#12185,#12183,#10207,.T.);
#15342=EDGE_CURVE('',#12184,#12187,#10208,.T.);
#15343=EDGE_CURVE('',#12188,#12187,#200,.T.);
#15344=EDGE_CURVE('',#12188,#12189,#10209,.T.);
#15345=EDGE_CURVE('',#12189,#12184,#201,.T.);
#15346=EDGE_CURVE('',#12189,#12190,#202,.T.);
#15347=EDGE_CURVE('',#12179,#12190,#203,.T.);
#15348=EDGE_CURVE('',#12190,#12191,#204,.T.);
#15349=EDGE_CURVE('',#12180,#12191,#205,.T.);
#15350=EDGE_CURVE('',#12192,#12193,#206,.T.);
#15351=EDGE_CURVE('',#12191,#12193,#207,.T.);
#15352=EDGE_CURVE('',#12190,#12192,#208,.T.);
#15353=EDGE_CURVE('',#12189,#12194,#10210,.T.);
#15354=EDGE_CURVE('',#12194,#12192,#209,.T.);
#15355=EDGE_CURVE('',#12194,#12188,#10211,.T.);
#15356=EDGE_CURVE('',#12195,#12196,#210,.T.);
#15357=EDGE_CURVE('',#12197,#12196,#211,.T.);
#15358=EDGE_CURVE('',#12198,#12197,#212,.T.);
#15359=EDGE_CURVE('',#12198,#12195,#213,.T.);
#15360=EDGE_CURVE('',#12198,#12199,#214,.T.);
#15361=EDGE_CURVE('',#12199,#12200,#10212,.T.);
#15362=EDGE_CURVE('',#12195,#12200,#215,.T.);
#15363=EDGE_CURVE('',#12200,#12201,#10213,.T.);
#15364=EDGE_CURVE('',#12201,#12199,#10214,.T.);
#15365=EDGE_CURVE('',#12201,#12188,#10215,.T.);
#15366=EDGE_CURVE('',#12199,#12194,#10216,.T.);
#15367=EDGE_CURVE('',#12201,#12186,#216,.T.);
#15368=EDGE_CURVE('',#12186,#12202,#10217,.T.);
#15369=EDGE_CURVE('',#12200,#12202,#217,.T.);
#15370=EDGE_CURVE('',#12202,#12185,#10218,.T.);
#15371=EDGE_CURVE('',#12203,#12204,#218,.T.);
#15372=EDGE_CURVE('',#12205,#12204,#219,.T.);
#15373=EDGE_CURVE('',#12206,#12205,#10219,.T.);
#15374=EDGE_CURVE('',#12206,#12203,#220,.T.);
#15375=EDGE_CURVE('',#12203,#12185,#221,.T.);
#15376=EDGE_CURVE('',#12206,#12202,#222,.T.);
#15377=EDGE_CURVE('',#12195,#12206,#223,.T.);
#15378=EDGE_CURVE('',#12196,#12205,#224,.T.);
#15379=EDGE_CURVE('',#12207,#12208,#10220,.T.);
#15380=EDGE_CURVE('',#12209,#12208,#225,.T.);
#15381=EDGE_CURVE('',#12210,#12209,#226,.T.);
#15382=EDGE_CURVE('',#12210,#12207,#227,.T.);
#15383=EDGE_CURVE('',#12211,#12210,#228,.T.);
#15384=EDGE_CURVE('',#12211,#12212,#10221,.T.);
#15385=EDGE_CURVE('',#12212,#12207,#229,.T.);
#15386=EDGE_CURVE('',#12213,#12214,#10222,.T.);
#15387=EDGE_CURVE('',#12214,#12215,#10223,.T.);
#15388=EDGE_CURVE('',#12215,#12211,#10224,.T.);
#15389=EDGE_CURVE('',#12213,#12211,#10225,.T.);
#15390=EDGE_CURVE('',#12212,#12215,#10226,.T.);
#15391=EDGE_CURVE('',#12216,#12215,#230,.T.);
#15392=EDGE_CURVE('',#12216,#12217,#10227,.T.);
#15393=EDGE_CURVE('',#12217,#12212,#231,.T.);
#15394=EDGE_CURVE('',#12217,#12218,#232,.T.);
#15395=EDGE_CURVE('',#12207,#12218,#233,.T.);
#15396=EDGE_CURVE('',#12218,#12219,#234,.T.);
#15397=EDGE_CURVE('',#12208,#12219,#235,.T.);
#15398=EDGE_CURVE('',#12220,#12221,#236,.T.);
#15399=EDGE_CURVE('',#12219,#12221,#237,.T.);
#15400=EDGE_CURVE('',#12218,#12220,#238,.T.);
#15401=EDGE_CURVE('',#12217,#12222,#10228,.T.);
#15402=EDGE_CURVE('',#12222,#12220,#239,.T.);
#15403=EDGE_CURVE('',#12222,#12216,#10229,.T.);
#15404=EDGE_CURVE('',#12223,#12224,#10230,.T.);
#15405=EDGE_CURVE('',#12225,#12224,#240,.T.);
#15406=EDGE_CURVE('',#12226,#12225,#241,.T.);
#15407=EDGE_CURVE('',#12226,#12223,#242,.T.);
#15408=EDGE_CURVE('',#12226,#12227,#243,.T.);
#15409=EDGE_CURVE('',#12227,#12228,#10231,.T.);
#15410=EDGE_CURVE('',#12223,#12228,#244,.T.);
#15411=EDGE_CURVE('',#12228,#12229,#10232,.T.);
#15412=EDGE_CURVE('',#12229,#12227,#10233,.T.);
#15413=EDGE_CURVE('',#12229,#12216,#10234,.T.);
#15414=EDGE_CURVE('',#12227,#12222,#10235,.T.);
#15415=EDGE_CURVE('',#12229,#12214,#245,.T.);
#15416=EDGE_CURVE('',#12214,#12230,#10236,.T.);
#15417=EDGE_CURVE('',#12228,#12230,#246,.T.);
#15418=EDGE_CURVE('',#12230,#12213,#10237,.T.);
#15419=EDGE_CURVE('',#12231,#12232,#247,.T.);
#15420=EDGE_CURVE('',#12233,#12232,#248,.T.);
#15421=EDGE_CURVE('',#12234,#12233,#10238,.T.);
#15422=EDGE_CURVE('',#12234,#12231,#249,.T.);
#15423=EDGE_CURVE('',#12231,#12213,#250,.T.);
#15424=EDGE_CURVE('',#12234,#12230,#251,.T.);
#15425=EDGE_CURVE('',#12223,#12234,#252,.T.);
#15426=EDGE_CURVE('',#12224,#12233,#253,.T.);
#15427=EDGE_CURVE('',#12235,#12236,#254,.T.);
#15428=EDGE_CURVE('',#12237,#12236,#255,.T.);
#15429=EDGE_CURVE('',#12238,#12237,#256,.T.);
#15430=EDGE_CURVE('',#12238,#12235,#257,.T.);
#15431=EDGE_CURVE('',#12239,#12238,#258,.T.);
#15432=EDGE_CURVE('',#12239,#12240,#10239,.T.);
#15433=EDGE_CURVE('',#12240,#12235,#259,.T.);
#15434=EDGE_CURVE('',#12241,#12242,#10240,.T.);
#15435=EDGE_CURVE('',#12242,#12243,#10241,.T.);
#15436=EDGE_CURVE('',#12243,#12239,#10242,.T.);
#15437=EDGE_CURVE('',#12241,#12239,#10243,.T.);
#15438=EDGE_CURVE('',#12240,#12243,#10244,.T.);
#15439=EDGE_CURVE('',#12244,#12243,#260,.T.);
#15440=EDGE_CURVE('',#12244,#12245,#10245,.T.);
#15441=EDGE_CURVE('',#12245,#12240,#261,.T.);
#15442=EDGE_CURVE('',#12245,#12246,#262,.T.);
#15443=EDGE_CURVE('',#12235,#12246,#263,.T.);
#15444=EDGE_CURVE('',#12246,#12247,#10246,.T.);
#15445=EDGE_CURVE('',#12236,#12247,#264,.T.);
#15446=EDGE_CURVE('',#12248,#12249,#265,.T.);
#15447=EDGE_CURVE('',#12247,#12249,#266,.T.);
#15448=EDGE_CURVE('',#12246,#12248,#267,.T.);
#15449=EDGE_CURVE('',#12245,#12250,#10247,.T.);
#15450=EDGE_CURVE('',#12250,#12248,#268,.T.);
#15451=EDGE_CURVE('',#12250,#12244,#10248,.T.);
#15452=EDGE_CURVE('',#12251,#12252,#269,.T.);
#15453=EDGE_CURVE('',#12253,#12252,#270,.T.);
#15454=EDGE_CURVE('',#12254,#12253,#271,.T.);
#15455=EDGE_CURVE('',#12254,#12251,#272,.T.);
#15456=EDGE_CURVE('',#12254,#12255,#273,.T.);
#15457=EDGE_CURVE('',#12255,#12256,#10249,.T.);
#15458=EDGE_CURVE('',#12251,#12256,#274,.T.);
#15459=EDGE_CURVE('',#12256,#12257,#10250,.T.);
#15460=EDGE_CURVE('',#12257,#12255,#10251,.T.);
#15461=EDGE_CURVE('',#12257,#12244,#10252,.T.);
#15462=EDGE_CURVE('',#12255,#12250,#10253,.T.);
#15463=EDGE_CURVE('',#12257,#12242,#275,.T.);
#15464=EDGE_CURVE('',#12242,#12258,#10254,.T.);
#15465=EDGE_CURVE('',#12256,#12258,#276,.T.);
#15466=EDGE_CURVE('',#12258,#12241,#10255,.T.);
#15467=EDGE_CURVE('',#12259,#12260,#277,.T.);
#15468=EDGE_CURVE('',#12261,#12260,#278,.T.);
#15469=EDGE_CURVE('',#12262,#12261,#279,.T.);
#15470=EDGE_CURVE('',#12262,#12259,#280,.T.);
#15471=EDGE_CURVE('',#12259,#12241,#281,.T.);
#15472=EDGE_CURVE('',#12262,#12258,#282,.T.);
#15473=EDGE_CURVE('',#12251,#12262,#283,.T.);
#15474=EDGE_CURVE('',#12252,#12261,#284,.T.);
#15475=EDGE_CURVE('',#12263,#12264,#285,.T.);
#15476=EDGE_CURVE('',#12265,#12264,#286,.T.);
#15477=EDGE_CURVE('',#12266,#12265,#287,.T.);
#15478=EDGE_CURVE('',#12266,#12263,#288,.T.);
#15479=EDGE_CURVE('',#12267,#12266,#289,.T.);
#15480=EDGE_CURVE('',#12267,#12268,#10256,.T.);
#15481=EDGE_CURVE('',#12268,#12263,#290,.T.);
#15482=EDGE_CURVE('',#12269,#12270,#10257,.T.);
#15483=EDGE_CURVE('',#12270,#12271,#10258,.T.);
#15484=EDGE_CURVE('',#12271,#12267,#10259,.T.);
#15485=EDGE_CURVE('',#12269,#12267,#10260,.T.);
#15486=EDGE_CURVE('',#12268,#12271,#10261,.T.);
#15487=EDGE_CURVE('',#12272,#12271,#291,.T.);
#15488=EDGE_CURVE('',#12272,#12273,#10262,.T.);
#15489=EDGE_CURVE('',#12273,#12268,#292,.T.);
#15490=EDGE_CURVE('',#12273,#12274,#293,.T.);
#15491=EDGE_CURVE('',#12263,#12274,#294,.T.);
#15492=EDGE_CURVE('',#12274,#12275,#295,.T.);
#15493=EDGE_CURVE('',#12264,#12275,#296,.T.);
#15494=EDGE_CURVE('',#12276,#12277,#297,.T.);
#15495=EDGE_CURVE('',#12275,#12277,#298,.T.);
#15496=EDGE_CURVE('',#12274,#12276,#299,.T.);
#15497=EDGE_CURVE('',#12273,#12278,#10263,.T.);
#15498=EDGE_CURVE('',#12278,#12276,#300,.T.);
#15499=EDGE_CURVE('',#12278,#12272,#10264,.T.);
#15500=EDGE_CURVE('',#12279,#12280,#10265,.T.);
#15501=EDGE_CURVE('',#12281,#12280,#301,.T.);
#15502=EDGE_CURVE('',#12282,#12281,#302,.T.);
#15503=EDGE_CURVE('',#12282,#12279,#303,.T.);
#15504=EDGE_CURVE('',#12282,#12283,#304,.T.);
#15505=EDGE_CURVE('',#12283,#12284,#10266,.T.);
#15506=EDGE_CURVE('',#12279,#12284,#305,.T.);
#15507=EDGE_CURVE('',#12284,#12285,#10267,.T.);
#15508=EDGE_CURVE('',#12285,#12283,#10268,.T.);
#15509=EDGE_CURVE('',#12285,#12272,#10269,.T.);
#15510=EDGE_CURVE('',#12283,#12278,#10270,.T.);
#15511=EDGE_CURVE('',#12285,#12270,#306,.T.);
#15512=EDGE_CURVE('',#12270,#12286,#10271,.T.);
#15513=EDGE_CURVE('',#12284,#12286,#307,.T.);
#15514=EDGE_CURVE('',#12286,#12269,#10272,.T.);
#15515=EDGE_CURVE('',#12287,#12288,#308,.T.);
#15516=EDGE_CURVE('',#12289,#12288,#309,.T.);
#15517=EDGE_CURVE('',#12290,#12289,#10273,.T.);
#15518=EDGE_CURVE('',#12290,#12287,#310,.T.);
#15519=EDGE_CURVE('',#12287,#12269,#311,.T.);
#15520=EDGE_CURVE('',#12290,#12286,#312,.T.);
#15521=EDGE_CURVE('',#12279,#12290,#313,.T.);
#15522=EDGE_CURVE('',#12280,#12289,#314,.T.);
#15523=EDGE_CURVE('',#12291,#12292,#315,.T.);
#15524=EDGE_CURVE('',#12291,#12293,#10274,.T.);
#15525=EDGE_CURVE('',#12293,#12294,#316,.T.);
#15526=EDGE_CURVE('',#12292,#12294,#317,.T.);
#15527=EDGE_CURVE('',#12294,#12295,#318,.T.);
#15528=EDGE_CURVE('',#12296,#12295,#319,.T.);
#15529=EDGE_CURVE('',#12292,#12296,#320,.T.);
#15530=EDGE_CURVE('',#12297,#12298,#321,.T.);
#15531=EDGE_CURVE('',#12295,#12298,#322,.T.);
#15532=EDGE_CURVE('',#12294,#12297,#323,.T.);
#15533=EDGE_CURVE('',#12299,#12293,#324,.T.);
#15534=EDGE_CURVE('',#12299,#12297,#325,.T.);
#15535=EDGE_CURVE('',#12293,#12300,#10275,.T.);
#15536=EDGE_CURVE('',#12301,#12300,#326,.T.);
#15537=EDGE_CURVE('',#12301,#12299,#10276,.T.);
#15538=EDGE_CURVE('',#12300,#12291,#10277,.T.);
#15539=EDGE_CURVE('',#12302,#12303,#10278,.T.);
#15540=EDGE_CURVE('',#12303,#12300,#10279,.T.);
#15541=EDGE_CURVE('',#12302,#12291,#10280,.T.);
#15542=EDGE_CURVE('',#12304,#12303,#327,.T.);
#15543=EDGE_CURVE('',#12304,#12301,#10281,.T.);
#15544=EDGE_CURVE('',#12303,#12305,#10282,.T.);
#15545=EDGE_CURVE('',#12306,#12305,#328,.T.);
#15546=EDGE_CURVE('',#12306,#12304,#10283,.T.);
#15547=EDGE_CURVE('',#12305,#12302,#10284,.T.);
#15548=EDGE_CURVE('',#12307,#12308,#329,.T.);
#15549=EDGE_CURVE('',#12309,#12308,#330,.T.);
#15550=EDGE_CURVE('',#12310,#12309,#10285,.T.);
#15551=EDGE_CURVE('',#12310,#12307,#331,.T.);
#15552=EDGE_CURVE('',#12307,#12302,#332,.T.);
#15553=EDGE_CURVE('',#12310,#12305,#333,.T.);
#15554=EDGE_CURVE('',#12311,#12306,#334,.T.);
#15555=EDGE_CURVE('',#12311,#12310,#335,.T.);
#15556=EDGE_CURVE('',#12312,#12309,#336,.T.);
#15557=EDGE_CURVE('',#12311,#12312,#10286,.T.);
#15558=EDGE_CURVE('',#12313,#12312,#337,.T.);
#15559=EDGE_CURVE('',#12314,#12313,#338,.T.);
#15560=EDGE_CURVE('',#12314,#12311,#339,.T.);
#15561=EDGE_CURVE('',#12314,#12315,#340,.T.);
#15562=EDGE_CURVE('',#12315,#12306,#10287,.T.);
#15563=EDGE_CURVE('',#12304,#12315,#10288,.T.);
#15564=EDGE_CURVE('',#12316,#12301,#10289,.T.);
#15565=EDGE_CURVE('',#12315,#12316,#10290,.T.);
#15566=EDGE_CURVE('',#12299,#12316,#10291,.T.);
#15567=EDGE_CURVE('',#12316,#12317,#341,.T.);
#15568=EDGE_CURVE('',#12297,#12317,#342,.T.);
#15569=EDGE_CURVE('',#12317,#12318,#343,.T.);
#15570=EDGE_CURVE('',#12298,#12318,#344,.T.);
#15571=EDGE_CURVE('',#12319,#12320,#10292,.T.);
#15572=EDGE_CURVE('',#12321,#12320,#345,.T.);
#15573=EDGE_CURVE('',#12322,#12321,#346,.T.);
#15574=EDGE_CURVE('',#12322,#12319,#347,.T.);
#15575=EDGE_CURVE('',#12323,#12322,#348,.T.);
#15576=EDGE_CURVE('',#12323,#12324,#10293,.T.);
#15577=EDGE_CURVE('',#12324,#12319,#349,.T.);
#15578=EDGE_CURVE('',#12325,#12326,#10294,.T.);
#15579=EDGE_CURVE('',#12326,#12327,#10295,.T.);
#15580=EDGE_CURVE('',#12327,#12323,#10296,.T.);
#15581=EDGE_CURVE('',#12325,#12323,#10297,.T.);
#15582=EDGE_CURVE('',#12324,#12327,#10298,.T.);
#15583=EDGE_CURVE('',#12328,#12327,#350,.T.);
#15584=EDGE_CURVE('',#12328,#12329,#10299,.T.);
#15585=EDGE_CURVE('',#12329,#12324,#351,.T.);
#15586=EDGE_CURVE('',#12329,#12330,#352,.T.);
#15587=EDGE_CURVE('',#12319,#12330,#353,.T.);
#15588=EDGE_CURVE('',#12330,#12331,#10300,.T.);
#15589=EDGE_CURVE('',#12320,#12331,#354,.T.);
#15590=EDGE_CURVE('',#12332,#12333,#355,.T.);
#15591=EDGE_CURVE('',#12331,#12333,#356,.T.);
#15592=EDGE_CURVE('',#12330,#12332,#357,.T.);
#15593=EDGE_CURVE('',#12329,#12334,#10301,.T.);
#15594=EDGE_CURVE('',#12334,#12332,#358,.T.);
#15595=EDGE_CURVE('',#12334,#12328,#10302,.T.);
#15596=EDGE_CURVE('',#12335,#12336,#359,.T.);
#15597=EDGE_CURVE('',#12337,#12336,#360,.T.);
#15598=EDGE_CURVE('',#12338,#12337,#361,.T.);
#15599=EDGE_CURVE('',#12338,#12335,#362,.T.);
#15600=EDGE_CURVE('',#12338,#12339,#363,.T.);
#15601=EDGE_CURVE('',#12339,#12340,#10303,.T.);
#15602=EDGE_CURVE('',#12335,#12340,#364,.T.);
#15603=EDGE_CURVE('',#12340,#12341,#10304,.T.);
#15604=EDGE_CURVE('',#12341,#12339,#10305,.T.);
#15605=EDGE_CURVE('',#12341,#12328,#10306,.T.);
#15606=EDGE_CURVE('',#12339,#12334,#10307,.T.);
#15607=EDGE_CURVE('',#12341,#12326,#365,.T.);
#15608=EDGE_CURVE('',#12326,#12342,#10308,.T.);
#15609=EDGE_CURVE('',#12340,#12342,#366,.T.);
#15610=EDGE_CURVE('',#12342,#12325,#10309,.T.);
#15611=EDGE_CURVE('',#12343,#12344,#367,.T.);
#15612=EDGE_CURVE('',#12345,#12344,#368,.T.);
#15613=EDGE_CURVE('',#12346,#12345,#10310,.T.);
#15614=EDGE_CURVE('',#12346,#12343,#369,.T.);
#15615=EDGE_CURVE('',#12343,#12325,#370,.T.);
#15616=EDGE_CURVE('',#12346,#12342,#371,.T.);
#15617=EDGE_CURVE('',#12335,#12346,#372,.T.);
#15618=EDGE_CURVE('',#12336,#12345,#373,.T.);
#15619=EDGE_CURVE('',#12125,#12308,#10311,.T.);
#15620=EDGE_CURVE('',#12313,#12137,#10312,.T.);
#15621=EDGE_CURVE('',#12153,#12148,#10313,.T.);
#15622=EDGE_CURVE('',#12141,#12165,#10314,.T.);
#15623=EDGE_CURVE('',#12181,#12176,#10315,.T.);
#15624=EDGE_CURVE('',#12169,#12193,#10316,.T.);
#15625=EDGE_CURVE('',#12209,#12204,#10317,.T.);
#15626=EDGE_CURVE('',#12197,#12221,#10318,.T.);
#15627=EDGE_CURVE('',#12237,#12232,#10319,.T.);
#15628=EDGE_CURVE('',#12225,#12249,#10320,.T.);
#15629=EDGE_CURVE('',#12265,#12260,#10321,.T.);
#15630=EDGE_CURVE('',#12253,#12277,#10322,.T.);
#15631=EDGE_CURVE('',#12321,#12288,#10323,.T.);
#15632=EDGE_CURVE('',#12281,#12333,#10324,.T.);
#15633=EDGE_CURVE('',#12296,#12344,#10325,.T.);
#15634=EDGE_CURVE('',#12337,#12318,#10326,.T.);
#15635=EDGE_CURVE('',#12347,#12347,#10327,.T.);
#15636=EDGE_CURVE('',#12348,#12348,#10328,.T.);
#15637=EDGE_CURVE('',#12348,#12347,#6894,.T.);
#15638=EDGE_CURVE('',#12349,#12349,#10329,.T.);
#15639=EDGE_CURVE('',#12350,#12350,#10330,.T.);
#15640=EDGE_CURVE('',#12350,#12349,#6895,.T.);
#15641=EDGE_CURVE('',#12351,#12351,#10331,.T.);
#15642=EDGE_CURVE('',#12352,#12352,#10332,.T.);
#15643=EDGE_CURVE('',#12352,#12351,#6896,.T.);
#15644=EDGE_CURVE('',#12353,#12353,#10333,.T.);
#15645=EDGE_CURVE('',#12354,#12354,#10334,.T.);
#15646=EDGE_CURVE('',#12354,#12353,#6897,.T.);
#15647=EDGE_CURVE('',#12355,#12355,#10335,.T.);
#15648=EDGE_CURVE('',#12355,#12356,#6898,.T.);
#15649=EDGE_CURVE('',#12356,#12356,#10336,.T.);
#15650=EDGE_CURVE('',#12357,#12357,#10337,.T.);
#15651=EDGE_CURVE('',#12357,#12358,#6899,.T.);
#15652=EDGE_CURVE('',#12358,#12358,#10338,.T.);
#15653=EDGE_CURVE('',#12359,#12359,#10339,.T.);
#15654=EDGE_CURVE('',#12359,#12360,#6900,.T.);
#15655=EDGE_CURVE('',#12360,#12360,#10340,.T.);
#21072=ORIENTED_EDGE('',*,*,#15229,.F.);
#21073=ORIENTED_EDGE('',*,*,#15229,.T.);
#21074=ORIENTED_EDGE('',*,*,#15230,.T.);
#21075=ORIENTED_EDGE('',*,*,#15231,.F.);
#21076=ORIENTED_EDGE('',*,*,#15230,.F.);
#21077=ORIENTED_EDGE('',*,*,#15232,.T.);
#21078=ORIENTED_EDGE('',*,*,#15233,.T.);
#21079=ORIENTED_EDGE('',*,*,#15234,.T.);
#21080=ORIENTED_EDGE('',*,*,#15232,.F.);
#21081=ORIENTED_EDGE('',*,*,#15234,.F.);
#21082=ORIENTED_EDGE('',*,*,#15235,.T.);
#21083=ORIENTED_EDGE('',*,*,#15236,.F.);
#21084=ORIENTED_EDGE('',*,*,#15237,.F.);
#21085=ORIENTED_EDGE('',*,*,#15238,.T.);
#21086=ORIENTED_EDGE('',*,*,#15239,.F.);
#21087=ORIENTED_EDGE('',*,*,#15240,.T.);
#21088=ORIENTED_EDGE('',*,*,#15241,.T.);
#21089=ORIENTED_EDGE('',*,*,#15238,.F.);
#21090=ORIENTED_EDGE('',*,*,#15242,.T.);
#21091=ORIENTED_EDGE('',*,*,#15243,.T.);
#21092=ORIENTED_EDGE('',*,*,#15244,.T.);
#21093=ORIENTED_EDGE('',*,*,#15245,.F.);
#21094=ORIENTED_EDGE('',*,*,#15240,.F.);
#21095=ORIENTED_EDGE('',*,*,#15244,.F.);
#21096=ORIENTED_EDGE('',*,*,#15246,.F.);
#21097=ORIENTED_EDGE('',*,*,#15246,.T.);
#21098=ORIENTED_EDGE('',*,*,#15247,.F.);
#21099=ORIENTED_EDGE('',*,*,#15248,.T.);
#21100=ORIENTED_EDGE('',*,*,#15249,.T.);
#21101=ORIENTED_EDGE('',*,*,#15241,.F.);
#21102=ORIENTED_EDGE('',*,*,#15249,.F.);
#21103=ORIENTED_EDGE('',*,*,#15250,.T.);
#21104=ORIENTED_EDGE('',*,*,#15251,.F.);
#21105=ORIENTED_EDGE('',*,*,#15252,.T.);
#21106=ORIENTED_EDGE('',*,*,#15253,.F.);
#21107=ORIENTED_EDGE('',*,*,#15235,.F.);
#21108=ORIENTED_EDGE('',*,*,#15251,.T.);
#21109=ORIENTED_EDGE('',*,*,#15254,.T.);
#21110=ORIENTED_EDGE('',*,*,#15255,.F.);
#21111=ORIENTED_EDGE('',*,*,#15252,.F.);
#21112=ORIENTED_EDGE('',*,*,#15256,.T.);
#21113=ORIENTED_EDGE('',*,*,#15250,.F.);
#21114=ORIENTED_EDGE('',*,*,#15257,.T.);
#21115=ORIENTED_EDGE('',*,*,#15258,.T.);
#21116=ORIENTED_EDGE('',*,*,#15256,.F.);
#21117=ORIENTED_EDGE('',*,*,#15248,.F.);
#21118=ORIENTED_EDGE('',*,*,#15259,.F.);
#21119=ORIENTED_EDGE('',*,*,#15257,.F.);
#21120=ORIENTED_EDGE('',*,*,#15260,.T.);
#21121=ORIENTED_EDGE('',*,*,#15261,.F.);
#21122=ORIENTED_EDGE('',*,*,#15262,.F.);
#21123=ORIENTED_EDGE('',*,*,#15263,.T.);
#21124=ORIENTED_EDGE('',*,*,#15264,.T.);
#21125=ORIENTED_EDGE('',*,*,#15265,.T.);
#21126=ORIENTED_EDGE('',*,*,#15266,.F.);
#21127=ORIENTED_EDGE('',*,*,#15263,.F.);
#21128=ORIENTED_EDGE('',*,*,#15267,.F.);
#21129=ORIENTED_EDGE('',*,*,#15265,.F.);
#21130=ORIENTED_EDGE('',*,*,#15268,.F.);
#21131=ORIENTED_EDGE('',*,*,#15259,.T.);
#21132=ORIENTED_EDGE('',*,*,#15269,.F.);
#21133=ORIENTED_EDGE('',*,*,#15268,.T.);
#21134=ORIENTED_EDGE('',*,*,#15270,.T.);
#21135=ORIENTED_EDGE('',*,*,#15247,.T.);
#21136=ORIENTED_EDGE('',*,*,#15243,.F.);
#21137=ORIENTED_EDGE('',*,*,#15271,.F.);
#21138=ORIENTED_EDGE('',*,*,#15269,.T.);
#21139=ORIENTED_EDGE('',*,*,#15272,.T.);
#21140=ORIENTED_EDGE('',*,*,#15273,.F.);
#21141=ORIENTED_EDGE('',*,*,#15267,.T.);
#21142=ORIENTED_EDGE('',*,*,#15271,.T.);
#21143=ORIENTED_EDGE('',*,*,#15274,.F.);
#21144=ORIENTED_EDGE('',*,*,#15272,.F.);
#21145=ORIENTED_EDGE('',*,*,#15242,.F.);
#21146=ORIENTED_EDGE('',*,*,#15275,.T.);
#21147=ORIENTED_EDGE('',*,*,#15276,.F.);
#21148=ORIENTED_EDGE('',*,*,#15277,.F.);
#21149=ORIENTED_EDGE('',*,*,#15278,.T.);
#21150=ORIENTED_EDGE('',*,*,#15279,.F.);
#21151=ORIENTED_EDGE('',*,*,#15278,.F.);
#21152=ORIENTED_EDGE('',*,*,#15280,.T.);
#21153=ORIENTED_EDGE('',*,*,#15274,.T.);
#21154=ORIENTED_EDGE('',*,*,#15266,.T.);
#21155=ORIENTED_EDGE('',*,*,#15273,.T.);
#21156=ORIENTED_EDGE('',*,*,#15280,.F.);
#21157=ORIENTED_EDGE('',*,*,#15281,.F.);
#21158=ORIENTED_EDGE('',*,*,#15277,.T.);
#21159=ORIENTED_EDGE('',*,*,#15282,.F.);
#21160=ORIENTED_EDGE('',*,*,#15260,.F.);
#21161=ORIENTED_EDGE('',*,*,#15281,.T.);
#21162=ORIENTED_EDGE('',*,*,#15283,.T.);
#21163=ORIENTED_EDGE('',*,*,#15284,.F.);
#21164=ORIENTED_EDGE('',*,*,#15285,.F.);
#21165=ORIENTED_EDGE('',*,*,#15286,.T.);
#21166=ORIENTED_EDGE('',*,*,#15287,.F.);
#21167=ORIENTED_EDGE('',*,*,#15288,.T.);
#21168=ORIENTED_EDGE('',*,*,#15289,.T.);
#21169=ORIENTED_EDGE('',*,*,#15286,.F.);
#21170=ORIENTED_EDGE('',*,*,#15290,.T.);
#21171=ORIENTED_EDGE('',*,*,#15291,.T.);
#21172=ORIENTED_EDGE('',*,*,#15292,.T.);
#21173=ORIENTED_EDGE('',*,*,#15293,.F.);
#21174=ORIENTED_EDGE('',*,*,#15288,.F.);
#21175=ORIENTED_EDGE('',*,*,#15292,.F.);
#21176=ORIENTED_EDGE('',*,*,#15294,.F.);
#21177=ORIENTED_EDGE('',*,*,#15294,.T.);
#21178=ORIENTED_EDGE('',*,*,#15295,.F.);
#21179=ORIENTED_EDGE('',*,*,#15296,.T.);
#21180=ORIENTED_EDGE('',*,*,#15297,.T.);
#21181=ORIENTED_EDGE('',*,*,#15289,.F.);
#21182=ORIENTED_EDGE('',*,*,#15297,.F.);
#21183=ORIENTED_EDGE('',*,*,#15298,.T.);
#21184=ORIENTED_EDGE('',*,*,#15299,.F.);
#21185=ORIENTED_EDGE('',*,*,#15300,.T.);
#21186=ORIENTED_EDGE('',*,*,#15301,.F.);
#21187=ORIENTED_EDGE('',*,*,#15283,.F.);
#21188=ORIENTED_EDGE('',*,*,#15299,.T.);
#21189=ORIENTED_EDGE('',*,*,#15302,.T.);
#21190=ORIENTED_EDGE('',*,*,#15303,.F.);
#21191=ORIENTED_EDGE('',*,*,#15300,.F.);
#21192=ORIENTED_EDGE('',*,*,#15304,.T.);
#21193=ORIENTED_EDGE('',*,*,#15298,.F.);
#21194=ORIENTED_EDGE('',*,*,#15305,.T.);
#21195=ORIENTED_EDGE('',*,*,#15306,.T.);
#21196=ORIENTED_EDGE('',*,*,#15304,.F.);
#21197=ORIENTED_EDGE('',*,*,#15296,.F.);
#21198=ORIENTED_EDGE('',*,*,#15307,.F.);
#21199=ORIENTED_EDGE('',*,*,#15305,.F.);
#21200=ORIENTED_EDGE('',*,*,#15308,.T.);
#21201=ORIENTED_EDGE('',*,*,#15309,.F.);
#21202=ORIENTED_EDGE('',*,*,#15310,.F.);
#21203=ORIENTED_EDGE('',*,*,#15311,.T.);
#21204=ORIENTED_EDGE('',*,*,#15312,.T.);
#21205=ORIENTED_EDGE('',*,*,#15313,.T.);
#21206=ORIENTED_EDGE('',*,*,#15314,.F.);
#21207=ORIENTED_EDGE('',*,*,#15311,.F.);
#21208=ORIENTED_EDGE('',*,*,#15315,.F.);
#21209=ORIENTED_EDGE('',*,*,#15313,.F.);
#21210=ORIENTED_EDGE('',*,*,#15316,.F.);
#21211=ORIENTED_EDGE('',*,*,#15307,.T.);
#21212=ORIENTED_EDGE('',*,*,#15317,.F.);
#21213=ORIENTED_EDGE('',*,*,#15316,.T.);
#21214=ORIENTED_EDGE('',*,*,#15318,.T.);
#21215=ORIENTED_EDGE('',*,*,#15295,.T.);
#21216=ORIENTED_EDGE('',*,*,#15291,.F.);
#21217=ORIENTED_EDGE('',*,*,#15319,.F.);
#21218=ORIENTED_EDGE('',*,*,#15317,.T.);
#21219=ORIENTED_EDGE('',*,*,#15320,.T.);
#21220=ORIENTED_EDGE('',*,*,#15321,.F.);
#21221=ORIENTED_EDGE('',*,*,#15315,.T.);
#21222=ORIENTED_EDGE('',*,*,#15319,.T.);
#21223=ORIENTED_EDGE('',*,*,#15322,.F.);
#21224=ORIENTED_EDGE('',*,*,#15320,.F.);
#21225=ORIENTED_EDGE('',*,*,#15290,.F.);
#21226=ORIENTED_EDGE('',*,*,#15323,.T.);
#21227=ORIENTED_EDGE('',*,*,#15324,.F.);
#21228=ORIENTED_EDGE('',*,*,#15325,.F.);
#21229=ORIENTED_EDGE('',*,*,#15326,.T.);
#21230=ORIENTED_EDGE('',*,*,#15327,.F.);
#21231=ORIENTED_EDGE('',*,*,#15326,.F.);
#21232=ORIENTED_EDGE('',*,*,#15328,.T.);
#21233=ORIENTED_EDGE('',*,*,#15322,.T.);
#21234=ORIENTED_EDGE('',*,*,#15314,.T.);
#21235=ORIENTED_EDGE('',*,*,#15321,.T.);
#21236=ORIENTED_EDGE('',*,*,#15328,.F.);
#21237=ORIENTED_EDGE('',*,*,#15329,.F.);
#21238=ORIENTED_EDGE('',*,*,#15325,.T.);
#21239=ORIENTED_EDGE('',*,*,#15330,.F.);
#21240=ORIENTED_EDGE('',*,*,#15308,.F.);
#21241=ORIENTED_EDGE('',*,*,#15329,.T.);
#21242=ORIENTED_EDGE('',*,*,#15331,.T.);
#21243=ORIENTED_EDGE('',*,*,#15332,.F.);
#21244=ORIENTED_EDGE('',*,*,#15333,.F.);
#21245=ORIENTED_EDGE('',*,*,#15334,.T.);
#21246=ORIENTED_EDGE('',*,*,#15335,.F.);
#21247=ORIENTED_EDGE('',*,*,#15336,.T.);
#21248=ORIENTED_EDGE('',*,*,#15337,.T.);
#21249=ORIENTED_EDGE('',*,*,#15334,.F.);
#21250=ORIENTED_EDGE('',*,*,#15338,.T.);
#21251=ORIENTED_EDGE('',*,*,#15339,.T.);
#21252=ORIENTED_EDGE('',*,*,#15340,.T.);
#21253=ORIENTED_EDGE('',*,*,#15341,.F.);
#21254=ORIENTED_EDGE('',*,*,#15336,.F.);
#21255=ORIENTED_EDGE('',*,*,#15340,.F.);
#21256=ORIENTED_EDGE('',*,*,#15342,.F.);
#21257=ORIENTED_EDGE('',*,*,#15342,.T.);
#21258=ORIENTED_EDGE('',*,*,#15343,.F.);
#21259=ORIENTED_EDGE('',*,*,#15344,.T.);
#21260=ORIENTED_EDGE('',*,*,#15345,.T.);
#21261=ORIENTED_EDGE('',*,*,#15337,.F.);
#21262=ORIENTED_EDGE('',*,*,#15345,.F.);
#21263=ORIENTED_EDGE('',*,*,#15346,.T.);
#21264=ORIENTED_EDGE('',*,*,#15347,.F.);
#21265=ORIENTED_EDGE('',*,*,#15348,.T.);
#21266=ORIENTED_EDGE('',*,*,#15349,.F.);
#21267=ORIENTED_EDGE('',*,*,#15331,.F.);
#21268=ORIENTED_EDGE('',*,*,#15347,.T.);
#21269=ORIENTED_EDGE('',*,*,#15350,.T.);
#21270=ORIENTED_EDGE('',*,*,#15351,.F.);
#21271=ORIENTED_EDGE('',*,*,#15348,.F.);
#21272=ORIENTED_EDGE('',*,*,#15352,.T.);
#21273=ORIENTED_EDGE('',*,*,#15346,.F.);
#21274=ORIENTED_EDGE('',*,*,#15353,.T.);
#21275=ORIENTED_EDGE('',*,*,#15354,.T.);
#21276=ORIENTED_EDGE('',*,*,#15352,.F.);
#21277=ORIENTED_EDGE('',*,*,#15344,.F.);
#21278=ORIENTED_EDGE('',*,*,#15355,.F.);
#21279=ORIENTED_EDGE('',*,*,#15353,.F.);
#21280=ORIENTED_EDGE('',*,*,#15356,.T.);
#21281=ORIENTED_EDGE('',*,*,#15357,.F.);
#21282=ORIENTED_EDGE('',*,*,#15358,.F.);
#21283=ORIENTED_EDGE('',*,*,#15359,.T.);
#21284=ORIENTED_EDGE('',*,*,#15360,.T.);
#21285=ORIENTED_EDGE('',*,*,#15361,.T.);
#21286=ORIENTED_EDGE('',*,*,#15362,.F.);
#21287=ORIENTED_EDGE('',*,*,#15359,.F.);
#21288=ORIENTED_EDGE('',*,*,#15363,.F.);
#21289=ORIENTED_EDGE('',*,*,#15361,.F.);
#21290=ORIENTED_EDGE('',*,*,#15364,.F.);
#21291=ORIENTED_EDGE('',*,*,#15355,.T.);
#21292=ORIENTED_EDGE('',*,*,#15365,.F.);
#21293=ORIENTED_EDGE('',*,*,#15364,.T.);
#21294=ORIENTED_EDGE('',*,*,#15366,.T.);
#21295=ORIENTED_EDGE('',*,*,#15343,.T.);
#21296=ORIENTED_EDGE('',*,*,#15339,.F.);
#21297=ORIENTED_EDGE('',*,*,#15367,.F.);
#21298=ORIENTED_EDGE('',*,*,#15365,.T.);
#21299=ORIENTED_EDGE('',*,*,#15368,.T.);
#21300=ORIENTED_EDGE('',*,*,#15369,.F.);
#21301=ORIENTED_EDGE('',*,*,#15363,.T.);
#21302=ORIENTED_EDGE('',*,*,#15367,.T.);
#21303=ORIENTED_EDGE('',*,*,#15370,.F.);
#21304=ORIENTED_EDGE('',*,*,#15368,.F.);
#21305=ORIENTED_EDGE('',*,*,#15338,.F.);
#21306=ORIENTED_EDGE('',*,*,#15371,.T.);
#21307=ORIENTED_EDGE('',*,*,#15372,.F.);
#21308=ORIENTED_EDGE('',*,*,#15373,.F.);
#21309=ORIENTED_EDGE('',*,*,#15374,.T.);
#21310=ORIENTED_EDGE('',*,*,#15375,.F.);
#21311=ORIENTED_EDGE('',*,*,#15374,.F.);
#21312=ORIENTED_EDGE('',*,*,#15376,.T.);
#21313=ORIENTED_EDGE('',*,*,#15370,.T.);
#21314=ORIENTED_EDGE('',*,*,#15362,.T.);
#21315=ORIENTED_EDGE('',*,*,#15369,.T.);
#21316=ORIENTED_EDGE('',*,*,#15376,.F.);
#21317=ORIENTED_EDGE('',*,*,#15377,.F.);
#21318=ORIENTED_EDGE('',*,*,#15373,.T.);
#21319=ORIENTED_EDGE('',*,*,#15378,.F.);
#21320=ORIENTED_EDGE('',*,*,#15356,.F.);
#21321=ORIENTED_EDGE('',*,*,#15377,.T.);
#21322=ORIENTED_EDGE('',*,*,#15379,.T.);
#21323=ORIENTED_EDGE('',*,*,#15380,.F.);
#21324=ORIENTED_EDGE('',*,*,#15381,.F.);
#21325=ORIENTED_EDGE('',*,*,#15382,.T.);
#21326=ORIENTED_EDGE('',*,*,#15383,.F.);
#21327=ORIENTED_EDGE('',*,*,#15384,.T.);
#21328=ORIENTED_EDGE('',*,*,#15385,.T.);
#21329=ORIENTED_EDGE('',*,*,#15382,.F.);
#21330=ORIENTED_EDGE('',*,*,#15386,.T.);
#21331=ORIENTED_EDGE('',*,*,#15387,.T.);
#21332=ORIENTED_EDGE('',*,*,#15388,.T.);
#21333=ORIENTED_EDGE('',*,*,#15389,.F.);
#21334=ORIENTED_EDGE('',*,*,#15384,.F.);
#21335=ORIENTED_EDGE('',*,*,#15388,.F.);
#21336=ORIENTED_EDGE('',*,*,#15390,.F.);
#21337=ORIENTED_EDGE('',*,*,#15390,.T.);
#21338=ORIENTED_EDGE('',*,*,#15391,.F.);
#21339=ORIENTED_EDGE('',*,*,#15392,.T.);
#21340=ORIENTED_EDGE('',*,*,#15393,.T.);
#21341=ORIENTED_EDGE('',*,*,#15385,.F.);
#21342=ORIENTED_EDGE('',*,*,#15393,.F.);
#21343=ORIENTED_EDGE('',*,*,#15394,.T.);
#21344=ORIENTED_EDGE('',*,*,#15395,.F.);
#21345=ORIENTED_EDGE('',*,*,#15396,.T.);
#21346=ORIENTED_EDGE('',*,*,#15397,.F.);
#21347=ORIENTED_EDGE('',*,*,#15379,.F.);
#21348=ORIENTED_EDGE('',*,*,#15395,.T.);
#21349=ORIENTED_EDGE('',*,*,#15398,.T.);
#21350=ORIENTED_EDGE('',*,*,#15399,.F.);
#21351=ORIENTED_EDGE('',*,*,#15396,.F.);
#21352=ORIENTED_EDGE('',*,*,#15400,.T.);
#21353=ORIENTED_EDGE('',*,*,#15394,.F.);
#21354=ORIENTED_EDGE('',*,*,#15401,.T.);
#21355=ORIENTED_EDGE('',*,*,#15402,.T.);
#21356=ORIENTED_EDGE('',*,*,#15400,.F.);
#21357=ORIENTED_EDGE('',*,*,#15392,.F.);
#21358=ORIENTED_EDGE('',*,*,#15403,.F.);
#21359=ORIENTED_EDGE('',*,*,#15401,.F.);
#21360=ORIENTED_EDGE('',*,*,#15404,.T.);
#21361=ORIENTED_EDGE('',*,*,#15405,.F.);
#21362=ORIENTED_EDGE('',*,*,#15406,.F.);
#21363=ORIENTED_EDGE('',*,*,#15407,.T.);
#21364=ORIENTED_EDGE('',*,*,#15408,.T.);
#21365=ORIENTED_EDGE('',*,*,#15409,.T.);
#21366=ORIENTED_EDGE('',*,*,#15410,.F.);
#21367=ORIENTED_EDGE('',*,*,#15407,.F.);
#21368=ORIENTED_EDGE('',*,*,#15411,.F.);
#21369=ORIENTED_EDGE('',*,*,#15409,.F.);
#21370=ORIENTED_EDGE('',*,*,#15412,.F.);
#21371=ORIENTED_EDGE('',*,*,#15403,.T.);
#21372=ORIENTED_EDGE('',*,*,#15413,.F.);
#21373=ORIENTED_EDGE('',*,*,#15412,.T.);
#21374=ORIENTED_EDGE('',*,*,#15414,.T.);
#21375=ORIENTED_EDGE('',*,*,#15391,.T.);
#21376=ORIENTED_EDGE('',*,*,#15387,.F.);
#21377=ORIENTED_EDGE('',*,*,#15415,.F.);
#21378=ORIENTED_EDGE('',*,*,#15413,.T.);
#21379=ORIENTED_EDGE('',*,*,#15416,.T.);
#21380=ORIENTED_EDGE('',*,*,#15417,.F.);
#21381=ORIENTED_EDGE('',*,*,#15411,.T.);
#21382=ORIENTED_EDGE('',*,*,#15415,.T.);
#21383=ORIENTED_EDGE('',*,*,#15418,.F.);
#21384=ORIENTED_EDGE('',*,*,#15416,.F.);
#21385=ORIENTED_EDGE('',*,*,#15386,.F.);
#21386=ORIENTED_EDGE('',*,*,#15419,.T.);
#21387=ORIENTED_EDGE('',*,*,#15420,.F.);
#21388=ORIENTED_EDGE('',*,*,#15421,.F.);
#21389=ORIENTED_EDGE('',*,*,#15422,.T.);
#21390=ORIENTED_EDGE('',*,*,#15423,.F.);
#21391=ORIENTED_EDGE('',*,*,#15422,.F.);
#21392=ORIENTED_EDGE('',*,*,#15424,.T.);
#21393=ORIENTED_EDGE('',*,*,#15418,.T.);
#21394=ORIENTED_EDGE('',*,*,#15410,.T.);
#21395=ORIENTED_EDGE('',*,*,#15417,.T.);
#21396=ORIENTED_EDGE('',*,*,#15424,.F.);
#21397=ORIENTED_EDGE('',*,*,#15425,.F.);
#21398=ORIENTED_EDGE('',*,*,#15421,.T.);
#21399=ORIENTED_EDGE('',*,*,#15426,.F.);
#21400=ORIENTED_EDGE('',*,*,#15404,.F.);
#21401=ORIENTED_EDGE('',*,*,#15425,.T.);
#21402=ORIENTED_EDGE('',*,*,#15427,.T.);
#21403=ORIENTED_EDGE('',*,*,#15428,.F.);
#21404=ORIENTED_EDGE('',*,*,#15429,.F.);
#21405=ORIENTED_EDGE('',*,*,#15430,.T.);
#21406=ORIENTED_EDGE('',*,*,#15431,.F.);
#21407=ORIENTED_EDGE('',*,*,#15432,.T.);
#21408=ORIENTED_EDGE('',*,*,#15433,.T.);
#21409=ORIENTED_EDGE('',*,*,#15430,.F.);
#21410=ORIENTED_EDGE('',*,*,#15434,.T.);
#21411=ORIENTED_EDGE('',*,*,#15435,.T.);
#21412=ORIENTED_EDGE('',*,*,#15436,.T.);
#21413=ORIENTED_EDGE('',*,*,#15437,.F.);
#21414=ORIENTED_EDGE('',*,*,#15432,.F.);
#21415=ORIENTED_EDGE('',*,*,#15436,.F.);
#21416=ORIENTED_EDGE('',*,*,#15438,.F.);
#21417=ORIENTED_EDGE('',*,*,#15438,.T.);
#21418=ORIENTED_EDGE('',*,*,#15439,.F.);
#21419=ORIENTED_EDGE('',*,*,#15440,.T.);
#21420=ORIENTED_EDGE('',*,*,#15441,.T.);
#21421=ORIENTED_EDGE('',*,*,#15433,.F.);
#21422=ORIENTED_EDGE('',*,*,#15441,.F.);
#21423=ORIENTED_EDGE('',*,*,#15442,.T.);
#21424=ORIENTED_EDGE('',*,*,#15443,.F.);
#21425=ORIENTED_EDGE('',*,*,#15444,.T.);
#21426=ORIENTED_EDGE('',*,*,#15445,.F.);
#21427=ORIENTED_EDGE('',*,*,#15427,.F.);
#21428=ORIENTED_EDGE('',*,*,#15443,.T.);
#21429=ORIENTED_EDGE('',*,*,#15446,.T.);
#21430=ORIENTED_EDGE('',*,*,#15447,.F.);
#21431=ORIENTED_EDGE('',*,*,#15444,.F.);
#21432=ORIENTED_EDGE('',*,*,#15448,.T.);
#21433=ORIENTED_EDGE('',*,*,#15442,.F.);
#21434=ORIENTED_EDGE('',*,*,#15449,.T.);
#21435=ORIENTED_EDGE('',*,*,#15450,.T.);
#21436=ORIENTED_EDGE('',*,*,#15448,.F.);
#21437=ORIENTED_EDGE('',*,*,#15440,.F.);
#21438=ORIENTED_EDGE('',*,*,#15451,.F.);
#21439=ORIENTED_EDGE('',*,*,#15449,.F.);
#21440=ORIENTED_EDGE('',*,*,#15452,.T.);
#21441=ORIENTED_EDGE('',*,*,#15453,.F.);
#21442=ORIENTED_EDGE('',*,*,#15454,.F.);
#21443=ORIENTED_EDGE('',*,*,#15455,.T.);
#21444=ORIENTED_EDGE('',*,*,#15456,.T.);
#21445=ORIENTED_EDGE('',*,*,#15457,.T.);
#21446=ORIENTED_EDGE('',*,*,#15458,.F.);
#21447=ORIENTED_EDGE('',*,*,#15455,.F.);
#21448=ORIENTED_EDGE('',*,*,#15459,.F.);
#21449=ORIENTED_EDGE('',*,*,#15457,.F.);
#21450=ORIENTED_EDGE('',*,*,#15460,.F.);
#21451=ORIENTED_EDGE('',*,*,#15451,.T.);
#21452=ORIENTED_EDGE('',*,*,#15461,.F.);
#21453=ORIENTED_EDGE('',*,*,#15460,.T.);
#21454=ORIENTED_EDGE('',*,*,#15462,.T.);
#21455=ORIENTED_EDGE('',*,*,#15439,.T.);
#21456=ORIENTED_EDGE('',*,*,#15435,.F.);
#21457=ORIENTED_EDGE('',*,*,#15463,.F.);
#21458=ORIENTED_EDGE('',*,*,#15461,.T.);
#21459=ORIENTED_EDGE('',*,*,#15464,.T.);
#21460=ORIENTED_EDGE('',*,*,#15465,.F.);
#21461=ORIENTED_EDGE('',*,*,#15459,.T.);
#21462=ORIENTED_EDGE('',*,*,#15463,.T.);
#21463=ORIENTED_EDGE('',*,*,#15466,.F.);
#21464=ORIENTED_EDGE('',*,*,#15464,.F.);
#21465=ORIENTED_EDGE('',*,*,#15434,.F.);
#21466=ORIENTED_EDGE('',*,*,#15467,.T.);
#21467=ORIENTED_EDGE('',*,*,#15468,.F.);
#21468=ORIENTED_EDGE('',*,*,#15469,.F.);
#21469=ORIENTED_EDGE('',*,*,#15470,.T.);
#21470=ORIENTED_EDGE('',*,*,#15471,.F.);
#21471=ORIENTED_EDGE('',*,*,#15470,.F.);
#21472=ORIENTED_EDGE('',*,*,#15472,.T.);
#21473=ORIENTED_EDGE('',*,*,#15466,.T.);
#21474=ORIENTED_EDGE('',*,*,#15458,.T.);
#21475=ORIENTED_EDGE('',*,*,#15465,.T.);
#21476=ORIENTED_EDGE('',*,*,#15472,.F.);
#21477=ORIENTED_EDGE('',*,*,#15473,.F.);
#21478=ORIENTED_EDGE('',*,*,#15469,.T.);
#21479=ORIENTED_EDGE('',*,*,#15474,.F.);
#21480=ORIENTED_EDGE('',*,*,#15452,.F.);
#21481=ORIENTED_EDGE('',*,*,#15473,.T.);
#21482=ORIENTED_EDGE('',*,*,#15475,.T.);
#21483=ORIENTED_EDGE('',*,*,#15476,.F.);
#21484=ORIENTED_EDGE('',*,*,#15477,.F.);
#21485=ORIENTED_EDGE('',*,*,#15478,.T.);
#21486=ORIENTED_EDGE('',*,*,#15479,.F.);
#21487=ORIENTED_EDGE('',*,*,#15480,.T.);
#21488=ORIENTED_EDGE('',*,*,#15481,.T.);
#21489=ORIENTED_EDGE('',*,*,#15478,.F.);
#21490=ORIENTED_EDGE('',*,*,#15482,.T.);
#21491=ORIENTED_EDGE('',*,*,#15483,.T.);
#21492=ORIENTED_EDGE('',*,*,#15484,.T.);
#21493=ORIENTED_EDGE('',*,*,#15485,.F.);
#21494=ORIENTED_EDGE('',*,*,#15480,.F.);
#21495=ORIENTED_EDGE('',*,*,#15484,.F.);
#21496=ORIENTED_EDGE('',*,*,#15486,.F.);
#21497=ORIENTED_EDGE('',*,*,#15486,.T.);
#21498=ORIENTED_EDGE('',*,*,#15487,.F.);
#21499=ORIENTED_EDGE('',*,*,#15488,.T.);
#21500=ORIENTED_EDGE('',*,*,#15489,.T.);
#21501=ORIENTED_EDGE('',*,*,#15481,.F.);
#21502=ORIENTED_EDGE('',*,*,#15489,.F.);
#21503=ORIENTED_EDGE('',*,*,#15490,.T.);
#21504=ORIENTED_EDGE('',*,*,#15491,.F.);
#21505=ORIENTED_EDGE('',*,*,#15492,.T.);
#21506=ORIENTED_EDGE('',*,*,#15493,.F.);
#21507=ORIENTED_EDGE('',*,*,#15475,.F.);
#21508=ORIENTED_EDGE('',*,*,#15491,.T.);
#21509=ORIENTED_EDGE('',*,*,#15494,.T.);
#21510=ORIENTED_EDGE('',*,*,#15495,.F.);
#21511=ORIENTED_EDGE('',*,*,#15492,.F.);
#21512=ORIENTED_EDGE('',*,*,#15496,.T.);
#21513=ORIENTED_EDGE('',*,*,#15490,.F.);
#21514=ORIENTED_EDGE('',*,*,#15497,.T.);
#21515=ORIENTED_EDGE('',*,*,#15498,.T.);
#21516=ORIENTED_EDGE('',*,*,#15496,.F.);
#21517=ORIENTED_EDGE('',*,*,#15488,.F.);
#21518=ORIENTED_EDGE('',*,*,#15499,.F.);
#21519=ORIENTED_EDGE('',*,*,#15497,.F.);
#21520=ORIENTED_EDGE('',*,*,#15500,.T.);
#21521=ORIENTED_EDGE('',*,*,#15501,.F.);
#21522=ORIENTED_EDGE('',*,*,#15502,.F.);
#21523=ORIENTED_EDGE('',*,*,#15503,.T.);
#21524=ORIENTED_EDGE('',*,*,#15504,.T.);
#21525=ORIENTED_EDGE('',*,*,#15505,.T.);
#21526=ORIENTED_EDGE('',*,*,#15506,.F.);
#21527=ORIENTED_EDGE('',*,*,#15503,.F.);
#21528=ORIENTED_EDGE('',*,*,#15507,.F.);
#21529=ORIENTED_EDGE('',*,*,#15505,.F.);
#21530=ORIENTED_EDGE('',*,*,#15508,.F.);
#21531=ORIENTED_EDGE('',*,*,#15499,.T.);
#21532=ORIENTED_EDGE('',*,*,#15509,.F.);
#21533=ORIENTED_EDGE('',*,*,#15508,.T.);
#21534=ORIENTED_EDGE('',*,*,#15510,.T.);
#21535=ORIENTED_EDGE('',*,*,#15487,.T.);
#21536=ORIENTED_EDGE('',*,*,#15483,.F.);
#21537=ORIENTED_EDGE('',*,*,#15511,.F.);
#21538=ORIENTED_EDGE('',*,*,#15509,.T.);
#21539=ORIENTED_EDGE('',*,*,#15512,.T.);
#21540=ORIENTED_EDGE('',*,*,#15513,.F.);
#21541=ORIENTED_EDGE('',*,*,#15507,.T.);
#21542=ORIENTED_EDGE('',*,*,#15511,.T.);
#21543=ORIENTED_EDGE('',*,*,#15514,.F.);
#21544=ORIENTED_EDGE('',*,*,#15512,.F.);
#21545=ORIENTED_EDGE('',*,*,#15482,.F.);
#21546=ORIENTED_EDGE('',*,*,#15515,.T.);
#21547=ORIENTED_EDGE('',*,*,#15516,.F.);
#21548=ORIENTED_EDGE('',*,*,#15517,.F.);
#21549=ORIENTED_EDGE('',*,*,#15518,.T.);
#21550=ORIENTED_EDGE('',*,*,#15519,.F.);
#21551=ORIENTED_EDGE('',*,*,#15518,.F.);
#21552=ORIENTED_EDGE('',*,*,#15520,.T.);
#21553=ORIENTED_EDGE('',*,*,#15514,.T.);
#21554=ORIENTED_EDGE('',*,*,#15506,.T.);
#21555=ORIENTED_EDGE('',*,*,#15513,.T.);
#21556=ORIENTED_EDGE('',*,*,#15520,.F.);
#21557=ORIENTED_EDGE('',*,*,#15521,.F.);
#21558=ORIENTED_EDGE('',*,*,#15517,.T.);
#21559=ORIENTED_EDGE('',*,*,#15522,.F.);
#21560=ORIENTED_EDGE('',*,*,#15500,.F.);
#21561=ORIENTED_EDGE('',*,*,#15521,.T.);
#21562=ORIENTED_EDGE('',*,*,#15523,.F.);
#21563=ORIENTED_EDGE('',*,*,#15524,.T.);
#21564=ORIENTED_EDGE('',*,*,#15525,.T.);
#21565=ORIENTED_EDGE('',*,*,#15526,.F.);
#21566=ORIENTED_EDGE('',*,*,#15527,.T.);
#21567=ORIENTED_EDGE('',*,*,#15528,.F.);
#21568=ORIENTED_EDGE('',*,*,#15529,.F.);
#21569=ORIENTED_EDGE('',*,*,#15526,.T.);
#21570=ORIENTED_EDGE('',*,*,#15530,.T.);
#21571=ORIENTED_EDGE('',*,*,#15531,.F.);
#21572=ORIENTED_EDGE('',*,*,#15527,.F.);
#21573=ORIENTED_EDGE('',*,*,#15532,.T.);
#21574=ORIENTED_EDGE('',*,*,#15525,.F.);
#21575=ORIENTED_EDGE('',*,*,#15533,.F.);
#21576=ORIENTED_EDGE('',*,*,#15534,.T.);
#21577=ORIENTED_EDGE('',*,*,#15532,.F.);
#21578=ORIENTED_EDGE('',*,*,#15535,.T.);
#21579=ORIENTED_EDGE('',*,*,#15536,.F.);
#21580=ORIENTED_EDGE('',*,*,#15537,.T.);
#21581=ORIENTED_EDGE('',*,*,#15533,.T.);
#21582=ORIENTED_EDGE('',*,*,#15524,.F.);
#21583=ORIENTED_EDGE('',*,*,#15538,.F.);
#21584=ORIENTED_EDGE('',*,*,#15535,.F.);
#21585=ORIENTED_EDGE('',*,*,#15539,.T.);
#21586=ORIENTED_EDGE('',*,*,#15540,.T.);
#21587=ORIENTED_EDGE('',*,*,#15538,.T.);
#21588=ORIENTED_EDGE('',*,*,#15541,.F.);
#21589=ORIENTED_EDGE('',*,*,#15536,.T.);
#21590=ORIENTED_EDGE('',*,*,#15540,.F.);
#21591=ORIENTED_EDGE('',*,*,#15542,.F.);
#21592=ORIENTED_EDGE('',*,*,#15543,.T.);
#21593=ORIENTED_EDGE('',*,*,#15544,.T.);
#21594=ORIENTED_EDGE('',*,*,#15545,.F.);
#21595=ORIENTED_EDGE('',*,*,#15546,.T.);
#21596=ORIENTED_EDGE('',*,*,#15542,.T.);
#21597=ORIENTED_EDGE('',*,*,#15547,.F.);
#21598=ORIENTED_EDGE('',*,*,#15544,.F.);
#21599=ORIENTED_EDGE('',*,*,#15539,.F.);
#21600=ORIENTED_EDGE('',*,*,#15548,.T.);
#21601=ORIENTED_EDGE('',*,*,#15549,.F.);
#21602=ORIENTED_EDGE('',*,*,#15550,.F.);
#21603=ORIENTED_EDGE('',*,*,#15551,.T.);
#21604=ORIENTED_EDGE('',*,*,#15552,.F.);
#21605=ORIENTED_EDGE('',*,*,#15551,.F.);
#21606=ORIENTED_EDGE('',*,*,#15553,.T.);
#21607=ORIENTED_EDGE('',*,*,#15547,.T.);
#21608=ORIENTED_EDGE('',*,*,#15554,.T.);
#21609=ORIENTED_EDGE('',*,*,#15545,.T.);
#21610=ORIENTED_EDGE('',*,*,#15553,.F.);
#21611=ORIENTED_EDGE('',*,*,#15555,.F.);
#21612=ORIENTED_EDGE('',*,*,#15550,.T.);
#21613=ORIENTED_EDGE('',*,*,#15556,.F.);
#21614=ORIENTED_EDGE('',*,*,#15557,.F.);
#21615=ORIENTED_EDGE('',*,*,#15555,.T.);
#21616=ORIENTED_EDGE('',*,*,#15557,.T.);
#21617=ORIENTED_EDGE('',*,*,#15558,.F.);
#21618=ORIENTED_EDGE('',*,*,#15559,.F.);
#21619=ORIENTED_EDGE('',*,*,#15560,.T.);
#21620=ORIENTED_EDGE('',*,*,#15561,.T.);
#21621=ORIENTED_EDGE('',*,*,#15562,.T.);
#21622=ORIENTED_EDGE('',*,*,#15554,.F.);
#21623=ORIENTED_EDGE('',*,*,#15560,.F.);
#21624=ORIENTED_EDGE('',*,*,#15546,.F.);
#21625=ORIENTED_EDGE('',*,*,#15562,.F.);
#21626=ORIENTED_EDGE('',*,*,#15563,.F.);
#21627=ORIENTED_EDGE('',*,*,#15564,.T.);
#21628=ORIENTED_EDGE('',*,*,#15543,.F.);
#21629=ORIENTED_EDGE('',*,*,#15563,.T.);
#21630=ORIENTED_EDGE('',*,*,#15565,.T.);
#21631=ORIENTED_EDGE('',*,*,#15537,.F.);
#21632=ORIENTED_EDGE('',*,*,#15564,.F.);
#21633=ORIENTED_EDGE('',*,*,#15566,.F.);
#21634=ORIENTED_EDGE('',*,*,#15534,.F.);
#21635=ORIENTED_EDGE('',*,*,#15566,.T.);
#21636=ORIENTED_EDGE('',*,*,#15567,.T.);
#21637=ORIENTED_EDGE('',*,*,#15568,.F.);
#21638=ORIENTED_EDGE('',*,*,#15569,.T.);
#21639=ORIENTED_EDGE('',*,*,#15570,.F.);
#21640=ORIENTED_EDGE('',*,*,#15530,.F.);
#21641=ORIENTED_EDGE('',*,*,#15568,.T.);
#21642=ORIENTED_EDGE('',*,*,#15571,.T.);
#21643=ORIENTED_EDGE('',*,*,#15572,.F.);
#21644=ORIENTED_EDGE('',*,*,#15573,.F.);
#21645=ORIENTED_EDGE('',*,*,#15574,.T.);
#21646=ORIENTED_EDGE('',*,*,#15575,.F.);
#21647=ORIENTED_EDGE('',*,*,#15576,.T.);
#21648=ORIENTED_EDGE('',*,*,#15577,.T.);
#21649=ORIENTED_EDGE('',*,*,#15574,.F.);
#21650=ORIENTED_EDGE('',*,*,#15578,.T.);
#21651=ORIENTED_EDGE('',*,*,#15579,.T.);
#21652=ORIENTED_EDGE('',*,*,#15580,.T.);
#21653=ORIENTED_EDGE('',*,*,#15581,.F.);
#21654=ORIENTED_EDGE('',*,*,#15576,.F.);
#21655=ORIENTED_EDGE('',*,*,#15580,.F.);
#21656=ORIENTED_EDGE('',*,*,#15582,.F.);
#21657=ORIENTED_EDGE('',*,*,#15582,.T.);
#21658=ORIENTED_EDGE('',*,*,#15583,.F.);
#21659=ORIENTED_EDGE('',*,*,#15584,.T.);
#21660=ORIENTED_EDGE('',*,*,#15585,.T.);
#21661=ORIENTED_EDGE('',*,*,#15577,.F.);
#21662=ORIENTED_EDGE('',*,*,#15585,.F.);
#21663=ORIENTED_EDGE('',*,*,#15586,.T.);
#21664=ORIENTED_EDGE('',*,*,#15587,.F.);
#21665=ORIENTED_EDGE('',*,*,#15588,.T.);
#21666=ORIENTED_EDGE('',*,*,#15589,.F.);
#21667=ORIENTED_EDGE('',*,*,#15571,.F.);
#21668=ORIENTED_EDGE('',*,*,#15587,.T.);
#21669=ORIENTED_EDGE('',*,*,#15590,.T.);
#21670=ORIENTED_EDGE('',*,*,#15591,.F.);
#21671=ORIENTED_EDGE('',*,*,#15588,.F.);
#21672=ORIENTED_EDGE('',*,*,#15592,.T.);
#21673=ORIENTED_EDGE('',*,*,#15586,.F.);
#21674=ORIENTED_EDGE('',*,*,#15593,.T.);
#21675=ORIENTED_EDGE('',*,*,#15594,.T.);
#21676=ORIENTED_EDGE('',*,*,#15592,.F.);
#21677=ORIENTED_EDGE('',*,*,#15584,.F.);
#21678=ORIENTED_EDGE('',*,*,#15595,.F.);
#21679=ORIENTED_EDGE('',*,*,#15593,.F.);
#21680=ORIENTED_EDGE('',*,*,#15596,.T.);
#21681=ORIENTED_EDGE('',*,*,#15597,.F.);
#21682=ORIENTED_EDGE('',*,*,#15598,.F.);
#21683=ORIENTED_EDGE('',*,*,#15599,.T.);
#21684=ORIENTED_EDGE('',*,*,#15600,.T.);
#21685=ORIENTED_EDGE('',*,*,#15601,.T.);
#21686=ORIENTED_EDGE('',*,*,#15602,.F.);
#21687=ORIENTED_EDGE('',*,*,#15599,.F.);
#21688=ORIENTED_EDGE('',*,*,#15603,.F.);
#21689=ORIENTED_EDGE('',*,*,#15601,.F.);
#21690=ORIENTED_EDGE('',*,*,#15604,.F.);
#21691=ORIENTED_EDGE('',*,*,#15595,.T.);
#21692=ORIENTED_EDGE('',*,*,#15605,.F.);
#21693=ORIENTED_EDGE('',*,*,#15604,.T.);
#21694=ORIENTED_EDGE('',*,*,#15606,.T.);
#21695=ORIENTED_EDGE('',*,*,#15583,.T.);
#21696=ORIENTED_EDGE('',*,*,#15579,.F.);
#21697=ORIENTED_EDGE('',*,*,#15607,.F.);
#21698=ORIENTED_EDGE('',*,*,#15605,.T.);
#21699=ORIENTED_EDGE('',*,*,#15608,.T.);
#21700=ORIENTED_EDGE('',*,*,#15609,.F.);
#21701=ORIENTED_EDGE('',*,*,#15603,.T.);
#21702=ORIENTED_EDGE('',*,*,#15607,.T.);
#21703=ORIENTED_EDGE('',*,*,#15610,.F.);
#21704=ORIENTED_EDGE('',*,*,#15608,.F.);
#21705=ORIENTED_EDGE('',*,*,#15578,.F.);
#21706=ORIENTED_EDGE('',*,*,#15611,.T.);
#21707=ORIENTED_EDGE('',*,*,#15612,.F.);
#21708=ORIENTED_EDGE('',*,*,#15613,.F.);
#21709=ORIENTED_EDGE('',*,*,#15614,.T.);
#21710=ORIENTED_EDGE('',*,*,#15615,.F.);
#21711=ORIENTED_EDGE('',*,*,#15614,.F.);
#21712=ORIENTED_EDGE('',*,*,#15616,.T.);
#21713=ORIENTED_EDGE('',*,*,#15610,.T.);
#21714=ORIENTED_EDGE('',*,*,#15602,.T.);
#21715=ORIENTED_EDGE('',*,*,#15609,.T.);
#21716=ORIENTED_EDGE('',*,*,#15616,.F.);
#21717=ORIENTED_EDGE('',*,*,#15617,.F.);
#21718=ORIENTED_EDGE('',*,*,#15613,.T.);
#21719=ORIENTED_EDGE('',*,*,#15618,.F.);
#21720=ORIENTED_EDGE('',*,*,#15596,.F.);
#21721=ORIENTED_EDGE('',*,*,#15617,.T.);
#21722=ORIENTED_EDGE('',*,*,#15549,.T.);
#21723=ORIENTED_EDGE('',*,*,#15619,.F.);
#21724=ORIENTED_EDGE('',*,*,#15236,.T.);
#21725=ORIENTED_EDGE('',*,*,#15253,.T.);
#21726=ORIENTED_EDGE('',*,*,#15255,.T.);
#21727=ORIENTED_EDGE('',*,*,#15620,.F.);
#21728=ORIENTED_EDGE('',*,*,#15558,.T.);
#21729=ORIENTED_EDGE('',*,*,#15556,.T.);
#21730=ORIENTED_EDGE('',*,*,#15276,.T.);
#21731=ORIENTED_EDGE('',*,*,#15621,.F.);
#21732=ORIENTED_EDGE('',*,*,#15284,.T.);
#21733=ORIENTED_EDGE('',*,*,#15301,.T.);
#21734=ORIENTED_EDGE('',*,*,#15303,.T.);
#21735=ORIENTED_EDGE('',*,*,#15622,.F.);
#21736=ORIENTED_EDGE('',*,*,#15261,.T.);
#21737=ORIENTED_EDGE('',*,*,#15282,.T.);
#21738=ORIENTED_EDGE('',*,*,#15324,.T.);
#21739=ORIENTED_EDGE('',*,*,#15623,.F.);
#21740=ORIENTED_EDGE('',*,*,#15332,.T.);
#21741=ORIENTED_EDGE('',*,*,#15349,.T.);
#21742=ORIENTED_EDGE('',*,*,#15351,.T.);
#21743=ORIENTED_EDGE('',*,*,#15624,.F.);
#21744=ORIENTED_EDGE('',*,*,#15309,.T.);
#21745=ORIENTED_EDGE('',*,*,#15330,.T.);
#21746=ORIENTED_EDGE('',*,*,#15372,.T.);
#21747=ORIENTED_EDGE('',*,*,#15625,.F.);
#21748=ORIENTED_EDGE('',*,*,#15380,.T.);
#21749=ORIENTED_EDGE('',*,*,#15397,.T.);
#21750=ORIENTED_EDGE('',*,*,#15399,.T.);
#21751=ORIENTED_EDGE('',*,*,#15626,.F.);
#21752=ORIENTED_EDGE('',*,*,#15357,.T.);
#21753=ORIENTED_EDGE('',*,*,#15378,.T.);
#21754=ORIENTED_EDGE('',*,*,#15420,.T.);
#21755=ORIENTED_EDGE('',*,*,#15627,.F.);
#21756=ORIENTED_EDGE('',*,*,#15428,.T.);
#21757=ORIENTED_EDGE('',*,*,#15445,.T.);
#21758=ORIENTED_EDGE('',*,*,#15447,.T.);
#21759=ORIENTED_EDGE('',*,*,#15628,.F.);
#21760=ORIENTED_EDGE('',*,*,#15405,.T.);
#21761=ORIENTED_EDGE('',*,*,#15426,.T.);
#21762=ORIENTED_EDGE('',*,*,#15468,.T.);
#21763=ORIENTED_EDGE('',*,*,#15629,.F.);
#21764=ORIENTED_EDGE('',*,*,#15476,.T.);
#21765=ORIENTED_EDGE('',*,*,#15493,.T.);
#21766=ORIENTED_EDGE('',*,*,#15495,.T.);
#21767=ORIENTED_EDGE('',*,*,#15630,.F.);
#21768=ORIENTED_EDGE('',*,*,#15453,.T.);
#21769=ORIENTED_EDGE('',*,*,#15474,.T.);
#21770=ORIENTED_EDGE('',*,*,#15516,.T.);
#21771=ORIENTED_EDGE('',*,*,#15631,.F.);
#21772=ORIENTED_EDGE('',*,*,#15572,.T.);
#21773=ORIENTED_EDGE('',*,*,#15589,.T.);
#21774=ORIENTED_EDGE('',*,*,#15591,.T.);
#21775=ORIENTED_EDGE('',*,*,#15632,.F.);
#21776=ORIENTED_EDGE('',*,*,#15501,.T.);
#21777=ORIENTED_EDGE('',*,*,#15522,.T.);
#21778=ORIENTED_EDGE('',*,*,#15612,.T.);
#21779=ORIENTED_EDGE('',*,*,#15633,.F.);
#21780=ORIENTED_EDGE('',*,*,#15528,.T.);
#21781=ORIENTED_EDGE('',*,*,#15531,.T.);
#21782=ORIENTED_EDGE('',*,*,#15570,.T.);
#21783=ORIENTED_EDGE('',*,*,#15634,.F.);
#21784=ORIENTED_EDGE('',*,*,#15597,.T.);
#21785=ORIENTED_EDGE('',*,*,#15618,.T.);
#21786=ORIENTED_EDGE('',*,*,#15635,.T.);
#21787=ORIENTED_EDGE('',*,*,#15636,.T.);
#21788=ORIENTED_EDGE('',*,*,#15637,.T.);
#21789=ORIENTED_EDGE('',*,*,#15635,.F.);
#21790=ORIENTED_EDGE('',*,*,#15637,.F.);
#21791=ORIENTED_EDGE('',*,*,#15638,.T.);
#21792=ORIENTED_EDGE('',*,*,#15639,.T.);
#21793=ORIENTED_EDGE('',*,*,#15640,.T.);
#21794=ORIENTED_EDGE('',*,*,#15638,.F.);
#21795=ORIENTED_EDGE('',*,*,#15640,.F.);
#21796=ORIENTED_EDGE('',*,*,#15641,.T.);
#21797=ORIENTED_EDGE('',*,*,#15642,.T.);
#21798=ORIENTED_EDGE('',*,*,#15643,.T.);
#21799=ORIENTED_EDGE('',*,*,#15641,.F.);
#21800=ORIENTED_EDGE('',*,*,#15643,.F.);
#21801=ORIENTED_EDGE('',*,*,#15254,.F.);
#21802=ORIENTED_EDGE('',*,*,#15258,.F.);
#21803=ORIENTED_EDGE('',*,*,#15270,.F.);
#21804=ORIENTED_EDGE('',*,*,#15264,.F.);
#21805=ORIENTED_EDGE('',*,*,#15262,.T.);
#21806=ORIENTED_EDGE('',*,*,#15622,.T.);
#21807=ORIENTED_EDGE('',*,*,#15302,.F.);
#21808=ORIENTED_EDGE('',*,*,#15306,.F.);
#21809=ORIENTED_EDGE('',*,*,#15318,.F.);
#21810=ORIENTED_EDGE('',*,*,#15312,.F.);
#21811=ORIENTED_EDGE('',*,*,#15310,.T.);
#21812=ORIENTED_EDGE('',*,*,#15624,.T.);
#21813=ORIENTED_EDGE('',*,*,#15350,.F.);
#21814=ORIENTED_EDGE('',*,*,#15354,.F.);
#21815=ORIENTED_EDGE('',*,*,#15366,.F.);
#21816=ORIENTED_EDGE('',*,*,#15360,.F.);
#21817=ORIENTED_EDGE('',*,*,#15358,.T.);
#21818=ORIENTED_EDGE('',*,*,#15626,.T.);
#21819=ORIENTED_EDGE('',*,*,#15398,.F.);
#21820=ORIENTED_EDGE('',*,*,#15402,.F.);
#21821=ORIENTED_EDGE('',*,*,#15414,.F.);
#21822=ORIENTED_EDGE('',*,*,#15408,.F.);
#21823=ORIENTED_EDGE('',*,*,#15406,.T.);
#21824=ORIENTED_EDGE('',*,*,#15628,.T.);
#21825=ORIENTED_EDGE('',*,*,#15446,.F.);
#21826=ORIENTED_EDGE('',*,*,#15450,.F.);
#21827=ORIENTED_EDGE('',*,*,#15462,.F.);
#21828=ORIENTED_EDGE('',*,*,#15456,.F.);
#21829=ORIENTED_EDGE('',*,*,#15454,.T.);
#21830=ORIENTED_EDGE('',*,*,#15630,.T.);
#21831=ORIENTED_EDGE('',*,*,#15494,.F.);
#21832=ORIENTED_EDGE('',*,*,#15498,.F.);
#21833=ORIENTED_EDGE('',*,*,#15510,.F.);
#21834=ORIENTED_EDGE('',*,*,#15504,.F.);
#21835=ORIENTED_EDGE('',*,*,#15502,.T.);
#21836=ORIENTED_EDGE('',*,*,#15632,.T.);
#21837=ORIENTED_EDGE('',*,*,#15590,.F.);
#21838=ORIENTED_EDGE('',*,*,#15594,.F.);
#21839=ORIENTED_EDGE('',*,*,#15606,.F.);
#21840=ORIENTED_EDGE('',*,*,#15600,.F.);
#21841=ORIENTED_EDGE('',*,*,#15598,.T.);
#21842=ORIENTED_EDGE('',*,*,#15634,.T.);
#21843=ORIENTED_EDGE('',*,*,#15569,.F.);
#21844=ORIENTED_EDGE('',*,*,#15567,.F.);
#21845=ORIENTED_EDGE('',*,*,#15565,.F.);
#21846=ORIENTED_EDGE('',*,*,#15561,.F.);
#21847=ORIENTED_EDGE('',*,*,#15559,.T.);
#21848=ORIENTED_EDGE('',*,*,#15620,.T.);
#21849=ORIENTED_EDGE('',*,*,#15233,.F.);
#21850=ORIENTED_EDGE('',*,*,#15642,.F.);
#21851=ORIENTED_EDGE('',*,*,#15644,.F.);
#21852=ORIENTED_EDGE('',*,*,#15636,.F.);
#21853=ORIENTED_EDGE('',*,*,#15639,.F.);
#21854=ORIENTED_EDGE('',*,*,#15645,.T.);
#21855=ORIENTED_EDGE('',*,*,#15646,.T.);
#21856=ORIENTED_EDGE('',*,*,#15644,.T.);
#21857=ORIENTED_EDGE('',*,*,#15646,.F.);
#21858=ORIENTED_EDGE('',*,*,#15647,.F.);
#21859=ORIENTED_EDGE('',*,*,#15647,.T.);
#21860=ORIENTED_EDGE('',*,*,#15648,.T.);
#21861=ORIENTED_EDGE('',*,*,#15649,.F.);
#21862=ORIENTED_EDGE('',*,*,#15648,.F.);
#21863=ORIENTED_EDGE('',*,*,#15650,.F.);
#21864=ORIENTED_EDGE('',*,*,#15650,.T.);
#21865=ORIENTED_EDGE('',*,*,#15651,.T.);
#21866=ORIENTED_EDGE('',*,*,#15652,.F.);
#21867=ORIENTED_EDGE('',*,*,#15651,.F.);
#21868=ORIENTED_EDGE('',*,*,#15653,.F.);
#21869=ORIENTED_EDGE('',*,*,#15653,.T.);
#21870=ORIENTED_EDGE('',*,*,#15654,.T.);
#21871=ORIENTED_EDGE('',*,*,#15655,.F.);
#21872=ORIENTED_EDGE('',*,*,#15654,.F.);
#21873=ORIENTED_EDGE('',*,*,#15541,.T.);
#21874=ORIENTED_EDGE('',*,*,#15523,.T.);
#21875=ORIENTED_EDGE('',*,*,#15529,.T.);
#21876=ORIENTED_EDGE('',*,*,#15633,.T.);
#21877=ORIENTED_EDGE('',*,*,#15611,.F.);
#21878=ORIENTED_EDGE('',*,*,#15615,.T.);
#21879=ORIENTED_EDGE('',*,*,#15581,.T.);
#21880=ORIENTED_EDGE('',*,*,#15575,.T.);
#21881=ORIENTED_EDGE('',*,*,#15573,.T.);
#21882=ORIENTED_EDGE('',*,*,#15631,.T.);
#21883=ORIENTED_EDGE('',*,*,#15515,.F.);
#21884=ORIENTED_EDGE('',*,*,#15519,.T.);
#21885=ORIENTED_EDGE('',*,*,#15485,.T.);
#21886=ORIENTED_EDGE('',*,*,#15479,.T.);
#21887=ORIENTED_EDGE('',*,*,#15477,.T.);
#21888=ORIENTED_EDGE('',*,*,#15629,.T.);
#21889=ORIENTED_EDGE('',*,*,#15467,.F.);
#21890=ORIENTED_EDGE('',*,*,#15471,.T.);
#21891=ORIENTED_EDGE('',*,*,#15437,.T.);
#21892=ORIENTED_EDGE('',*,*,#15431,.T.);
#21893=ORIENTED_EDGE('',*,*,#15429,.T.);
#21894=ORIENTED_EDGE('',*,*,#15627,.T.);
#21895=ORIENTED_EDGE('',*,*,#15419,.F.);
#21896=ORIENTED_EDGE('',*,*,#15423,.T.);
#21897=ORIENTED_EDGE('',*,*,#15389,.T.);
#21898=ORIENTED_EDGE('',*,*,#15383,.T.);
#21899=ORIENTED_EDGE('',*,*,#15381,.T.);
#21900=ORIENTED_EDGE('',*,*,#15625,.T.);
#21901=ORIENTED_EDGE('',*,*,#15371,.F.);
#21902=ORIENTED_EDGE('',*,*,#15375,.T.);
#21903=ORIENTED_EDGE('',*,*,#15341,.T.);
#21904=ORIENTED_EDGE('',*,*,#15335,.T.);
#21905=ORIENTED_EDGE('',*,*,#15333,.T.);
#21906=ORIENTED_EDGE('',*,*,#15623,.T.);
#21907=ORIENTED_EDGE('',*,*,#15323,.F.);
#21908=ORIENTED_EDGE('',*,*,#15327,.T.);
#21909=ORIENTED_EDGE('',*,*,#15293,.T.);
#21910=ORIENTED_EDGE('',*,*,#15287,.T.);
#21911=ORIENTED_EDGE('',*,*,#15285,.T.);
#21912=ORIENTED_EDGE('',*,*,#15621,.T.);
#21913=ORIENTED_EDGE('',*,*,#15275,.F.);
#21914=ORIENTED_EDGE('',*,*,#15279,.T.);
#21915=ORIENTED_EDGE('',*,*,#15245,.T.);
#21916=ORIENTED_EDGE('',*,*,#15239,.T.);
#21917=ORIENTED_EDGE('',*,*,#15237,.T.);
#21918=ORIENTED_EDGE('',*,*,#15619,.T.);
#21919=ORIENTED_EDGE('',*,*,#15548,.F.);
#21920=ORIENTED_EDGE('',*,*,#15552,.T.);
#21921=ORIENTED_EDGE('',*,*,#15231,.T.);
#21922=ORIENTED_EDGE('',*,*,#15655,.T.);
#21923=ORIENTED_EDGE('',*,*,#15645,.F.);
#21924=ORIENTED_EDGE('',*,*,#15649,.T.);
#21925=ORIENTED_EDGE('',*,*,#15652,.T.);
#24095=CYLINDRICAL_SURFACE('',#27717,2.);
#24096=CYLINDRICAL_SURFACE('',#27721,2.);
#24097=CYLINDRICAL_SURFACE('',#27917,2.);
#24098=CYLINDRICAL_SURFACE('',#27921,2.);
#24099=CYLINDRICAL_SURFACE('',#27925,2.);
#24100=CYLINDRICAL_SURFACE('',#27929,13.5);
#24101=CYLINDRICAL_SURFACE('',#27933,2.);
#24102=CYLINDRICAL_SURFACE('',#27937,2.);
#24103=CYLINDRICAL_SURFACE('',#27941,2.);
#25073=ADVANCED_FACE('',(#3120),#2016,.F.);
#25074=ADVANCED_FACE('',(#3121),#24095,.T.);
#25075=ADVANCED_FACE('',(#3122),#2017,.T.);
#25076=ADVANCED_FACE('',(#3123),#24096,.T.);
#25077=ADVANCED_FACE('',(#3124),#404,.F.);
#25078=ADVANCED_FACE('',(#3125),#405,.T.);
#25079=ADVANCED_FACE('',(#3126),#406,.T.);
#25080=ADVANCED_FACE('',(#3127),#37,.T.);
#25081=ADVANCED_FACE('',(#3128),#407,.T.);
#25082=ADVANCED_FACE('',(#3129),#11,.T.);
#25083=ADVANCED_FACE('',(#3130),#408,.F.);
#25084=ADVANCED_FACE('',(#3131),#409,.F.);
#25085=ADVANCED_FACE('',(#3132),#410,.T.);
#25086=ADVANCED_FACE('',(#3133),#38,.T.);
#25087=ADVANCED_FACE('',(#3134),#411,.F.);
#25088=ADVANCED_FACE('',(#3135),#412,.T.);
#25089=ADVANCED_FACE('',(#3136),#39,.T.);
#25090=ADVANCED_FACE('',(#3137),#413,.T.);
#25091=ADVANCED_FACE('',(#3138),#12,.T.);
#25092=ADVANCED_FACE('',(#3139),#414,.T.);
#25093=ADVANCED_FACE('',(#3140),#40,.T.);
#25094=ADVANCED_FACE('',(#3141),#415,.F.);
#25095=ADVANCED_FACE('',(#3142),#416,.T.);
#25096=ADVANCED_FACE('',(#3143),#13,.T.);
#25097=ADVANCED_FACE('',(#3144),#417,.F.);
#25098=ADVANCED_FACE('',(#3145),#418,.F.);
#25099=ADVANCED_FACE('',(#3146),#419,.T.);
#25100=ADVANCED_FACE('',(#3147),#420,.T.);
#25101=ADVANCED_FACE('',(#3148),#41,.T.);
#25102=ADVANCED_FACE('',(#3149),#421,.T.);
#25103=ADVANCED_FACE('',(#3150),#14,.T.);
#25104=ADVANCED_FACE('',(#3151),#422,.F.);
#25105=ADVANCED_FACE('',(#3152),#423,.F.);
#25106=ADVANCED_FACE('',(#3153),#424,.T.);
#25107=ADVANCED_FACE('',(#3154),#42,.T.);
#25108=ADVANCED_FACE('',(#3155),#425,.F.);
#25109=ADVANCED_FACE('',(#3156),#426,.T.);
#25110=ADVANCED_FACE('',(#3157),#43,.T.);
#25111=ADVANCED_FACE('',(#3158),#427,.T.);
#25112=ADVANCED_FACE('',(#3159),#15,.T.);
#25113=ADVANCED_FACE('',(#3160),#428,.T.);
#25114=ADVANCED_FACE('',(#3161),#44,.T.);
#25115=ADVANCED_FACE('',(#3162),#429,.F.);
#25116=ADVANCED_FACE('',(#3163),#430,.T.);
#25117=ADVANCED_FACE('',(#3164),#16,.T.);
#25118=ADVANCED_FACE('',(#3165),#431,.F.);
#25119=ADVANCED_FACE('',(#3166),#432,.F.);
#25120=ADVANCED_FACE('',(#3167),#433,.T.);
#25121=ADVANCED_FACE('',(#3168),#434,.T.);
#25122=ADVANCED_FACE('',(#3169),#45,.T.);
#25123=ADVANCED_FACE('',(#3170),#435,.T.);
#25124=ADVANCED_FACE('',(#3171),#17,.T.);
#25125=ADVANCED_FACE('',(#3172),#436,.F.);
#25126=ADVANCED_FACE('',(#3173),#437,.F.);
#25127=ADVANCED_FACE('',(#3174),#438,.T.);
#25128=ADVANCED_FACE('',(#3175),#46,.T.);
#25129=ADVANCED_FACE('',(#3176),#439,.F.);
#25130=ADVANCED_FACE('',(#3177),#440,.T.);
#25131=ADVANCED_FACE('',(#3178),#47,.T.);
#25132=ADVANCED_FACE('',(#3179),#441,.T.);
#25133=ADVANCED_FACE('',(#3180),#18,.T.);
#25134=ADVANCED_FACE('',(#3181),#442,.T.);
#25135=ADVANCED_FACE('',(#3182),#48,.T.);
#25136=ADVANCED_FACE('',(#3183),#443,.F.);
#25137=ADVANCED_FACE('',(#3184),#444,.T.);
#25138=ADVANCED_FACE('',(#3185),#19,.T.);
#25139=ADVANCED_FACE('',(#3186),#445,.F.);
#25140=ADVANCED_FACE('',(#3187),#446,.F.);
#25141=ADVANCED_FACE('',(#3188),#447,.T.);
#25142=ADVANCED_FACE('',(#3189),#448,.T.);
#25143=ADVANCED_FACE('',(#3190),#49,.T.);
#25144=ADVANCED_FACE('',(#3191),#449,.T.);
#25145=ADVANCED_FACE('',(#3192),#20,.T.);
#25146=ADVANCED_FACE('',(#3193),#450,.F.);
#25147=ADVANCED_FACE('',(#3194),#451,.F.);
#25148=ADVANCED_FACE('',(#3195),#452,.T.);
#25149=ADVANCED_FACE('',(#3196),#50,.T.);
#25150=ADVANCED_FACE('',(#3197),#453,.F.);
#25151=ADVANCED_FACE('',(#3198),#454,.T.);
#25152=ADVANCED_FACE('',(#3199),#51,.T.);
#25153=ADVANCED_FACE('',(#3200),#455,.T.);
#25154=ADVANCED_FACE('',(#3201),#21,.T.);
#25155=ADVANCED_FACE('',(#3202),#456,.T.);
#25156=ADVANCED_FACE('',(#3203),#52,.T.);
#25157=ADVANCED_FACE('',(#3204),#457,.F.);
#25158=ADVANCED_FACE('',(#3205),#458,.T.);
#25159=ADVANCED_FACE('',(#3206),#22,.T.);
#25160=ADVANCED_FACE('',(#3207),#459,.F.);
#25161=ADVANCED_FACE('',(#3208),#460,.F.);
#25162=ADVANCED_FACE('',(#3209),#461,.T.);
#25163=ADVANCED_FACE('',(#3210),#462,.T.);
#25164=ADVANCED_FACE('',(#3211),#53,.T.);
#25165=ADVANCED_FACE('',(#3212),#463,.T.);
#25166=ADVANCED_FACE('',(#3213),#23,.T.);
#25167=ADVANCED_FACE('',(#3214),#464,.F.);
#25168=ADVANCED_FACE('',(#3215),#465,.F.);
#25169=ADVANCED_FACE('',(#3216),#466,.T.);
#25170=ADVANCED_FACE('',(#3217),#54,.T.);
#25171=ADVANCED_FACE('',(#3218),#467,.F.);
#25172=ADVANCED_FACE('',(#3219),#468,.T.);
#25173=ADVANCED_FACE('',(#3220),#55,.T.);
#25174=ADVANCED_FACE('',(#3221),#469,.T.);
#25175=ADVANCED_FACE('',(#3222),#24,.T.);
#25176=ADVANCED_FACE('',(#3223),#470,.T.);
#25177=ADVANCED_FACE('',(#3224),#56,.T.);
#25178=ADVANCED_FACE('',(#3225),#471,.F.);
#25179=ADVANCED_FACE('',(#3226),#472,.T.);
#25180=ADVANCED_FACE('',(#3227),#25,.T.);
#25181=ADVANCED_FACE('',(#3228),#473,.F.);
#25182=ADVANCED_FACE('',(#3229),#474,.F.);
#25183=ADVANCED_FACE('',(#3230),#475,.T.);
#25184=ADVANCED_FACE('',(#3231),#476,.T.);
#25185=ADVANCED_FACE('',(#3232),#57,.T.);
#25186=ADVANCED_FACE('',(#3233),#477,.T.);
#25187=ADVANCED_FACE('',(#3234),#26,.T.);
#25188=ADVANCED_FACE('',(#3235),#478,.F.);
#25189=ADVANCED_FACE('',(#3236),#479,.F.);
#25190=ADVANCED_FACE('',(#3237),#480,.T.);
#25191=ADVANCED_FACE('',(#3238),#58,.T.);
#25192=ADVANCED_FACE('',(#3239),#481,.F.);
#25193=ADVANCED_FACE('',(#3240),#482,.T.);
#25194=ADVANCED_FACE('',(#3241),#59,.T.);
#25195=ADVANCED_FACE('',(#3242),#483,.T.);
#25196=ADVANCED_FACE('',(#3243),#27,.T.);
#25197=ADVANCED_FACE('',(#3244),#484,.T.);
#25198=ADVANCED_FACE('',(#3245),#60,.T.);
#25199=ADVANCED_FACE('',(#3246),#485,.F.);
#25200=ADVANCED_FACE('',(#3247),#486,.T.);
#25201=ADVANCED_FACE('',(#3248),#28,.T.);
#25202=ADVANCED_FACE('',(#3249),#487,.F.);
#25203=ADVANCED_FACE('',(#3250),#488,.T.);
#25204=ADVANCED_FACE('',(#3251),#489,.F.);
#25205=ADVANCED_FACE('',(#3252),#490,.F.);
#25206=ADVANCED_FACE('',(#3253),#29,.T.);
#25207=ADVANCED_FACE('',(#3254),#491,.T.);
#25208=ADVANCED_FACE('',(#3255),#61,.T.);
#25209=ADVANCED_FACE('',(#3256),#492,.T.);
#25210=ADVANCED_FACE('',(#3257),#30,.T.);
#25211=ADVANCED_FACE('',(#3258),#493,.T.);
#25212=ADVANCED_FACE('',(#3259),#62,.T.);
#25213=ADVANCED_FACE('',(#3260),#494,.F.);
#25214=ADVANCED_FACE('',(#3261),#495,.T.);
#25215=ADVANCED_FACE('',(#3262),#31,.T.);
#25216=ADVANCED_FACE('',(#3263),#496,.F.);
#25217=ADVANCED_FACE('',(#3264),#497,.F.);
#25218=ADVANCED_FACE('',(#3265),#498,.T.);
#25219=ADVANCED_FACE('',(#3266),#63,.T.);
#25220=ADVANCED_FACE('',(#3267),#499,.T.);
#25221=ADVANCED_FACE('',(#3268),#64,.T.);
#25222=ADVANCED_FACE('',(#3269),#500,.T.);
#25223=ADVANCED_FACE('',(#3270),#501,.F.);
#25224=ADVANCED_FACE('',(#3271),#502,.F.);
#25225=ADVANCED_FACE('',(#3272),#503,.T.);
#25226=ADVANCED_FACE('',(#3273),#504,.T.);
#25227=ADVANCED_FACE('',(#3274),#65,.T.);
#25228=ADVANCED_FACE('',(#3275),#505,.T.);
#25229=ADVANCED_FACE('',(#3276),#32,.T.);
#25230=ADVANCED_FACE('',(#3277),#506,.F.);
#25231=ADVANCED_FACE('',(#3278),#507,.F.);
#25232=ADVANCED_FACE('',(#3279),#508,.T.);
#25233=ADVANCED_FACE('',(#3280),#66,.T.);
#25234=ADVANCED_FACE('',(#3281),#509,.F.);
#25235=ADVANCED_FACE('',(#3282),#510,.T.);
#25236=ADVANCED_FACE('',(#3283),#67,.T.);
#25237=ADVANCED_FACE('',(#3284),#511,.T.);
#25238=ADVANCED_FACE('',(#3285),#33,.T.);
#25239=ADVANCED_FACE('',(#3286),#512,.T.);
#25240=ADVANCED_FACE('',(#3287),#68,.T.);
#25241=ADVANCED_FACE('',(#3288),#513,.F.);
#25242=ADVANCED_FACE('',(#3289),#514,.T.);
#25243=ADVANCED_FACE('',(#3290),#34,.T.);
#25244=ADVANCED_FACE('',(#3291),#515,.F.);
#25245=ADVANCED_FACE('',(#3292),#516,.F.);
#25246=ADVANCED_FACE('',(#3293),#517,.F.);
#25247=ADVANCED_FACE('',(#3294),#518,.F.);
#25248=ADVANCED_FACE('',(#3295),#519,.F.);
#25249=ADVANCED_FACE('',(#3296),#520,.F.);
#25250=ADVANCED_FACE('',(#3297),#521,.F.);
#25251=ADVANCED_FACE('',(#3298),#522,.F.);
#25252=ADVANCED_FACE('',(#3299),#523,.F.);
#25253=ADVANCED_FACE('',(#3300),#2018,.T.);
#25254=ADVANCED_FACE('',(#3301),#24097,.T.);
#25255=ADVANCED_FACE('',(#3302),#2019,.T.);
#25256=ADVANCED_FACE('',(#3303),#24098,.T.);
#25257=ADVANCED_FACE('',(#3304),#2020,.T.);
#25258=ADVANCED_FACE('',(#3305),#24099,.T.);
#25259=ADVANCED_FACE('',(#3306,#1393,#1394,#1395,#1396,#1397),#2021,.F.);
#25260=ADVANCED_FACE('',(#3307),#24100,.F.);
#25261=ADVANCED_FACE('',(#3308),#2022,.F.);
#25262=ADVANCED_FACE('',(#3309),#24101,.T.);
#25263=ADVANCED_FACE('',(#3310),#2023,.F.);
#25264=ADVANCED_FACE('',(#3311),#24102,.T.);
#25265=ADVANCED_FACE('',(#3312),#2024,.F.);
#25266=ADVANCED_FACE('',(#3313),#24103,.T.);
#25267=ADVANCED_FACE('',(#3314,#1398,#1399,#1400,#1401,#1402),#2025,.T.);
#25681=CLOSED_SHELL('',(#25073,#25074,#25075,#25076,#25077,#25078,#25079,
#25080,#25081,#25082,#25083,#25084,#25085,#25086,#25087,#25088,#25089,#25090,
#25091,#25092,#25093,#25094,#25095,#25096,#25097,#25098,#25099,#25100,#25101,
#25102,#25103,#25104,#25105,#25106,#25107,#25108,#25109,#25110,#25111,#25112,
#25113,#25114,#25115,#25116,#25117,#25118,#25119,#25120,#25121,#25122,#25123,
#25124,#25125,#25126,#25127,#25128,#25129,#25130,#25131,#25132,#25133,#25134,
#25135,#25136,#25137,#25138,#25139,#25140,#25141,#25142,#25143,#25144,#25145,
#25146,#25147,#25148,#25149,#25150,#25151,#25152,#25153,#25154,#25155,#25156,
#25157,#25158,#25159,#25160,#25161,#25162,#25163,#25164,#25165,#25166,#25167,
#25168,#25169,#25170,#25171,#25172,#25173,#25174,#25175,#25176,#25177,#25178,
#25179,#25180,#25181,#25182,#25183,#25184,#25185,#25186,#25187,#25188,#25189,
#25190,#25191,#25192,#25193,#25194,#25195,#25196,#25197,#25198,#25199,#25200,
#25201,#25202,#25203,#25204,#25205,#25206,#25207,#25208,#25209,#25210,#25211,
#25212,#25213,#25214,#25215,#25216,#25217,#25218,#25219,#25220,#25221,#25222,
#25223,#25224,#25225,#25226,#25227,#25228,#25229,#25230,#25231,#25232,#25233,
#25234,#25235,#25236,#25237,#25238,#25239,#25240,#25241,#25242,#25243,#25244,
#25245,#25246,#25247,#25248,#25249,#25250,#25251,#25252,#25253,#25254,#25255,
#25256,#25257,#25258,#25259,#25260,#25261,#25262,#25263,#25264,#25265,#25266,
#25267));
#27714=AXIS2_PLACEMENT_3D('',#41230,#33511,#33512);
#27715=AXIS2_PLACEMENT_3D('',#41231,#33513,#33514);
#27716=AXIS2_PLACEMENT_3D('',#41233,#33515,#33516);
#27717=AXIS2_PLACEMENT_3D('',#41234,#33517,#33518);
#27718=AXIS2_PLACEMENT_3D('',#41237,#33520,#33521);
#27719=AXIS2_PLACEMENT_3D('',#41238,#33522,#33523);
#27720=AXIS2_PLACEMENT_3D('',#41240,#33524,#33525);
#27721=AXIS2_PLACEMENT_3D('',#41241,#33526,#33527);
#27722=AXIS2_PLACEMENT_3D('',#41243,#33528,#33529);
#27723=AXIS2_PLACEMENT_3D('',#41287,#33531,#33532);
#27724=AXIS2_PLACEMENT_3D('',#41500,#33533,#33534);
#27725=AXIS2_PLACEMENT_3D('',#41600,#33535,#33536);
#27726=AXIS2_PLACEMENT_3D('',#41602,#33537,#33538);
#27727=AXIS2_PLACEMENT_3D('',#41603,#33539,#33540);
#27728=AXIS2_PLACEMENT_3D('',#41604,#33541,#33542);
#27729=AXIS2_PLACEMENT_3D('',#41605,#33543,#33544);
#27730=AXIS2_PLACEMENT_3D('',#41606,#33545,#33546);
#27731=AXIS2_PLACEMENT_3D('',#41839,#33547,#33548);
#27732=AXIS2_PLACEMENT_3D('',#42537,#33549,#33550);
#27733=AXIS2_PLACEMENT_3D('',#42629,#33551,#33552);
#27734=AXIS2_PLACEMENT_3D('',#42630,#33553,#33554);
#27735=AXIS2_PLACEMENT_3D('',#42947,#33555,#33556);
#27736=AXIS2_PLACEMENT_3D('',#43006,#33557,#33558);
#27737=AXIS2_PLACEMENT_3D('',#43008,#33559,#33560);
#27738=AXIS2_PLACEMENT_3D('',#43009,#33561,#33562);
#27739=AXIS2_PLACEMENT_3D('',#43034,#33563,#33564);
#27740=AXIS2_PLACEMENT_3D('',#43035,#33565,#33566);
#27741=AXIS2_PLACEMENT_3D('',#43351,#33567,#33568);
#27742=AXIS2_PLACEMENT_3D('',#43509,#33569,#33570);
#27743=AXIS2_PLACEMENT_3D('',#43510,#33571,#33572);
#27744=AXIS2_PLACEMENT_3D('',#43608,#33573,#33574);
#27745=AXIS2_PLACEMENT_3D('',#44397,#33575,#33576);
#27746=AXIS2_PLACEMENT_3D('',#44497,#33577,#33578);
#27747=AXIS2_PLACEMENT_3D('',#44499,#33579,#33580);
#27748=AXIS2_PLACEMENT_3D('',#44500,#33581,#33582);
#27749=AXIS2_PLACEMENT_3D('',#44501,#33583,#33584);
#27750=AXIS2_PLACEMENT_3D('',#44502,#33585,#33586);
#27751=AXIS2_PLACEMENT_3D('',#44503,#33587,#33588);
#27752=AXIS2_PLACEMENT_3D('',#44736,#33589,#33590);
#27753=AXIS2_PLACEMENT_3D('',#45071,#33591,#33592);
#27754=AXIS2_PLACEMENT_3D('',#45347,#33593,#33594);
#27755=AXIS2_PLACEMENT_3D('',#45439,#33595,#33596);
#27756=AXIS2_PLACEMENT_3D('',#45440,#33597,#33598);
#27757=AXIS2_PLACEMENT_3D('',#45763,#33599,#33600);
#27758=AXIS2_PLACEMENT_3D('',#45822,#33601,#33602);
#27759=AXIS2_PLACEMENT_3D('',#45824,#33603,#33604);
#27760=AXIS2_PLACEMENT_3D('',#45825,#33605,#33606);
#27761=AXIS2_PLACEMENT_3D('',#45850,#33607,#33608);
#27762=AXIS2_PLACEMENT_3D('',#45851,#33609,#33610);
#27763=AXIS2_PLACEMENT_3D('',#46167,#33611,#33612);
#27764=AXIS2_PLACEMENT_3D('',#46325,#33613,#33614);
#27765=AXIS2_PLACEMENT_3D('',#46326,#33615,#33616);
#27766=AXIS2_PLACEMENT_3D('',#46423,#33617,#33618);
#27767=AXIS2_PLACEMENT_3D('',#47181,#33619,#33620);
#27768=AXIS2_PLACEMENT_3D('',#47281,#33621,#33622);
#27769=AXIS2_PLACEMENT_3D('',#47283,#33623,#33624);
#27770=AXIS2_PLACEMENT_3D('',#47284,#33625,#33626);
#27771=AXIS2_PLACEMENT_3D('',#47285,#33627,#33628);
#27772=AXIS2_PLACEMENT_3D('',#47286,#33629,#33630);
#27773=AXIS2_PLACEMENT_3D('',#47287,#33631,#33632);
#27774=AXIS2_PLACEMENT_3D('',#47520,#33633,#33634);
#27775=AXIS2_PLACEMENT_3D('',#48198,#33635,#33636);
#27776=AXIS2_PLACEMENT_3D('',#48290,#33637,#33638);
#27777=AXIS2_PLACEMENT_3D('',#48291,#33639,#33640);
#27778=AXIS2_PLACEMENT_3D('',#48616,#33641,#33642);
#27779=AXIS2_PLACEMENT_3D('',#48675,#33643,#33644);
#27780=AXIS2_PLACEMENT_3D('',#48677,#33645,#33646);
#27781=AXIS2_PLACEMENT_3D('',#48678,#33647,#33648);
#27782=AXIS2_PLACEMENT_3D('',#48703,#33649,#33650);
#27783=AXIS2_PLACEMENT_3D('',#48704,#33651,#33652);
#27784=AXIS2_PLACEMENT_3D('',#49053,#33653,#33654);
#27785=AXIS2_PLACEMENT_3D('',#49211,#33655,#33656);
#27786=AXIS2_PLACEMENT_3D('',#49212,#33657,#33658);
#27787=AXIS2_PLACEMENT_3D('',#49309,#33659,#33660);
#27788=AXIS2_PLACEMENT_3D('',#49808,#33661,#33662);
#27789=AXIS2_PLACEMENT_3D('',#50021,#33663,#33664);
#27790=AXIS2_PLACEMENT_3D('',#50121,#33665,#33666);
#27791=AXIS2_PLACEMENT_3D('',#50123,#33667,#33668);
#27792=AXIS2_PLACEMENT_3D('',#50124,#33669,#33670);
#27793=AXIS2_PLACEMENT_3D('',#50125,#33671,#33672);
#27794=AXIS2_PLACEMENT_3D('',#50126,#33673,#33674);
#27795=AXIS2_PLACEMENT_3D('',#50127,#33675,#33676);
#27796=AXIS2_PLACEMENT_3D('',#50360,#33677,#33678);
#27797=AXIS2_PLACEMENT_3D('',#51055,#33679,#33680);
#27798=AXIS2_PLACEMENT_3D('',#51147,#33681,#33682);
#27799=AXIS2_PLACEMENT_3D('',#51148,#33683,#33684);
#27800=AXIS2_PLACEMENT_3D('',#51195,#33685,#33686);
#27801=AXIS2_PLACEMENT_3D('',#51419,#33687,#33688);
#27802=AXIS2_PLACEMENT_3D('',#51478,#33689,#33690);
#27803=AXIS2_PLACEMENT_3D('',#51480,#33691,#33692);
#27804=AXIS2_PLACEMENT_3D('',#51481,#33693,#33694);
#27805=AXIS2_PLACEMENT_3D('',#51506,#33695,#33696);
#27806=AXIS2_PLACEMENT_3D('',#51507,#33697,#33698);
#27807=AXIS2_PLACEMENT_3D('',#51853,#33699,#33700);
#27808=AXIS2_PLACEMENT_3D('',#52011,#33701,#33702);
#27809=AXIS2_PLACEMENT_3D('',#52012,#33703,#33704);
#27810=AXIS2_PLACEMENT_3D('',#52113,#33705,#33706);
#27811=AXIS2_PLACEMENT_3D('',#52887,#33707,#33708);
#27812=AXIS2_PLACEMENT_3D('',#52987,#33709,#33710);
#27813=AXIS2_PLACEMENT_3D('',#52989,#33711,#33712);
#27814=AXIS2_PLACEMENT_3D('',#52990,#33713,#33714);
#27815=AXIS2_PLACEMENT_3D('',#52991,#33715,#33716);
#27816=AXIS2_PLACEMENT_3D('',#52992,#33717,#33718);
#27817=AXIS2_PLACEMENT_3D('',#52993,#33719,#33720);
#27818=AXIS2_PLACEMENT_3D('',#53226,#33721,#33722);
#27819=AXIS2_PLACEMENT_3D('',#53561,#33723,#33724);
#27820=AXIS2_PLACEMENT_3D('',#53837,#33725,#33726);
#27821=AXIS2_PLACEMENT_3D('',#53929,#33727,#33728);
#27822=AXIS2_PLACEMENT_3D('',#53930,#33729,#33730);
#27823=AXIS2_PLACEMENT_3D('',#54280,#33731,#33732);
#27824=AXIS2_PLACEMENT_3D('',#54339,#33733,#33734);
#27825=AXIS2_PLACEMENT_3D('',#54341,#33735,#33736);
#27826=AXIS2_PLACEMENT_3D('',#54342,#33737,#33738);
#27827=AXIS2_PLACEMENT_3D('',#54367,#33739,#33740);
#27828=AXIS2_PLACEMENT_3D('',#54368,#33741,#33742);
#27829=AXIS2_PLACEMENT_3D('',#54714,#33743,#33744);
#27830=AXIS2_PLACEMENT_3D('',#54872,#33745,#33746);
#27831=AXIS2_PLACEMENT_3D('',#54873,#33747,#33748);
#27832=AXIS2_PLACEMENT_3D('',#55808,#33749,#33750);
#27833=AXIS2_PLACEMENT_3D('',#55908,#33751,#33752);
#27834=AXIS2_PLACEMENT_3D('',#55910,#33753,#33754);
#27835=AXIS2_PLACEMENT_3D('',#55911,#33755,#33756);
#27836=AXIS2_PLACEMENT_3D('',#55912,#33757,#33758);
#27837=AXIS2_PLACEMENT_3D('',#55913,#33759,#33760);
#27838=AXIS2_PLACEMENT_3D('',#55914,#33761,#33762);
#27839=AXIS2_PLACEMENT_3D('',#56147,#33763,#33764);
#27840=AXIS2_PLACEMENT_3D('',#56822,#33765,#33766);
#27841=AXIS2_PLACEMENT_3D('',#56914,#33767,#33768);
#27842=AXIS2_PLACEMENT_3D('',#56915,#33769,#33770);
#27843=AXIS2_PLACEMENT_3D('',#56954,#33771,#33772);
#27844=AXIS2_PLACEMENT_3D('',#57175,#33773,#33774);
#27845=AXIS2_PLACEMENT_3D('',#57234,#33775,#33776);
#27846=AXIS2_PLACEMENT_3D('',#57236,#33777,#33778);
#27847=AXIS2_PLACEMENT_3D('',#57237,#33779,#33780);
#27848=AXIS2_PLACEMENT_3D('',#57262,#33781,#33782);
#27849=AXIS2_PLACEMENT_3D('',#57263,#33783,#33784);
#27850=AXIS2_PLACEMENT_3D('',#57606,#33785,#33786);
#27851=AXIS2_PLACEMENT_3D('',#57764,#33787,#33788);
#27852=AXIS2_PLACEMENT_3D('',#57765,#33789,#33790);
#27853=AXIS2_PLACEMENT_3D('',#57863,#33791,#33792);
#27854=AXIS2_PLACEMENT_3D('',#58434,#33793,#33794);
#27855=AXIS2_PLACEMENT_3D('',#59243,#33795,#33796);
#27856=AXIS2_PLACEMENT_3D('',#59411,#33797,#33798);
#27857=AXIS2_PLACEMENT_3D('',#59412,#33799,#33800);
#27858=AXIS2_PLACEMENT_3D('',#59413,#33801,#33802);
#27859=AXIS2_PLACEMENT_3D('',#59440,#33803,#33804);
#27860=AXIS2_PLACEMENT_3D('',#59441,#33805,#33806);
#27861=AXIS2_PLACEMENT_3D('',#59442,#33807,#33808);
#27862=AXIS2_PLACEMENT_3D('',#59678,#33809,#33810);
#27863=AXIS2_PLACEMENT_3D('',#59760,#33811,#33812);
#27864=AXIS2_PLACEMENT_3D('',#59919,#33813,#33814);
#27865=AXIS2_PLACEMENT_3D('',#59920,#33815,#33816);
#27866=AXIS2_PLACEMENT_3D('',#59921,#33817,#33818);
#27867=AXIS2_PLACEMENT_3D('',#60015,#33819,#33820);
#27868=AXIS2_PLACEMENT_3D('',#60532,#33821,#33822);
#27869=AXIS2_PLACEMENT_3D('',#60792,#33823,#33824);
#27870=AXIS2_PLACEMENT_3D('',#60793,#33825,#33826);
#27871=AXIS2_PLACEMENT_3D('',#60794,#33827,#33828);
#27872=AXIS2_PLACEMENT_3D('',#60820,#33829,#33830);
#27873=AXIS2_PLACEMENT_3D('',#60821,#33831,#33832);
#27874=AXIS2_PLACEMENT_3D('',#60822,#33833,#33834);
#27875=AXIS2_PLACEMENT_3D('',#60823,#33835,#33836);
#27876=AXIS2_PLACEMENT_3D('',#61155,#33837,#33838);
#27877=AXIS2_PLACEMENT_3D('',#61359,#33839,#33840);
#27878=AXIS2_PLACEMENT_3D('',#61459,#33841,#33842);
#27879=AXIS2_PLACEMENT_3D('',#61461,#33843,#33844);
#27880=AXIS2_PLACEMENT_3D('',#61462,#33845,#33846);
#27881=AXIS2_PLACEMENT_3D('',#61463,#33847,#33848);
#27882=AXIS2_PLACEMENT_3D('',#61464,#33849,#33850);
#27883=AXIS2_PLACEMENT_3D('',#61465,#33851,#33852);
#27884=AXIS2_PLACEMENT_3D('',#61698,#33853,#33854);
#27885=AXIS2_PLACEMENT_3D('',#62037,#33855,#33856);
#27886=AXIS2_PLACEMENT_3D('',#62317,#33857,#33858);
#27887=AXIS2_PLACEMENT_3D('',#62409,#33859,#33860);
#27888=AXIS2_PLACEMENT_3D('',#62410,#33861,#33862);
#27889=AXIS2_PLACEMENT_3D('',#62728,#33863,#33864);
#27890=AXIS2_PLACEMENT_3D('',#62787,#33865,#33866);
#27891=AXIS2_PLACEMENT_3D('',#62789,#33867,#33868);
#27892=AXIS2_PLACEMENT_3D('',#62790,#33869,#33870);
#27893=AXIS2_PLACEMENT_3D('',#62815,#33871,#33872);
#27894=AXIS2_PLACEMENT_3D('',#62816,#33873,#33874);
#27895=AXIS2_PLACEMENT_3D('',#63162,#33875,#33876);
#27896=AXIS2_PLACEMENT_3D('',#63320,#33877,#33878);
#27897=AXIS2_PLACEMENT_3D('',#63321,#33879,#33880);
#27898=AXIS2_PLACEMENT_3D('',#63413,#33881,#33882);
#27899=AXIS2_PLACEMENT_3D('',#63886,#33883,#33884);
#27900=AXIS2_PLACEMENT_3D('',#63887,#33885,#33886);
#27901=AXIS2_PLACEMENT_3D('',#63897,#33887,#33888);
#27902=AXIS2_PLACEMENT_3D('',#63898,#33889,#33890);
#27903=AXIS2_PLACEMENT_3D('',#63908,#33891,#33892);
#27904=AXIS2_PLACEMENT_3D('',#63909,#33893,#33894);
#27905=AXIS2_PLACEMENT_3D('',#63919,#33895,#33896);
#27906=AXIS2_PLACEMENT_3D('',#63920,#33897,#33898);
#27907=AXIS2_PLACEMENT_3D('',#63930,#33899,#33900);
#27908=AXIS2_PLACEMENT_3D('',#63931,#33901,#33902);
#27909=AXIS2_PLACEMENT_3D('',#63941,#33903,#33904);
#27910=AXIS2_PLACEMENT_3D('',#63942,#33905,#33906);
#27911=AXIS2_PLACEMENT_3D('',#63952,#33907,#33908);
#27912=AXIS2_PLACEMENT_3D('',#63953,#33909,#33910);
#27913=AXIS2_PLACEMENT_3D('',#63963,#33911,#33912);
#27914=AXIS2_PLACEMENT_3D('',#63964,#33913,#33914);
#27915=AXIS2_PLACEMENT_3D('',#63965,#33915,#33916);
#27916=AXIS2_PLACEMENT_3D('',#63967,#33917,#33918);
#27917=AXIS2_PLACEMENT_3D('',#63968,#33919,#33920);
#27918=AXIS2_PLACEMENT_3D('',#63970,#33921,#33922);
#27919=AXIS2_PLACEMENT_3D('',#63972,#33924,#33925);
#27920=AXIS2_PLACEMENT_3D('',#63974,#33926,#33927);
#27921=AXIS2_PLACEMENT_3D('',#63975,#33928,#33929);
#27922=AXIS2_PLACEMENT_3D('',#63977,#33930,#33931);
#27923=AXIS2_PLACEMENT_3D('',#63979,#33933,#33934);
#27924=AXIS2_PLACEMENT_3D('',#63981,#33935,#33936);
#27925=AXIS2_PLACEMENT_3D('',#63982,#33937,#33938);
#27926=AXIS2_PLACEMENT_3D('',#63984,#33939,#33940);
#27927=AXIS2_PLACEMENT_3D('',#63986,#33942,#33943);
#27928=AXIS2_PLACEMENT_3D('',#63988,#33944,#33945);
#27929=AXIS2_PLACEMENT_3D('',#63989,#33946,#33947);
#27930=AXIS2_PLACEMENT_3D('',#63991,#33948,#33949);
#27931=AXIS2_PLACEMENT_3D('',#63993,#33951,#33952);
#27932=AXIS2_PLACEMENT_3D('',#63995,#33953,#33954);
#27933=AXIS2_PLACEMENT_3D('',#63996,#33955,#33956);
#27934=AXIS2_PLACEMENT_3D('',#63999,#33958,#33959);
#27935=AXIS2_PLACEMENT_3D('',#64000,#33960,#33961);
#27936=AXIS2_PLACEMENT_3D('',#64002,#33962,#33963);
#27937=AXIS2_PLACEMENT_3D('',#64003,#33964,#33965);
#27938=AXIS2_PLACEMENT_3D('',#64006,#33967,#33968);
#27939=AXIS2_PLACEMENT_3D('',#64007,#33969,#33970);
#27940=AXIS2_PLACEMENT_3D('',#64009,#33971,#33972);
#27941=AXIS2_PLACEMENT_3D('',#64010,#33973,#33974);
#27942=AXIS2_PLACEMENT_3D('',#64013,#33976,#33977);
#27943=AXIS2_PLACEMENT_3D('',#64014,#33978,#33979);
#33511=DIRECTION('axis',(0.,0.,1.));
#33512=DIRECTION('refdir',(1.,0.,0.));
#33513=DIRECTION('center_axis',(-1.,0.,0.));
#33514=DIRECTION('ref_axis',(0.,0.,1.));
#33515=DIRECTION('center_axis',(-1.,0.,0.));
#33516=DIRECTION('ref_axis',(0.,0.923879532525282,-0.382683432331302));
#33517=DIRECTION('center_axis',(1.,0.,0.));
#33518=DIRECTION('ref_axis',(0.,-0.923879532525282,0.382683432331302));
#33519=DIRECTION('',(-1.,0.,0.));
#33520=DIRECTION('center_axis',(-1.,0.,0.));
#33521=DIRECTION('ref_axis',(0.,-0.923879532525282,0.382683432331302));
#33522=DIRECTION('center_axis',(-1.,0.,0.));
#33523=DIRECTION('ref_axis',(0.,0.,1.));
#33524=DIRECTION('center_axis',(-1.,0.,0.));
#33525=DIRECTION('ref_axis',(0.,0.382683432398878,-0.923879532497291));
#33526=DIRECTION('center_axis',(1.,0.,0.));
#33527=DIRECTION('ref_axis',(0.,-0.382683432398878,0.923879532497291));
#33528=DIRECTION('center_axis',(-1.,0.,0.));
#33529=DIRECTION('ref_axis',(0.,-0.382683432398878,0.923879532497291));
#33530=DIRECTION('',(-1.,0.,0.));
#33531=DIRECTION('center_axis',(-0.914213393717196,0.0442003138869465,0.402815346033865));
#33532=DIRECTION('ref_axis',(-0.263860958992393,0.689505825675568,-0.674506568299426));
#33533=DIRECTION('center_axis',(0.,-0.988888328046728,0.148660265884823));
#33534=DIRECTION('ref_axis',(1.,0.,0.));
#33535=DIRECTION('center_axis',(0.,-0.362081724527015,0.932146353725391));
#33536=DIRECTION('ref_axis',(1.,0.,0.));
#33537=DIRECTION('center_axis',(0.99999999999897,-1.32776773271782E-6,-5.45065136955466E-7));
#33538=DIRECTION('ref_axis',(1.43483054990958E-6,0.915158915916019,0.403093238119119));
#33539=DIRECTION('center_axis',(4.59701721133854E-17,0.403096564446046,
-0.915157450787456));
#33540=DIRECTION('ref_axis',(-0.0114743075678194,0.915097204111032,0.403070027779307));
#33541=DIRECTION('center_axis',(1.,-5.02651426597364E-10,-2.14769807745443E-10));
#33542=DIRECTION('ref_axis',(5.46578186166822E-10,0.915157853095838,0.403095651076784));
#33543=DIRECTION('center_axis',(3.99680239858264E-14,0.988888328046729,
-0.148660265884822));
#33544=DIRECTION('ref_axis',(0.797368987123014,0.089715294026903,0.596786280331648));
#33545=DIRECTION('center_axis',(-0.946369376470755,-0.140097818247825,0.291131593271074));
#33546=DIRECTION('ref_axis',(-0.0114718087515988,0.915097062809347,0.40307041970563));
#33547=DIRECTION('center_axis',(0.946369839460991,-0.140099137680288,0.291129453301823));
#33548=DIRECTION('ref_axis',(0.01147414714799,0.915097223790106,0.40306998766823));
#33549=DIRECTION('center_axis',(5.69602678185428E-6,-0.988889644020132,
0.148651511654917));
#33550=DIRECTION('ref_axis',(-0.999999999968588,-4.81341389039569E-6,6.29722243877274E-6));
#33551=DIRECTION('center_axis',(-0.946369839460985,0.1400991376803,-0.291129453301837));
#33552=DIRECTION('ref_axis',(-0.149612220002691,0.608622425476191,0.779227134302538));
#33553=DIRECTION('center_axis',(-4.95681495424892E-17,0.403096527878055,
-0.915157466894445));
#33554=DIRECTION('ref_axis',(-0.999999999986845,-4.69420780203386E-6,-2.06764292981134E-6));
#33555=DIRECTION('center_axis',(5.69064726501455E-6,-0.594138082881513,
-0.804363063819751));
#33556=DIRECTION('ref_axis',(-0.271605533892207,0.774125062247253,-0.571804881021329));
#33557=DIRECTION('center_axis',(-0.946369839249996,-0.106794560471235,0.304924661534112));
#33558=DIRECTION('ref_axis',(-0.149612220115205,0.981357835021728,-0.120635746085756));
#33559=DIRECTION('center_axis',(0.946369839249992,0.106794560471264,-0.304924661534114));
#33560=DIRECTION('ref_axis',(-0.271594468689797,0.774133377076023,-0.571798879916688));
#33561=DIRECTION('center_axis',(2.16840404869328E-18,-0.362081762350744,
0.93214633903319));
#33562=DIRECTION('ref_axis',(0.0114792119266392,0.932084921473315,0.362057905390321));
#33563=DIRECTION('center_axis',(1.,1.42364623010903E-9,-3.43713428943404E-9));
#33564=DIRECTION('ref_axis',(8.26276396146569E-11,0.915158418800611,0.403094366741047));
#33565=DIRECTION('center_axis',(0.999999999985404,-4.99170952627699E-6,
-2.06763424365629E-6));
#33566=DIRECTION('ref_axis',(5.40165508683492E-6,0.915152953201646,0.403106775206182));
#33567=DIRECTION('center_axis',(-0.946369788026362,0.106794703559617,-0.304924770398459));
#33568=DIRECTION('ref_axis',(-0.0114740731618296,0.932084948692918,0.362057998206362));
#33569=DIRECTION('center_axis',(0.,0.362081724527009,-0.932146353725394));
#33570=DIRECTION('ref_axis',(0.703038340194793,0.662897694664692,0.257495123496325));
#33571=DIRECTION('center_axis',(8.39574346860379E-6,-0.594120071126927,
-0.804376367761788));
#33572=DIRECTION('ref_axis',(0.999999999695544,2.3652778284159E-5,-7.03258707988771E-6));
#33573=DIRECTION('center_axis',(0.914210471289562,-0.316088169069029,0.253589202370894));
#33574=DIRECTION('ref_axis',(-0.277774690008402,-0.944426060401927,-0.17578577310019));
#33575=DIRECTION('center_axis',(0.,-0.594130960497972,0.804368324698181));
#33576=DIRECTION('ref_axis',(1.,0.,0.));
#33577=DIRECTION('center_axis',(0.,0.403096565020755,0.915157450534316));
#33578=DIRECTION('ref_axis',(1.,0.,0.));
#33579=DIRECTION('center_axis',(0.99999999999897,-1.32419981462018E-6,5.53416423203211E-7));
#33580=DIRECTION('ref_axis',(1.43473013400941E-6,0.932145037436602,-0.362085113171279));
#33581=DIRECTION('center_axis',(-3.66026653431106E-16,-0.362081725112371,
-0.932146353498017));
#33582=DIRECTION('ref_axis',(-0.0114743075678202,0.932084988407572,-0.36205788853593));
#33583=DIRECTION('center_axis',(1.,-5.07454201753425E-10,2.03628947473516E-10));
#33584=DIRECTION('ref_axis',(5.46751918028468E-10,0.932145992118772,-0.362082655448878));
#33585=DIRECTION('center_axis',(5.32906986477686E-15,0.59413096049796,-0.804368324698189));
#33586=DIRECTION('ref_axis',(0.797368987123025,0.485429918524157,0.358553332959033));
#33587=DIRECTION('center_axis',(-0.946369376471585,0.106797006503074,0.304925241130946));
#33588=DIRECTION('ref_axis',(-0.0114718087598166,0.932085165620904,-0.362057511499527));
#33589=DIRECTION('center_axis',(0.946369839460996,0.10679456034074,0.304924660924952));
#33590=DIRECTION('ref_axis',(0.0114741471479901,0.932084973959935,-0.362057930814027));
#33591=DIRECTION('center_axis',(-0.914215241706711,-0.316082336098155,-0.253579274858719));
#33592=DIRECTION('ref_axis',(0.277774402486775,-0.94442900415313,0.175770411154555));
#33593=DIRECTION('center_axis',(5.69660925919776E-6,-0.594138082100489,
0.804363064396608));
#33594=DIRECTION('ref_axis',(-0.999999999968596,1.04716010024955E-6,7.85561549530932E-6));
#33595=DIRECTION('center_axis',(-0.946369839460982,-0.106794560340743,-0.304924660924994));
#33596=DIRECTION('ref_axis',(-0.149612220002695,0.981357834986306,0.120635746513443));
#33597=DIRECTION('center_axis',(2.5539691584425E-16,-0.362081762359287,
-0.932146339029872));
#33598=DIRECTION('ref_axis',(-0.999999999986845,-4.78135051973835E-6,1.85726183743932E-6));
#33599=DIRECTION('center_axis',(5.691173724172E-6,-0.988889644483067,-0.148651508575471));
#33600=DIRECTION('ref_axis',(-0.27160553388917,0.143061970992072,-0.951716190057016));
#33601=DIRECTION('center_axis',(-0.946369839249997,0.140099138018724,0.291129453824832));
#33602=DIRECTION('ref_axis',(-0.149612220115206,0.6086224258037,-0.779227134025131));
#33603=DIRECTION('center_axis',(0.946369839249986,-0.140099138018723,-0.291129453824869));
#33604=DIRECTION('ref_axis',(-0.271594468689809,0.143072095009363,-0.951717825937253));
#33605=DIRECTION('center_axis',(-4.62303743181407E-16,0.403096527886377,
0.915157466890779));
#33606=DIRECTION('ref_axis',(0.0114792119266392,0.915097168699214,-0.403069968531799));
#33607=DIRECTION('center_axis',(1.,-1.42372070955575E-9,-3.43716518285929E-9));
#33608=DIRECTION('ref_axis',(8.25724334042756E-11,0.932145483973677,-0.362083963615458));
#33609=DIRECTION('center_axis',(0.999999999985404,-4.99170901781618E-6,
2.06763312228972E-6));
#33610=DIRECTION('ref_axis',(5.40165418784382E-6,0.93215039391184,-0.36207132322351));
#33611=DIRECTION('center_axis',(-0.946369788026357,-0.1400991138187,-0.291129631982323));
#33612=DIRECTION('ref_axis',(-0.0114740731618291,0.915097253577214,-0.403069922148152));
#33613=DIRECTION('center_axis',(-7.10542735092901E-15,-0.403096565020731,
-0.915157450534326));
#33614=DIRECTION('ref_axis',(0.703038340194823,0.650816003077036,-0.286662907183576));
#33615=DIRECTION('center_axis',(8.39582282804934E-6,-0.988886315401232,
-0.148673653152415));
#33616=DIRECTION('ref_axis',(0.999999999695544,1.17523290285004E-5,-2.16978224223302E-5));
#33617=DIRECTION('center_axis',(0.914211011085666,-0.0441933407252092,0.402821518597591));
#33618=DIRECTION('ref_axis',(-0.277773809559331,-0.79210955948066,0.543510953433555));
#33619=DIRECTION('center_axis',(0.,0.148660265884823,0.988888328046728));
#33620=DIRECTION('ref_axis',(1.,0.,0.));
#33621=DIRECTION('center_axis',(0.,0.932146353725392,0.362081724527015));
#33622=DIRECTION('ref_axis',(1.,0.,0.));
#33623=DIRECTION('center_axis',(0.999999999998973,-5.4644975272136E-7,1.32480760523532E-6));
#33624=DIRECTION('ref_axis',(1.43267969207677E-6,0.403093238650518,-0.915158915681962));
#33625=DIRECTION('center_axis',(5.46437894932694E-17,-0.915157450787408,
-0.403096564446155));
#33626=DIRECTION('ref_axis',(-0.0114743075683094,0.403070027779414,-0.915097204110979));
#33627=DIRECTION('center_axis',(1.,-2.14814139094165E-10,5.02758452718822E-10));
#33628=DIRECTION('ref_axis',(5.46693998289738E-10,0.403095651075575,-0.915157853096371));
#33629=DIRECTION('center_axis',(-1.15463180403498E-14,-0.148660265884754,
-0.988888328046739));
#33630=DIRECTION('ref_axis',(0.797368987123014,0.596786280331648,-0.089715294026903));
#33631=DIRECTION('center_axis',(-0.946369373547254,0.291131604593958,0.140097814466623));
#33632=DIRECTION('ref_axis',(-0.0114717933272592,0.40307043850639,-0.915097054721587));
#33633=DIRECTION('center_axis',(0.946369839460991,0.291129453301823,0.140099137680288));
#33634=DIRECTION('ref_axis',(0.01147414714799,0.40306998766823,-0.915097223790106));
#33635=DIRECTION('center_axis',(5.69602883164937E-6,0.148651511653502,0.988889644020345));
#33636=DIRECTION('ref_axis',(-0.999999999968588,6.29722269189983E-6,4.81341592428572E-6));
#33637=DIRECTION('center_axis',(-0.946369839460985,-0.291129453301837,-0.1400991376803));
#33638=DIRECTION('ref_axis',(-0.149612220002691,0.779227134302538,-0.608622425476191));
#33639=DIRECTION('center_axis',(4.98146360964622E-17,-0.915157466894445,
-0.403096527878055));
#33640=DIRECTION('ref_axis',(-0.999999999986845,-2.06764294367606E-6,4.69420783326464E-6));
#33641=DIRECTION('center_axis',(5.69120438802073E-6,-0.804363063194495,
0.594138083727999));
#33642=DIRECTION('ref_axis',(-0.271605533891507,-0.571804881957827,-0.774125061555757));
#33643=DIRECTION('center_axis',(-0.946369839249996,0.304924661534112,0.106794560471235));
#33644=DIRECTION('ref_axis',(-0.149612220115205,-0.120635746085756,-0.981357835021728));
#33645=DIRECTION('center_axis',(0.946369839249991,-0.30492466153412,-0.106794560471258));
#33646=DIRECTION('ref_axis',(-0.271594468689797,-0.571798879916688,-0.774133377076023));
#33647=DIRECTION('center_axis',(-8.67361619477312E-19,0.93214633903319,
0.362081762350744));
#33648=DIRECTION('ref_axis',(0.0114792119266496,0.362057905390321,-0.932084921473315));
#33649=DIRECTION('center_axis',(1.,-3.47834350169931E-9,-1.44071563802809E-9));
#33650=DIRECTION('ref_axis',(8.36176223912445E-11,0.403094366741542,-0.915158418800393));
#33651=DIRECTION('center_axis',(0.999999999985404,-2.06763381357569E-6,
4.99170850549968E-6));
#33652=DIRECTION('ref_axis',(5.40165397924269E-6,0.403106775646763,-0.915152953007579));
#33653=DIRECTION('center_axis',(-0.946369788023275,-0.304924770411269,-0.10679470355039));
#33654=DIRECTION('ref_axis',(-0.0114740731721401,0.362057998196173,-0.932084948696749));
#33655=DIRECTION('center_axis',(0.,-0.932146353725394,-0.362081724527009));
#33656=DIRECTION('ref_axis',(0.703038340194793,0.257495123496325,-0.662897694664692));
#33657=DIRECTION('center_axis',(8.39572065812752E-6,-0.804376367758035,
0.594120071132009));
#33658=DIRECTION('ref_axis',(0.999999999695545,-7.03260613071095E-6,-2.36527656856413E-5));
#33659=DIRECTION('center_axis',(0.914195196760818,0.253611443836588,0.31611450105076));
#33660=DIRECTION('ref_axis',(-0.277797379909012,-0.175793291241973,0.944417987159289));
#33661=DIRECTION('center_axis',(-0.914213474905294,0.253579021042076,-0.31608764985195));
#33662=DIRECTION('ref_axis',(-0.263860852594192,-0.964502442909986,-0.0106060402099417));
#33663=DIRECTION('center_axis',(0.,0.804368324698181,0.594130960497972));
#33664=DIRECTION('ref_axis',(1.,0.,0.));
#33665=DIRECTION('center_axis',(0.,0.915157450534316,-0.403096565020755));
#33666=DIRECTION('ref_axis',(1.,0.,0.));
#33667=DIRECTION('center_axis',(0.99999999999897,5.53268491474173E-7,1.32429836705055E-6));
#33668=DIRECTION('ref_axis',(1.43476843527578E-6,-0.362085113182452,-0.932145037432262));
#33669=DIRECTION('center_axis',(-1.14361645153771E-15,-0.932146353498067,
0.362081725112241));
#33670=DIRECTION('ref_axis',(-0.0114743075683103,-0.362057888535797,-0.932084988407617));
#33671=DIRECTION('center_axis',(1.,2.03540282763477E-10,5.0724014766387E-10));
#33672=DIRECTION('ref_axis',(5.46520268530975E-10,-0.362082655389443,-0.932145992141859));
#33673=DIRECTION('center_axis',(5.32906986477686E-15,-0.804368324698189,
-0.59413096049796));
#33674=DIRECTION('ref_axis',(0.797368987123025,0.358553332959033,-0.485429918524157));
#33675=DIRECTION('center_axis',(-0.946369376469017,0.304925241133014,-0.106797006519928));
#33676=DIRECTION('ref_axis',(-0.0114718087425804,-0.362057511495606,-0.932085165622639));
#33677=DIRECTION('center_axis',(0.946369839461072,0.304924660924732,-0.106794560340695));
#33678=DIRECTION('ref_axis',(0.0114741471479501,-0.362057930814027,-0.932084973959935));
#33679=DIRECTION('center_axis',(5.6966045490687E-6,0.804363064404739,0.59413808208948));
#33680=DIRECTION('ref_axis',(-0.999999999968597,7.8555843946347E-6,-1.04712592387451E-6));
#33681=DIRECTION('center_axis',(-0.946369839461086,-0.304924660924705,0.10679456034065));
#33682=DIRECTION('ref_axis',(-0.149612220002605,0.120635746513636,-0.981357834986296));
#33683=DIRECTION('center_axis',(-8.80522392098827E-17,-0.932146339029872,
0.362081762359287));
#33684=DIRECTION('ref_axis',(-0.999999999986845,1.85726372854635E-6,4.78135538727166E-6));
#33685=DIRECTION('center_axis',(0.914218329687893,-0.402804400843518,-0.0441979674167706));
#33686=DIRECTION('ref_axis',(0.263856242961101,0.674512925090226,-0.689501411845313));
#33687=DIRECTION('center_axis',(5.69118558432375E-6,-0.148651508574067,
0.988889644483278));
#33688=DIRECTION('ref_axis',(-0.271605533890658,-0.951716190057283,-0.143061970987472));
#33689=DIRECTION('center_axis',(-0.946369839249939,0.291129453824956,-0.14009913801886));
#33690=DIRECTION('ref_axis',(-0.149612220115201,-0.779227134025074,-0.608622425803773));
#33691=DIRECTION('center_axis',(0.946369839249922,-0.291129453825002,0.140099138018879));
#33692=DIRECTION('ref_axis',(-0.271594468689889,-0.951717825937198,-0.143072095009577));
#33693=DIRECTION('center_axis',(-4.66640551278794E-16,0.915157466890779,
-0.403096527886377));
#33694=DIRECTION('ref_axis',(0.0114792119231403,-0.403069968531815,-0.915097168699251));
#33695=DIRECTION('center_axis',(1.,-3.48100020628989E-9,1.44187777759703E-9));
#33696=DIRECTION('ref_axis',(8.3625497048937E-11,-0.362083963618991,-0.932145483972304));
#33697=DIRECTION('center_axis',(0.999999999985404,2.06763318526536E-6,4.99170918161415E-6));
#33698=DIRECTION('ref_axis',(5.4016543633521E-6,-0.362071323230482,-0.932150393909132));
#33699=DIRECTION('center_axis',(-0.946369788023279,-0.291129631984834,0.140099113834277));
#33700=DIRECTION('ref_axis',(-0.0114740731721399,-0.403069922158076,-0.915097253572714));
#33701=DIRECTION('center_axis',(-7.10542735092901E-15,-0.915157450534326,
0.403096565020731));
#33702=DIRECTION('ref_axis',(0.703038340194823,-0.286662907183576,-0.650816003077037));
#33703=DIRECTION('center_axis',(8.39591592211414E-6,-0.148673653342516,
0.988886315372651));
#33704=DIRECTION('ref_axis',(0.999999999695531,-2.16983267807876E-5,-1.1752498999848E-5));
#33705=DIRECTION('center_axis',(0.914232678033534,0.402769058919062,0.0442232472019623));
#33706=DIRECTION('ref_axis',(-0.263805189109609,0.674511229537102,-0.68952260545046));
#33707=DIRECTION('center_axis',(0.,0.988888328046741,-0.148660265884739));
#33708=DIRECTION('ref_axis',(1.,0.,0.));
#33709=DIRECTION('center_axis',(0.,0.362081724527015,-0.932146353725391));
#33710=DIRECTION('ref_axis',(1.,0.,0.));
#33711=DIRECTION('center_axis',(0.99999999999897,1.32768040064921E-6,5.45217781452942E-7));
#33712=DIRECTION('ref_axis',(1.43481215715695E-6,-0.915158915917704,-0.403093238115296));
#33713=DIRECTION('center_axis',(-6.33174068731535E-17,-0.403096564446156,
0.915157450787408));
#33714=DIRECTION('ref_axis',(-0.0114743075687795,-0.915097204110974,-0.403070027779412));
#33715=DIRECTION('center_axis',(1.,5.02650926101981E-10,2.14770992296926E-10));
#33716=DIRECTION('ref_axis',(5.46578188866671E-10,-0.915157853076047,-0.403095651121716));
#33717=DIRECTION('center_axis',(-1.24344963511336E-14,-0.988888328046739,
0.148660265884755));
#33718=DIRECTION('ref_axis',(0.797368987123014,-0.0897152940269056,-0.596786280331648));
#33719=DIRECTION('center_axis',(-0.946369376466823,0.140097818233099,-0.29113159329094));
#33720=DIRECTION('ref_axis',(-0.0114718087263466,-0.915097062806538,-0.403070419712726));
#33721=DIRECTION('center_axis',(0.946369839461063,0.140099137680155,-0.291129453301653));
#33722=DIRECTION('ref_axis',(0.0114741471479502,-0.915097223790127,-0.403069987668184));
#33723=DIRECTION('center_axis',(-0.914215226225209,0.044196341358579,0.402811622906422));
#33724=DIRECTION('ref_axis',(0.277774424362039,0.792100604739657,0.54352368958621));
#33725=DIRECTION('center_axis',(5.69601044024649E-6,0.988889644017464,-0.148651511672664));
#33726=DIRECTION('ref_axis',(-0.999999999968588,4.81340434744809E-6,-6.29717598173139E-6));
#33727=DIRECTION('center_axis',(-0.946369839461086,-0.140099137680153,0.291129453301579));
#33728=DIRECTION('ref_axis',(-0.149612220002599,-0.608622425476095,-0.77922713430263));
#33729=DIRECTION('center_axis',(2.82299102089821E-17,-0.403096527878027,
0.915157466894457));
#33730=DIRECTION('ref_axis',(-0.999999999986845,4.69421254877053E-6,2.06764502067634E-6));
#33731=DIRECTION('center_axis',(5.69062401486436E-6,0.594138082870581,0.804363063827826));
#33732=DIRECTION('ref_axis',(-0.271605533887031,-0.774125062259951,0.571804881006597));
#33733=DIRECTION('center_axis',(-0.946369839249936,0.106794560471239,-0.304924661534296));
#33734=DIRECTION('ref_axis',(-0.149612220115201,-0.981357835021745,0.120635746085621));
#33735=DIRECTION('center_axis',(0.946369839249922,-0.106794560471299,0.304924661534318));
#33736=DIRECTION('ref_axis',(-0.271594468689908,-0.774133377076162,0.571798879916447));
#33737=DIRECTION('center_axis',(6.07153133634118E-18,0.362081762350716,
-0.932146339033201));
#33738=DIRECTION('ref_axis',(0.0114792119231299,-0.932084921473364,-0.362057905390307));
#33739=DIRECTION('center_axis',(1.,-1.44189805230485E-9,3.48090292427251E-9));
#33740=DIRECTION('ref_axis',(8.35672300487615E-11,-0.915158418800003,-0.403094366742427));
#33741=DIRECTION('center_axis',(0.999999999985404,4.99170888905771E-6,2.06763397278594E-6));
#33742=DIRECTION('ref_axis',(5.40165439448914E-6,-0.915152953203479,-0.403106775202021));
#33743=DIRECTION('center_axis',(-0.94636978802022,-0.106794703541145,0.304924770423991));
#33744=DIRECTION('ref_axis',(-0.0114740731824407,-0.932084948700573,-0.362057998186));
#33745=DIRECTION('center_axis',(0.,-0.362081724527009,0.932146353725394));
#33746=DIRECTION('ref_axis',(0.703038340194793,-0.662897694664692,-0.257495123496325));
#33747=DIRECTION('center_axis',(8.39592187383702E-6,0.594120070955224,0.804376367888607));
#33748=DIRECTION('ref_axis',(0.999999999695531,-2.36533086150239E-5,7.03275698865841E-6));
#33749=DIRECTION('center_axis',(0.,0.594130960497972,-0.804368324698181));
#33750=DIRECTION('ref_axis',(1.,0.,0.));
#33751=DIRECTION('center_axis',(0.,-0.403096565020755,-0.915157450534316));
#33752=DIRECTION('ref_axis',(1.,0.,0.));
#33753=DIRECTION('center_axis',(0.999999999998959,1.33168050215377E-6,-5.56325015337109E-7));
#33754=DIRECTION('ref_axis',(1.44275637767322E-6,-0.932145037436202,0.362085113172275));
#33755=DIRECTION('center_axis',(-3.49546780409327E-16,0.362081725112241,
0.932146353498067));
#33756=DIRECTION('ref_axis',(-0.01147430756877,-0.932084988407612,0.362057888535795));
#33757=DIRECTION('center_axis',(1.,5.0702609627477E-10,-2.034516191357E-10));
#33758=DIRECTION('ref_axis',(5.46288644440416E-10,-0.932145992141857,0.362082655389447));
#33759=DIRECTION('center_axis',(5.32906986477153E-15,-0.59413096049796,
0.804368324698189));
#33760=DIRECTION('ref_axis',(0.797368987123024,-0.485429918524159,-0.358553332959033));
#33761=DIRECTION('center_axis',(-0.946369376467426,-0.106797006532308,-0.304925241133614));
#33762=DIRECTION('ref_axis',(-0.0114718087296023,-0.932085165623876,0.362057511492832));
#33763=DIRECTION('center_axis',(0.946369839461072,-0.106794560340695,-0.304924660924732));
#33764=DIRECTION('ref_axis',(0.0114741471479501,-0.932084973959935,0.362057930814027));
#33765=DIRECTION('center_axis',(5.69661023326282E-6,0.594138082092942,-0.804363064402183));
#33766=DIRECTION('ref_axis',(-0.999999999968597,-1.04711976004056E-6,-7.85558690927704E-6));
#33767=DIRECTION('center_axis',(-0.946369839461086,0.10679456034065,0.304924660924705));
#33768=DIRECTION('ref_axis',(-0.149612220002605,-0.981357834986296,-0.120635746513635));
#33769=DIRECTION('center_axis',(-9.82680269052054E-16,0.362081762359287,
0.932146339029872));
#33770=DIRECTION('ref_axis',(-0.999999999986845,4.78135531787353E-6,-1.85726370254917E-6));
#33771=DIRECTION('center_axis',(0.914207423386785,-0.0441978182448416,0.402829169607777));
#33772=DIRECTION('ref_axis',(0.277780035610593,0.792112742359119,-0.54350313265748));
#33773=DIRECTION('center_axis',(5.69063497141659E-6,0.988889644328729,0.14865150960221));
#33774=DIRECTION('ref_axis',(-0.271605533888581,-0.143061972124941,0.951716189886891));
#33775=DIRECTION('center_axis',(-0.946369839249939,-0.14009913801886,-0.291129453824956));
#33776=DIRECTION('ref_axis',(-0.149612220115201,-0.608622425803773,0.779227134025074));
#33777=DIRECTION('center_axis',(0.946369839249922,0.140099138018879,0.291129453825002));
#33778=DIRECTION('ref_axis',(-0.271594468689889,-0.143072095009577,0.951717825937198));
#33779=DIRECTION('center_axis',(-4.64905828039839E-16,-0.403096527886377,
-0.915157466890779));
#33780=DIRECTION('ref_axis',(0.0114792119231195,-0.915097168699251,0.403069968531815));
#33781=DIRECTION('center_axis',(1.,1.44185618820045E-9,3.48094808359834E-9));
#33782=DIRECTION('ref_axis',(8.36242449135707E-11,-0.932145483976129,0.362083963609144));
#33783=DIRECTION('center_axis',(0.999999999985404,4.99171031427304E-6,-2.06763364991969E-6));
#33784=DIRECTION('ref_axis',(5.401655587451E-6,-0.93215039373556,0.362071323677343));
#33785=DIRECTION('center_axis',(-0.946369788020201,0.140099113849831,0.291129631987354));
#33786=DIRECTION('ref_axis',(-0.0114740731824505,-0.915097253568243,0.403069922167932));
#33787=DIRECTION('center_axis',(-7.10542735092901E-15,0.403096565020731,
0.915157450534326));
#33788=DIRECTION('ref_axis',(0.703038340194823,-0.650816003077036,0.286662907183576));
#33789=DIRECTION('center_axis',(8.39589975016415E-6,0.988886315372978,0.148673653340339));
#33790=DIRECTION('ref_axis',(0.999999999695531,-1.1752482826665E-5,2.16983279843357E-5));
#33791=DIRECTION('center_axis',(0.91423776319055,0.0441882734077247,-0.402761354712172));
#33792=DIRECTION('ref_axis',(-0.277733517155144,0.792111374696756,-0.543528898518422));
#33793=DIRECTION('center_axis',(0.,-0.804368324698238,-0.594130960497894));
#33794=DIRECTION('ref_axis',(1.,0.,0.));
#33795=DIRECTION('center_axis',(-0.946369376471938,-0.304925241130843,0.106797006500241));
#33796=DIRECTION('ref_axis',(-0.0114718087725454,0.362057511526751,0.932085165610172));
#33797=DIRECTION('center_axis',(0.946369839460996,-0.304924660924952,0.10679456034074));
#33798=DIRECTION('ref_axis',(0.0114741471479901,0.362057930814027,0.932084973959935));
#33799=DIRECTION('center_axis',(6.21724817557921E-15,0.804368324698188,
0.594130960497961));
#33800=DIRECTION('ref_axis',(0.797368987123025,-0.358553332959034,0.485429918524156));
#33801=DIRECTION('center_axis',(-3.62123525610159E-16,0.932146353497273,
-0.362081725114285));
#33802=DIRECTION('ref_axis',(-0.0114743075668696,0.362057888537847,0.932084988406839));
#33803=DIRECTION('center_axis',(0.,-0.915157450534316,0.403096565020755));
#33804=DIRECTION('ref_axis',(1.,0.,0.));
#33805=DIRECTION('center_axis',(0.99999999999897,-5.53543085154133E-7,-1.32450328423587E-6));
#33806=DIRECTION('ref_axis',(1.43505887409419E-6,0.36208511306403,0.932145037478261));
#33807=DIRECTION('center_axis',(1.,-2.03585803597008E-10,-5.07346683735424E-10));
#33808=DIRECTION('ref_axis',(5.46636077372728E-10,0.362082655398668,0.932145992138275));
#33809=DIRECTION('center_axis',(1.,3.43715707468504E-9,-1.42371735165538E-9));
#33810=DIRECTION('ref_axis',(8.25722386253937E-11,0.362083963618065,0.932145483972664));
#33811=DIRECTION('center_axis',(-0.946369788029458,0.291129631979785,-0.140099113803026));
#33812=DIRECTION('ref_axis',(-0.0114740731514592,0.403069922138164,0.915097253581743));
#33813=DIRECTION('center_axis',(0.946369839249986,0.291129453824869,-0.140099138018723));
#33814=DIRECTION('ref_axis',(-0.271594468689809,0.951717825937253,0.143072095009363));
#33815=DIRECTION('center_axis',(-6.21724893205666E-15,0.915157450534326,
-0.403096565020732));
#33816=DIRECTION('ref_axis',(0.703038340194823,0.286662907183576,0.650816003077036));
#33817=DIRECTION('center_axis',(8.39574223448429E-6,0.148673653134807,-0.98888631540388));
#33818=DIRECTION('ref_axis',(0.999999999695544,2.16978339305183E-5,1.17522492591548E-5));
#33819=DIRECTION('center_axis',(0.914205544031138,-0.4028338123391,-0.0441943763286409));
#33820=DIRECTION('ref_axis',(-0.277781996737481,-0.543507170848629,-0.792109283826832));
#33821=DIRECTION('center_axis',(0.914204745777582,0.402835190649233,0.0441983254472605));
#33822=DIRECTION('ref_axis',(0.27778213558618,-0.543496513633425,-0.792116547496323));
#33823=DIRECTION('center_axis',(5.69119916378401E-6,0.148651508534004,-0.988889644489301));
#33824=DIRECTION('ref_axis',(-0.271605533901061,0.951716190060724,0.143061970944832));
#33825=DIRECTION('center_axis',(-0.946369839249997,-0.291129453824832,0.140099138018724));
#33826=DIRECTION('ref_axis',(-0.149612220115206,0.779227134025131,0.6086224258037));
#33827=DIRECTION('center_axis',(3.61689795277913E-16,-0.915157466892033,
0.40309652788353));
#33828=DIRECTION('ref_axis',(0.0114792119270605,0.40306996852895,0.915097168700464));
#33829=DIRECTION('center_axis',(-5.78221668413099E-16,0.932146339028668,
-0.362081762362386));
#33830=DIRECTION('ref_axis',(-0.999999999986845,-1.85727697257704E-6,-4.78138948141498E-6));
#33831=DIRECTION('center_axis',(0.999999999985307,-2.07451115399164E-6,
-5.00831315533298E-6));
#33832=DIRECTION('ref_axis',(5.41962207941293E-6,0.362071324606221,0.932150393374655));
#33833=DIRECTION('center_axis',(-0.946369839460982,0.304924660924994,-0.106794560340743));
#33834=DIRECTION('ref_axis',(-0.149612220002695,-0.120635746513443,0.981357834986306));
#33835=DIRECTION('center_axis',(5.69602760281014E-6,-0.804363065044909,
-0.594138081222803));
#33836=DIRECTION('ref_axis',(-0.999999999968588,-7.85643176174389E-6,1.04924418822824E-6));
#33837=DIRECTION('center_axis',(-0.914212817311013,-0.402816410519734,0.0442025347718617));
#33838=DIRECTION('ref_axis',(-0.263860258991997,0.674506642529295,0.689506020937115));
#33839=DIRECTION('center_axis',(0.,-0.148660265884688,-0.988888328046749));
#33840=DIRECTION('ref_axis',(1.,0.,0.));
#33841=DIRECTION('center_axis',(0.,-0.932146353725392,-0.362081724527015));
#33842=DIRECTION('ref_axis',(1.,0.,0.));
#33843=DIRECTION('center_axis',(0.99999999999897,5.47330121552162E-7,-1.32692265765345E-6));
#33844=DIRECTION('ref_axis',(1.43497017188914E-6,-0.403093238651766,0.915158915681408));
#33845=DIRECTION('center_axis',(5.03069808033274E-17,0.915157450787411,
0.403096564446147));
#33846=DIRECTION('ref_axis',(-0.0114743075692297,-0.403070027779401,0.915097204110973));
#33847=DIRECTION('center_axis',(1.,2.14836896434712E-10,-5.02811714092292E-10));
#33848=DIRECTION('ref_axis',(5.46751921211513E-10,-0.403095651121802,0.915157853076009));
#33849=DIRECTION('center_axis',(-1.24344963511336E-14,0.148660265884755,
0.988888328046739));
#33850=DIRECTION('ref_axis',(0.797368987123014,-0.596786280331648,0.0897152940269056));
#33851=DIRECTION('center_axis',(-0.946369373540832,-0.291131604623066,-0.140097814449519));
#33852=DIRECTION('ref_axis',(-0.0114717932857128,-0.403070438540629,0.915097054707027));
#33853=DIRECTION('center_axis',(0.946369839461063,-0.291129453301653,-0.140099137680155));
#33854=DIRECTION('ref_axis',(0.0114741471479502,-0.403069987668184,0.915097223790127));
#33855=DIRECTION('center_axis',(-0.914214770745398,0.402812647158067,-0.0441964279150493));
#33856=DIRECTION('ref_axis',(0.277778098123834,0.54353084089538,-0.792094409270932));
#33857=DIRECTION('center_axis',(5.69660473288689E-6,-0.148651510563523,
-0.988889644184189));
#33858=DIRECTION('ref_axis',(-0.999999999968597,-6.29516651701536E-6,-4.81430738979412E-6));
#33859=DIRECTION('center_axis',(-0.946369839461086,0.291129453301579,0.140099137680153));
#33860=DIRECTION('ref_axis',(-0.149612220002599,-0.77922713430263,0.608622425476095));
#33861=DIRECTION('center_axis',(-5.33840324484981E-17,0.915157466894457,
0.403096527878027));
#33862=DIRECTION('ref_axis',(-0.999999999986845,2.06764506632629E-6,-4.69421265261294E-6));
#33863=DIRECTION('center_axis',(5.69062333891971E-6,0.804363063828125,-0.594138082870176));
#33864=DIRECTION('ref_axis',(-0.271605533887638,0.571804881005956,0.774125062260211));
#33865=DIRECTION('center_axis',(-0.946369839249936,-0.304924661534296,-0.106794560471239));
#33866=DIRECTION('ref_axis',(-0.149612220115201,0.120635746085621,0.981357835021745));
#33867=DIRECTION('center_axis',(0.946369839249921,0.304924661534324,0.106794560471294));
#33868=DIRECTION('ref_axis',(-0.271594468689907,0.571798879916447,0.774133377076162));
#33869=DIRECTION('center_axis',(6.07153133634118E-18,-0.932146339033201,
-0.362081762350716));
#33870=DIRECTION('ref_axis',(0.0114792119231299,-0.362057905390307,0.932084921473364));
#33871=DIRECTION('center_axis',(1.,3.48092280083978E-9,1.44184515186693E-9));
#33872=DIRECTION('ref_axis',(8.3623632745154E-11,-0.403094366742872,0.915158418799807));
#33873=DIRECTION('center_axis',(0.999999999985404,2.06763417181339E-6,-4.99170934833527E-6));
#33874=DIRECTION('ref_axis',(5.40165489491138E-6,-0.403106776244474,0.915152952744299));
#33875=DIRECTION('center_axis',(-0.946369788017145,0.304924770436739,0.106794703531991));
#33876=DIRECTION('ref_axis',(-0.0114740731926795,-0.362057998175877,0.93208494870438));
#33877=DIRECTION('center_axis',(0.,0.932146353725394,0.362081724527009));
#33878=DIRECTION('ref_axis',(0.703038340194793,-0.257495123496325,0.662897694664692));
#33879=DIRECTION('center_axis',(8.39546862823305E-6,0.804376367829452,-0.594120071035321));
#33880=DIRECTION('ref_axis',(0.999999999695535,7.03312350208447E-6,2.36530419473628E-5));
#33881=DIRECTION('center_axis',(0.91416849261592,-0.253716090150975,-0.316107754898293));
#33882=DIRECTION('ref_axis',(-0.263983855302915,-0.964467992945735,0.0106777676803009));
#33883=DIRECTION('center_axis',(1.,0.,0.));
#33884=DIRECTION('ref_axis',(0.,0.8413441809447,0.54049974023166));
#33885=DIRECTION('center_axis',(-1.,0.,0.));
#33886=DIRECTION('ref_axis',(0.,0.54049869329636,0.8413448535202));
#33887=DIRECTION('center_axis',(1.,0.,0.));
#33888=DIRECTION('ref_axis',(0.,0.97711086402508,-0.212730720405307));
#33889=DIRECTION('center_axis',(-1.,0.,0.));
#33890=DIRECTION('ref_axis',(0.,0.977110930685622,0.212730414221093));
#33891=DIRECTION('center_axis',(1.,0.,0.));
#33892=DIRECTION('ref_axis',(0.,0.540499043132554,-0.841344628777526));
#33893=DIRECTION('center_axis',(-1.,0.,0.));
#33894=DIRECTION('ref_axis',(0.,0.841344788899846,-0.540498793884939));
#33895=DIRECTION('center_axis',(1.,0.,0.));
#33896=DIRECTION('ref_axis',(0.,-0.212729213948611,-0.977111192000586));
#33897=DIRECTION('center_axis',(-1.,0.,0.));
#33898=DIRECTION('ref_axis',(0.,0.212730320256165,-0.977110951143067));
#33899=DIRECTION('center_axis',(1.,0.,0.));
#33900=DIRECTION('ref_axis',(0.,-0.841345052956848,-0.540498382851456));
#33901=DIRECTION('center_axis',(-1.,0.,0.));
#33902=DIRECTION('ref_axis',(0.,-0.540502256823511,-0.841342564220242));
#33903=DIRECTION('center_axis',(1.,0.,0.));
#33904=DIRECTION('ref_axis',(0.,-0.977111001077189,0.212730090899086));
#33905=DIRECTION('center_axis',(-1.,0.,0.));
#33906=DIRECTION('ref_axis',(0.,-0.977111063757368,-0.212729802996537));
#33907=DIRECTION('center_axis',(1.,0.,0.));
#33908=DIRECTION('ref_axis',(0.,-0.540504506536072,0.84134111893702));
#33909=DIRECTION('center_axis',(-1.,0.,0.));
#33910=DIRECTION('ref_axis',(0.,-0.841344883607578,0.540498646462089));
#33911=DIRECTION('center_axis',(1.,0.,0.));
#33912=DIRECTION('ref_axis',(0.,0.212729805568991,0.977111063197311));
#33913=DIRECTION('center_axis',(-1.,0.,0.));
#33914=DIRECTION('ref_axis',(0.,-0.212725316405191,0.977112040535941));
#33915=DIRECTION('center_axis',(-1.,0.,0.));
#33916=DIRECTION('ref_axis',(0.,0.,1.));
#33917=DIRECTION('center_axis',(-1.,0.,0.));
#33918=DIRECTION('ref_axis',(0.,0.923879532497291,0.382683432398878));
#33919=DIRECTION('center_axis',(1.,0.,0.));
#33920=DIRECTION('ref_axis',(0.,-0.923879532497291,-0.382683432398878));
#33921=DIRECTION('center_axis',(-1.,0.,0.));
#33922=DIRECTION('ref_axis',(0.,-0.923879532497291,-0.382683432398878));
#33923=DIRECTION('',(-1.,0.,0.));
#33924=DIRECTION('center_axis',(-1.,0.,0.));
#33925=DIRECTION('ref_axis',(0.,0.,1.));
#33926=DIRECTION('center_axis',(-1.,0.,0.));
#33927=DIRECTION('ref_axis',(0.,-0.382683432398878,0.923879532497291));
#33928=DIRECTION('center_axis',(1.,0.,0.));
#33929=DIRECTION('ref_axis',(0.,0.382683432398878,-0.923879532497291));
#33930=DIRECTION('center_axis',(-1.,0.,0.));
#33931=DIRECTION('ref_axis',(0.,0.382683432398878,-0.923879532497291));
#33932=DIRECTION('',(-1.,0.,0.));
#33933=DIRECTION('center_axis',(-1.,0.,0.));
#33934=DIRECTION('ref_axis',(0.,0.,1.));
#33935=DIRECTION('center_axis',(-1.,0.,0.));
#33936=DIRECTION('ref_axis',(0.,-0.923879532497291,-0.382683432398878));
#33937=DIRECTION('center_axis',(1.,0.,0.));
#33938=DIRECTION('ref_axis',(0.,0.923879532497291,0.382683432398878));
#33939=DIRECTION('center_axis',(-1.,0.,0.));
#33940=DIRECTION('ref_axis',(0.,0.923879532497291,0.382683432398878));
#33941=DIRECTION('',(-1.,0.,0.));
#33942=DIRECTION('center_axis',(1.,0.,0.));
#33943=DIRECTION('ref_axis',(0.,1.,0.));
#33944=DIRECTION('center_axis',(-1.,0.,0.));
#33945=DIRECTION('ref_axis',(0.,-0.382683432398878,0.923879532497291));
#33946=DIRECTION('center_axis',(-1.,0.,0.));
#33947=DIRECTION('ref_axis',(0.,0.382683432398878,-0.923879532497291));
#33948=DIRECTION('center_axis',(1.,0.,0.));
#33949=DIRECTION('ref_axis',(0.,-0.382683432398878,0.923879532497291));
#33950=DIRECTION('',(-1.,0.,0.));
#33951=DIRECTION('center_axis',(-1.,0.,0.));
#33952=DIRECTION('ref_axis',(0.,0.,1.));
#33953=DIRECTION('center_axis',(-1.,0.,0.));
#33954=DIRECTION('ref_axis',(0.,0.382683432331302,0.923879532525282));
#33955=DIRECTION('center_axis',(1.,0.,0.));
#33956=DIRECTION('ref_axis',(0.,-0.382683432331302,-0.923879532525282));
#33957=DIRECTION('',(-1.,0.,0.));
#33958=DIRECTION('center_axis',(-1.,0.,0.));
#33959=DIRECTION('ref_axis',(0.,-0.382683432331302,-0.923879532525282));
#33960=DIRECTION('center_axis',(-1.,0.,0.));
#33961=DIRECTION('ref_axis',(0.,0.,1.));
#33962=DIRECTION('center_axis',(-1.,0.,0.));
#33963=DIRECTION('ref_axis',(0.,-0.923879532525282,0.382683432331302));
#33964=DIRECTION('center_axis',(1.,0.,0.));
#33965=DIRECTION('ref_axis',(0.,0.923879532525282,-0.382683432331302));
#33966=DIRECTION('',(-1.,0.,0.));
#33967=DIRECTION('center_axis',(-1.,0.,0.));
#33968=DIRECTION('ref_axis',(0.,0.923879532525282,-0.382683432331302));
#33969=DIRECTION('center_axis',(-1.,0.,0.));
#33970=DIRECTION('ref_axis',(0.,0.,1.));
#33971=DIRECTION('center_axis',(-1.,0.,0.));
#33972=DIRECTION('ref_axis',(0.,-0.382683432331302,-0.923879532525282));
#33973=DIRECTION('center_axis',(1.,0.,0.));
#33974=DIRECTION('ref_axis',(0.,0.382683432331302,0.923879532525282));
#33975=DIRECTION('',(-1.,0.,0.));
#33976=DIRECTION('center_axis',(-1.,0.,0.));
#33977=DIRECTION('ref_axis',(0.,0.382683432331302,0.923879532525282));
#33978=DIRECTION('center_axis',(1.,0.,0.));
#33979=DIRECTION('ref_axis',(0.,1.,0.));
#41230=CARTESIAN_POINT('',(0.,0.,0.));
#41231=CARTESIAN_POINT('Origin',(8.3,0.,0.));
#41232=CARTESIAN_POINT('',(8.3,-16.1678918191954,6.69696006579904));
#41233=CARTESIAN_POINT('Origin',(8.3,-18.015650884246,7.46232693046164));
#41234=CARTESIAN_POINT('Origin',(8.3,-18.015650884246,7.46232693046164));
#41235=CARTESIAN_POINT('',(7.,-16.1678918191954,6.69696006579904));
#41236=CARTESIAN_POINT('',(8.3,-16.1678918191954,6.69696006579904));
#41237=CARTESIAN_POINT('Origin',(7.,-18.015650884246,7.46232693046164));
#41238=CARTESIAN_POINT('Origin',(-8.3,0.,0.));
#41239=CARTESIAN_POINT('',(-8.3,-6.69696006698037,16.1678918187026));
#41240=CARTESIAN_POINT('Origin',(-8.3,-7.46232693177812,18.0156508836972));
#41241=CARTESIAN_POINT('Origin',(-7.,-7.46232693177812,18.0156508836972));
#41242=CARTESIAN_POINT('',(-7.,-6.69696006698037,16.1678918187026));
#41243=CARTESIAN_POINT('Origin',(-7.,-7.46232693177812,18.0156508836972));
#41244=CARTESIAN_POINT('',(-7.,-6.69696006698036,16.1678918187026));
#41245=CARTESIAN_POINT('Ctrl Pts',(7.10525808636416,14.3565635298793,7.16063659654178));
#41246=CARTESIAN_POINT('Ctrl Pts',(7.10575876444043,14.3387789637918,7.19592366196931));
#41247=CARTESIAN_POINT('Ctrl Pts',(7.10223937876377,14.2836777370554,7.30797308590476));
#41248=CARTESIAN_POINT('Ctrl Pts',(7.06770483392813,14.1927233116185,7.50815817028447));
#41249=CARTESIAN_POINT('Ctrl Pts',(6.97267785327267,14.0924356480638,7.75900571169227));
#41250=CARTESIAN_POINT('Ctrl Pts',(6.81702606252464,14.010417021847,8.00596596099621));
#41251=CARTESIAN_POINT('Ctrl Pts',(6.60785644388706,13.9583672553273,8.22304070094113));
#41252=CARTESIAN_POINT('Ctrl Pts',(6.40912170184387,13.9451967772279,8.35867896670148));
#41253=CARTESIAN_POINT('Ctrl Pts',(6.28621415412844,13.9496957605692,8.41828411660249));
#41254=CARTESIAN_POINT('Ctrl Pts',(6.24974104220345,13.9520455424819,8.43403152063555));
#41255=CARTESIAN_POINT('Ctrl Pts',(6.81652863846456,13.838553574665,6.9039568015009));
#41256=CARTESIAN_POINT('Ctrl Pts',(6.81697830810448,13.8228760451423,6.93504899056999));
#41257=CARTESIAN_POINT('Ctrl Pts',(6.81382002318898,13.7743041309446,7.03391985983529));
#41258=CARTESIAN_POINT('Ctrl Pts',(6.78271672624039,13.6942666755865,7.21111662303983));
#41259=CARTESIAN_POINT('Ctrl Pts',(6.69707233669569,13.606593950197,7.43348605086638));
#41260=CARTESIAN_POINT('Ctrl Pts',(6.5570604709967,13.5357964998358,7.6522164860747));
#41261=CARTESIAN_POINT('Ctrl Pts',(6.36965839370619,13.4919926525689,7.84392391935531));
#41262=CARTESIAN_POINT('Ctrl Pts',(6.19259577880842,13.4820718993109,7.96318830858491));
#41263=CARTESIAN_POINT('Ctrl Pts',(6.08364035524788,13.4867937044583,8.01543121257244));
#41264=CARTESIAN_POINT('Ctrl Pts',(6.05135731015642,13.4890581680742,8.02922278350448));
#41265=CARTESIAN_POINT('Ctrl Pts',(7.059396511537,13.3051669887233,6.63188003220261));
#41266=CARTESIAN_POINT('Ctrl Pts',(7.05998753389128,13.2848957072356,6.67210384463059));
#41267=CARTESIAN_POINT('Ctrl Pts',(7.05582531382928,13.2222257804441,6.79953300552684));
#41268=CARTESIAN_POINT('Ctrl Pts',(7.01532499205948,13.1191751284561,7.02616529659645));
#41269=CARTESIAN_POINT('Ctrl Pts',(6.90406234216587,13.0054588505149,7.31013013126185));
#41270=CARTESIAN_POINT('Ctrl Pts',(6.72098844767873,12.9119197076438,7.59124630672048));
#41271=CARTESIAN_POINT('Ctrl Pts',(6.47267893719941,12.8520752435282,7.8409976590492));
#41272=CARTESIAN_POINT('Ctrl Pts',(6.23373408548986,12.8370545490279,7.9994819202324));
#41273=CARTESIAN_POINT('Ctrl Pts',(6.08428318984346,12.8428248784391,8.07006964139502));
#41274=CARTESIAN_POINT('Ctrl Pts',(6.0397814795314,12.8457670018725,8.08880192603315));
#41275=CARTESIAN_POINT('Ctrl Pts',(7.66907949078917,13.1178290552721,6.52876987767165));
#41276=CARTESIAN_POINT('Ctrl Pts',(7.66990836900527,13.0893786582693,6.58525885810878));
#41277=CARTESIAN_POINT('Ctrl Pts',(7.66405799361575,13.001544514722,6.76361524924263));
#41278=CARTESIAN_POINT('Ctrl Pts',(7.60770496051459,12.8571579080423,7.07858023439957));
#41279=CARTESIAN_POINT('Ctrl Pts',(7.45319621673626,12.6964022703982,7.47244067179396));
#41280=CARTESIAN_POINT('Ctrl Pts',(7.19756079194026,12.5615820193213,7.86424907202288));
#41281=CARTESIAN_POINT('Ctrl Pts',(6.8469730169815,12.4722893095407,8.21609142295753));
#41282=CARTESIAN_POINT('Ctrl Pts',(6.5045565862393,12.4472780949918,8.44279153754262));
#41283=CARTESIAN_POINT('Ctrl Pts',(6.28762425993378,12.4542118419042,8.54499034275498));
#41284=CARTESIAN_POINT('Ctrl Pts',(6.22278112148675,12.4581351147872,8.57220928430822));
#41285=CARTESIAN_POINT('',(6.26385989006508,13.9442649556658,8.42071839528551));
#41286=CARTESIAN_POINT('',(6.24996405537491,12.462652577598,8.55168635783618));
#41287=CARTESIAN_POINT('Origin',(6.527841919986,13.2547471496042,9.09516599269981));
#41288=CARTESIAN_POINT('',(6.99999974236212,12.522062102245,8.04447864893747));
#41289=CARTESIAN_POINT('Ctrl Pts',(6.99999974236211,12.522062102245,8.04447864893747));
#41290=CARTESIAN_POINT('Ctrl Pts',(6.96024020545819,12.5123170532408,8.0837285342973));
#41291=CARTESIAN_POINT('Ctrl Pts',(6.91936977290025,12.503714608425,8.1213744417));
#41292=CARTESIAN_POINT('Ctrl Pts',(6.87744629964271,12.4962259287422,8.15746842834184));
#41293=CARTESIAN_POINT('Ctrl Pts',(6.86099027054929,12.4932864315786,8.17163623573287));
#41294=CARTESIAN_POINT('Ctrl Pts',(6.84437149112919,12.4905187525983,8.18556475250955));
#41295=CARTESIAN_POINT('Ctrl Pts',(6.82759161373763,12.4879220071344,8.19925635360236));
#41296=CARTESIAN_POINT('Ctrl Pts',(6.78468135220824,12.4812814921664,8.23426913527763));
#41297=CARTESIAN_POINT('Ctrl Pts',(6.74072035702834,12.475757087696,8.26773445620468));
#41298=CARTESIAN_POINT('Ctrl Pts',(6.69574230972554,12.4713366684958,8.29968211651214));
#41299=CARTESIAN_POINT('Ctrl Pts',(6.6800137959596,12.4697908783068,8.31085399357369));
#41300=CARTESIAN_POINT('Ctrl Pts',(6.66416056770558,12.4683803043908,8.32184004829003));
#41301=CARTESIAN_POINT('Ctrl Pts',(6.64818302246812,12.4671051370951,8.33264074697925));
#41302=CARTESIAN_POINT('Ctrl Pts',(6.60309229515852,12.4635064478127,8.36312173464732));
#41303=CARTESIAN_POINT('Ctrl Pts',(6.55702091386446,12.4609871974691,8.39212045625367));
#41304=CARTESIAN_POINT('Ctrl Pts',(6.50995241026026,12.4595681035583,8.41963042001002));
#41305=CARTESIAN_POINT('Ctrl Pts',(6.47702541470063,12.4585753696636,8.43887514599639));
#41306=CARTESIAN_POINT('Ctrl Pts',(6.44360979526878,12.4581215517176,8.45739066466166));
#41307=CARTESIAN_POINT('Ctrl Pts',(6.40969282388381,12.4582216998138,8.47516391515914));
#41308=CARTESIAN_POINT('Ctrl Pts',(6.36201368421857,12.4583624840547,8.50014884919573));
#41309=CARTESIAN_POINT('Ctrl Pts',(6.31334405099426,12.4595968496478,8.52366882448567));
#41310=CARTESIAN_POINT('Ctrl Pts',(6.26366968657578,12.4619696814476,8.54566654336259));
#41311=CARTESIAN_POINT('Ctrl Pts',(6.25912282970996,12.4621868744945,8.54768006643991));
#41312=CARTESIAN_POINT('Ctrl Pts',(6.2545675471324,12.4624136250554,8.54968080571952));
#41313=CARTESIAN_POINT('Ctrl Pts',(6.25000382373019,12.4626499791555,8.55166869888726));
#41314=CARTESIAN_POINT('',(6.99999606125493,13.9487024276541,6.97712715716362));
#41315=CARTESIAN_POINT('Ctrl Pts',(6.99999606125493,13.9487024276541,6.97712715716362));
#41316=CARTESIAN_POINT('Ctrl Pts',(6.99999606606441,13.9358724268105,6.98267129810995));
#41317=CARTESIAN_POINT('Ctrl Pts',(7.00000000000004,13.9229986563094,6.9881153971666));
#41318=CARTESIAN_POINT('Ctrl Pts',(7.00000000000004,13.6749072302415,7.09781423197374));
#41319=CARTESIAN_POINT('Ctrl Pts',(7.,13.4053213379188,7.2183592608038));
#41320=CARTESIAN_POINT('Ctrl Pts',(7.,12.7992520694899,7.66953465501947));
#41321=CARTESIAN_POINT('Ctrl Pts',(7.,12.6300164231238,7.87643705196837));
#41322=CARTESIAN_POINT('Ctrl Pts',(7.,12.5220620628349,8.04447855424198));
#41323=CARTESIAN_POINT('Ctrl Pts',(6.99999606140003,13.9486969304546,6.97712309905536));
#41324=CARTESIAN_POINT('Ctrl Pts',(6.99999536779159,13.9433045112521,7.01221037447256));
#41325=CARTESIAN_POINT('Ctrl Pts',(6.99896236212046,13.9382287844098,7.04671544578038));
#41326=CARTESIAN_POINT('Ctrl Pts',(6.99701513979328,13.9334693017443,7.08055243275489));
#41327=CARTESIAN_POINT('Ctrl Pts',(6.99449897394573,13.9273191834102,7.12427598184388));
#41328=CARTESIAN_POINT('Ctrl Pts',(6.9904577666072,13.9216970366755,7.16688325413103));
#41329=CARTESIAN_POINT('Ctrl Pts',(6.98515768913276,13.9165800087812,7.20824924966308));
#41330=CARTESIAN_POINT('Ctrl Pts',(6.97960905378658,13.9112230074962,7.25155518736795));
#41331=CARTESIAN_POINT('Ctrl Pts',(6.97268032573301,13.9064197080891,7.29350069158915));
#41332=CARTESIAN_POINT('Ctrl Pts',(6.96463852783938,13.9021395728506,7.33398304499541));
#41333=CARTESIAN_POINT('Ctrl Pts',(6.96415125729609,13.9018802298715,7.33643596144504));
#41334=CARTESIAN_POINT('Ctrl Pts',(6.96365989003301,13.9016228061328,7.3388835179058));
#41335=CARTESIAN_POINT('Ctrl Pts',(6.96316448163874,13.9013672942434,7.34132569605035));
#41336=CARTESIAN_POINT('Ctrl Pts',(6.95799163377406,13.8986993456442,7.36682590183251));
#41337=CARTESIAN_POINT('Ctrl Pts',(6.95237869952793,13.8962398510606,7.39173933731414));
#41338=CARTESIAN_POINT('Ctrl Pts',(6.9463938451743,13.8939765412023,7.41605279480567));
#41339=CARTESIAN_POINT('Ctrl Pts',(6.93615532258882,13.8901046091998,7.45764677002194));
#41340=CARTESIAN_POINT('Ctrl Pts',(6.92483052998138,13.8868069446777,7.49748294940497));
#41341=CARTESIAN_POINT('Ctrl Pts',(6.91272362793161,13.8840207080244,7.53552531468417));
#41342=CARTESIAN_POINT('Ctrl Pts',(6.90315152938264,13.881817821463,7.56560280833131));
#41343=CARTESIAN_POINT('Ctrl Pts',(6.89308951924174,13.8799346003301,7.59455980286787));
#41344=CARTESIAN_POINT('Ctrl Pts',(6.8826706408791,13.8783389004979,7.62239342398978));
#41345=CARTESIAN_POINT('Ctrl Pts',(6.87533228532583,13.8772149971066,7.64199755036675));
#41346=CARTESIAN_POINT('Ctrl Pts',(6.86781666408516,13.8762336651835,7.66104471293685));
#41347=CARTESIAN_POINT('Ctrl Pts',(6.86017007183178,13.8753814225812,7.67953970156442));
#41348=CARTESIAN_POINT('Ctrl Pts',(6.85479764883003,13.8747826450332,7.69253410469556));
#41349=CARTESIAN_POINT('Ctrl Pts',(6.84936048743326,13.8742475952939,7.70525598262344));
#41350=CARTESIAN_POINT('Ctrl Pts',(6.84387352152024,13.873771654449,7.71770759717752));
#41351=CARTESIAN_POINT('Ctrl Pts',(6.84113003856374,13.8735336840265,7.72393340445457));
#41352=CARTESIAN_POINT('Ctrl Pts',(6.83837409665091,13.8733104945881,7.73009164254231));
#41353=CARTESIAN_POINT('Ctrl Pts',(6.83560747470963,13.8731015090751,7.73618264957294));
#41354=CARTESIAN_POINT('Ctrl Pts',(6.834224163739,13.8729970163186,7.73922815308825));
#41355=CARTESIAN_POINT('Ctrl Pts',(6.83283818228316,13.872896074765,7.74225684864267));
#41356=CARTESIAN_POINT('Ctrl Pts',(6.83144974880931,13.8727986130004,7.74526877931514));
#41357=CARTESIAN_POINT('Ctrl Pts',(6.83037192053051,13.872722954319,7.74760691370453));
#41358=CARTESIAN_POINT('Ctrl Pts',(6.82975121547303,13.8726804790969,7.74894835834072));
#41359=CARTESIAN_POINT('Ctrl Pts',(6.82852034694564,13.8725984441275,7.75159111902282));
#41360=CARTESIAN_POINT('Ctrl Pts',(6.8281656390886,13.8725748035456,7.75235270156179));
#41361=CARTESIAN_POINT('Ctrl Pts',(6.82776004912312,13.8725479813548,7.75322223757905));
#41362=CARTESIAN_POINT('Ctrl Pts',(6.82727730836574,13.8725165961712,7.75425432019889));
#41363=CARTESIAN_POINT('Ctrl Pts',(6.8030109284669,13.8709389278715,7.80613497986339));
#41364=CARTESIAN_POINT('Ctrl Pts',(6.7766335741503,13.8703548649644,7.85606962617251));
#41365=CARTESIAN_POINT('Ctrl Pts',(6.7484292363882,13.8708003188642,7.90384512223861));
#41366=CARTESIAN_POINT('Ctrl Pts',(6.7167315359438,13.8713009462639,7.95753804620159));
#41367=CARTESIAN_POINT('Ctrl Pts',(6.68272740983891,13.8731013428253,8.00850413011352));
#41368=CARTESIAN_POINT('Ctrl Pts',(6.64688040419033,13.8761972878495,8.05653888670308));
#41369=CARTESIAN_POINT('Ctrl Pts',(6.62069061176507,13.8784591827018,8.09163303979949));
#41370=CARTESIAN_POINT('Ctrl Pts',(6.5935158735721,13.8814130955261,8.12516272712827));
#41371=CARTESIAN_POINT('Ctrl Pts',(6.56552118186522,13.8850622912798,8.15705338823882));
#41372=CARTESIAN_POINT('Ctrl Pts',(6.5257680754455,13.8902442332231,8.2023388608633));
#41373=CARTESIAN_POINT('Ctrl Pts',(6.48436398694375,13.8968272260797,8.24431925736261));
#41374=CARTESIAN_POINT('Ctrl Pts',(6.4418307408238,13.9047546569829,8.28288850294924));
#41375=CARTESIAN_POINT('Ctrl Pts',(6.41084892356005,13.9105291096292,8.31098288623228));
#41376=CARTESIAN_POINT('Ctrl Pts',(6.37926681377584,13.9170173724247,8.33726749311037));
#41377=CARTESIAN_POINT('Ctrl Pts',(6.3472701253487,13.9242018519261,8.36170618883195));
#41378=CARTESIAN_POINT('Ctrl Pts',(6.31974251564985,13.9303828524397,8.38273145458419));
#41379=CARTESIAN_POINT('Ctrl Pts',(6.29190792468545,13.9370791086268,8.40239070177926));
#41380=CARTESIAN_POINT('Ctrl Pts',(6.26389359063877,13.9442618466046,8.42068885095676));
#41381=CARTESIAN_POINT('Ctrl Pts',(6.99933866930047,24.2330493761347,10.8743218589222));
#41382=CARTESIAN_POINT('Ctrl Pts',(6.99933866930047,24.1955798268354,10.8803485939721));
#41383=CARTESIAN_POINT('Ctrl Pts',(6.99933866930047,23.5851360656717,10.9752954456166));
#41384=CARTESIAN_POINT('Ctrl Pts',(6.99933866930047,22.3847716450475,11.0599202839285));
#41385=CARTESIAN_POINT('Ctrl Pts',(6.99933866930047,20.6450523072803,10.9047326082907));
#41386=CARTESIAN_POINT('Ctrl Pts',(6.99933866930047,18.949091407574,10.4757482566013));
#41387=CARTESIAN_POINT('Ctrl Pts',(6.99933866930047,17.3424628342019,9.78232775497157));
#41388=CARTESIAN_POINT('Ctrl Pts',(6.99933866930047,15.866963491147,8.84436513563102));
#41389=CARTESIAN_POINT('Ctrl Pts',(6.99933866930047,14.7344858431782,7.8388947861151));
#41390=CARTESIAN_POINT('Ctrl Pts',(6.99933866930047,14.1224303484372,7.13859345335349));
#41391=CARTESIAN_POINT('Ctrl Pts',(6.99933866930047,13.9057057558426,6.86526372126548));
#41392=CARTESIAN_POINT('Ctrl Pts',(7.01706607775066,24.3104707875623,11.3553300652331));
#41393=CARTESIAN_POINT('Ctrl Pts',(7.01706607775066,24.2713372052229,11.3616240778769));
#41394=CARTESIAN_POINT('Ctrl Pts',(7.01706607775066,23.6337964680017,11.4607818239098));
#41395=CARTESIAN_POINT('Ctrl Pts',(7.01706607775066,22.3805053518595,11.5491624475826));
#41396=CARTESIAN_POINT('Ctrl Pts',(7.01706607775066,20.5628206844035,11.3870392019886));
#41397=CARTESIAN_POINT('Ctrl Pts',(7.01706607775066,18.7918025555526,10.9390217567355));
#41398=CARTESIAN_POINT('Ctrl Pts',(7.01706607775066,17.1135755732343,10.2147680382133));
#41399=CARTESIAN_POINT('Ctrl Pts',(7.01706607775066,15.5722878143257,9.23492874463336));
#41400=CARTESIAN_POINT('Ctrl Pts',(7.01706607775066,14.3895391493755,8.18482486590383));
#41401=CARTESIAN_POINT('Ctrl Pts',(7.01706607775066,13.7503337411648,7.45348156383166));
#41402=CARTESIAN_POINT('Ctrl Pts',(7.01706607775066,13.5239371293929,7.16794926614792));
#41403=CARTESIAN_POINT('Ctrl Pts',(6.72659992294722,24.3728605839284,11.7429489873457));
#41404=CARTESIAN_POINT('Ctrl Pts',(6.72659992294722,24.3323860458921,11.749458384781));
#41405=CARTESIAN_POINT('Ctrl Pts',(6.72659992294722,23.6730092973298,11.8520094665702));
#41406=CARTESIAN_POINT('Ctrl Pts',(6.72659992294722,22.377067373154,11.9434166778419));
#41407=CARTESIAN_POINT('Ctrl Pts',(6.72659992294722,20.4965545945406,11.7757044254197));
#41408=CARTESIAN_POINT('Ctrl Pts',(6.72659992294722,18.6650518380346,11.3123492226921));
#41409=CARTESIAN_POINT('Ctrl Pts',(6.72659992294722,16.9291275072387,10.563248655114));
#41410=CARTESIAN_POINT('Ctrl Pts',(6.72659992294722,15.3348243641778,9.54966317775517));
#41411=CARTESIAN_POINT('Ctrl Pts',(6.72659992294722,14.111564961231,8.46359151249178));
#41412=CARTESIAN_POINT('Ctrl Pts',(6.72659992294722,13.4504808822296,7.70723313889616));
#41413=CARTESIAN_POINT('Ctrl Pts',(6.72659992294722,13.2162901047889,7.41186744281947));
#41414=CARTESIAN_POINT('Ctrl Pts',(6.25333238742997,24.3925555985452,11.8653113090695));
#41415=CARTESIAN_POINT('Ctrl Pts',(6.25333238742997,24.3516577518376,11.8718886985001));
#41416=CARTESIAN_POINT('Ctrl Pts',(6.25333238742997,23.6853878799162,11.9755109778418));
#41417=CARTESIAN_POINT('Ctrl Pts',(6.25333238742997,22.3759820828512,12.0678736127627));
#41418=CARTESIAN_POINT('Ctrl Pts',(6.25333238742997,20.4756359237962,11.8983970402517));
#41419=CARTESIAN_POINT('Ctrl Pts',(6.25333238742997,18.6250395703447,11.4302000625049));
#41420=CARTESIAN_POINT('Ctrl Pts',(6.25333238742997,16.8709015221175,10.6732559197938));
#41421=CARTESIAN_POINT('Ctrl Pts',(6.25333238742997,15.2598626493954,9.64901755331904));
#41422=CARTESIAN_POINT('Ctrl Pts',(6.25333238742997,14.0238149441382,8.55159169037091));
#41423=CARTESIAN_POINT('Ctrl Pts',(6.25333238742997,13.3558242751811,7.78733663770481));
#41424=CARTESIAN_POINT('Ctrl Pts',(6.25333238742997,13.1191730600493,7.48886676536423));
#41425=CARTESIAN_POINT('',(7.,24.1259420764688,10.92778018982));
#41426=CARTESIAN_POINT('Ctrl Pts',(7.00000000000002,24.1259420781411,10.9277802009508));
#41427=CARTESIAN_POINT('Ctrl Pts',(7.00000000000002,23.9636071437087,10.9521697339675));
#41428=CARTESIAN_POINT('Ctrl Pts',(7.00000000006073,23.8012468343643,10.9728907888933));
#41429=CARTESIAN_POINT('Ctrl Pts',(6.99999999867344,23.6387645225613,10.989991664534));
#41430=CARTESIAN_POINT('Ctrl Pts',(6.99999999728331,23.4759486337289,11.0071276483612));
#41431=CARTESIAN_POINT('Ctrl Pts',(6.99999999422997,23.3130097833915,11.0206285917113));
#41432=CARTESIAN_POINT('Ctrl Pts',(6.99999999314808,23.1498443962042,11.0304911374634));
#41433=CARTESIAN_POINT('Ctrl Pts',(6.99999999207001,22.987253229421,11.0403189744142));
#41434=CARTESIAN_POINT('Ctrl Pts',(6.9999999947222,22.8244366655206,11.0465339774628));
#41435=CARTESIAN_POINT('Ctrl Pts',(6.99999999803543,22.6612927248816,11.0490812228026));
#41436=CARTESIAN_POINT('Ctrl Pts',(6.99999999907234,22.6102348488692,11.0498784141431));
#41437=CARTESIAN_POINT('Ctrl Pts',(7.00000000000002,22.5591449386156,11.0503159845158));
#41438=CARTESIAN_POINT('Ctrl Pts',(7.00000000000002,22.5080199866575,11.0503912040686));
#41439=CARTESIAN_POINT('Ctrl Pts',(7.00000000000002,22.4670944974344,11.0504514172694));
#41440=CARTESIAN_POINT('Ctrl Pts',(6.99999999938402,22.4261461216709,11.0502844809917));
#41441=CARTESIAN_POINT('Ctrl Pts',(6.9999999984721,22.3851800827051,11.04988913167));
#41442=CARTESIAN_POINT('Ctrl Pts',(6.99999999416127,22.1915272268588,11.0480202537617));
#41443=CARTESIAN_POINT('Ctrl Pts',(6.99999998574681,21.9974791816599,11.0410431158288));
#41444=CARTESIAN_POINT('Ctrl Pts',(6.99999998500532,21.8035299183916,11.0289289304663));
#41445=CARTESIAN_POINT('Ctrl Pts',(6.99999998426226,21.6091706679596,11.0167891370638));
#41446=CARTESIAN_POINT('Ctrl Pts',(6.99999998984224,21.4149110357627,10.9994905471205));
#41447=CARTESIAN_POINT('Ctrl Pts',(6.99999999473001,21.221250784181,10.9770564362198));
#41448=CARTESIAN_POINT('Ctrl Pts',(6.99999999759809,21.1076129763808,10.9638923348521));
#41449=CARTESIAN_POINT('Ctrl Pts',(7.00000000000002,20.9941815671557,10.9489609450939));
#41450=CARTESIAN_POINT('Ctrl Pts',(7.00000000000002,20.881057063376,10.932275312452));
#41451=CARTESIAN_POINT('Ctrl Pts',(7.00000000000002,20.8030386971055,10.9207677631995));
#41452=CARTESIAN_POINT('Ctrl Pts',(6.99999999890227,20.7251678797296,10.9084197072691));
#41453=CARTESIAN_POINT('Ctrl Pts',(6.99999999758225,20.6474551518283,10.8952337790289));
#41454=CARTESIAN_POINT('Ctrl Pts',(6.99999999346296,20.4049430664632,10.8540854749948));
#41455=CARTESIAN_POINT('Ctrl Pts',(6.9999999892588,20.1639700234044,10.8047816167284));
#41456=CARTESIAN_POINT('Ctrl Pts',(6.99999999152161,19.9249049441579,10.7474302395335));
#41457=CARTESIAN_POINT('Ctrl Pts',(6.99999999354309,19.7113353073924,10.6961951832294));
#41458=CARTESIAN_POINT('Ctrl Pts',(7.00000000000002,19.499288118559,10.6385367924637));
#41459=CARTESIAN_POINT('Ctrl Pts',(7.00000000000002,19.2890338727372,10.5744977121983));
#41460=CARTESIAN_POINT('Ctrl Pts',(7.00000000000002,19.1765541929259,10.5402387358075));
#41461=CARTESIAN_POINT('Ctrl Pts',(6.99999999803037,19.0645809749219,10.5041682245751));
#41462=CARTESIAN_POINT('Ctrl Pts',(6.99999999636324,18.9531931449385,10.4663010056192));
#41463=CARTESIAN_POINT('Ctrl Pts',(6.99999999271541,18.709465928779,10.3834439119742));
#41464=CARTESIAN_POINT('Ctrl Pts',(6.99999999204987,18.4685424549483,10.2919812981329));
#41465=CARTESIAN_POINT('Ctrl Pts',(6.99999999506635,18.2311664503793,10.19223200664));
#41466=CARTESIAN_POINT('Ctrl Pts',(6.99999999705716,18.0745037563495,10.1263997724123));
#41467=CARTESIAN_POINT('Ctrl Pts',(7.00000000000002,17.9193859910228,10.056959169959));
#41468=CARTESIAN_POINT('Ctrl Pts',(7.00000000000002,17.7660225335621,9.9840134765408));
#41469=CARTESIAN_POINT('Ctrl Pts',(7.00000000000002,17.6246298314655,9.91676154528239));
#41470=CARTESIAN_POINT('Ctrl Pts',(6.99999999722481,17.4847359912375,9.84651984572386));
#41471=CARTESIAN_POINT('Ctrl Pts',(6.99999999446473,17.3464266497251,9.77332726001044));
#41472=CARTESIAN_POINT('Ctrl Pts',(6.9999999900828,17.1268453052524,9.6571259521259));
#41473=CARTESIAN_POINT('Ctrl Pts',(6.99999998784248,16.9112559387415,9.53348886601782));
#41474=CARTESIAN_POINT('Ctrl Pts',(6.99999999262692,16.7000168930179,9.40257873636276));
#41475=CARTESIAN_POINT('Ctrl Pts',(6.99999999531398,16.58137961056,9.32905623972729));
#41476=CARTESIAN_POINT('Ctrl Pts',(7.00000000000002,16.4641150846931,9.25323890923894));
#41477=CARTESIAN_POINT('Ctrl Pts',(7.00000000000002,16.3482916764188,9.17515025230581));
#41478=CARTESIAN_POINT('Ctrl Pts',(7.00000000000002,16.1866097165453,9.06614355594835));
#41479=CARTESIAN_POINT('Ctrl Pts',(6.9999999901482,16.0276912247442,8.9527563196008));
#41480=CARTESIAN_POINT('Ctrl Pts',(6.99999998525263,15.8719358528285,8.83523144981877));
#41481=CARTESIAN_POINT('Ctrl Pts',(6.99999998003391,15.7058991336856,8.70994881233221));
#41482=CARTESIAN_POINT('Ctrl Pts',(6.99999998145009,15.5434575723926,8.5799641511856));
#41483=CARTESIAN_POINT('Ctrl Pts',(6.99999998835947,15.3849965664812,8.44567633217485));
#41484=CARTESIAN_POINT('Ctrl Pts',(6.99999999308645,15.2765870454925,8.35380465655442));
#41485=CARTESIAN_POINT('Ctrl Pts',(7.00000000000002,15.170039918213,8.25991974581256));
#41486=CARTESIAN_POINT('Ctrl Pts',(7.00000000000002,15.0654684156701,8.1641590081593));
#41487=CARTESIAN_POINT('Ctrl Pts',(7.00000000000002,14.9424780843168,8.05153133648764));
#41488=CARTESIAN_POINT('Ctrl Pts',(6.99999999283352,14.822282594585,7.9362684620195));
#41489=CARTESIAN_POINT('Ctrl Pts',(6.99999999157257,14.7047659435611,7.81832386853829));
#41490=CARTESIAN_POINT('Ctrl Pts',(6.99999999107894,14.6587611849019,7.77215158136899));
#41491=CARTESIAN_POINT('Ctrl Pts',(6.99999999110871,14.6131673062471,7.72556786584807));
#41492=CARTESIAN_POINT('Ctrl Pts',(6.99999999149981,14.5679787260292,7.67856824982574));
#41493=CARTESIAN_POINT('Ctrl Pts',(6.99999999249457,14.453039403995,7.55902247132562));
#41494=CARTESIAN_POINT('Ctrl Pts',(6.99999999551026,14.3407195515746,7.43678843307566));
#41495=CARTESIAN_POINT('Ctrl Pts',(6.99999999717045,14.2309770599541,7.31179318524976));
#41496=CARTESIAN_POINT('Ctrl Pts',(6.99999999862373,14.1349114849696,7.2023757647465));
#41497=CARTESIAN_POINT('Ctrl Pts',(6.99999999923215,14.0408212492114,7.09084181894597));
#41498=CARTESIAN_POINT('Ctrl Pts',(6.99999999922773,13.9487034978523,6.97712164368536));
#41499=CARTESIAN_POINT('',(6.27159471697284,24.2690139179361,11.8794981306053));
#41500=CARTESIAN_POINT('Origin',(5.999999877385,24.1259420367213,10.9277801432448));
#41501=CARTESIAN_POINT('Ctrl Pts',(6.27159470457053,24.26901364136,11.8794980693503));
#41502=CARTESIAN_POINT('Ctrl Pts',(6.2719396690107,24.039518107917,11.9138782735934));
#41503=CARTESIAN_POINT('Ctrl Pts',(6.27225782568409,23.8113319140033,11.941274195107));
#41504=CARTESIAN_POINT('Ctrl Pts',(6.27254917030223,23.5849163742437,11.9620370266173));
#41505=CARTESIAN_POINT('Ctrl Pts',(6.27284515820514,23.3548923524162,11.9831307643245));
#41506=CARTESIAN_POINT('Ctrl Pts',(6.27311347261641,23.1266958261604,11.9973783297609));
#41507=CARTESIAN_POINT('Ctrl Pts',(6.27335410997358,22.9007562998605,12.0051465943053));
#41508=CARTESIAN_POINT('Ctrl Pts',(6.27354178810334,22.7245413171485,12.0112052270059));
#41509=CARTESIAN_POINT('Ctrl Pts',(6.27371263094327,22.5496981016224,12.0133226279267));
#41510=CARTESIAN_POINT('Ctrl Pts',(6.2738666371627,22.3764084710344,12.0116720903062));
#41511=CARTESIAN_POINT('Ctrl Pts',(6.2740686874815,22.1490590481532,12.009506647549));
#41512=CARTESIAN_POINT('Ctrl Pts',(6.27424175783396,21.9243852735233,12.0008569230838));
#41513=CARTESIAN_POINT('Ctrl Pts',(6.27438584596713,21.7027333503043,11.9862082337932));
#41514=CARTESIAN_POINT('Ctrl Pts',(6.27447251904989,21.5694034565529,11.9773966333418));
#41515=CARTESIAN_POINT('Ctrl Pts',(6.27454870533157,21.4371659929971,11.9664140729929));
#41516=CARTESIAN_POINT('Ctrl Pts',(6.27461440446078,21.3060877225297,11.9533633529954));
#41517=CARTESIAN_POINT('Ctrl Pts',(6.27472591349752,21.0836127544107,11.931212782157));
#41518=CARTESIAN_POINT('Ctrl Pts',(6.27480721195824,20.8644797540508,11.903105353766));
#41519=CARTESIAN_POINT('Ctrl Pts',(6.27485829878145,20.6489747471807,11.8695299304313));
#41520=CARTESIAN_POINT('Ctrl Pts',(6.27487121247856,20.5944995183722,11.8610427546804));
#41521=CARTESIAN_POINT('Ctrl Pts',(6.27488219573365,20.5402558626649,11.8522061026172));
#41522=CARTESIAN_POINT('Ctrl Pts',(6.27489124853762,20.4862479066121,11.8430276976365));
#41523=CARTESIAN_POINT('Ctrl Pts',(6.274928126599,20.2662377612205,11.8056379802344));
#41524=CARTESIAN_POINT('Ctrl Pts',(6.27493296929566,20.0501427221489,11.7625788981377));
#41525=CARTESIAN_POINT('Ctrl Pts',(6.2749057765612,19.8381869495583,11.7143943058079));
#41526=CARTESIAN_POINT('Ctrl Pts',(6.2748825774797,19.6573599992307,11.6732863294727));
#41527=CARTESIAN_POINT('Ctrl Pts',(6.27483606174957,19.4795448826768,11.6284473784717));
#41528=CARTESIAN_POINT('Ctrl Pts',(6.27476622983678,19.3048541889533,11.5802014292858));
#41529=CARTESIAN_POINT('Ctrl Pts',(6.27472435185361,19.2000927175969,11.5512684820523));
#41530=CARTESIAN_POINT('Ctrl Pts',(6.27467408860072,19.0964544407097,11.5211100139507));
#41531=CARTESIAN_POINT('Ctrl Pts',(6.27461544159147,18.9939596224219,11.4897937642906));
#41532=CARTESIAN_POINT('Ctrl Pts',(6.27458611808684,18.942712213278,11.4741356394605));
#41533=CARTESIAN_POINT('Ctrl Pts',(6.27455469601115,18.89175067152,11.4581880604393));
#41534=CARTESIAN_POINT('Ctrl Pts',(6.27452117880938,18.8410772027574,11.4419593294567));
#41535=CARTESIAN_POINT('Ctrl Pts',(6.27450442020849,18.8157404683761,11.4338449639654));
#41536=CARTESIAN_POINT('Ctrl Pts',(6.27448713764832,18.7904757524208,11.4256603098872));
#41537=CARTESIAN_POINT('Ctrl Pts',(6.27446933112943,18.7652833218196,11.4174063983605));
#41538=CARTESIAN_POINT('Ctrl Pts',(6.27445391930054,18.743478867389,11.4102625049979));
#41539=CARTESIAN_POINT('Ctrl Pts',(6.27443872964694,18.7225457056324,11.403338948886));
#41540=CARTESIAN_POINT('Ctrl Pts',(6.27442216592055,18.7003621707754,11.3959298239849));
#41541=CARTESIAN_POINT('Ctrl Pts',(6.27441959224871,18.6969152930875,11.3947785941438));
#41542=CARTESIAN_POINT('Ctrl Pts',(6.27441698540273,18.6934382597025,11.3936155447334));
#41543=CARTESIAN_POINT('Ctrl Pts',(6.27441433939461,18.6899231479741,11.3924379185985));
#41544=CARTESIAN_POINT('Ctrl Pts',(6.27440279742353,18.6745901195145,11.3873010761774));
#41545=CARTESIAN_POINT('Ctrl Pts',(6.27439106562786,18.6592579780417,11.382129846888));
#41546=CARTESIAN_POINT('Ctrl Pts',(6.27437914400858,18.6439268888218,11.3769241436729));
#41547=CARTESIAN_POINT('Ctrl Pts',(6.27420011122339,18.4136924266768,11.2987475534373));
#41548=CARTESIAN_POINT('Ctrl Pts',(6.27397826832473,18.1836911572812,11.2127950683308));
#41549=CARTESIAN_POINT('Ctrl Pts',(6.27371361959025,17.9544926702115,11.1188688297047));
#41550=CARTESIAN_POINT('Ctrl Pts',(6.27345239281417,17.7282577631024,11.0261570751799));
#41551=CARTESIAN_POINT('Ctrl Pts',(6.27314946001023,17.5028049754159,10.925676404779));
#41552=CARTESIAN_POINT('Ctrl Pts',(6.27280482713072,17.2787307745671,10.8172504627899));
#41553=CARTESIAN_POINT('Ctrl Pts',(6.27260798324538,17.1507463629782,10.7553208415578));
#41554=CARTESIAN_POINT('Ctrl Pts',(6.27239753537388,17.0232125920257,10.6907994538667));
#41555=CARTESIAN_POINT('Ctrl Pts',(6.27217348492361,16.8962479574614,10.6236555852893));
#41556=CARTESIAN_POINT('Ctrl Pts',(6.27177013690949,16.6676791991513,10.5027794789503));
#41557=CARTESIAN_POINT('Ctrl Pts',(6.27132270387729,16.4409516512944,10.3734026114263));
#41558=CARTESIAN_POINT('Ctrl Pts',(6.2708311960293,16.2167886981205,10.2354141987361));
#41559=CARTESIAN_POINT('Ctrl Pts',(6.27036732517286,16.0052302021626,10.1051847355933));
#41560=CARTESIAN_POINT('Ctrl Pts',(6.26986419786731,15.7959563703179,9.96728507323921));
#41561=CARTESIAN_POINT('Ctrl Pts',(6.26932182415434,15.5896233810682,9.82164183491594));
#41562=CARTESIAN_POINT('Ctrl Pts',(6.26905884857566,15.4895806689094,9.75102518450816));
#41563=CARTESIAN_POINT('Ctrl Pts',(6.26878664660819,15.3902300307254,9.67858839365913));
#41564=CARTESIAN_POINT('Ctrl Pts',(6.26850521961789,15.2916503517775,9.60432480011758));
#41565=CARTESIAN_POINT('Ctrl Pts',(6.26791729668106,15.0857097122666,9.44918235991527));
#41566=CARTESIAN_POINT('Ctrl Pts',(6.26728911325593,14.8831313073574,9.28606507446861));
#41567=CARTESIAN_POINT('Ctrl Pts',(6.26662068408126,14.684548134728,9.11502581381811));
#41568=CARTESIAN_POINT('Ctrl Pts',(6.26595956673244,14.488137227508,8.94585752070546));
#41569=CARTESIAN_POINT('Ctrl Pts',(6.2652590792745,14.2956345992665,8.76893957558176));
#41570=CARTESIAN_POINT('Ctrl Pts',(6.2645192393273,14.1076929658034,8.5843545277584));
#41571=CARTESIAN_POINT('Ctrl Pts',(6.26430323424039,14.0528211668106,8.53046272393284));
#41572=CARTESIAN_POINT('Ctrl Pts',(6.26408387470152,13.9983384205356,8.47591757105517));
#41573=CARTESIAN_POINT('Ctrl Pts',(6.26386116120914,13.9442616338432,8.42072164456287));
#41574=CARTESIAN_POINT('Ctrl Pts',(6.99999999998952,24.7867299441601,9.33248386901283));
#41575=CARTESIAN_POINT('Ctrl Pts',(6.99999999998952,24.7867268023266,9.33249195739188));
#41576=CARTESIAN_POINT('Ctrl Pts',(6.99999999998952,24.68190835415,9.60233773525705));
#41577=CARTESIAN_POINT('Ctrl Pts',(6.99999999998952,24.4674877122422,10.1365860426111));
#41578=CARTESIAN_POINT('Ctrl Pts',(6.99999999998952,24.2412750070288,10.6659267308771));
#41579=CARTESIAN_POINT('Ctrl Pts',(6.99999999998952,24.1259369154038,10.9277807259288));
#41580=CARTESIAN_POINT('Ctrl Pts',(7.00000270566332,25.3377021368914,9.54650237055708));
#41581=CARTESIAN_POINT('Ctrl Pts',(7.00000270566332,25.33769894728,9.5465105819364));
#41582=CARTESIAN_POINT('Ctrl Pts',(7.00000270566332,25.2312865215935,9.8204599139257));
#41583=CARTESIAN_POINT('Ctrl Pts',(7.00000270566332,25.0136084416684,10.362824287923));
#41584=CARTESIAN_POINT('Ctrl Pts',(7.00000270566332,24.7839592082931,10.9002066230296));
#41585=CARTESIAN_POINT('Ctrl Pts',(7.00000270566332,24.6668671666914,11.1660426394581));
#41586=CARTESIAN_POINT('Ctrl Pts',(6.57967197777962,25.725143338898,9.69699923153085));
#41587=CARTESIAN_POINT('Ctrl Pts',(6.57967197777962,25.7251401156893,9.69700752940341));
#41588=CARTESIAN_POINT('Ctrl Pts',(6.57967197777962,25.617606812089,9.97384246245126));
#41589=CARTESIAN_POINT('Ctrl Pts',(6.57967197777962,25.3976381162041,10.5219140185141));
#41590=CARTESIAN_POINT('Ctrl Pts',(6.57967197777962,25.1655723314695,11.0649512040096));
#41591=CARTESIAN_POINT('Ctrl Pts',(6.57967197777962,25.0472469200172,11.3335873602045));
#41592=CARTESIAN_POINT('Ctrl Pts',(5.98852435812819,25.7188194279223,9.69454278460176));
#41593=CARTESIAN_POINT('Ctrl Pts',(5.98852435812819,25.718816205262,9.69455108106255));
#41594=CARTESIAN_POINT('Ctrl Pts',(5.98852435812819,25.6113011969081,9.97133891461738));
#41595=CARTESIAN_POINT('Ctrl Pts',(5.98852435812819,25.3913698890145,10.5193173166418));
#41596=CARTESIAN_POINT('Ctrl Pts',(5.98852435812819,25.1593435478338,11.0622622022752));
#41597=CARTESIAN_POINT('Ctrl Pts',(5.98852435812819,25.0410382677488,11.3308526538974));
#41598=CARTESIAN_POINT('',(6.99999999994009,24.7867180661821,9.33250873276066));
#41599=CARTESIAN_POINT('',(5.98852583812743,25.7188097531253,9.69456766830281));
#41600=CARTESIAN_POINT('Origin',(5.999999999061,24.7867247845918,9.33250979146072));
#41601=CARTESIAN_POINT('',(5.9885258135532,25.0410389643412,11.3308503205391));
#41602=CARTESIAN_POINT('Origin',(5.98846855808858,-11.4751154935115,-4.75314843118749));
#41603=CARTESIAN_POINT('Origin',(6.,24.1259421517583,10.9277801936249));
#41604=CARTESIAN_POINT('Origin',(6.99999997874242,-11.4664779467208,-4.74946027036764));
#41605=CARTESIAN_POINT('Origin',(5.999999877385,24.1259420367213,10.9277801432448));
#41606=CARTESIAN_POINT('Origin',(5.99999764421527,24.1259401206149,10.9277792069261));
#41607=CARTESIAN_POINT('Ctrl Pts',(-6.09415743589287,25.0685176670397,11.2705948926489));
#41608=CARTESIAN_POINT('Ctrl Pts',(-6.05606588732271,25.0626152520279,11.2828610723339));
#41609=CARTESIAN_POINT('Ctrl Pts',(-5.71207088618283,25.0098877697791,11.3926635700215));
#41610=CARTESIAN_POINT('Ctrl Pts',(-5.02599367392107,24.9149190577036,11.5942416721674));
#41611=CARTESIAN_POINT('Ctrl Pts',(-3.98564775783899,24.7979400134299,11.8483582951752));
#41612=CARTESIAN_POINT('Ctrl Pts',(-2.81213472137221,24.6988235435346,12.0680547776604));
#41613=CARTESIAN_POINT('Ctrl Pts',(-1.52041606170006,24.629776117468,12.2244388462329));
#41614=CARTESIAN_POINT('Ctrl Pts',(-0.18938368979716,24.6028735621445,12.2876144937024));
#41615=CARTESIAN_POINT('Ctrl Pts',(1.08604876859294,24.6176047392936,12.2527453884866));
#41616=CARTESIAN_POINT('Ctrl Pts',(2.24115591625819,24.6651918941777,12.143937035736));
#41617=CARTESIAN_POINT('Ctrl Pts',(3.27282426521286,24.735605003468,11.9862434179946));
#41618=CARTESIAN_POINT('Ctrl Pts',(4.19977149222157,24.8213849139756,11.797279536956));
#41619=CARTESIAN_POINT('Ctrl Pts',(5.05677934758209,24.9199603491257,11.5836987166178));
#41620=CARTESIAN_POINT('Ctrl Pts',(5.68020727784929,25.0054672272717,11.4020597285418));
#41621=CARTESIAN_POINT('Ctrl Pts',(6.02208888462226,25.0573454648108,11.2938086928354));
#41622=CARTESIAN_POINT('Ctrl Pts',(6.09402271352824,25.0684922274053,11.2706461600882));
#41623=CARTESIAN_POINT('Ctrl Pts',(-6.21832045053098,24.9356363004755,11.6022681603765));
#41624=CARTESIAN_POINT('Ctrl Pts',(-6.17949927506643,24.9295088225807,11.6147172343648));
#41625=CARTESIAN_POINT('Ctrl Pts',(-5.82891139943057,24.8747368508288,11.726143286659));
#41626=CARTESIAN_POINT('Ctrl Pts',(-5.12960176764218,24.7754946259934,11.9304638300121));
#41627=CARTESIAN_POINT('Ctrl Pts',(-4.06864373240013,24.6520241911184,12.1875933298324));
#41628=CARTESIAN_POINT('Ctrl Pts',(-2.87116826711582,24.5463532301321,12.4094995450073));
#41629=CARTESIAN_POINT('Ctrl Pts',(-1.55239219352023,24.4718951869516,12.5670902012212));
#41630=CARTESIAN_POINT('Ctrl Pts',(-0.193327228898783,24.4423488465848,
12.6304801584094));
#41631=CARTESIAN_POINT('Ctrl Pts',(1.10884029560539,24.458591025936,12.595525156871));
#41632=CARTESIAN_POINT('Ctrl Pts',(2.28827733619991,24.5101590878462,12.4860015055859));
#41633=CARTESIAN_POINT('Ctrl Pts',(3.34130595899083,24.5856379456193,12.3268930309681));
#41634=CARTESIAN_POINT('Ctrl Pts',(4.28702500002799,24.6768035896854,12.1359205564239));
#41635=CARTESIAN_POINT('Ctrl Pts',(5.16096421537736,24.7807262870167,11.9197644114018));
#41636=CARTESIAN_POINT('Ctrl Pts',(5.79643509966697,24.8701221577978,11.7356686956827));
#41637=CARTESIAN_POINT('Ctrl Pts',(6.14487117451663,24.9240358177971,11.6258273593906));
#41638=CARTESIAN_POINT('Ctrl Pts',(6.21818308061221,24.935607236778,11.6023191866738));
#41639=CARTESIAN_POINT('Ctrl Pts',(-6.32908148189132,24.6417686601331,11.8134211097232));
#41640=CARTESIAN_POINT('Ctrl Pts',(-6.28955536353039,24.6354614716029,11.8259897628201));
#41641=CARTESIAN_POINT('Ctrl Pts',(-5.9326099399111,24.5790644008174,11.9384537675389));
#41642=CARTESIAN_POINT('Ctrl Pts',(-5.22075534857246,24.4765500531428,12.1441201140726));
#41643=CARTESIAN_POINT('Ctrl Pts',(-4.14076534440852,24.3483246298362,12.4018806751728));
#41644=CARTESIAN_POINT('Ctrl Pts',(-2.92177802351305,24.2380190316229,12.623417756821));
#41645=CARTESIAN_POINT('Ctrl Pts',(-1.57939308859398,24.1598585351471,12.7799736491164));
#41646=CARTESIAN_POINT('Ctrl Pts',(-0.196603179997715,24.1285646331443,
12.8424291350917));
#41647=CARTESIAN_POINT('Ctrl Pts',(1.12799353750622,24.145800396657,12.8080494910814));
#41648=CARTESIAN_POINT('Ctrl Pts',(2.32845047098897,24.2000621596312,12.6994858356328));
#41649=CARTESIAN_POINT('Ctrl Pts',(3.40035685412353,24.2790638500178,12.541010654418));
#41650=CARTESIAN_POINT('Ctrl Pts',(4.36306687247048,24.37407672428,12.3501091583462));
#41651=CARTESIAN_POINT('Ctrl Pts',(5.25267862906944,24.4819336875387,12.1333190695919));
#41652=CARTESIAN_POINT('Ctrl Pts',(5.89955400274272,24.5743007947612,11.9480450763936));
#41653=CARTESIAN_POINT('Ctrl Pts',(6.25429750719079,24.6298264279853,11.8372049534228));
#41654=CARTESIAN_POINT('Ctrl Pts',(6.32894084676985,24.6417369929965,11.8134705227596));
#41655=CARTESIAN_POINT('Ctrl Pts',(-6.3948835653583,24.2701531214398,11.8436584888777));
#41656=CARTESIAN_POINT('Ctrl Pts',(-6.35487788326796,24.2637628345041,11.8562492153957));
#41657=CARTESIAN_POINT('Ctrl Pts',(-5.99362024492343,24.2066236152637,11.9688687058286));
#41658=CARTESIAN_POINT('Ctrl Pts',(-5.27348028276714,24.1027722982909,12.1740977236281));
#41659=CARTESIAN_POINT('Ctrl Pts',(-4.18145907214454,23.9728859143447,12.4299220155458));
#41660=CARTESIAN_POINT('Ctrl Pts',(-2.94953904132581,23.8611893602657,12.6486097593309));
#41661=CARTESIAN_POINT('Ctrl Pts',(-1.59372167501731,23.7820925676294,12.8021784804847));
#41662=CARTESIAN_POINT('Ctrl Pts',(-0.198277517951755,23.7504469244805,
12.8628138246229));
#41663=CARTESIAN_POINT('Ctrl Pts',(1.13804826101955,23.7678747864035,12.8295086797204));
#41664=CARTESIAN_POINT('Ctrl Pts',(2.35022440053216,23.822773196571,12.7233112457001));
#41665=CARTESIAN_POINT('Ctrl Pts',(3.43314706917537,23.9027483421861,12.5673423471683));
#41666=CARTESIAN_POINT('Ctrl Pts',(4.40622700507742,23.9989711658464,12.3785763590503));
#41667=CARTESIAN_POINT('Ctrl Pts',(5.30578879644537,24.1082261614275,12.163278950266));
#41668=CARTESIAN_POINT('Ctrl Pts',(5.96018277708729,24.201798828066,11.9784436509294));
#41669=CARTESIAN_POINT('Ctrl Pts',(6.31919090105992,24.2580531508172,11.8674819873968));
#41670=CARTESIAN_POINT('Ctrl Pts',(6.39473997516368,24.2701206149759,11.8437053722807));
#41671=CARTESIAN_POINT('',(-5.98852245733775,25.0410395152739,11.3308498383567));
#41672=CARTESIAN_POINT('Ctrl Pts',(-5.98852261949159,25.0410393033428,11.3308502493368));
#41673=CARTESIAN_POINT('Ctrl Pts',(-5.87207793491996,25.0233585862853,11.367676505058));
#41674=CARTESIAN_POINT('Ctrl Pts',(-5.74893720729897,25.0052500193778,11.4056119122923));
#41675=CARTESIAN_POINT('Ctrl Pts',(-5.6190981775558,24.986894679695,11.4442931780282));
#41676=CARTESIAN_POINT('Ctrl Pts',(-5.51159709980728,24.9716972556058,11.4763195861391));
#41677=CARTESIAN_POINT('Ctrl Pts',(-5.3995042185231,24.9563309052265,11.508856518002));
#41678=CARTESIAN_POINT('Ctrl Pts',(-5.28282127163981,24.9409034536848,11.5416713122482));
#41679=CARTESIAN_POINT('Ctrl Pts',(-5.21054205127972,24.9313469229375,11.5619984278014));
#41680=CARTESIAN_POINT('Ctrl Pts',(-5.13650113482633,24.9217682042197,11.582429041541));
#41681=CARTESIAN_POINT('Ctrl Pts',(-5.06069864646884,24.9121968136603,11.6028960441539));
#41682=CARTESIAN_POINT('Ctrl Pts',(-5.00141638199723,24.90471139044,11.6189025142333));
#41683=CARTESIAN_POINT('Ctrl Pts',(-4.94105673142941,24.8972304452503,11.6349311595742));
#41684=CARTESIAN_POINT('Ctrl Pts',(-4.87961956272349,24.8897694846537,11.6509486356637));
#41685=CARTESIAN_POINT('Ctrl Pts',(-4.80962202785255,24.8812689488946,11.6691979115456));
#41686=CARTESIAN_POINT('Ctrl Pts',(-4.73822586615999,24.872794473703,11.6874324435812));
#41687=CARTESIAN_POINT('Ctrl Pts',(-4.66543107683349,24.8643703477828,11.7055991591889));
#41688=CARTESIAN_POINT('Ctrl Pts',(-4.62903368217023,24.8601582848227,11.7146825169927));
#41689=CARTESIAN_POINT('Ctrl Pts',(-4.59228663064168,24.8559588042056,11.7237489184915));
#41690=CARTESIAN_POINT('Ctrl Pts',(-4.55518992231137,24.8517750652626,11.7327913774651));
#41691=CARTESIAN_POINT('Ctrl Pts',(-4.53664156814622,24.8496831957911,11.7373126069519));
#41692=CARTESIAN_POINT('Ctrl Pts',(-4.51800579978205,24.8475952614153,11.7418278506626));
#41693=CARTESIAN_POINT('Ctrl Pts',(-4.49928261723233,24.8455116586679,11.7463362265013));
#41694=CARTESIAN_POINT('Ctrl Pts',(-4.48992102595747,24.8444698572942,11.7485904144207));
#41695=CARTESIAN_POINT('Ctrl Pts',(-4.48053758113626,24.8434291388063,11.7508428853625));
#41696=CARTESIAN_POINT('Ctrl Pts',(-4.47113228277049,24.8423895531611,11.7530935278688));
#41697=CARTESIAN_POINT('Ctrl Pts',(-4.46172698440472,24.8413499675159,11.7553441703752));
#41698=CARTESIAN_POINT('Ctrl Pts',(-4.45105740215062,24.8401751261721,11.7578884213725));
#41699=CARTESIAN_POINT('Ctrl Pts',(-4.44285082704132,24.8392742447742,11.7598398582553));
#41700=CARTESIAN_POINT('Ctrl Pts',(-4.30874234749329,24.82455241101,11.7917294382317));
#41701=CARTESIAN_POINT('Ctrl Pts',(-4.17030708102564,24.8100278948711,11.8233188134517));
#41702=CARTESIAN_POINT('Ctrl Pts',(-4.02753713404441,24.7958393518128,11.854288220348));
#41703=CARTESIAN_POINT('Ctrl Pts',(-3.89073584503476,24.7822439767314,11.8839629164088));
#41704=CARTESIAN_POINT('Ctrl Pts',(-3.74995452320826,24.7689570371205,11.9130681133127));
#41705=CARTESIAN_POINT('Ctrl Pts',(-3.60520088693431,24.7561100633647,11.9413069555636));
#41706=CARTESIAN_POINT('Ctrl Pts',(-3.45728944070361,24.7429828320437,11.9701618299883));
#41707=CARTESIAN_POINT('Ctrl Pts',(-3.30522643392144,24.7303154547137,11.9981112189699));
#41708=CARTESIAN_POINT('Ctrl Pts',(-3.14901186672775,24.7182538149112,12.024819615501));
#41709=CARTESIAN_POINT('Ctrl Pts',(-3.07090458313091,24.7122229950099,12.0381738137665));
#41710=CARTESIAN_POINT('Ctrl Pts',(-2.99175940932096,24.7063436716989,12.0512175142174));
#41711=CARTESIAN_POINT('Ctrl Pts',(-2.91157634444144,24.700634331209,12.063907458552));
#41712=CARTESIAN_POINT('Ctrl Pts',(-2.89518327517228,24.6994670820614,12.0665018609587));
#41713=CARTESIAN_POINT('Ctrl Pts',(-2.87874682718898,24.6983069354887,12.0690814800435));
#41714=CARTESIAN_POINT('Ctrl Pts',(-2.86226699502409,24.6971540534798,12.0716459347082));
#41715=CARTESIAN_POINT('Ctrl Pts',(-2.8384431040123,24.6954874020809,12.0753532108399));
#41716=CARTESIAN_POINT('Ctrl Pts',(-2.81452854523531,24.6938359325218,12.0790287957438));
#41717=CARTESIAN_POINT('Ctrl Pts',(-2.79052332865339,24.6922001294037,12.0826715709229));
#41718=CARTESIAN_POINT('Ctrl Pts',(-2.77021808960921,24.6908164562663,12.0857528770442));
#41719=CARTESIAN_POINT('Ctrl Pts',(-2.74984798236282,24.6894439939256,12.0888107047357));
#41720=CARTESIAN_POINT('Ctrl Pts',(-2.72941300692308,24.6880830383011,12.0918443696352));
#41721=CARTESIAN_POINT('Ctrl Pts',(-2.71919551920321,24.6874025604888,12.093361202085));
#41722=CARTESIAN_POINT('Ctrl Pts',(-2.70896181443498,24.6867249593443,12.0948719938314));
#41723=CARTESIAN_POINT('Ctrl Pts',(-2.69871189261957,24.6860502718866,12.0963766590913));
#41724=CARTESIAN_POINT('Ctrl Pts',(-2.68846197080415,24.6853755844289,12.0978813243511));
#41725=CARTESIAN_POINT('Ctrl Pts',(-2.67679403336437,24.6846126296739,12.0995833127281));
#41726=CARTESIAN_POINT('Ctrl Pts',(-2.66791347603294,24.6840349875721,12.1008721895521));
#41727=CARTESIAN_POINT('Ctrl Pts',(-2.4821521808828,24.6719520133897,12.1278325952085));
#41728=CARTESIAN_POINT('Ctrl Pts',(-2.29149550277842,24.6608332437257,12.1527602433646));
#41729=CARTESIAN_POINT('Ctrl Pts',(-2.09593759986156,24.650876181895,12.1751838538152));
#41730=CARTESIAN_POINT('Ctrl Pts',(-1.99233080678487,24.6456009195335,12.1870639074123));
#41731=CARTESIAN_POINT('Ctrl Pts',(-1.8873486430624,24.6406519782498,12.1982403723087));
#41732=CARTESIAN_POINT('Ctrl Pts',(-1.78099278865241,24.6360604107183,12.2086380279229));
#41733=CARTESIAN_POINT('Ctrl Pts',(-1.70012356698525,24.6325691455261,12.2165440366833));
#41734=CARTESIAN_POINT('Ctrl Pts',(-1.61846022911966,24.6292839247932,12.224000922958));
#41735=CARTESIAN_POINT('Ctrl Pts',(-1.53600131366634,24.6262173530196,12.2309772469221));
#41736=CARTESIAN_POINT('Ctrl Pts',(-1.46189047453595,24.623461238582,12.2372472932862));
#41737=CARTESIAN_POINT('Ctrl Pts',(-1.38713698026269,24.6208817564744,12.2431291335178));
#41738=CARTESIAN_POINT('Ctrl Pts',(-1.31174209049372,24.6184872332426,12.2485996392047));
#41739=CARTESIAN_POINT('Ctrl Pts',(-1.23210084282666,24.6159578467241,12.2543782523125));
#41740=CARTESIAN_POINT('Ctrl Pts',(-1.15174319434939,24.6136348616426,12.2596978632149));
#41741=CARTESIAN_POINT('Ctrl Pts',(-1.07066914350866,24.6115276457487,12.2645315222443));
#41742=CARTESIAN_POINT('Ctrl Pts',(-1.0301321180883,24.6104740378018,12.266948351759));
#41743=CARTESIAN_POINT('Ctrl Pts',(-0.989415992075765,24.6094743681992,
12.2692436913045));
#41744=CARTESIAN_POINT('Ctrl Pts',(-0.948520765373996,24.6085297687523,
12.2714141896979));
#41745=CARTESIAN_POINT('Ctrl Pts',(-0.928073152023112,24.6080574690288,
12.2724994388946));
#41746=CARTESIAN_POINT('Ctrl Pts',(-0.907580763500364,24.6075989365854,
12.2735534776725));
#41747=CARTESIAN_POINT('Ctrl Pts',(-0.887043599803289,24.6071543101594,
12.2745758886923));
#41748=CARTESIAN_POINT('Ctrl Pts',(-0.876775017954752,24.6069319969463,
12.2750870942022));
#41749=CARTESIAN_POINT('Ctrl Pts',(-0.866495242312671,24.6067131602211,
12.2755903927643));
#41750=CARTESIAN_POINT('Ctrl Pts',(-0.856204272877411,24.606497817139,12.2760857323367));
#41751=CARTESIAN_POINT('Ctrl Pts',(-0.845913303442152,24.6062824740569,
12.276581071909));
#41752=CARTESIAN_POINT('Ctrl Pts',(-0.833923452112789,24.6060365318656,
12.2771468969945));
#41753=CARTESIAN_POINT('Ctrl Pts',(-0.825297783192767,24.6058622858817,
12.2775478220662));
#41754=CARTESIAN_POINT('Ctrl Pts',(-0.603448600429803,24.6013807402201,
12.2878594744521));
#41755=CARTESIAN_POINT('Ctrl Pts',(-0.37948689987281,24.5986967762817,12.2941000099995));
#41756=CARTESIAN_POINT('Ctrl Pts',(-0.153407991024057,24.5978627736661,
12.2960214975774));
#41757=CARTESIAN_POINT('Ctrl Pts',(-0.0982029330636953,24.5976591228127,
12.2964906958483));
#41758=CARTESIAN_POINT('Ctrl Pts',(-0.0428716688643059,24.5975658351456,
12.2967021493351));
#41759=CARTESIAN_POINT('Ctrl Pts',(0.0125852473994843,24.5975839691981,
12.2966545842673));
#41760=CARTESIAN_POINT('Ctrl Pts',(0.153868872215892,24.5976301680285,12.296533406141));
#41761=CARTESIAN_POINT('Ctrl Pts',(0.295970723308233,24.5984017381627,12.2947266476478));
#41762=CARTESIAN_POINT('Ctrl Pts',(0.438890814847712,24.5999222771681,12.2912014538534));
#41763=CARTESIAN_POINT('Ctrl Pts',(0.510350860617452,24.6006825466707,12.2894388569562));
#41764=CARTESIAN_POINT('Ctrl Pts',(0.582015466023035,24.601630062137,12.2872466528321));
#41765=CARTESIAN_POINT('Ctrl Pts',(0.653884631028569,24.6027671760295,12.2846220155009));
#41766=CARTESIAN_POINT('Ctrl Pts',(0.689819213531337,24.6033357329758,12.2833096968352));
#41767=CARTESIAN_POINT('Ctrl Pts',(0.725804935920057,24.6039516899836,12.2818892701023));
#41768=CARTESIAN_POINT('Ctrl Pts',(0.761841798120305,24.6046153250416,12.2803604223681));
#41769=CARTESIAN_POINT('Ctrl Pts',(0.779860229220428,24.6049471425706,12.279595998501));
#41770=CARTESIAN_POINT('Ctrl Pts',(0.797891445272787,24.605290879649,12.2788044694029));
#41771=CARTESIAN_POINT('Ctrl Pts',(0.815935446265884,24.6056465689519,12.2779858007266));
#41772=CARTESIAN_POINT('Ctrl Pts',(0.83397944725898,24.6060022582549,12.2771671320502));
#41773=CARTESIAN_POINT('Ctrl Pts',(0.853658583894958,24.6064039841691,12.2762429440323));
#41774=CARTESIAN_POINT('Ctrl Pts',(0.87010580405451,24.6067495256734,12.2754483431328));
#41775=CARTESIAN_POINT('Ctrl Pts',(0.954941294067503,24.6085318440561,12.2713497565011));
#41776=CARTESIAN_POINT('Ctrl Pts',(1.03915646094878,24.6105620309033,12.2666905034544));
#41777=CARTESIAN_POINT('Ctrl Pts',(1.12274548009874,24.6128302696018,12.2614976172157));
#41778=CARTESIAN_POINT('Ctrl Pts',(1.34023153233054,24.6187318854487,12.2479865084693));
#41779=CARTESIAN_POINT('Ctrl Pts',(1.55347748717843,24.6262439843172,12.2308663947161));
#41780=CARTESIAN_POINT('Ctrl Pts',(1.762483134133,24.6351832068705,12.2106215991613));
#41781=CARTESIAN_POINT('Ctrl Pts',(1.93916409218177,24.6427398945867,12.1935078516322));
#41782=CARTESIAN_POINT('Ctrl Pts',(2.11281537507269,24.651316669607,12.1741602852205));
#41783=CARTESIAN_POINT('Ctrl Pts',(2.28344819732607,24.6608102578807,12.1528458878894));
#41784=CARTESIAN_POINT('Ctrl Pts',(2.31468206971439,24.6625480333024,12.1489443456335));
#41785=CARTESIAN_POINT('Ctrl Pts',(2.34581483060569,24.6643165454681,12.1449768417802));
#41786=CARTESIAN_POINT('Ctrl Pts',(2.37684657670109,24.6661151441892,12.14094498894));
#41787=CARTESIAN_POINT('Ctrl Pts',(2.47767146802531,24.6719589507231,12.1278451419897));
#41788=CARTESIAN_POINT('Ctrl Pts',(2.57829977290601,24.6781690799161,12.1139563702973));
#41789=CARTESIAN_POINT('Ctrl Pts',(2.67796169946932,24.6846878928205,12.0994139041198));
#41790=CARTESIAN_POINT('Ctrl Pts',(2.7797715261016,24.6913471982798,12.0845580207209));
#41791=CARTESIAN_POINT('Ctrl Pts',(2.88057272277316,24.6983286237912,12.0690200677786));
#41792=CARTESIAN_POINT('Ctrl Pts',(2.97955491921082,24.7055476241427,12.0529926455354));
#41793=CARTESIAN_POINT('Ctrl Pts',(3.01344853081799,24.7080195635714,12.0475045149005));
#41794=CARTESIAN_POINT('Ctrl Pts',(3.04712895742347,24.7105191649477,12.041959394733));
#41795=CARTESIAN_POINT('Ctrl Pts',(3.08056397514964,24.7130424427068,12.0363662321172));
#41796=CARTESIAN_POINT('Ctrl Pts',(3.15906127928106,24.7189664862736,12.023234844226));
#41797=CARTESIAN_POINT('Ctrl Pts',(3.23641909095361,24.7250360856396,12.0098052009448));
#41798=CARTESIAN_POINT('Ctrl Pts',(3.31263593447761,24.7312319284034,11.9961212804716));
#41799=CARTESIAN_POINT('Ctrl Pts',(3.45649514762954,24.742926575198,11.9702928947618));
#41800=CARTESIAN_POINT('Ctrl Pts',(3.59628911990336,24.7550705254824,11.9435601098344));
#41801=CARTESIAN_POINT('Ctrl Pts',(3.73202210256371,24.7675395543834,11.9162079919652));
#41802=CARTESIAN_POINT('Ctrl Pts',(3.83584437063496,24.7770771246613,11.8952863349142));
#41803=CARTESIAN_POINT('Ctrl Pts',(3.93728959584421,24.7868049511524,11.8740020174483));
#41804=CARTESIAN_POINT('Ctrl Pts',(4.03635777754101,24.7966696197805,11.8524749977332));
#41805=CARTESIAN_POINT('Ctrl Pts',(4.06112482296521,24.7991357869376,11.8470932428044));
#41806=CARTESIAN_POINT('Ctrl Pts',(4.08675526253289,24.8017100309838,11.8414789509819));
#41807=CARTESIAN_POINT('Ctrl Pts',(4.11470923698786,24.8045497714992,11.8352904735459));
#41808=CARTESIAN_POINT('Ctrl Pts',(4.14266321144283,24.8073895120145,11.82910199611));
#41809=CARTESIAN_POINT('Ctrl Pts',(4.17043865119258,24.8102415991542,11.8228911837828));
#41810=CARTESIAN_POINT('Ctrl Pts',(4.19803555625679,24.8131048456758,11.8166606647739));
#41811=CARTESIAN_POINT('Ctrl Pts',(4.20574811713802,24.8139050427654,11.8149194094749));
#41812=CARTESIAN_POINT('Ctrl Pts',(4.21344673423827,24.8147061117068,11.8131766143782));
#41813=CARTESIAN_POINT('Ctrl Pts',(4.22113140699254,24.8155080272097,11.8114323353406));
#41814=CARTESIAN_POINT('Ctrl Pts',(4.26844096707861,24.820444902322,11.8006939374182));
#41815=CARTESIAN_POINT('Ctrl Pts',(4.31522201697745,24.8254138542797,11.7898993285224));
#41816=CARTESIAN_POINT('Ctrl Pts',(4.36147457069009,24.8304091817874,11.7790615486346));
#41817=CARTESIAN_POINT('Ctrl Pts',(4.51942902572204,24.8474684395116,11.7420500654077));
#41818=CARTESIAN_POINT('Ctrl Pts',(4.67122070919016,24.8648335220303,11.7045405147502));
#41819=CARTESIAN_POINT('Ctrl Pts',(4.81684736731411,24.8822895362551,11.6670123777528));
#41820=CARTESIAN_POINT('Ctrl Pts',(4.86949798788909,24.8886006745696,11.6534442596116));
#41821=CARTESIAN_POINT('Ctrl Pts',(4.92134287229698,24.8949238271383,11.639873245553));
#41822=CARTESIAN_POINT('Ctrl Pts',(4.97238230295595,24.9012492749469,11.6263204404126));
#41823=CARTESIAN_POINT('Ctrl Pts',(5.00462682834192,24.9052454218437,11.6177583588266));
#41824=CARTESIAN_POINT('Ctrl Pts',(5.03654983709019,24.9092421091841,11.609204372807));
#41825=CARTESIAN_POINT('Ctrl Pts',(5.06815129371138,24.9132371956239,11.600663060826));
#41826=CARTESIAN_POINT('Ctrl Pts',(5.21039120872686,24.931219302034,11.5622181402369));
#41827=CARTESIAN_POINT('Ctrl Pts',(5.34611635892373,24.9491683164726,11.5240340989402));
#41828=CARTESIAN_POINT('Ctrl Pts',(5.47532628982706,24.9669060425853,11.4865024016981));
#41829=CARTESIAN_POINT('Ctrl Pts',(5.60705266944068,24.9849892226247,11.4482397498733));
#41830=CARTESIAN_POINT('Ctrl Pts',(5.73200777566556,25.0028526551875,11.4106549774584));
#41831=CARTESIAN_POINT('Ctrl Pts',(5.85019315529358,25.0203177622383,11.3741100912551));
#41832=CARTESIAN_POINT('Ctrl Pts',(5.86232961592042,25.0221112546714,11.3703572956562));
#41833=CARTESIAN_POINT('Ctrl Pts',(5.87439468833947,25.0239005565685,11.3666154218325));
#41834=CARTESIAN_POINT('Ctrl Pts',(5.88638837412032,25.025685481493,11.3628848318741));
#41835=CARTESIAN_POINT('Ctrl Pts',(5.92102986643391,25.0308408994504,11.3521097285629));
#41836=CARTESIAN_POINT('Ctrl Pts',(5.95507582044337,25.0359598050818,11.3414287803088));
#41837=CARTESIAN_POINT('Ctrl Pts',(5.98852582161158,25.0410382878129,11.330850113083));
#41838=CARTESIAN_POINT('',(-6.27159361731522,24.2690120888703,11.879497561603));
#41839=CARTESIAN_POINT('Origin',(-5.999994980806,24.1259380084193,10.9277770011849));
#41840=CARTESIAN_POINT('Ctrl Pts',(-6.27159386307668,24.269012372504,11.8794985003143));
#41841=CARTESIAN_POINT('Ctrl Pts',(-6.19708064355491,24.257447552827,11.9025009420341));
#41842=CARTESIAN_POINT('Ctrl Pts',(-6.11543893234907,24.2450493535732,11.9272858599129));
#41843=CARTESIAN_POINT('Ctrl Pts',(-6.02658469700067,24.2319368708288,11.9536191464949));
#41844=CARTESIAN_POINT('Ctrl Pts',(-5.93855993474233,24.2189467958857,11.9797066062742));
#41845=CARTESIAN_POINT('Ctrl Pts',(-5.84345652710574,24.2052557303348,12.0073137939348));
#41846=CARTESIAN_POINT('Ctrl Pts',(-5.74118379376358,24.1909996650877,12.0361672876422));
#41847=CARTESIAN_POINT('Ctrl Pts',(-5.64049529917842,24.176964431047,12.0645738311068));
#41848=CARTESIAN_POINT('Ctrl Pts',(-5.53285770076121,24.1623816026613,12.0941884706608));
#41849=CARTESIAN_POINT('Ctrl Pts',(-5.41817811424983,24.1474001738651,12.1247040182081));
#41850=CARTESIAN_POINT('Ctrl Pts',(-5.37925230863917,24.1423150126535,12.13506194073));
#41851=CARTESIAN_POINT('Ctrl Pts',(-5.33951512841442,24.1371840902973,12.1455232546647));
#41852=CARTESIAN_POINT('Ctrl Pts',(-5.29896282541134,24.1320137374897,12.1560746713286));
#41853=CARTESIAN_POINT('Ctrl Pts',(-5.21821392328632,24.1217183835418,12.1770849530728));
#41854=CARTESIAN_POINT('Ctrl Pts',(-5.13423307029617,24.1112663286752,12.1984531632364));
#41855=CARTESIAN_POINT('Ctrl Pts',(-5.04699092036662,24.100713815105,12.2200666333059));
#41856=CARTESIAN_POINT('Ctrl Pts',(-4.92201158417912,24.0855967399048,12.2510291570879));
#41857=CARTESIAN_POINT('Ctrl Pts',(-4.79033922609239,24.0702724377968,12.2824971537965));
#41858=CARTESIAN_POINT('Ctrl Pts',(-4.65188793009117,24.0549260394076,12.3140996072383));
#41859=CARTESIAN_POINT('Ctrl Pts',(-4.51343663408995,24.0395796410183,12.3457020606801));
#41860=CARTESIAN_POINT('Ctrl Pts',(-4.36820620262285,24.0242110240233,12.3774392325216));
#41861=CARTESIAN_POINT('Ctrl Pts',(-4.21611372758432,24.0090302236472,12.4088898513687));
#41862=CARTESIAN_POINT('Ctrl Pts',(-4.07083064523525,23.9945290889224,12.438932382051));
#41863=CARTESIAN_POINT('Ctrl Pts',(-3.9192856554265,23.9801993615862,12.4687131290188));
#41864=CARTESIAN_POINT('Ctrl Pts',(-3.7614235687259,23.9662478755224,12.4978242922883));
#41865=CARTESIAN_POINT('Ctrl Pts',(-3.73054864789812,23.963519221438,12.503517900424));
#41866=CARTESIAN_POINT('Ctrl Pts',(-3.69943212037155,23.9608051084921,12.5091857580551));
#41867=CARTESIAN_POINT('Ctrl Pts',(-3.66807362860842,23.9581071913898,12.514824611152));
#41868=CARTESIAN_POINT('Ctrl Pts',(-3.58017498071281,23.9505448613129,12.5306304594259));
#41869=CARTESIAN_POINT('Ctrl Pts',(-3.49037513304142,23.9431096153184,12.5462087339496));
#41870=CARTESIAN_POINT('Ctrl Pts',(-3.39866711183985,23.9358394491402,12.5614848729961));
#41871=CARTESIAN_POINT('Ctrl Pts',(-3.35281310123906,23.9322043660511,12.5691229425193));
#41872=CARTESIAN_POINT('Ctrl Pts',(-3.30648203830319,23.9286105462567,12.5766854205411));
#41873=CARTESIAN_POINT('Ctrl Pts',(-3.25967322154924,23.92506300707,12.5841625650012));
#41874=CARTESIAN_POINT('Ctrl Pts',(-3.23626881317227,23.9232892374766,12.5879011372313));
#41875=CARTESIAN_POINT('Ctrl Pts',(-3.21274496574493,23.9215270376051,12.591618372388));
#41876=CARTESIAN_POINT('Ctrl Pts',(-3.18910159554922,23.9197770412036,12.5953130281382));
#41877=CARTESIAN_POINT('Ctrl Pts',(-3.17727991045136,23.9189020430028,12.5971603560134));
#41878=CARTESIAN_POINT('Ctrl Pts',(-3.16542834462672,23.9180300956426,12.5990020388008));
#41879=CARTESIAN_POINT('Ctrl Pts',(-3.15354688824311,23.9171612793004,12.6008379195334));
#41880=CARTESIAN_POINT('Ctrl Pts',(-3.14166543185951,23.9162924629581,12.6026738002661));
#41881=CARTESIAN_POINT('Ctrl Pts',(-3.12814004122944,23.9153102008938,12.6047504367141));
#41882=CARTESIAN_POINT('Ctrl Pts',(-3.11781283770736,23.9145643037385,12.6063279975685));
#41883=CARTESIAN_POINT('Ctrl Pts',(-3.07662183306194,23.9115892240741,12.6126202446754));
#41884=CARTESIAN_POINT('Ctrl Pts',(-3.03569007115575,23.9086934856334,12.6187479999135));
#41885=CARTESIAN_POINT('Ctrl Pts',(-2.99501928702404,23.9058749439134,12.6247156162381));
#41886=CARTESIAN_POINT('Ctrl Pts',(-2.79740326461739,23.8921798796164,12.6537117771556));
#41887=CARTESIAN_POINT('Ctrl Pts',(-2.60595262443292,23.8803068051101,12.6789288382829));
#41888=CARTESIAN_POINT('Ctrl Pts',(-2.42086041740396,23.8700053894468,12.7008770362872));
#41889=CARTESIAN_POINT('Ctrl Pts',(-2.23093226975246,23.8594348266634,12.7233986791924));
#41890=CARTESIAN_POINT('Ctrl Pts',(-2.04769883486201,23.8505189268116,12.7424787292335));
#41891=CARTESIAN_POINT('Ctrl Pts',(-1.87131988108705,23.8429960706186,12.7586446085497));
#41892=CARTESIAN_POINT('Ctrl Pts',(-1.78117209842544,23.8391511175186,12.7669070352391));
#41893=CARTESIAN_POINT('Ctrl Pts',(-1.69281414034322,23.8356702230497,12.7744077954315));
#41894=CARTESIAN_POINT('Ctrl Pts',(-1.60626302545199,23.8325195648083,12.7812145895975));
#41895=CARTESIAN_POINT('Ctrl Pts',(-1.43906926035782,23.8264333299335,12.794363507971));
#41896=CARTESIAN_POINT('Ctrl Pts',(-1.27862001152862,23.8215783542681,12.8049253098459));
#41897=CARTESIAN_POINT('Ctrl Pts',(-1.12501483737541,23.8177149735438,12.8133805318948));
#41898=CARTESIAN_POINT('Ctrl Pts',(-0.969937943776955,23.8138145770577,
12.8219167649825));
#41899=CARTESIAN_POINT('Ctrl Pts',(-0.821836508844503,23.8109247554415,
12.82830598725));
#41900=CARTESIAN_POINT('Ctrl Pts',(-0.68078060386382,23.8088158620706,12.8330037588192));
#41901=CARTESIAN_POINT('Ctrl Pts',(-0.538386326148549,23.8066869590064,
12.8377461039877));
#41902=CARTESIAN_POINT('Ctrl Pts',(-0.403171528273148,23.8053537628513,
12.8407648857556));
#41903=CARTESIAN_POINT('Ctrl Pts',(-0.275181359097709,23.804598937094,12.8424872539434));
#41904=CARTESIAN_POINT('Ctrl Pts',(-0.236216706984929,23.8043691419212,
12.8430116026312));
#41905=CARTESIAN_POINT('Ctrl Pts',(-0.197921471761721,23.8041930881746,
12.8434155026696));
#41906=CARTESIAN_POINT('Ctrl Pts',(-0.160296520170288,23.8040650105823,
12.8437102229334));
#41907=CARTESIAN_POINT('Ctrl Pts',(-0.153989049541499,23.8040435395739,
12.8437596300244));
#41908=CARTESIAN_POINT('Ctrl Pts',(-0.147700415760366,23.8040234172524,
12.8438059679572));
#41909=CARTESIAN_POINT('Ctrl Pts',(-0.141430622130303,23.8040046157402,
12.8438492897956));
#41910=CARTESIAN_POINT('Ctrl Pts',(-0.103047756612804,23.8038895153152,
12.8441145004857));
#41911=CARTESIAN_POINT('Ctrl Pts',(-0.0662555271181962,23.8038251183766,
12.8442644027209));
#41912=CARTESIAN_POINT('Ctrl Pts',(-0.0289807949193498,23.803801947349,
12.8443170163513));
#41913=CARTESIAN_POINT('Ctrl Pts',(-0.0185588386823882,23.8037954687663,
12.8443317270392));
#41914=CARTESIAN_POINT('Ctrl Pts',(-0.00809916138173642,23.8037923566792,
12.8443385556309));
#41915=CARTESIAN_POINT('Ctrl Pts',(0.00244355159875256,23.8037927379189,
12.8443372526226));
#41916=CARTESIAN_POINT('Ctrl Pts',(0.127127933612357,23.8037972466852,12.8443218424727));
#41917=CARTESIAN_POINT('Ctrl Pts',(0.258986326506927,23.8042924730393,12.8431696778079));
#41918=CARTESIAN_POINT('Ctrl Pts',(0.397985511715484,23.8054910530804,12.8404650188549));
#41919=CARTESIAN_POINT('Ctrl Pts',(0.535666539858683,23.8066782667474,12.8377860087235));
#41920=CARTESIAN_POINT('Ctrl Pts',(0.680353891965151,23.8085556400841,12.8335836971678));
#41921=CARTESIAN_POINT('Ctrl Pts',(0.831993331814887,23.8113495659765,12.8274126597883));
#41922=CARTESIAN_POINT('Ctrl Pts',(0.942271900153292,23.8133814262087,12.8229248222703));
#41923=CARTESIAN_POINT('Ctrl Pts',(1.05622686550899,23.815898445416,12.8173949054093));
#41924=CARTESIAN_POINT('Ctrl Pts',(1.17382842541542,23.8189939856533,12.8106381116661));
#41925=CARTESIAN_POINT('Ctrl Pts',(1.33438952036287,23.8232203184531,12.8014130792551));
#41926=CARTESIAN_POINT('Ctrl Pts',(1.5017497937385,23.8285247626977,12.7899019055094));
#41927=CARTESIAN_POINT('Ctrl Pts',(1.67579823257016,23.8351501275165,12.7756189141176));
#41928=CARTESIAN_POINT('Ctrl Pts',(1.84379921228085,23.8415452884728,12.7618321972523));
#41929=CARTESIAN_POINT('Ctrl Pts',(2.01803188912892,23.8491713462831,12.7454626456316));
#41930=CARTESIAN_POINT('Ctrl Pts',(2.19835974409792,23.8582571099095,12.7260476068924));
#41931=CARTESIAN_POINT('Ctrl Pts',(2.26108749646338,23.8614176284601,12.7192940094384));
#41932=CARTESIAN_POINT('Ctrl Pts',(2.32455242973094,23.8647548580991,12.7121716847517));
#41933=CARTESIAN_POINT('Ctrl Pts',(2.38874762162472,23.8682786803638,12.7046604832679));
#41934=CARTESIAN_POINT('Ctrl Pts',(2.47500692939018,23.8730136528792,12.694567655108));
#41935=CARTESIAN_POINT('Ctrl Pts',(2.56258480368602,23.8780855236188,12.6837727027421));
#41936=CARTESIAN_POINT('Ctrl Pts',(2.65146457977943,23.8835179280606,12.6722277590264));
#41937=CARTESIAN_POINT('Ctrl Pts',(2.72897715545603,23.8882555599372,12.6621593456845));
#41938=CARTESIAN_POINT('Ctrl Pts',(2.80747992660754,23.893267461597,12.6515204889937));
#41939=CARTESIAN_POINT('Ctrl Pts',(2.88696060483214,23.8985693823657,12.6402790380552));
#41940=CARTESIAN_POINT('Ctrl Pts',(2.92670094394444,23.90122034275,12.6346583125859));
#41941=CARTESIAN_POINT('Ctrl Pts',(2.96668575863641,23.9039438070294,12.6288869308983));
#41942=CARTESIAN_POINT('Ctrl Pts',(3.00691339184227,23.9067417699088,12.622960840973));
#41943=CARTESIAN_POINT('Ctrl Pts',(3.02702720844519,23.9081407513484,12.6199977960103));
#41944=CARTESIAN_POINT('Ctrl Pts',(3.04720172962192,23.9095583573876,12.616996073527));
#41945=CARTESIAN_POINT('Ctrl Pts',(3.06743674365025,23.9109948367397,12.6139551648845));
#41946=CARTESIAN_POINT('Ctrl Pts',(3.07755425066441,23.9117130764157,12.6124347105632));
#41947=CARTESIAN_POINT('Ctrl Pts',(3.08768688088734,23.9124360344167,12.6109044596733));
#41948=CARTESIAN_POINT('Ctrl Pts',(3.09783460737601,23.9131637418684,12.609364348521));
#41949=CARTESIAN_POINT('Ctrl Pts',(3.10798233386467,23.9138914493201,12.6078242373688));
#41950=CARTESIAN_POINT('Ctrl Pts',(3.11649242505667,23.9145041902963,12.6065275687504));
#41951=CARTESIAN_POINT('Ctrl Pts',(3.1283230485401,23.9153611437042,12.6047143704876));
#41952=CARTESIAN_POINT('Ctrl Pts',(3.24396953136792,23.9237380181527,12.5869900297497));
#41953=CARTESIAN_POINT('Ctrl Pts',(3.3568243586389,23.9324158983593,12.5687080553323));
#41954=CARTESIAN_POINT('Ctrl Pts',(3.46689563032691,23.9413247217354,12.5500051077454));
#41955=CARTESIAN_POINT('Ctrl Pts',(3.63913334366982,23.9552651018488,12.5207390433515));
#41956=CARTESIAN_POINT('Ctrl Pts',(3.80455492701866,23.9697695395805,12.490444984664));
#41957=CARTESIAN_POINT('Ctrl Pts',(3.96321661984212,23.9845904106421,12.4596112646828));
#41958=CARTESIAN_POINT('Ctrl Pts',(4.12187831266557,23.9994112817037,12.4287775447016));
#41959=CARTESIAN_POINT('Ctrl Pts',(4.27378038616038,24.0145487274433,12.3974038969458));
#41960=CARTESIAN_POINT('Ctrl Pts',(4.41899134479992,24.0297826839403,12.3659258747014));
#41961=CARTESIAN_POINT('Ctrl Pts',(4.56352096943963,24.0449451622747,12.3345955482439));
#41962=CARTESIAN_POINT('Ctrl Pts',(4.70142263439583,24.0602034826833,12.3031616819607));
#41963=CARTESIAN_POINT('Ctrl Pts',(4.83277716212323,24.0753674355567,12.2720080573813));
#41964=CARTESIAN_POINT('Ctrl Pts',(4.9053251093476,24.0837425838808,12.2548017109314));
#41965=CARTESIAN_POINT('Ctrl Pts',(4.9758759694648,24.0920893585459,12.237679993631));
#41966=CARTESIAN_POINT('Ctrl Pts',(5.04444366271275,24.1003786573682,12.2207014769521));
#41967=CARTESIAN_POINT('Ctrl Pts',(5.13538874063298,24.1113732073027,12.1981819426176));
#41968=CARTESIAN_POINT('Ctrl Pts',(5.22284501885468,24.1222664368161,12.175914753616));
#41969=CARTESIAN_POINT('Ctrl Pts',(5.3068450680899,24.1329958452549,12.1540254663863));
#41970=CARTESIAN_POINT('Ctrl Pts',(5.42689981753904,24.1483305558126,12.1227408074139));
#41971=CARTESIAN_POINT('Ctrl Pts',(5.5398950609485,24.1633299521138,12.0922300430563));
#41972=CARTESIAN_POINT('Ctrl Pts',(5.6459278454596,24.1778363423683,12.062817169183));
#41973=CARTESIAN_POINT('Ctrl Pts',(5.75378710239914,24.1925926130909,12.0328976425474));
#41974=CARTESIAN_POINT('Ctrl Pts',(5.85444212010429,24.2068387252984,12.0041140585228));
#41975=CARTESIAN_POINT('Ctrl Pts',(5.94798769898028,24.2204300315958,11.9767579553003));
#41976=CARTESIAN_POINT('Ctrl Pts',(6.02496474147653,24.2316140829963,11.9542470900558));
#41977=CARTESIAN_POINT('Ctrl Pts',(6.0971276192275,24.242355142051,11.932701864461));
#41978=CARTESIAN_POINT('Ctrl Pts',(6.16452450090078,24.2525832703824,11.9122610048017));
#41979=CARTESIAN_POINT('Ctrl Pts',(6.20165912102731,24.2582188079735,11.900998413126));
#41980=CARTESIAN_POINT('Ctrl Pts',(6.23734677868856,24.2636988328348,11.8900707158152));
#41981=CARTESIAN_POINT('Ctrl Pts',(6.27159479316366,24.2690136880232,11.8794983798008));
#41982=CARTESIAN_POINT('Ctrl Pts',(-6.390311350216,24.5118553841645,11.8061920238492));
#41983=CARTESIAN_POINT('Ctrl Pts',(-4.260207566811,24.1870632643171,12.4817966807133));
#41984=CARTESIAN_POINT('Ctrl Pts',(0.0001663376446825,23.8622675910407,
13.1582619392195));
#41985=CARTESIAN_POINT('Ctrl Pts',(4.2605402421,24.1870886272834,12.4817438562278));
#41986=CARTESIAN_POINT('Ctrl Pts',(6.39081036315,24.511931475205,11.806033745832));
#41987=CARTESIAN_POINT('Ctrl Pts',(-6.390311350216,23.5459013914926,11.972049816479));
#41988=CARTESIAN_POINT('Ctrl Pts',(-4.260207566811,23.2652611637952,12.607762371841));
#41989=CARTESIAN_POINT('Ctrl Pts',(0.0001663376446825,22.9846427151217,
13.246147024971));
#41990=CARTESIAN_POINT('Ctrl Pts',(4.2605402421,23.2652830770076,12.6077125210326));
#41991=CARTESIAN_POINT('Ctrl Pts',(6.39081036315,23.5459671387971,11.9719008842438));
#41992=CARTESIAN_POINT('Ctrl Pts',(-6.390311350216,21.4528944638882,12.0713624052953));
#41993=CARTESIAN_POINT('Ctrl Pts',(-4.260207566811,21.2792418481892,12.6592431178696));
#41994=CARTESIAN_POINT('Ctrl Pts',(0.0001663376446825,21.1056362242977,
13.2456913466391));
#41995=CARTESIAN_POINT('Ctrl Pts',(4.2605402421,21.2792554048749,12.6591973227215));
#41996=CARTESIAN_POINT('Ctrl Pts',(6.39081036315,21.452935146549,12.0712246788794));
#41997=CARTESIAN_POINT('Ctrl Pts',(-6.390311350216,18.3168609136256,11.387980855255));
#41998=CARTESIAN_POINT('Ctrl Pts',(-4.260207566811,18.3050659001773,12.0191856806278));
#41999=CARTESIAN_POINT('Ctrl Pts',(0.0001663376446825,18.2929947474349,
12.6510858022935));
#42000=CARTESIAN_POINT('Ctrl Pts',(4.2605402421,18.3050668428002,12.019136336187));
#42001=CARTESIAN_POINT('Ctrl Pts',(6.39081036315,18.3168636769111,11.3878329790519));
#42002=CARTESIAN_POINT('Ctrl Pts',(-6.390311350216,15.6639828127201,9.9696585797627));
#42003=CARTESIAN_POINT('Ctrl Pts',(-4.260207566811,15.7525582543281,10.7489240488924));
#42004=CARTESIAN_POINT('Ctrl Pts',(0.0001663376446825,15.8420472730181,
11.5272475946804));
#42005=CARTESIAN_POINT('Ctrl Pts',(4.2605402421,15.7525512662236,10.748863270397));
#42006=CARTESIAN_POINT('Ctrl Pts',(6.39081036315,15.6639620616126,9.96947601647265));
#42007=CARTESIAN_POINT('Ctrl Pts',(-6.390311350216,14.2540946963906,8.71288811092588));
#42008=CARTESIAN_POINT('Ctrl Pts',(-4.260207566811,14.3565358989963,9.62694787697193));
#42009=CARTESIAN_POINT('Ctrl Pts',(0.0001663376446825,14.4576055194805,
10.542393035863));
#42010=CARTESIAN_POINT('Ctrl Pts',(4.2605402421,14.3565280065696,9.62687639078721));
#42011=CARTESIAN_POINT('Ctrl Pts',(6.39081036315,14.2540706968538,8.71267396857703));
#42012=CARTESIAN_POINT('Ctrl Pts',(-6.390311350216,13.724648700715,8.13903540228875));
#42013=CARTESIAN_POINT('Ctrl Pts',(-4.260207566811,13.8218533779545,9.11395898716084));
#42014=CARTESIAN_POINT('Ctrl Pts',(0.0001663376446825,13.9179753162775,
10.089995002773));
#42015=CARTESIAN_POINT('Ctrl Pts',(4.2605402421,13.8218458718956,9.11388276950054));
#42016=CARTESIAN_POINT('Ctrl Pts',(6.39081036315,13.7246259279729,8.13880700099865));
#42017=CARTESIAN_POINT('',(-6.26386060039021,13.9442583526775,8.42071136781886));
#42018=CARTESIAN_POINT('Ctrl Pts',(-6.27159552384944,24.2690121660566,11.8794980574134));
#42019=CARTESIAN_POINT('Ctrl Pts',(-6.27195777359875,24.0278185402074,11.915653438685));
#42020=CARTESIAN_POINT('Ctrl Pts',(-6.27229031327705,23.7878332541021,11.9441024445887));
#42021=CARTESIAN_POINT('Ctrl Pts',(-6.27259314313041,23.5495553889474,11.9652318805794));
#42022=CARTESIAN_POINT('Ctrl Pts',(-6.27289863582021,23.3091823043902,11.9865471114371));
#42023=CARTESIAN_POINT('Ctrl Pts',(-6.27317389390043,23.0705467110858,12.0004135052685));
#42024=CARTESIAN_POINT('Ctrl Pts',(-6.27341891762367,22.8341074530425,12.0072245125909));
#42025=CARTESIAN_POINT('Ctrl Pts',(-6.2736675427923,22.5941929271239,12.014135630509));
#42026=CARTESIAN_POINT('Ctrl Pts',(-6.27388503828152,22.3565397309245,12.0137824613571));
#42027=CARTESIAN_POINT('Ctrl Pts',(-6.27407140435525,22.1215733217137,12.0065719180718));
#42028=CARTESIAN_POINT('Ctrl Pts',(-6.27421804489091,21.9366920318044,12.0008983643582));
#42029=CARTESIAN_POINT('Ctrl Pts',(-6.27434541260364,21.7534730872847,11.9909791988217));
#42030=CARTESIAN_POINT('Ctrl Pts',(-6.27445350762203,21.5721011929276,11.9770107164691));
#42031=CARTESIAN_POINT('Ctrl Pts',(-6.2745026299563,21.4896791631684,11.9706629266297));
#42032=CARTESIAN_POINT('Ctrl Pts',(-6.27454777223563,21.4076383057737,11.963478898258));
#42033=CARTESIAN_POINT('Ctrl Pts',(-6.27458893447209,21.3259943042553,11.9554821771386));
#42034=CARTESIAN_POINT('Ctrl Pts',(-6.27470712627363,21.0915645829234,11.9325206726958));
#42035=CARTESIAN_POINT('Ctrl Pts',(-6.27479250328971,20.8604106337727,11.9028603060025));
#42036=CARTESIAN_POINT('Ctrl Pts',(-6.27484506552035,20.6328684194097,11.8670439018405));
#42037=CARTESIAN_POINT('Ctrl Pts',(-6.27489762775099,20.4053262050468,11.8312274976785));
#42038=CARTESIAN_POINT('Ctrl Pts',(-6.27491737519619,20.1813955353361,11.7892550171273));
#42039=CARTESIAN_POINT('Ctrl Pts',(-6.27490430785594,19.9613622611599,11.7416481083875));
#42040=CARTESIAN_POINT('Ctrl Pts',(-6.27489476770969,19.800721336778,11.7068914659862));
#42041=CARTESIAN_POINT('Ctrl Pts',(-6.27486753862054,19.6418692732658,11.669064473988));
#42042=CARTESIAN_POINT('Ctrl Pts',(-6.27482283777318,19.485219732692,11.6284222396903));
#42043=CARTESIAN_POINT('Ctrl Pts',(-6.27477792003791,19.32781013067,11.5875828098224));
#42044=CARTESIAN_POINT('Ctrl Pts',(-6.27471536058765,19.1726247739736,11.5439009383169));
#42045=CARTESIAN_POINT('Ctrl Pts',(-6.27463537978378,19.0200566298959,11.4976809493562));
#42046=CARTESIAN_POINT('Ctrl Pts',(-6.2745769103504,18.9085227054517,11.4638921346092));
#42047=CARTESIAN_POINT('Ctrl Pts',(-6.27450913052138,18.7983869345835,11.4287478520123));
#42048=CARTESIAN_POINT('Ctrl Pts',(-6.27443212638912,18.6897925869713,11.3923813180313));
#42049=CARTESIAN_POINT('Ctrl Pts',(-6.274356354692,18.5829362693268,11.3565968228697));
#42050=CARTESIAN_POINT('Ctrl Pts',(-6.27427024754847,18.4758583327785,11.3190562070229));
#42051=CARTESIAN_POINT('Ctrl Pts',(-6.27417380495852,18.3686262100774,11.2797074661865));
#42052=CARTESIAN_POINT('Ctrl Pts',(-6.27399075528872,18.1650978243038,11.2050228893736));
#42053=CARTESIAN_POINT('Ctrl Pts',(-6.27377047250067,17.9610111107778,11.1238234851248));
#42054=CARTESIAN_POINT('Ctrl Pts',(-6.27351295659435,17.7568354136725,11.0358411780908));
#42055=CARTESIAN_POINT('Ctrl Pts',(-6.27325823283633,17.5548735169924,10.9488128301787));
#42056=CARTESIAN_POINT('Ctrl Pts',(-6.27296707899227,17.3528244668957,10.8551477982201));
#42057=CARTESIAN_POINT('Ctrl Pts',(-6.27263949506218,17.1511911386934,10.7546004677717));
#42058=CARTESIAN_POINT('Ctrl Pts',(-6.27231699830121,16.9526890472353,10.6556145731159));
#42059=CARTESIAN_POINT('Ctrl Pts',(-6.27195919414059,16.7545898242303,10.5499584205239));
#42060=CARTESIAN_POINT('Ctrl Pts',(-6.27156608258035,16.5574215753287,10.4374120685186));
#42061=CARTESIAN_POINT('Ctrl Pts',(-6.27136275125215,16.4554391205203,10.3791990787438));
#42062=CARTESIAN_POINT('Ctrl Pts',(-6.271149974038,16.3537065297169,10.3191429768495));
#42063=CARTESIAN_POINT('Ctrl Pts',(-6.27092775093789,16.2523021361105,10.2572149522302));
#42064=CARTESIAN_POINT('Ctrl Pts',(-6.27050608269128,16.0598873384097,10.1397065494349));
#42065=CARTESIAN_POINT('Ctrl Pts',(-6.27005040505914,15.8686512520362,10.0154573241263));
#42066=CARTESIAN_POINT('Ctrl Pts',(-6.26956071763076,15.6791659370351,9.88428219016649));
#42067=CARTESIAN_POINT('Ctrl Pts',(-6.2693850513209,15.6111915841536,9.8372255364886));
#42068=CARTESIAN_POINT('Ctrl Pts',(-6.26920500834835,15.5434429948885,9.78927774773558));
#42069=CARTESIAN_POINT('Ctrl Pts',(-6.26902058869414,15.4759481427354,9.74043078888112));
#42070=CARTESIAN_POINT('Ctrl Pts',(-6.26850854120704,15.2885463737326,9.60480553439552));
#42071=CARTESIAN_POINT('Ctrl Pts',(-6.26796275325752,15.1030977555619,9.46224615032455));
#42072=CARTESIAN_POINT('Ctrl Pts',(-6.26738322443976,14.9201595432571,9.31269267423412));
#42073=CARTESIAN_POINT('Ctrl Pts',(-6.26681231188111,14.7399412009397,9.16536271397456));
#42074=CARTESIAN_POINT('Ctrl Pts',(-6.26620865429388,14.5621591566521,9.01124503746522));
#42075=CARTESIAN_POINT('Ctrl Pts',(-6.26557225129009,14.3873869151172,8.85031163435012));
#42076=CARTESIAN_POINT('Ctrl Pts',(-6.2650258403793,14.2373287615404,8.71213540505762));
#42077=CARTESIAN_POINT('Ctrl Pts',(-6.26445529016119,14.0894899890531,8.56893517534428));
#42078=CARTESIAN_POINT('Ctrl Pts',(-6.26386060039021,13.9442583526775,8.42071136781886));
#42079=CARTESIAN_POINT('Ctrl Pts',(6.26385989006508,13.9442649556658,8.42071839528551));
#42080=CARTESIAN_POINT('Ctrl Pts',(5.97553496877593,13.9555618354838,8.54505430197946));
#42081=CARTESIAN_POINT('Ctrl Pts',(5.6853707846613,13.9652272416059,8.6607532436919));
#42082=CARTESIAN_POINT('Ctrl Pts',(5.39385482794471,13.9735175248353,8.76768516072829));
#42083=CARTESIAN_POINT('Ctrl Pts',(5.12004274101568,13.9813043361571,8.86812306365763));
#42084=CARTESIAN_POINT('Ctrl Pts',(4.84503808318898,13.9878781560399,8.96082580983451));
#42085=CARTESIAN_POINT('Ctrl Pts',(4.5692448129743,13.9934626776619,9.04572743851788));
#42086=CARTESIAN_POINT('Ctrl Pts',(4.3128000449903,13.9986554126063,9.12467272406537));
#42087=CARTESIAN_POINT('Ctrl Pts',(4.05567343468833,14.0029929135767,9.1968728374423));
#42088=CARTESIAN_POINT('Ctrl Pts',(3.79818974563082,14.0066630216774,9.26231788137843));
#42089=CARTESIAN_POINT('Ctrl Pts',(3.57801043857143,14.0098014024479,9.31828121046181));
#42090=CARTESIAN_POINT('Ctrl Pts',(3.35757002508127,14.0124518967487,9.36930547712606));
#42091=CARTESIAN_POINT('Ctrl Pts',(3.13707157603067,14.0147362856601,9.41541459537568));
#42092=CARTESIAN_POINT('Ctrl Pts',(2.89171879902103,14.0172781682249,9.46672107964674));
#42093=CARTESIAN_POINT('Ctrl Pts',(2.64632878443407,14.019382025325,9.51194774108423));
#42094=CARTESIAN_POINT('Ctrl Pts',(2.40114096253886,14.0211091486273,9.551085447327));
#42095=CARTESIAN_POINT('Ctrl Pts',(2.15971436100687,14.0228097775822,9.58962277490271));
#42096=CARTESIAN_POINT('Ctrl Pts',(1.91848379641032,14.0241451642015,9.62225648551632));
#42097=CARTESIAN_POINT('Ctrl Pts',(1.67767784848676,14.0251785145865,9.6490282183982));
#42098=CARTESIAN_POINT('Ctrl Pts',(1.43858372990708,14.0262045191416,9.67560963771709));
#42099=CARTESIAN_POINT('Ctrl Pts',(1.19990821247035,14.0269327812144,9.69641204968543));
#42100=CARTESIAN_POINT('Ctrl Pts',(0.961875035736572,14.0274295673342,9.71152720644804));
#42101=CARTESIAN_POINT('Ctrl Pts',(0.725661536800911,14.0279225557033,9.72652681328793));
#42102=CARTESIAN_POINT('Ctrl Pts',(0.490080595180857,14.0281876071765,9.73592574969795));
#42103=CARTESIAN_POINT('Ctrl Pts',(0.25535085833806,14.0282936152756,9.73986490944068));
#42104=CARTESIAN_POINT('Ctrl Pts',(0.170488783179417,14.0283319404891,9.74128903777927));
#42105=CARTESIAN_POINT('Ctrl Pts',(0.0857379644516537,14.0283495164129,
9.74200003828909));
#42106=CARTESIAN_POINT('Ctrl Pts',(0.00110873407505763,14.0283497281836,
9.74200624557126));
#42107=CARTESIAN_POINT('Ctrl Pts',(0.000739158498271593,14.0283497291084,
9.74200627267844));
#42108=CARTESIAN_POINT('Ctrl Pts',(0.000369580473237724,14.0283497297032,
9.74200628634741));
#42109=CARTESIAN_POINT('Ctrl Pts',(8.91737066575231E-13,14.0283497299677,
9.7420062865774));
#42110=CARTESIAN_POINT('Ctrl Pts',(-0.229875715873488,14.0283498944901,
9.74200642962535));
#42111=CARTESIAN_POINT('Ctrl Pts',(-0.460698230103008,14.0282219407555,
9.7368030522104));
#42112=CARTESIAN_POINT('Ctrl Pts',(-0.692242317170722,14.0278986126043,
9.7262389182912));
#42113=CARTESIAN_POINT('Ctrl Pts',(-0.925634833270699,14.0275727033069,
9.71559045031673));
#42114=CARTESIAN_POINT('Ctrl Pts',(-1.15976048890447,14.0270482745718,9.69949530223137));
#42115=CARTESIAN_POINT('Ctrl Pts',(-1.39438862141758,14.0262607078353,9.67784538975412));
#42116=CARTESIAN_POINT('Ctrl Pts',(-1.63050058604344,14.0254681603796,9.65605855918853));
#42117=CARTESIAN_POINT('Ctrl Pts',(-1.86712140316056,14.0244091222216,9.6286465415942));
#42118=CARTESIAN_POINT('Ctrl Pts',(-2.10401600611877,14.0230222437544,9.59555206923531));
#42119=CARTESIAN_POINT('Ctrl Pts',(-2.34376748131239,14.0216186399818,9.56205848825154));
#42120=CARTESIAN_POINT('Ctrl Pts',(-2.58379938570262,14.0198792216485,9.52274461255295));
#42121=CARTESIAN_POINT('Ctrl Pts',(-2.82386804518254,14.017745249659,9.47760437142254));
#42122=CARTESIAN_POINT('Ctrl Pts',(-2.92799179665629,14.0168196929055,9.45802592557663));
#42123=CARTESIAN_POINT('Ctrl Pts',(-3.03212246239736,14.015819976852,9.43735210851414));
#42124=CARTESIAN_POINT('Ctrl Pts',(-3.13624016075678,14.0147416014962,9.41558544311034));
#42125=CARTESIAN_POINT('Ctrl Pts',(-3.39906091201799,14.0120194954027,9.36064059277251));
#42126=CARTESIAN_POINT('Ctrl Pts',(-3.66179324841398,14.0087772393006,9.29871252238622));
#42127=CARTESIAN_POINT('Ctrl Pts',(-3.92409365960145,14.0048094640642,9.22976650998086));
#42128=CARTESIAN_POINT('Ctrl Pts',(-4.19384459535778,14.0007289859664,9.15886211727017));
#42129=CARTESIAN_POINT('Ctrl Pts',(-4.46313872013994,13.9958811280336,9.08053601144839));
#42130=CARTESIAN_POINT('Ctrl Pts',(-4.7316024125131,13.9900514247656,8.99481051658923));
#42131=CARTESIAN_POINT('Ctrl Pts',(-5.02536872517533,13.9836722737607,8.90100542025272));
#42132=CARTESIAN_POINT('Ctrl Pts',(-5.31814069269643,13.9761172542124,8.79834071961033));
#42133=CARTESIAN_POINT('Ctrl Pts',(-5.60942878308013,13.967118242421,8.68691055918608));
#42134=CARTESIAN_POINT('Ctrl Pts',(-5.82848128650871,13.9603508663204,8.60311360213842));
#42135=CARTESIAN_POINT('Ctrl Pts',(-6.04669462191043,13.9527671398283,8.51436109383324));
#42136=CARTESIAN_POINT('Ctrl Pts',(-6.26386060039021,13.9442583526775,8.42071136781886));
#42137=CARTESIAN_POINT('Ctrl Pts',(6.38278051433227,13.9389660638327,8.36834463281926));
#42138=CARTESIAN_POINT('Ctrl Pts',(6.32403324549604,13.9421685246813,8.39503501693572));
#42139=CARTESIAN_POINT('Ctrl Pts',(5.68184080001437,13.9762293289878,8.68229415577496));
#42140=CARTESIAN_POINT('Ctrl Pts',(4.34156912266226,14.0269131243102,9.18193694262902));
#42141=CARTESIAN_POINT('Ctrl Pts',(2.26092021150987,14.0637866398188,9.66364676264392));
#42142=CARTESIAN_POINT('Ctrl Pts',(0.00240395732475112,14.0745321264826,
9.84161531252271));
#42143=CARTESIAN_POINT('Ctrl Pts',(-2.25657178139371,14.063833427226,9.66436170214786));
#42144=CARTESIAN_POINT('Ctrl Pts',(-4.338287360545,14.0270060790976,9.18297638358755));
#42145=CARTESIAN_POINT('Ctrl Pts',(-5.68009484646612,13.9763119235712,8.68302746369451));
#42146=CARTESIAN_POINT('Ctrl Pts',(-6.32334697022109,13.9422059231002,8.39534680690008));
#42147=CARTESIAN_POINT('Ctrl Pts',(-6.38277685455529,13.9389662535686,8.36834631006795));
#42148=CARTESIAN_POINT('Ctrl Pts',(6.17958116000266,13.4711650513731,7.96890660962997));
#42149=CARTESIAN_POINT('Ctrl Pts',(6.1226739972167,13.4744252864521,7.99459326956682));
#42150=CARTESIAN_POINT('Ctrl Pts',(5.50060489987548,13.5091207438235,8.27105239462829));
#42151=CARTESIAN_POINT('Ctrl Pts',(4.2025290500201,13.5611784708113,8.75195270223154));
#42152=CARTESIAN_POINT('Ctrl Pts',(2.1881646903414,13.5997630398516,9.21553749016288));
#42153=CARTESIAN_POINT('Ctrl Pts',(0.00232641633904755,13.61123690215,9.38677394813154));
#42154=CARTESIAN_POINT('Ctrl Pts',(-2.1839555556712,13.5998126299275,9.21622544229542));
#42155=CARTESIAN_POINT('Ctrl Pts',(-4.19935107275343,13.5612746813947,8.75295313615389));
#42156=CARTESIAN_POINT('Ctrl Pts',(-5.49891374142447,13.5092050955935,8.27175816634109));
#42157=CARTESIAN_POINT('Ctrl Pts',(-6.12200921769724,13.4744633603779,7.9948933334426));
#42158=CARTESIAN_POINT('Ctrl Pts',(-6.17957761500318,13.4711652453848,7.96890822259208));
#42159=CARTESIAN_POINT('Ctrl Pts',(6.17623978391479,12.827683761815,8.03328661654028));
#42160=CARTESIAN_POINT('Ctrl Pts',(6.11949336784761,12.8309117803229,8.05865899529169));
#42161=CARTESIAN_POINT('Ctrl Pts',(5.49914553135681,12.8652660029562,8.33176046636725));
#42162=CARTESIAN_POINT('Ctrl Pts',(4.20380863758019,12.9168465271217,8.80737082236057));
#42163=CARTESIAN_POINT('Ctrl Pts',(2.19033539306753,12.9551041637359,9.26687615010052));
#42164=CARTESIAN_POINT('Ctrl Pts',(0.00232951170839197,12.9664788697453,
9.43690573902765));
#42165=CARTESIAN_POINT('Ctrl Pts',(-2.1861248230667,12.9551533347932,9.26755884677766));
#42166=CARTESIAN_POINT('Ctrl Pts',(-4.20063536172209,12.9169418985469,8.80836121435707));
#42167=CARTESIAN_POINT('Ctrl Pts',(-5.49745868616426,12.8653495464233,8.33245792548714));
#42168=CARTESIAN_POINT('Ctrl Pts',(-6.11883046631787,12.8309494760218,8.05895538885718));
#42169=CARTESIAN_POINT('Ctrl Pts',(-6.17623624830767,12.8276839516259,8.03328821131818));
#42170=CARTESIAN_POINT('Ctrl Pts',(6.37340476901101,12.4448304032706,8.51423772060993));
#42171=CARTESIAN_POINT('Ctrl Pts',(6.3150446279235,12.4479587126635,8.54019211278279));
#42172=CARTESIAN_POINT('Ctrl Pts',(5.67700089063687,12.4812342950838,8.81958759200811));
#42173=CARTESIAN_POINT('Ctrl Pts',(4.34341280116177,12.5308239076974,9.30682734629494));
#42174=CARTESIAN_POINT('Ctrl Pts',(2.26536172811636,12.5669539973985,9.77894272739411));
#42175=CARTESIAN_POINT('Ctrl Pts',(0.00241050191523341,12.5774756952153,
9.95406181961986));
#42176=CARTESIAN_POINT('Ctrl Pts',(-2.26101109566215,12.5669998368927,9.77964527734846));
#42177=CARTESIAN_POINT('Ctrl Pts',(-4.34014276397128,12.5309149451459,9.30784321494086));
#42178=CARTESIAN_POINT('Ctrl Pts',(-5.6752653684065,12.481315031728,8.82030142532417));
#42179=CARTESIAN_POINT('Ctrl Pts',(-6.31436287541252,12.4479952405102,8.54049530748422));
#42180=CARTESIAN_POINT('Ctrl Pts',(-6.37340113191404,12.4448305832978,8.51423935521795));
#42181=CARTESIAN_POINT('',(-6.24994613508499,12.4626544380175,8.55169233715956));
#42182=CARTESIAN_POINT('Ctrl Pts',(-6.26386069634234,13.9442581018172,8.42071161317167));
#42183=CARTESIAN_POINT('Ctrl Pts',(-6.25435355654046,13.921854531114,8.40152900018476));
#42184=CARTESIAN_POINT('Ctrl Pts',(-6.24502268537409,13.897989865073,8.38292185729494));
#42185=CARTESIAN_POINT('Ctrl Pts',(-6.23597096179262,13.8726803662576,8.3651180362238));
#42186=CARTESIAN_POINT('Ctrl Pts',(-6.22714672203217,13.8480069343136,8.34776165272734));
#42187=CARTESIAN_POINT('Ctrl Pts',(-6.21858806970101,13.8219601170672,8.33116941791119));
#42188=CARTESIAN_POINT('Ctrl Pts',(-6.21039638859803,13.7946031445368,8.31556098565713));
#42189=CARTESIAN_POINT('Ctrl Pts',(-6.20233097480313,13.7676678548374,8.30019314317934));
#42190=CARTESIAN_POINT('Ctrl Pts',(-6.19462163292192,13.7394623695002,8.28577976268739));
#42191=CARTESIAN_POINT('Ctrl Pts',(-6.18736652633831,13.7100972516111,8.27252821600619));
#42192=CARTESIAN_POINT('Ctrl Pts',(-6.18023889772469,13.6812481021057,8.25950950949774));
#42193=CARTESIAN_POINT('Ctrl Pts',(-6.17355002094219,13.6512798568704,8.24761292078403));
#42194=CARTESIAN_POINT('Ctrl Pts',(-6.16738941348011,13.620345973838,8.23702171420378));
#42195=CARTESIAN_POINT('Ctrl Pts',(-6.16659032270645,13.6163335480056,8.23564793158376));
#42196=CARTESIAN_POINT('Ctrl Pts',(-6.1658001106991,13.6123049414575,8.23429608356915));
#42197=CARTESIAN_POINT('Ctrl Pts',(-6.16501896364319,13.6082605474023,8.23296654294361));
#42198=CARTESIAN_POINT('Ctrl Pts',(-6.15908815391333,13.5775537407484,8.22287208964124));
#42199=CARTESIAN_POINT('Ctrl Pts',(-6.15368082067904,13.5459334635958,8.21406594528197));
#42200=CARTESIAN_POINT('Ctrl Pts',(-6.14887156047967,13.5135955556427,8.20669591986198));
#42201=CARTESIAN_POINT('Ctrl Pts',(-6.14412391166845,13.4816719283307,8.19942031176982));
#42202=CARTESIAN_POINT('Ctrl Pts',(-6.13995938296957,13.449049524448,8.19354481691035));
#42203=CARTESIAN_POINT('Ctrl Pts',(-6.13643647742053,13.4159520378045,8.189177663298));
#42204=CARTESIAN_POINT('Ctrl Pts',(-6.13293425826425,13.3830488985821,8.18483615347701));
#42205=CARTESIAN_POINT('Ctrl Pts',(-6.13006636899709,13.3496769587491,8.18198574296722));
#42206=CARTESIAN_POINT('Ctrl Pts',(-6.12787339203533,13.316081408502,8.1806916287397));
#42207=CARTESIAN_POINT('Ctrl Pts',(-6.12568785535798,13.2825998405052,8.17940190515472));
#42208=CARTESIAN_POINT('Ctrl Pts',(-6.1241727979026,13.2488970071633,8.17965815933266));
#42209=CARTESIAN_POINT('Ctrl Pts',(-6.12334885433878,13.2152293057791,8.18147908566606));
#42210=CARTESIAN_POINT('Ctrl Pts',(-6.1225256521799,13.1815918994312,8.18329837348458));
#42211=CARTESIAN_POINT('Ctrl Pts',(-6.12239236539064,13.1479904376347,8.18667952416076));
#42212=CARTESIAN_POINT('Ctrl Pts',(-6.12294864311801,13.1146814724604,8.191593587105));
#42213=CARTESIAN_POINT('Ctrl Pts',(-6.12350763165346,13.0812101887036,8.19653159686738));
#42214=CARTESIAN_POINT('Ctrl Pts',(-6.12476287848253,13.0480351256725,8.20301730216947));
#42215=CARTESIAN_POINT('Ctrl Pts',(-6.1266928382439,13.0154042565278,8.21097459157634));
#42216=CARTESIAN_POINT('Ctrl Pts',(-6.12863026531057,12.9826471336302,8.21896266893571));
#42217=CARTESIAN_POINT('Ctrl Pts',(-6.13124748503553,12.9504391894584,8.22843331212406));
#42218=CARTESIAN_POINT('Ctrl Pts',(-6.13450288131641,12.9190064842205,8.23926726261598));
#42219=CARTESIAN_POINT('Ctrl Pts',(-6.13779568054161,12.8872126322519,8.25022569001086));
#42220=CARTESIAN_POINT('Ctrl Pts',(-6.14174118213299,12.8562125836447,8.26257835469243));
#42221=CARTESIAN_POINT('Ctrl Pts',(-6.14627889801488,12.826204107595,8.27616627166071));
#42222=CARTESIAN_POINT('Ctrl Pts',(-6.14958305285243,12.8043533232162,8.286060364361));
#42223=CARTESIAN_POINT('Ctrl Pts',(-6.15320081635984,12.7830275102378,8.29660860123681));
#42224=CARTESIAN_POINT('Ctrl Pts',(-6.15710430190698,12.7622886877713,8.30774088573614));
#42225=CARTESIAN_POINT('Ctrl Pts',(-6.16256073867545,12.733299193107,8.32330200559314));
#42226=CARTESIAN_POINT('Ctrl Pts',(-6.1685756007687,12.705458756018,8.34000451766156));
#42227=CARTESIAN_POINT('Ctrl Pts',(-6.17506225395425,12.6788942981287,8.35764310234325));
#42228=CARTESIAN_POINT('Ctrl Pts',(-6.18169729474581,12.651722156092,8.3756851843724));
#42229=CARTESIAN_POINT('Ctrl Pts',(-6.18882560675837,12.6258851317298,8.39470584497923));
#42230=CARTESIAN_POINT('Ctrl Pts',(-6.19634894750703,12.601465159828,8.41447879406655));
#42231=CARTESIAN_POINT('Ctrl Pts',(-6.20398372215225,12.5766834852314,8.43454461527502));
#42232=CARTESIAN_POINT('Ctrl Pts',(-6.2120249611779,12.5533609154971,8.45538439871226));
#42233=CARTESIAN_POINT('Ctrl Pts',(-6.22036981861811,12.5315294058142,8.47676724150478));
#42234=CARTESIAN_POINT('Ctrl Pts',(-6.22891479907769,12.5091743416349,8.49866287904461));
#42235=CARTESIAN_POINT('Ctrl Pts',(-6.23777780844621,12.4883823171592,8.5211272362734));
#42236=CARTESIAN_POINT('Ctrl Pts',(-6.24685350902485,12.4691365256179,8.54392966360548));
#42237=CARTESIAN_POINT('Ctrl Pts',(-6.24788171874652,12.4669561198417,8.54651300990006));
#42238=CARTESIAN_POINT('Ctrl Pts',(-6.24891266659523,12.4647955116567,8.54910071944511));
#42239=CARTESIAN_POINT('Ctrl Pts',(-6.24994620609389,12.4626546405112,8.55169247610414));
#42240=CARTESIAN_POINT('Ctrl Pts',(6.24994601334268,12.4626534654496,8.55169428461515));
#42241=CARTESIAN_POINT('Ctrl Pts',(6.23069497655085,12.4636500190818,8.56008041467674));
#42242=CARTESIAN_POINT('Ctrl Pts',(6.211425284112,12.4646384328761,8.56843158879158));
#42243=CARTESIAN_POINT('Ctrl Pts',(6.19213699687127,12.4656187797136,8.57674767820393));
#42244=CARTESIAN_POINT('Ctrl Pts',(5.88885444681381,12.4810334241091,8.70750707493049));
#42245=CARTESIAN_POINT('Ctrl Pts',(5.58097437610039,12.4944537936397,8.82959653937889));
#42246=CARTESIAN_POINT('Ctrl Pts',(5.26879164882413,12.5061905913634,8.94246194328229));
#42247=CARTESIAN_POINT('Ctrl Pts',(5.13451964215371,12.5112386713645,8.99100615454598));
#42248=CARTESIAN_POINT('Ctrl Pts',(4.99945172301877,12.5159752836543,9.03784334970954));
#42249=CARTESIAN_POINT('Ctrl Pts',(4.86361169851994,12.520425116014,9.08292645927752));
#42250=CARTESIAN_POINT('Ctrl Pts',(4.71266624403642,12.5253697703631,9.13302281702168));
#42251=CARTESIAN_POINT('Ctrl Pts',(4.56077038142756,12.5299567332287,9.1809571968488));
#42252=CARTESIAN_POINT('Ctrl Pts',(4.40795808112894,12.5342112095376,9.22667388688011));
#42253=CARTESIAN_POINT('Ctrl Pts',(4.32197583622981,12.5366050575669,9.25239710176902));
#42254=CARTESIAN_POINT('Ctrl Pts',(4.23570343975212,12.538893643089,9.27741816074338));
#42255=CARTESIAN_POINT('Ctrl Pts',(4.14914956176477,12.5410807812621,9.30172798252948));
#42256=CARTESIAN_POINT('Ctrl Pts',(4.02895850398687,12.5441179005297,9.33548525906989));
#42257=CARTESIAN_POINT('Ctrl Pts',(3.90822293847248,12.5469599285777,9.36787098065101));
#42258=CARTESIAN_POINT('Ctrl Pts',(3.78696267046352,12.5496164712603,9.39886142343057));
#42259=CARTESIAN_POINT('Ctrl Pts',(3.72633253645904,12.5509447426016,9.41435664482034));
#42260=CARTESIAN_POINT('Ctrl Pts',(3.66557122374829,12.5522266313763,9.42950303834137));
#42261=CARTESIAN_POINT('Ctrl Pts',(3.60468130682292,12.5534631219089,9.44429775672225));
#42262=CARTESIAN_POINT('Ctrl Pts',(3.57423634836023,12.5540813671752,9.45169511591269));
#42263=CARTESIAN_POINT('Ctrl Pts',(3.54375923868042,12.5546882621973,9.4590045558101));
#42264=CARTESIAN_POINT('Ctrl Pts',(3.51325030186749,12.5552839216038,9.46622572232529));
#42265=CARTESIAN_POINT('Ctrl Pts',(3.49799583346103,12.5555817513071,9.46983630558289));
#42266=CARTESIAN_POINT('Ctrl Pts',(3.48273340826245,12.5558767720639,9.47342482046282));
#42267=CARTESIAN_POINT('Ctrl Pts',(3.46746306711973,12.5561689974362,9.47699122308885));
#42268=CARTESIAN_POINT('Ctrl Pts',(3.45982789654837,12.5563151101224,9.47877442440187));
#42269=CARTESIAN_POINT('Ctrl Pts',(3.45219074699045,12.5564605239598,9.48055209764942));
#42270=CARTESIAN_POINT('Ctrl Pts',(3.44455162357435,12.5566052405941,9.48232423737314));
#42271=CARTESIAN_POINT('Ctrl Pts',(3.43691250015825,12.5567499572284,9.48409637709687));
#42272=CARTESIAN_POINT('Ctrl Pts',(3.43039508137458,12.5568729052858,9.4856040723575));
#42273=CARTESIAN_POINT('Ctrl Pts',(3.4216283368855,12.5570373005128,9.48762405051808));
#42274=CARTESIAN_POINT('Ctrl Pts',(3.12615752408291,12.5625780107953,9.55570457798095));
#42275=CARTESIAN_POINT('Ctrl Pts',(2.82904436899774,12.5671333706468,9.61510893169583));
#42276=CARTESIAN_POINT('Ctrl Pts',(2.5305765003445,12.5708912511799,9.66564787830496));
#42277=CARTESIAN_POINT('Ctrl Pts',(2.45380963084996,12.5718577898085,9.67864665347041));
#42278=CARTESIAN_POINT('Ctrl Pts',(2.37695303288142,12.5727715296055,9.69105871051769));
#42279=CARTESIAN_POINT('Ctrl Pts',(2.30001138902235,12.5736355847826,9.70288031846971));
#42280=CARTESIAN_POINT('Ctrl Pts',(2.00430329850994,12.5769563886242,9.74831403861067));
#42281=CARTESIAN_POINT('Ctrl Pts',(1.70734002773116,12.579543664529,9.78503027763991));
#42282=CARTESIAN_POINT('Ctrl Pts',(1.40947860217307,12.5814672979525,9.8129598758294));
#42283=CARTESIAN_POINT('Ctrl Pts',(1.11351805136661,12.583378655244,9.84071123453076));
#42284=CARTESIAN_POINT('Ctrl Pts',(0.816670228620736,12.5846347306945,9.85978783707557));
#42285=CARTESIAN_POINT('Ctrl Pts',(0.519277169781786,12.5853002264282,9.87007147871222));
#42286=CARTESIAN_POINT('Ctrl Pts',(0.34720187942253,12.5856852904646,9.87602172054868));
#42287=CARTESIAN_POINT('Ctrl Pts',(0.17494393792049,12.5858725678027,9.87902720484474));
#42288=CARTESIAN_POINT('Ctrl Pts',(0.00256942855689103,12.5858741620931,
9.87905705024713));
#42289=CARTESIAN_POINT('Ctrl Pts',(0.00208301752298114,12.5858741665919,
9.8790571344657));
#42290=CARTESIAN_POINT('Ctrl Pts',(0.00159660556107809,12.585874169612,
9.87905719498614));
#42291=CARTESIAN_POINT('Ctrl Pts',(0.00111019267267243,12.585874171153,
9.87905723180882));
#42292=CARTESIAN_POINT('Ctrl Pts',(-0.295689077035793,12.5858751114415,
9.87907970025826));
#42293=CARTESIAN_POINT('Ctrl Pts',(-0.59216539376131,12.5852965639793,9.87032024515954));
#42294=CARTESIAN_POINT('Ctrl Pts',(-0.887982512549591,12.5841115795841,
9.85287673127805));
#42295=CARTESIAN_POINT('Ctrl Pts',(-1.16622061432549,12.582997013226,9.83646980320515));
#42296=CARTESIAN_POINT('Ctrl Pts',(-1.44387582449546,12.5813459890709,9.81237963964323));
#42297=CARTESIAN_POINT('Ctrl Pts',(-1.72065714500414,12.5791334160587,9.78064720860151));
#42298=CARTESIAN_POINT('Ctrl Pts',(-1.91270535705508,12.5775981943529,9.75862926087877));
#42299=CARTESIAN_POINT('Ctrl Pts',(-2.10433775772286,12.5757815284213,9.73294467202123));
#42300=CARTESIAN_POINT('Ctrl Pts',(-2.29545568635781,12.5736541883739,9.70362171541517));
#42301=CARTESIAN_POINT('Ctrl Pts',(-2.38847948222357,12.5726187373949,9.6893492044635));
#42302=CARTESIAN_POINT('Ctrl Pts',(-2.48138138565884,12.5715096738354,9.67421459522921));
#42303=CARTESIAN_POINT('Ctrl Pts',(-2.57415306840246,12.5703203186287,9.65822585627093));
#42304=CARTESIAN_POINT('Ctrl Pts',(-2.71583889015522,12.5685038724371,9.63380700828738));
#42305=CARTESIAN_POINT('Ctrl Pts',(-2.85721797693568,12.5665035069359,9.6073921841135));
#42306=CARTESIAN_POINT('Ctrl Pts',(-2.99825373023941,12.5643006664828,9.5790023299836));
#42307=CARTESIAN_POINT('Ctrl Pts',(-3.06877160689128,12.5631992462562,9.56480740291865));
#42308=CARTESIAN_POINT('Ctrl Pts',(-3.13920364858881,12.5620471897453,9.55011870466143));
#42309=CARTESIAN_POINT('Ctrl Pts',(-3.20954536092081,12.5608417729686,9.53493913971815));
#42310=CARTESIAN_POINT('Ctrl Pts',(-3.24471621708681,12.5602390645802,9.52734935724652));
#42311=CARTESIAN_POINT('Ctrl Pts',(-3.27986449077428,12.5596230149951,9.51963685722513));
#42312=CARTESIAN_POINT('Ctrl Pts',(-3.31498962206888,12.5589932686438,9.51180200761284));
#42313=CARTESIAN_POINT('Ctrl Pts',(-3.33255218771618,12.5586783954681,9.50788458280669));
#42314=CARTESIAN_POINT('Ctrl Pts',(-3.35010896775377,12.5583600980292,9.50393657054786));
#42315=CARTESIAN_POINT('Ctrl Pts',(-3.36765989244758,12.5580383304446,9.49995801774782));
#42316=CARTESIAN_POINT('Ctrl Pts',(-3.37643535479449,12.5578774466524,9.4979687413478));
#42317=CARTESIAN_POINT('Ctrl Pts',(-3.38520935330468,12.5577156953191,9.49597182980904));
#42318=CARTESIAN_POINT('Ctrl Pts',(-3.39398187927851,12.5575530706168,9.49396728905644));
#42319=CARTESIAN_POINT('Ctrl Pts',(-3.40275440525234,12.5573904459144,9.49196274830384));
#42320=CARTESIAN_POINT('Ctrl Pts',(-3.41264857437856,12.5572058961111,9.48969190419738));
#42321=CARTESIAN_POINT('Ctrl Pts',(-3.42029503089472,12.5570625705361,9.48793078509275));
#42322=CARTESIAN_POINT('Ctrl Pts',(-3.73523036312535,12.5511594064357,9.41539540492774));
#42323=CARTESIAN_POINT('Ctrl Pts',(-4.04684827865571,12.5441153173257,9.33340063046015));
#42324=CARTESIAN_POINT('Ctrl Pts',(-4.35476458587455,12.5357286915261,9.24241813984974));
#42325=CARTESIAN_POINT('Ctrl Pts',(-4.37141519515592,12.5352751837836,9.23749825133756));
#42326=CARTESIAN_POINT('Ctrl Pts',(-4.38805498128561,12.5348177506726,9.23255206914417));
#42327=CARTESIAN_POINT('Ctrl Pts',(-4.40468388372678,12.5343563604153,9.22757966359974));
#42328=CARTESIAN_POINT('Ctrl Pts',(-4.72137612663838,12.5255693273601,9.13288175613993));
#42329=CARTESIAN_POINT('Ctrl Pts',(-5.03412129600066,12.5153470262873,9.02867719447994));
#42330=CARTESIAN_POINT('Ctrl Pts',(-5.34263369729778,12.5034361680417,8.91548494251033));
#42331=CARTESIAN_POINT('Ctrl Pts',(-5.62883951435732,12.4923865087679,8.81047690774881));
#42332=CARTESIAN_POINT('Ctrl Pts',(-5.91140270403815,12.4798837868993,8.69773306331674));
#42333=CARTESIAN_POINT('Ctrl Pts',(-6.19008882563368,12.4657244727602,8.5776282226717));
#42334=CARTESIAN_POINT('Ctrl Pts',(-6.21006122604612,12.4647097272467,8.56902075433024));
#42335=CARTESIAN_POINT('Ctrl Pts',(-6.23001371009115,12.4636864722795,8.5603754643636));
#42336=CARTESIAN_POINT('Ctrl Pts',(-6.24994620609389,12.4626546405112,8.55169247610414));
#42337=CARTESIAN_POINT('Ctrl Pts',(-6.25033451892106,13.9524682946008,8.43424269718798));
#42338=CARTESIAN_POINT('Ctrl Pts',(-6.28964915527219,13.9499438768096,8.41725253533479));
#42339=CARTESIAN_POINT('Ctrl Pts',(-6.41587003176774,13.9456274217175,8.35546025032207));
#42340=CARTESIAN_POINT('Ctrl Pts',(-6.61738868014126,13.9601645971529,8.21564074144287));
#42341=CARTESIAN_POINT('Ctrl Pts',(-6.82546143491885,14.0139067293176,7.99585604153587));
#42342=CARTESIAN_POINT('Ctrl Pts',(-6.97865008580523,14.0972105237428,7.74767876286032));
#42343=CARTESIAN_POINT('Ctrl Pts',(-7.07088219512303,14.1979515509549,7.49741012515146));
#42344=CARTESIAN_POINT('Ctrl Pts',(-7.10309704013408,14.2876054220639,7.30105159475886));
#42345=CARTESIAN_POINT('Ctrl Pts',(-7.10603159331704,14.3411724770656,7.19238285727497));
#42346=CARTESIAN_POINT('Ctrl Pts',(-7.10553695258355,14.3576106538258,7.15978428397002));
#42347=CARTESIAN_POINT('Ctrl Pts',(-6.05203636717249,13.4902976546902,8.02965348203525));
#42348=CARTESIAN_POINT('Ctrl Pts',(-6.08682726586427,13.4878645169164,8.01477622955758));
#42349=CARTESIAN_POINT('Ctrl Pts',(-6.19871067963014,13.4832750812962,7.96062311161307));
#42350=CARTESIAN_POINT('Ctrl Pts',(-6.37826045300425,13.4943571901332,7.83768099576627));
#42351=CARTESIAN_POINT('Ctrl Pts',(-6.56468542531687,13.5396514048005,7.64357855148817));
#42352=CARTESIAN_POINT('Ctrl Pts',(-6.70247684352513,13.611603280852,7.42378168844978));
#42353=CARTESIAN_POINT('Ctrl Pts',(-6.78559032245747,13.6996962165107,7.20196003959929));
#42354=CARTESIAN_POINT('Ctrl Pts',(-6.81459591395992,13.7785918003254,7.02819754060553));
#42355=CARTESIAN_POINT('Ctrl Pts',(-6.81722831460514,13.8258046273339,6.93233707607369));
#42356=CARTESIAN_POINT('Ctrl Pts',(-6.81678408764493,13.8402931100199,6.90361903188319));
#42357=CARTESIAN_POINT('Ctrl Pts',(-6.04019940720743,12.8475122295882,8.08818863513551));
#42358=CARTESIAN_POINT('Ctrl Pts',(-6.08811776273061,12.8443535265405,8.0679992039008));
#42359=CARTESIAN_POINT('Ctrl Pts',(-6.24139727010769,12.8387982128404,7.99491913859305));
#42360=CARTESIAN_POINT('Ctrl Pts',(-6.48332443625395,12.855390802314,7.83181228543884));
#42361=CARTESIAN_POINT('Ctrl Pts',(-6.72998275228084,12.9170968299401,7.57931248656608));
#42362=CARTESIAN_POINT('Ctrl Pts',(-6.90994194479098,13.0119770818171,7.29716053986814));
#42363=CARTESIAN_POINT('Ctrl Pts',(-7.01783236561899,13.1260881497257,7.01412193064447));
#42364=CARTESIAN_POINT('Ctrl Pts',(-7.05558995176488,13.2275881118917,6.79197606898948));
#42365=CARTESIAN_POINT('Ctrl Pts',(-7.05905913300314,13.2884728039491,6.66847100666564));
#42366=CARTESIAN_POINT('Ctrl Pts',(-7.05847594073483,13.3071939532727,6.631342309306));
#42367=CARTESIAN_POINT('Ctrl Pts',(-6.22296948742552,12.4591929883744,8.5705424543499));
#42368=CARTESIAN_POINT('Ctrl Pts',(-6.29279077977321,12.4549825546712,8.54120721875926));
#42369=CARTESIAN_POINT('Ctrl Pts',(-6.51521132942963,12.4484219402862,8.43543016078593));
#42370=CARTESIAN_POINT('Ctrl Pts',(-6.86168798984531,12.4757659175238,8.20227041545799));
#42371=CARTESIAN_POINT('Ctrl Pts',(-7.20973653489465,12.5676491290619,7.84677325666152));
#42372=CARTESIAN_POINT('Ctrl Pts',(-7.46091871314674,12.7042381878061,7.45368528454406));
#42373=CARTESIAN_POINT('Ctrl Pts',(-7.61072991218324,12.8654448707582,7.06115049381582));
#42374=CARTESIAN_POINT('Ctrl Pts',(-7.66328349318344,13.0076307346436,6.75235057956903));
#42375=CARTESIAN_POINT('Ctrl Pts',(-7.66816263515553,13.092970744036,6.57943675512195));
#42376=CARTESIAN_POINT('Ctrl Pts',(-7.667345053712,13.1192454833185,6.5272921268927));
#42377=CARTESIAN_POINT('',(-7.00000965177205,13.9487143132752,6.97711954466479));
#42378=CARTESIAN_POINT('',(-6.99999993499287,12.5220622648568,8.04448038251042));
#42379=CARTESIAN_POINT('Ctrl Pts',(-7.,13.9487143133546,6.97711954466507));
#42380=CARTESIAN_POINT('Ctrl Pts',(-7.,13.846910345019,7.02110369792794));
#42381=CARTESIAN_POINT('Ctrl Pts',(-7.,13.7565099975373,7.06259440190032));
#42382=CARTESIAN_POINT('Ctrl Pts',(-7.,13.6789127775256,7.10068312190857));
#42383=CARTESIAN_POINT('Ctrl Pts',(-7.,13.6401141675198,7.1197274819127));
#42384=CARTESIAN_POINT('Ctrl Pts',(-7.,13.604491505167,7.13788022505646));
#42385=CARTESIAN_POINT('Ctrl Pts',(-7.,13.5720954527481,7.15485418320256));
#42386=CARTESIAN_POINT('Ctrl Pts',(-7.,13.5558974265387,7.16334116227561));
#42387=CARTESIAN_POINT('Ctrl Pts',(-7.,13.540504937586,7.17153231301748));
#42388=CARTESIAN_POINT('Ctrl Pts',(-7.,13.5259184564153,7.17938775396613));
#42389=CARTESIAN_POINT('Ctrl Pts',(-7.,13.51862521583,7.18331547444047));
#42390=CARTESIAN_POINT('Ctrl Pts',(-7.,13.5115334771902,7.1871592674665));
#42391=CARTESIAN_POINT('Ctrl Pts',(-7.,13.5046429162458,7.19091413159631));
#42392=CARTESIAN_POINT('Ctrl Pts',(-7.,13.5011976357736,7.19279156366121));
#42393=CARTESIAN_POINT('Ctrl Pts',(-7.,13.4978026497252,7.19464676350206));
#42394=CARTESIAN_POINT('Ctrl Pts',(-7.,13.4944579155314,7.19647910844843));
#42395=CARTESIAN_POINT('Ctrl Pts',(-7.,13.4911131813377,7.19831145339479));
#42396=CARTESIAN_POINT('Ctrl Pts',(-7.,13.4892957406687,7.19930781525711));
#42397=CARTESIAN_POINT('Ctrl Pts',(-7.,13.4845744203103,7.20190695851936));
#42398=CARTESIAN_POINT('Ctrl Pts',(-7.,13.4090332945757,7.24349325071527));
#42399=CARTESIAN_POINT('Ctrl Pts',(-7.,13.3377847769944,7.28575717229597));
#42400=CARTESIAN_POINT('Ctrl Pts',(-7.,13.2713234786593,7.32831597848984));
#42401=CARTESIAN_POINT('Ctrl Pts',(-7.,13.2048621803243,7.3708747846837));
#42402=CARTESIAN_POINT('Ctrl Pts',(-7.,13.1444944017751,7.41273743687651));
#42403=CARTESIAN_POINT('Ctrl Pts',(-7.,13.0865047257911,7.45589780088873));
#42404=CARTESIAN_POINT('Ctrl Pts',(-7.,12.9705253738232,7.54221852891318));
#42405=CARTESIAN_POINT('Ctrl Pts',(-7.,12.862547855931,7.63579225294218));
#42406=CARTESIAN_POINT('Ctrl Pts',(-7.,12.7672508104679,7.73516747733596));
#42407=CARTESIAN_POINT('Ctrl Pts',(-7.,12.6719537650047,7.83454270172974));
#42408=CARTESIAN_POINT('Ctrl Pts',(-7.,12.5894810238525,7.93953389973554));
#42409=CARTESIAN_POINT('Ctrl Pts',(-7.,12.5220625166805,8.04448025538917));
#42410=CARTESIAN_POINT('Ctrl Pts',(-6.24994601297787,12.4626540898072,8.55169209823018));
#42411=CARTESIAN_POINT('Ctrl Pts',(-6.29982459974781,12.4600703735468,8.52996671717355));
#42412=CARTESIAN_POINT('Ctrl Pts',(-6.34869133122363,12.4586319660299,8.50671213387563));
#42413=CARTESIAN_POINT('Ctrl Pts',(-6.39656316448639,12.4582896059969,8.48199166741002));
#42414=CARTESIAN_POINT('Ctrl Pts',(-6.40601602277147,12.4582220029691,8.47711031964634));
#42415=CARTESIAN_POINT('Ctrl Pts',(-6.41543005269687,12.4581972219153,8.47217168167151));
#42416=CARTESIAN_POINT('Ctrl Pts',(-6.42480532433733,12.4582150091077,8.46717604859161));
#42417=CARTESIAN_POINT('Ctrl Pts',(-6.47308062566086,12.4583065992079,8.44145245342739));
#42418=CARTESIAN_POINT('Ctrl Pts',(-6.52033005210395,12.4595246094188,8.41422082064656));
#42419=CARTESIAN_POINT('Ctrl Pts',(-6.56658748121657,12.4618304449742,8.38551103548151));
#42420=CARTESIAN_POINT('Ctrl Pts',(-6.59417368647316,12.4632055592886,8.36838959052382));
#42421=CARTESIAN_POINT('Ctrl Pts',(-6.62140669136586,12.4649680995324,8.35074167140086));
#42422=CARTESIAN_POINT('Ctrl Pts',(-6.64828936293074,12.4671144548114,8.33256747406087));
#42423=CARTESIAN_POINT('Ctrl Pts',(-6.69395208409199,12.4707602391369,8.30169690736654));
#42424=CARTESIAN_POINT('Ctrl Pts',(-6.73859596814244,12.4755104312674,8.26931746786413));
#42425=CARTESIAN_POINT('Ctrl Pts',(-6.78220333696888,12.481366936842,8.23541025459223));
#42426=CARTESIAN_POINT('Ctrl Pts',(-6.80279898250507,12.4841329490125,8.21939596699677));
#42427=CARTESIAN_POINT('Ctrl Pts',(-6.8231629161368,12.4871460991754,8.20304046823201));
#42428=CARTESIAN_POINT('Ctrl Pts',(-6.84329031163055,12.4904084556441,8.18633971751031));
#42429=CARTESIAN_POINT('Ctrl Pts',(-6.88574258186573,12.4972893478318,8.15111485282334));
#42430=CARTESIAN_POINT('Ctrl Pts',(-6.92714539678634,12.5052775790726,8.11435523631283));
#42431=CARTESIAN_POINT('Ctrl Pts',(-6.96745644081089,12.5143953175279,8.07601416781882));
#42432=CARTESIAN_POINT('Ctrl Pts',(-6.97838520010813,12.5168672348728,8.06561949015891));
#42433=CARTESIAN_POINT('Ctrl Pts',(-6.98923346199965,12.5194222870681,8.05510847215563));
#42434=CARTESIAN_POINT('Ctrl Pts',(-6.99999980168616,12.522061165543,8.04447997453359));
#42435=CARTESIAN_POINT('Ctrl Pts',(-6.26385678721994,13.9442683198787,8.42070161672651));
#42436=CARTESIAN_POINT('Ctrl Pts',(-6.29456573149968,13.9363932840456,8.40064334074902));
#42437=CARTESIAN_POINT('Ctrl Pts',(-6.32505699633266,13.9291033776285,8.37895176101333));
#42438=CARTESIAN_POINT('Ctrl Pts',(-6.35516324043681,13.9224354844605,8.35562224165687));
#42439=CARTESIAN_POINT('Ctrl Pts',(-6.39907920397569,13.9127090319601,8.32159148319051));
#42440=CARTESIAN_POINT('Ctrl Pts',(-6.44217769161159,13.9043059353514,8.28407424509421));
#42441=CARTESIAN_POINT('Ctrl Pts',(-6.48397030176567,13.8972700933008,8.24317315549303));
#42442=CARTESIAN_POINT('Ctrl Pts',(-6.51466304337016,13.8921029290287,8.21313515188801));
#42443=CARTESIAN_POINT('Ctrl Pts',(-6.54465065466862,13.8876732740679,8.1812725167791));
#42444=CARTESIAN_POINT('Ctrl Pts',(-6.5737229708968,13.8840033212243,8.14763063810793));
#42445=CARTESIAN_POINT('Ctrl Pts',(-6.57468303811,13.8838821268423,8.14651966833004));
#42446=CARTESIAN_POINT('Ctrl Pts',(-6.57564210573341,13.883761761447,8.14540675847026));
#42447=CARTESIAN_POINT('Ctrl Pts',(-6.57660016725285,13.8836422247969,8.14429191158571));
#42448=CARTESIAN_POINT('Ctrl Pts',(-6.61458107806282,13.8789033737365,8.10009548032388));
#42449=CARTESIAN_POINT('Ctrl Pts',(-6.65098443579671,13.8754660854848,8.05285328625911));
#42450=CARTESIAN_POINT('Ctrl Pts',(-6.68538366622048,13.8733209517643,8.00276471114971));
#42451=CARTESIAN_POINT('Ctrl Pts',(-6.70990068011011,13.8717920724093,7.96706559007807));
#42452=CARTESIAN_POINT('Ctrl Pts',(-6.73339893888901,13.8709197261176,7.9299209974032));
#42453=CARTESIAN_POINT('Ctrl Pts',(-6.75570905449432,13.8707053657576,7.89140763570644));
#42454=CARTESIAN_POINT('Ctrl Pts',(-6.76177919350137,13.8706470425644,7.88092891550328));
#42455=CARTESIAN_POINT('Ctrl Pts',(-6.76776129395266,13.8706374583745,7.87034888571226));
#42456=CARTESIAN_POINT('Ctrl Pts',(-6.77365257560151,13.8706761862248,7.85966973489397));
#42457=CARTESIAN_POINT('Ctrl Pts',(-6.78330665419541,13.8707396497856,7.8421697463582));
#42458=CARTESIAN_POINT('Ctrl Pts',(-6.79271687941757,13.870932839958,7.82440357172246));
#42459=CARTESIAN_POINT('Ctrl Pts',(-6.80187061891861,13.8712539941027,7.80638101726204));
#42460=CARTESIAN_POINT('Ctrl Pts',(-6.80644748866912,13.8714145711751,7.79736974003183));
#42461=CARTESIAN_POINT('Ctrl Pts',(-6.81096023203815,13.8716071419432,7.78829436541889));
#42462=CARTESIAN_POINT('Ctrl Pts',(-6.81540721630231,13.8718315010089,7.77915614525578));
#42463=CARTESIAN_POINT('Ctrl Pts',(-6.81763070843439,13.8719436805418,7.77458703517423));
#42464=CARTESIAN_POINT('Ctrl Pts',(-6.81983776045167,13.8720638073409,7.77000221353246));
#42465=CARTESIAN_POINT('Ctrl Pts',(-6.82202816541374,13.8721918568295,7.7654018370919));
#42466=CARTESIAN_POINT('Ctrl Pts',(-6.82363152598122,13.8722855881278,7.76203439485721));
#42467=CARTESIAN_POINT('Ctrl Pts',(-6.82564555369224,13.8724098122046,7.75776604668181));
#42468=CARTESIAN_POINT('Ctrl Pts',(-6.82714766435398,13.8725074242894,7.75455631221724));
#42469=CARTESIAN_POINT('Ctrl Pts',(-6.82769763774233,13.8725431633667,7.75338112014642));
#42470=CARTESIAN_POINT('Ctrl Pts',(-6.82817948679385,13.8725750866858,7.75234811836397));
#42471=CARTESIAN_POINT('Ctrl Pts',(-6.8285492302672,13.8725997495507,7.75155420014755));
#42472=CARTESIAN_POINT('Ctrl Pts',(-6.8432998660531,13.8735836558616,7.71988143430211));
#42473=CARTESIAN_POINT('Ctrl Pts',(-6.85781064799793,13.8749528718461,7.6862938725749));
#42474=CARTESIAN_POINT('Ctrl Pts',(-6.87180028490507,13.8767952337077,7.65074685921025));
#42475=CARTESIAN_POINT('Ctrl Pts',(-6.87715735062103,13.8775007311863,7.63713480566915));
#42476=CARTESIAN_POINT('Ctrl Pts',(-6.88243753723721,13.8782756300721,7.6232356727681));
#42477=CARTESIAN_POINT('Ctrl Pts',(-6.88762322762864,13.8791249518407,7.60904793507498));
#42478=CARTESIAN_POINT('Ctrl Pts',(-6.90054947881501,13.881242036682,7.57368248759465));
#42479=CARTESIAN_POINT('Ctrl Pts',(-6.91289098172131,13.8838218102924,7.53652145582424));
#42480=CARTESIAN_POINT('Ctrl Pts',(-6.92437312452421,13.8869285469011,7.49757675561096));
#42481=CARTESIAN_POINT('Ctrl Pts',(-6.93225768998699,13.8890618828635,7.47083418294567));
#42482=CARTESIAN_POINT('Ctrl Pts',(-6.9397363802014,13.8914436322206,7.44325117588539));
#42483=CARTESIAN_POINT('Ctrl Pts',(-6.9467094345203,13.8940939133715,7.41484102592939));
#42484=CARTESIAN_POINT('Ctrl Pts',(-6.95354281588448,13.8966911083736,7.38699994218268));
#42485=CARTESIAN_POINT('Ctrl Pts',(-6.95989068062659,13.8995461624458,7.35836450547703));
#42486=CARTESIAN_POINT('Ctrl Pts',(-6.96564934887637,13.9026776268842,7.328955233001));
#42487=CARTESIAN_POINT('Ctrl Pts',(-6.97355724810228,13.9069778060463,7.28856992984403));
#42488=CARTESIAN_POINT('Ctrl Pts',(-6.98035516208629,13.9117996003484,7.24672344639869));
#42489=CARTESIAN_POINT('Ctrl Pts',(-6.98577699516258,13.9171733320292,7.20351888902676));
#42490=CARTESIAN_POINT('Ctrl Pts',(-6.99119882823886,13.9225470637101,7.16031433165482));
#42491=CARTESIAN_POINT('Ctrl Pts',(-6.99524529417623,13.9284726674529,7.11575137185419));
#42492=CARTESIAN_POINT('Ctrl Pts',(-6.99761122800613,13.9349758788666,7.0699751192112));
#42493=CARTESIAN_POINT('Ctrl Pts',(-6.99918436197109,13.9392999316473,7.03953801361207));
#42494=CARTESIAN_POINT('Ctrl Pts',(-7.00001350599334,13.9438793370277,7.00856523949188));
#42495=CARTESIAN_POINT('Ctrl Pts',(-7.00001296810904,13.9487143133882,6.97711954462543));
#42496=CARTESIAN_POINT('Ctrl Pts',(-6.23413001410206,24.3933910200767,11.8700319068232));
#42497=CARTESIAN_POINT('Ctrl Pts',(-6.23490531438389,23.8924703817557,11.9504777604879));
#42498=CARTESIAN_POINT('Ctrl Pts',(-6.23649310959702,22.7260279288224,12.0627647819659));
#42499=CARTESIAN_POINT('Ctrl Pts',(-6.23803996453712,20.8893409401919,11.9701373429924));
#42500=CARTESIAN_POINT('Ctrl Pts',(-6.23759277150523,18.9411611629796,11.5416381740992));
#42501=CARTESIAN_POINT('Ctrl Pts',(-6.23570360012082,17.0892587227143,10.7961451394149));
#42502=CARTESIAN_POINT('Ctrl Pts',(-6.23204977718706,15.3875854470211,9.75631584382835));
#42503=CARTESIAN_POINT('Ctrl Pts',(-6.22726122721249,14.0755190719303,8.61699454170999));
#42504=CARTESIAN_POINT('Ctrl Pts',(-6.22400168396393,13.3673833256599,7.8135002823412));
#42505=CARTESIAN_POINT('Ctrl Pts',(-6.22266615802228,13.1134096685017,7.49367917896873));
#42506=CARTESIAN_POINT('Ctrl Pts',(-6.72599000738659,24.374566153822,11.7530859083551));
#42507=CARTESIAN_POINT('Ctrl Pts',(-6.72668316439776,23.8785346950644,11.8323453484187));
#42508=CARTESIAN_POINT('Ctrl Pts',(-6.72805142643041,22.7235345615009,11.9427140669528));
#42509=CARTESIAN_POINT('Ctrl Pts',(-6.72941897542137,20.9054832736021,11.8502317181525));
#42510=CARTESIAN_POINT('Ctrl Pts',(-6.72902397759863,18.9767992612483,11.4262601894422));
#42511=CARTESIAN_POINT('Ctrl Pts',(-6.7273679204602,17.1431694184818,10.6891575760481));
#42512=CARTESIAN_POINT('Ctrl Pts',(-6.72416424438668,15.4573960102263,9.66125578100212));
#42513=CARTESIAN_POINT('Ctrl Pts',(-6.71993337962548,14.1564668032532,8.53485925833108));
#42514=CARTESIAN_POINT('Ctrl Pts',(-6.71707886547193,13.4537901856661,7.74006802512467));
#42515=CARTESIAN_POINT('Ctrl Pts',(-6.7158901469348,13.2016825422521,7.42368980520173));
#42516=CARTESIAN_POINT('Ctrl Pts',(-7.02718522254093,24.3100157396903,11.3520761820925));
#42517=CARTESIAN_POINT('Ctrl Pts',(-7.02756391671898,23.83092546813,11.4283598774116));
#42518=CARTESIAN_POINT('Ctrl Pts',(-7.02824882763447,22.7152040919926,11.5344319762806));
#42519=CARTESIAN_POINT('Ctrl Pts',(-7.02897714962795,20.9601377869518,11.4446324087422));
#42520=CARTESIAN_POINT('Ctrl Pts',(-7.02876722583613,19.0974452998546,11.0353399720625));
#42521=CARTESIAN_POINT('Ctrl Pts',(-7.02790268849586,17.3268264235393,10.3242145754422));
#42522=CARTESIAN_POINT('Ctrl Pts',(-7.02622933165022,15.6982356397987,9.33267256354404));
#42523=CARTESIAN_POINT('Ctrl Pts',(-7.0239793056009,14.4407048288934,8.24599539969497));
#42524=CARTESIAN_POINT('Ctrl Pts',(-7.02249262647073,13.7610260792249,7.47887533837767));
#42525=CARTESIAN_POINT('Ctrl Pts',(-7.02184966906143,13.5171517734752,7.17356121380424));
#42526=CARTESIAN_POINT('Ctrl Pts',(-6.99838062545647,24.2298260444632,10.8539091310108));
#42527=CARTESIAN_POINT('Ctrl Pts',(-6.99835912987599,23.7718327257578,10.9268138865563));
#42528=CARTESIAN_POINT('Ctrl Pts',(-6.99821532191765,22.70491909819,11.0282119310016));
#42529=CARTESIAN_POINT('Ctrl Pts',(-6.99814245128683,21.0278311164464,10.9423807653247));
#42530=CARTESIAN_POINT('Ctrl Pts',(-6.99816421467864,19.2468686121879,10.5510777432818));
#42531=CARTESIAN_POINT('Ctrl Pts',(-6.99828068958999,17.5546300565824,9.87141076730067));
#42532=CARTESIAN_POINT('Ctrl Pts',(-6.99850456871779,15.9978504212263,8.92371734687288));
#42533=CARTESIAN_POINT('Ctrl Pts',(-6.9987352349692,14.7957477561672,7.885044829661));
#42534=CARTESIAN_POINT('Ctrl Pts',(-6.99894167922838,14.1458833108553,7.15166848879572));
#42535=CARTESIAN_POINT('Ctrl Pts',(-6.99898903110029,13.9127708057857,6.8598833748166));
#42536=CARTESIAN_POINT('',(-7.0000030891987,24.1259430621517,10.927769589406));
#42537=CARTESIAN_POINT('Origin',(-5.99998370357417,24.1259473086569,10.9277595201361));
#42538=CARTESIAN_POINT('Ctrl Pts',(-7.00001101651647,24.1259401091757,10.9277661762092));
#42539=CARTESIAN_POINT('Ctrl Pts',(-7.00001786894362,23.9375950085174,10.9560764177985));
#42540=CARTESIAN_POINT('Ctrl Pts',(-7.00001802523644,23.7511663645914,10.9791078948017));
#42541=CARTESIAN_POINT('Ctrl Pts',(-7.0000155683334,23.5669992469552,10.9972403495527));
#42542=CARTESIAN_POINT('Ctrl Pts',(-7.00001306404721,23.3792803335476,11.0157225017793));
#42543=CARTESIAN_POINT('Ctrl Pts',(-7.00000784335981,23.1939109276873,11.0291149016377));
#42544=CARTESIAN_POINT('Ctrl Pts',(-7.00000354817182,23.0112027161862,11.0378133545419));
#42545=CARTESIAN_POINT('Ctrl Pts',(-7.00000225617267,22.9562438056513,11.0404298625303));
#42546=CARTESIAN_POINT('Ctrl Pts',(-7.00000104339791,22.901525326951,11.0426216090387));
#42547=CARTESIAN_POINT('Ctrl Pts',(-6.99999999754011,22.8470548580183,11.0443992462048));
#42548=CARTESIAN_POINT('Ctrl Pts',(-6.99999887667154,22.7886776712689,11.0463043786345));
#42549=CARTESIAN_POINT('Ctrl Pts',(-6.99999794691878,22.7305853409417,11.0477338782857));
#42550=CARTESIAN_POINT('Ctrl Pts',(-6.99999718088504,22.672784885931,11.0487021582321));
#42551=CARTESIAN_POINT('Ctrl Pts',(-6.99999462213136,22.4797162023915,11.0519364672786));
#42552=CARTESIAN_POINT('Ctrl Pts',(-6.99999387749987,22.2899077714107,11.0500263120017));
#42553=CARTESIAN_POINT('Ctrl Pts',(-6.99999403436582,22.1035888683532,11.0434957473627));
#42554=CARTESIAN_POINT('Ctrl Pts',(-6.99999406718812,22.0646038986033,11.0421293059511));
#42555=CARTESIAN_POINT('Ctrl Pts',(-6.99999414005244,22.025771533904,11.0405605106518));
#42556=CARTESIAN_POINT('Ctrl Pts',(-6.99999424550263,21.9870936117406,11.0387940509209));
#42557=CARTESIAN_POINT('Ctrl Pts',(-6.99999432423886,21.958214062736,11.0374750927786));
#42558=CARTESIAN_POINT('Ctrl Pts',(-6.99999441864918,21.9301065612872,11.0360814530954));
#42559=CARTESIAN_POINT('Ctrl Pts',(-6.99999453140906,21.901184348489,11.0345337171186));
#42560=CARTESIAN_POINT('Ctrl Pts',(-6.99999463684116,21.8741416641965,11.0330865617547));
#42561=CARTESIAN_POINT('Ctrl Pts',(-6.99999475849241,21.8463866742734,11.0315045689661));
#42562=CARTESIAN_POINT('Ctrl Pts',(-6.9999949035289,21.816624792391,11.0296819396473));
#42563=CARTESIAN_POINT('Ctrl Pts',(-6.99999520368225,21.7550325096593,11.025910004097));
#42564=CARTESIAN_POINT('Ctrl Pts',(-6.99999556267899,21.6935868205477,11.021626914985));
#42565=CARTESIAN_POINT('Ctrl Pts',(-6.99999595372439,21.6322954774274,11.0168388649797));
#42566=CARTESIAN_POINT('Ctrl Pts',(-6.99999673581519,21.5097127911868,11.0072627649692));
#42567=CARTESIAN_POINT('Ctrl Pts',(-6.99999764539657,21.3877474889111,10.9956668213854));
#42568=CARTESIAN_POINT('Ctrl Pts',(-6.99999847634418,21.2664589639591,10.9821001701665));
#42569=CARTESIAN_POINT('Ctrl Pts',(-6.99999902467301,21.1864226357584,10.9731477573148));
#42570=CARTESIAN_POINT('Ctrl Pts',(-6.99999953898571,21.1066809504165,10.9633371977035));
#42571=CARTESIAN_POINT('Ctrl Pts',(-6.99999996276695,21.0272503077224,10.9526825062929));
#42572=CARTESIAN_POINT('Ctrl Pts',(-7.00000126736565,20.7827252950085,10.9198823366822));
#42573=CARTESIAN_POINT('Ctrl Pts',(-7.00000171384875,20.5411518142187,10.8790835349701));
#42574=CARTESIAN_POINT('Ctrl Pts',(-7.0000017064317,20.3030234396079,10.8307721963177));
#42575=CARTESIAN_POINT('Ctrl Pts',(-7.00000169893534,20.0623489134957,10.7819442960097));
#42576=CARTESIAN_POINT('Ctrl Pts',(-7.00000122941436,19.8251935168243,10.7254423532093));
#42577=CARTESIAN_POINT('Ctrl Pts',(-7.00000072342785,19.5920157773719,10.6617527004579));
#42578=CARTESIAN_POINT('Ctrl Pts',(-7.00000046988916,19.4751755477949,10.6298392182077));
#42579=CARTESIAN_POINT('Ctrl Pts',(-7.00000020716688,19.3593332333778,10.5961208093747));
#42580=CARTESIAN_POINT('Ctrl Pts',(-6.99999998766512,19.2445418371312,10.5606572112207));
#42581=CARTESIAN_POINT('Ctrl Pts',(-6.99999993928862,19.2192426968463,10.5528413071195));
#42582=CARTESIAN_POINT('Ctrl Pts',(-6.99999989300543,19.1939945906656,10.5449406307592));
#42583=CARTESIAN_POINT('Ctrl Pts',(-6.99999984878294,19.1687979878635,10.5369559348259));
#42584=CARTESIAN_POINT('Ctrl Pts',(-6.9999996537447,19.0576712367164,10.5017403414804));
#42585=CARTESIAN_POINT('Ctrl Pts',(-6.99999949863667,18.9475464918459,10.4648905456778));
#42586=CARTESIAN_POINT('Ctrl Pts',(-6.99999938184581,18.8384625268113,10.4264702917995));
#42587=CARTESIAN_POINT('Ctrl Pts',(-6.99999932345038,18.7839205442939,10.4072601648604));
#42588=CARTESIAN_POINT('Ctrl Pts',(-6.99999927466556,18.7296387567356,10.3876574234024));
#42589=CARTESIAN_POINT('Ctrl Pts',(-6.9999992354737,18.6756217453312,10.3676698870215));
#42590=CARTESIAN_POINT('Ctrl Pts',(-6.99999921587777,18.648613239629,10.3576761188311));
#42591=CARTESIAN_POINT('Ctrl Pts',(-6.99999919868211,18.6216709279653,10.34758615191));
#42592=CARTESIAN_POINT('Ctrl Pts',(-6.99999918389647,18.5947953751795,10.3374009592937));
#42593=CARTESIAN_POINT('Ctrl Pts',(-6.99999917283135,18.5746825369799,10.3297786739865));
#42594=CARTESIAN_POINT('Ctrl Pts',(-6.9999991626883,18.5536617117961,10.3217399587041));
#42595=CARTESIAN_POINT('Ctrl Pts',(-6.99999915445983,18.5338560065227,10.3140993759427));
#42596=CARTESIAN_POINT('Ctrl Pts',(-6.9999991516931,18.5271965619125,10.3115303163214));
#42597=CARTESIAN_POINT('Ctrl Pts',(-6.99999914913279,18.5206743326982,10.3090066889746));
#42598=CARTESIAN_POINT('Ctrl Pts',(-6.99999914678741,18.5143695538256,10.3065606748832));
#42599=CARTESIAN_POINT('Ctrl Pts',(-6.99999907529418,18.3221833823898,10.231999759582));
#42600=CARTESIAN_POINT('Ctrl Pts',(-6.99999912491852,18.1296184436268,10.1510712626572));
#42601=CARTESIAN_POINT('Ctrl Pts',(-6.99999933315952,17.9371557774712,10.0634928028401));
#42602=CARTESIAN_POINT('Ctrl Pts',(-6.99999947285727,17.8080428721846,10.0047410999078));
#42603=CARTESIAN_POINT('Ctrl Pts',(-6.99999968443228,17.6789770014193,9.94299687733446));
#42604=CARTESIAN_POINT('Ctrl Pts',(-6.99999998816768,17.55011631383,9.87817756873086));
#42605=CARTESIAN_POINT('Ctrl Pts',(-7.00000042903666,17.3630762739412,9.78409297013374));
#42606=CARTESIAN_POINT('Ctrl Pts',(-7.00000106780699,17.1764663325097,9.68352877151032));
#42607=CARTESIAN_POINT('Ctrl Pts',(-7.0000015333121,16.9908081968233,9.57627840680166));
#42608=CARTESIAN_POINT('Ctrl Pts',(-7.00000199134818,16.8081289474422,9.47074887507177));
#42609=CARTESIAN_POINT('Ctrl Pts',(-7.0000022813204,16.6263711747535,9.35874596463026));
#42610=CARTESIAN_POINT('Ctrl Pts',(-7.00000202662872,16.4460793027373,9.24008888867506));
#42611=CARTESIAN_POINT('Ctrl Pts',(-7.00000181209412,16.2942139385447,9.14014040041301));
#42612=CARTESIAN_POINT('Ctrl Pts',(-7.00000121063197,16.1433894203617,9.03547088641571));
#42613=CARTESIAN_POINT('Ctrl Pts',(-6.99999998662461,15.9939582652679,8.92598176502494));
#42614=CARTESIAN_POINT('Ctrl Pts',(-6.99999852881509,15.8159837142825,8.79557872286767));
#42615=CARTESIAN_POINT('Ctrl Pts',(-6.99999617286935,15.6399850843186,8.65833774103931));
#42616=CARTESIAN_POINT('Ctrl Pts',(-6.99999449845862,15.4665283599749,8.51417822432004));
#42617=CARTESIAN_POINT('Ctrl Pts',(-6.99999284827035,15.2955809060811,8.37210415696424));
#42618=CARTESIAN_POINT('Ctrl Pts',(-6.99999186158984,15.127102326539,8.223310223894));
#42619=CARTESIAN_POINT('Ctrl Pts',(-6.99999320068044,14.9616764910547,8.06774693213457));
#42620=CARTESIAN_POINT('Ctrl Pts',(-6.99999413396005,14.8463829026477,7.95932704669855));
#42621=CARTESIAN_POINT('Ctrl Pts',(-6.99999620011851,14.732573021617,7.84761958458279));
#42622=CARTESIAN_POINT('Ctrl Pts',(-6.99999999965513,14.6204569866519,7.73261614629688));
#42623=CARTESIAN_POINT('Ctrl Pts',(-7.00000506883531,14.4708765406778,7.5791834496027));
#42624=CARTESIAN_POINT('Ctrl Pts',(-7.00001329848849,14.3243093935676,7.41988229083372));
#42625=CARTESIAN_POINT('Ctrl Pts',(-7.00001657716699,14.1813266553594,7.25479670165536));
#42626=CARTESIAN_POINT('Ctrl Pts',(-7.00001838080138,14.1026703972017,7.16398144043396));
#42627=CARTESIAN_POINT('Ctrl Pts',(-7.00001867122214,14.0250995430186,7.07141626669052));
#42628=CARTESIAN_POINT('Ctrl Pts',(-7.00001598720713,13.9487143130816,6.97711954471195));
#42629=CARTESIAN_POINT('Origin',(-5.999994980806,24.1259380084193,10.9277770011849));
#42630=CARTESIAN_POINT('Origin',(-6.,24.1259427055443,10.9277790621896));
#42631=CARTESIAN_POINT('Ctrl Pts',(-7.10781850275369,15.2163810752001,5.10138230547117));
#42632=CARTESIAN_POINT('Ctrl Pts',(-7.10965592212001,15.243638120146,5.01817377406916));
#42633=CARTESIAN_POINT('Ctrl Pts',(-7.09650767610584,15.3063332046137,4.83995160005142));
#42634=CARTESIAN_POINT('Ctrl Pts',(-7.01932069430837,15.4151469112539,4.57119042040278));
#42635=CARTESIAN_POINT('Ctrl Pts',(-6.87393092186964,15.5377052608318,4.31264986078896));
#42636=CARTESIAN_POINT('Ctrl Pts',(-6.66554646305825,15.6627867794142,4.09583198591426));
#42637=CARTESIAN_POINT('Ctrl Pts',(-6.44497302456871,15.7638564025997,3.96342727449913));
#42638=CARTESIAN_POINT('Ctrl Pts',(-6.29831085196003,15.8188935726671,3.91388110101737));
#42639=CARTESIAN_POINT('Ctrl Pts',(-6.24287183837156,15.8381896251399,3.89997079786695));
#42640=CARTESIAN_POINT('Ctrl Pts',(-6.8148660709738,14.6693917981612,4.91526501001416));
#42641=CARTESIAN_POINT('Ctrl Pts',(-6.81651061812386,14.6933027372077,4.84219421584678));
#42642=CARTESIAN_POINT('Ctrl Pts',(-6.80473712287996,14.7486587038382,4.68533569305599));
#42643=CARTESIAN_POINT('Ctrl Pts',(-6.73538317691255,14.8455315157831,4.44862592495412));
#42644=CARTESIAN_POINT('Ctrl Pts',(-6.60489820389822,14.9550819895903,4.221513592739));
#42645=CARTESIAN_POINT('Ctrl Pts',(-6.41858679306974,15.0669053982178,4.03209942015559));
#42646=CARTESIAN_POINT('Ctrl Pts',(-6.22251415808462,15.1569461567156,3.91737098109664));
#42647=CARTESIAN_POINT('Ctrl Pts',(-6.09292710476668,15.2057053040373,3.87479263718418));
#42648=CARTESIAN_POINT('Ctrl Pts',(-6.0440630425918,15.2227571048321,3.86287802597435));
#42649=CARTESIAN_POINT('Ctrl Pts',(-7.05538133470317,14.0958527991573,4.73239253440706));
#42650=CARTESIAN_POINT('Ctrl Pts',(-7.05754283669283,14.1268236090183,4.63786043739041));
#42651=CARTESIAN_POINT('Ctrl Pts',(-7.04209110197715,14.1976751412647,4.43640307164316));
#42652=CARTESIAN_POINT('Ctrl Pts',(-6.95206588367742,14.3202071651059,4.13340471860375));
#42653=CARTESIAN_POINT('Ctrl Pts',(-6.78206029032806,14.4587309981229,3.84080046654608));
#42654=CARTESIAN_POINT('Ctrl Pts',(-6.53634720729367,14.6016134734994,3.59312827978541));
#42655=CARTESIAN_POINT('Ctrl Pts',(-6.27298555123814,14.7190635414326,3.43984981302298));
#42656=CARTESIAN_POINT('Ctrl Pts',(-6.09561259560824,14.7842427841826,3.38184915974059));
#42657=CARTESIAN_POINT('Ctrl Pts',(-6.02821751691175,14.8072801448996,3.36552349019884));
#42658=CARTESIAN_POINT('Ctrl Pts',(-7.66703304724494,13.8868460483238,4.67749851121142));
#42659=CARTESIAN_POINT('Ctrl Pts',(-7.67007102559788,13.9305009829184,4.54444214041405));
#42660=CARTESIAN_POINT('Ctrl Pts',(-7.6483805489724,14.0291874424256,4.26262996939523));
#42661=CARTESIAN_POINT('Ctrl Pts',(-7.52318689543652,14.1975988325363,3.83989894765035));
#42662=CARTESIAN_POINT('Ctrl Pts',(-7.28601521757398,14.3874509907575,3.42923973707209));
#42663=CARTESIAN_POINT('Ctrl Pts',(-6.93967854664297,14.5846684088355,3.07710723531338));
#42664=CARTESIAN_POINT('Ctrl Pts',(-6.5628372219494,14.7493950807724,2.85516467155866));
#42665=CARTESIAN_POINT('Ctrl Pts',(-6.30520104433745,14.8425662279459,2.76979835072563));
#42666=CARTESIAN_POINT('Ctrl Pts',(-6.20672728843964,14.8757629841358,2.74564283123929));
#42667=CARTESIAN_POINT('',(-6.26386059984685,15.8144217559904,3.90573753014116));
#42668=CARTESIAN_POINT('',(-6.24994610153646,14.8593869932042,2.76546780225979));
#42669=CARTESIAN_POINT('Ctrl Pts',(-6.26385533697638,15.8144219674758,3.90575676779332));
#42670=CARTESIAN_POINT('Ctrl Pts',(-6.25431920294586,15.785024950916,3.90347124430492));
#42671=CARTESIAN_POINT('Ctrl Pts',(-6.2449664157803,15.7549995043499,3.89974752383157));
#42672=CARTESIAN_POINT('Ctrl Pts',(-6.23589798149847,15.724518813589,3.89443552233759));
#42673=CARTESIAN_POINT('Ctrl Pts',(-6.22705591741019,15.6947989950639,3.88925612133107));
#42674=CARTESIAN_POINT('Ctrl Pts',(-6.21848448219056,15.6646466824088,3.88256606616677));
#42675=CARTESIAN_POINT('Ctrl Pts',(-6.21028344947388,15.6342624944109,3.87425425030962));
#42676=CARTESIAN_POINT('Ctrl Pts',(-6.20220888165538,15.6043468490192,3.86607060769386));
#42677=CARTESIAN_POINT('Ctrl Pts',(-6.19449370857798,15.5742068731115,3.85631421861257));
#42678=CARTESIAN_POINT('Ctrl Pts',(-6.18723461420234,15.5440679323731,3.84491615956717));
#42679=CARTESIAN_POINT('Ctrl Pts',(-6.18010313606172,15.5144588398423,3.83371848052878));
#42680=CARTESIAN_POINT('Ctrl Pts',(-6.1734121821419,15.4848513800312,3.82093591445899));
#42681=CARTESIAN_POINT('Ctrl Pts',(-6.16724990086697,15.4554841750101,3.80654694090074));
#42682=CARTESIAN_POINT('Ctrl Pts',(-6.16645383918201,15.4516904327791,3.80468813082299));
#42683=CARTESIAN_POINT('Ctrl Pts',(-6.16566659105089,15.4479007265279,3.80280257837661));
#42684=CARTESIAN_POINT('Ctrl Pts',(-6.16488833747526,15.4441155924648,3.80089029683913));
#42685=CARTESIAN_POINT('Ctrl Pts',(-6.1589564514681,15.4152651194468,3.78631479542259));
#42686=CARTESIAN_POINT('Ctrl Pts',(-6.15354800793364,15.3866797106104,3.77018240242601));
#42687=CARTESIAN_POINT('Ctrl Pts',(-6.14873760388498,15.3586023645955,3.75252708013633));
#42688=CARTESIAN_POINT('Ctrl Pts',(-6.14398882657536,15.3308847212704,3.73509794257631));
#42689=CARTESIAN_POINT('Ctrl Pts',(-6.1398231365136,15.3036630123238,3.71618466794446));
#42690=CARTESIAN_POINT('Ctrl Pts',(-6.13629903821808,15.2771719432391,3.69586890326284));
#42691=CARTESIAN_POINT('Ctrl Pts',(-6.13279563454213,15.2508364380891,3.67567243917567));
#42692=CARTESIAN_POINT('Ctrl Pts',(-6.1299265293013,15.2252238223815,3.65409012001848));
#42693=CARTESIAN_POINT('Ctrl Pts',(-6.12773230732132,15.2005535737717,3.63124922072373));
#42694=CARTESIAN_POINT('Ctrl Pts',(-6.1255455309916,15.1759670386806,3.60848582741941));
#42695=CARTESIAN_POINT('Ctrl Pts',(-6.12402920434441,15.1523172315261,3.58447280976846));
#42696=CARTESIAN_POINT('Ctrl Pts',(-6.12320396530117,15.129798671608,3.5593782495565));
#42697=CARTESIAN_POINT('Ctrl Pts',(-6.12237946933404,15.107300388244,3.53430628542572));
#42698=CARTESIAN_POINT('Ctrl Pts',(-6.12224486166197,15.0859319388221,3.50815534111493));
#42699=CARTESIAN_POINT('Ctrl Pts',(-6.12279979543817,15.0658542612884,3.48112729768537));
#42700=CARTESIAN_POINT('Ctrl Pts',(-6.12335743311654,15.0456787557289,3.45396756073066));
#42701=CARTESIAN_POINT('Ctrl Pts',(-6.12461130491849,15.0268071072028,3.4259229058496));
#42702=CARTESIAN_POINT('Ctrl Pts',(-6.12653987018332,15.0093608390953,3.3972224952509));
#42703=CARTESIAN_POINT('Ctrl Pts',(-6.12847589670216,14.9918470746782,3.36841104819527));
#42704=CARTESIAN_POINT('Ctrl Pts',(-6.13109169581639,14.9757699798465,3.33893960549484));
#42705=CARTESIAN_POINT('Ctrl Pts',(-6.13434565659836,14.9612050732441,3.30905234390152));
#42706=CARTESIAN_POINT('Ctrl Pts',(-6.13763700560679,14.9464728148933,3.27882167567869));
#42707=CARTESIAN_POINT('Ctrl Pts',(-6.14158104247447,14.9332877444539,3.24816644452735));
#42708=CARTESIAN_POINT('Ctrl Pts',(-6.14611728449022,14.9216772847504,3.21733891367305));
#42709=CARTESIAN_POINT('Ctrl Pts',(-6.14942119404141,14.9132209659352,3.19488610509814));
#42710=CARTESIAN_POINT('Ctrl Pts',(-6.15303886477687,14.9055988304255,3.17234191617605));
#42711=CARTESIAN_POINT('Ctrl Pts',(-6.15694239071124,14.8988051599248,3.1497998363808));
#42712=CARTESIAN_POINT('Ctrl Pts',(-6.1623975114312,14.889311104208,3.11829760772158));
#42713=CARTESIAN_POINT('Ctrl Pts',(-6.16841114256548,14.8814366026319,3.08680088533039));
#42714=CARTESIAN_POINT('Ctrl Pts',(-6.17489884345628,14.8751254512654,3.05554519947911));
#42715=CARTESIAN_POINT('Ctrl Pts',(-6.18153496518978,14.8686699180261,3.02357446906709));
#42716=CARTESIAN_POINT('Ctrl Pts',(-6.1886667428536,14.8638495759053,2.99185656839097));
#42717=CARTESIAN_POINT('Ctrl Pts',(-6.19619836197334,14.8605615026144,2.96061010749823));
#42718=CARTESIAN_POINT('Ctrl Pts',(-6.20384154406425,14.8572247243612,2.92890080482331));
#42719=CARTESIAN_POINT('Ctrl Pts',(-6.21189614733935,14.8554652284595,2.89767739372793));
#42720=CARTESIAN_POINT('Ctrl Pts',(-6.22026195312469,14.8551414242366,2.86712645708341));
#42721=CARTESIAN_POINT('Ctrl Pts',(-6.2288284005593,14.8548098540417,2.83584280078556));
#42722=CARTESIAN_POINT('Ctrl Pts',(-6.23772083042933,14.8559828945091,2.80526447799116));
#42723=CARTESIAN_POINT('Ctrl Pts',(-6.24683682053218,14.8584845581957,2.77554348983372));
#42724=CARTESIAN_POINT('Ctrl Pts',(-6.24787035040546,14.8587681855498,2.77217385814505));
#42725=CARTESIAN_POINT('Ctrl Pts',(-6.24890676222108,14.8590688735896,2.76881519519068));
#42726=CARTESIAN_POINT('Ctrl Pts',(-6.24994591350264,14.8593863538791,2.76546768326257));
#42727=CARTESIAN_POINT('',(-7.00000135336451,14.5427413789166,3.16613017331584));
#42728=CARTESIAN_POINT('Ctrl Pts',(-7.00000153559549,14.542740500495,3.1661294352437));
#42729=CARTESIAN_POINT('Ctrl Pts',(-6.97364721274325,14.5565707108292,3.14316239933483));
#42730=CARTESIAN_POINT('Ctrl Pts',(-6.94679740601726,14.5702605952016,3.12104432197344));
#42731=CARTESIAN_POINT('Ctrl Pts',(-6.91946606855886,14.5838156764254,3.09975876986723));
#42732=CARTESIAN_POINT('Ctrl Pts',(-6.87663067475657,14.6050600536216,3.06639871172313));
#42733=CARTESIAN_POINT('Ctrl Pts',(-6.8326149259663,14.6259733629431,3.03508153386991));
#42734=CARTESIAN_POINT('Ctrl Pts',(-6.78747034343769,14.6465723854995,3.00575805068263));
#42735=CARTESIAN_POINT('Ctrl Pts',(-6.74232576090909,14.667171408056,2.97643456749534));
#42736=CARTESIAN_POINT('Ctrl Pts',(-6.6960516690935,14.6874563967845,2.94910431005622));
#42737=CARTESIAN_POINT('Ctrl Pts',(-6.6486547929194,14.7074421527635,2.9237597194014));
#42738=CARTESIAN_POINT('Ctrl Pts',(-6.6036789888132,14.7264070196151,2.89970975163018));
#42739=CARTESIAN_POINT('Ctrl Pts',(-6.55771201090129,14.7450958926099,2.87744892165356));
#42740=CARTESIAN_POINT('Ctrl Pts',(-6.51072378439587,14.7635200977768,2.85700612744214));
#42741=CARTESIAN_POINT('Ctrl Pts',(-6.5037844957592,14.7662410108025,2.85398710629316));
#42742=CARTESIAN_POINT('Ctrl Pts',(-6.4968228884971,14.7689561396818,2.8510078161327));
#42743=CARTESIAN_POINT('Ctrl Pts',(-6.48983882057931,14.7716655077748,2.84806843498458));
#42744=CARTESIAN_POINT('Ctrl Pts',(-6.44329065809342,14.7897231938838,2.82847773327587));
#42745=CARTESIAN_POINT('Ctrl Pts',(-6.39574608919368,14.8075257294178,2.81065598168833));
#42746=CARTESIAN_POINT('Ctrl Pts',(-6.34718915281274,14.8250699566923,2.79466001873052));
#42747=CARTESIAN_POINT('Ctrl Pts',(-6.31521652086591,14.8366220677448,2.78412737243107));
#42748=CARTESIAN_POINT('Ctrl Pts',(-6.28280457428078,14.8480620193034,2.77438725400823));
#42749=CARTESIAN_POINT('Ctrl Pts',(-6.24994591350294,14.859386353879,2.76546768326265));
#42750=CARTESIAN_POINT('',(-7.000010673752,14.7967990005536,4.92966193792747));
#42751=CARTESIAN_POINT('Ctrl Pts',(-7.000010673752,14.7967990005536,4.92966193792747));
#42752=CARTESIAN_POINT('Ctrl Pts',(-7.,14.7621679284434,4.84253808279512));
#42753=CARTESIAN_POINT('Ctrl Pts',(-7.,14.7150272228418,4.71628322423078));
#42754=CARTESIAN_POINT('Ctrl Pts',(-7.,14.675095371086,4.59667475186774));
#42755=CARTESIAN_POINT('Ctrl Pts',(-7.,14.6500761041033,4.51841274500377));
#42756=CARTESIAN_POINT('Ctrl Pts',(-7.,14.6389581414002,4.48205932201662));
#42757=CARTESIAN_POINT('Ctrl Pts',(-7.,14.5814663764124,4.28359371296804));
#42758=CARTESIAN_POINT('Ctrl Pts',(-7.,14.5473293834115,4.12815295854409));
#42759=CARTESIAN_POINT('Ctrl Pts',(-7.,14.4827650476056,3.68737356277082));
#42760=CARTESIAN_POINT('Ctrl Pts',(-7.,14.4884094371492,3.41567493764516));
#42761=CARTESIAN_POINT('Ctrl Pts',(-7.000002992025,14.5427411067738,3.16613061790934));
#42762=CARTESIAN_POINT('Ctrl Pts',(-7.00001531363849,14.7967990006772,4.92966193758492));
#42763=CARTESIAN_POINT('Ctrl Pts',(-7.00001196691825,14.8230711151817,4.89380607408238));
#42764=CARTESIAN_POINT('Ctrl Pts',(-6.99838322945502,14.8490064611586,4.85901685982402));
#42765=CARTESIAN_POINT('Ctrl Pts',(-6.99539548218125,14.8744859668073,4.82539406693647));
#42766=CARTESIAN_POINT('Ctrl Pts',(-6.99268063643135,14.8976381685438,4.79484238769247));
#42767=CARTESIAN_POINT('Ctrl Pts',(-6.98884285920536,14.9204144722212,4.76525326760272));
#42768=CARTESIAN_POINT('Ctrl Pts',(-6.98405836242474,14.9427429789628,4.73667880819996));
#42769=CARTESIAN_POINT('Ctrl Pts',(-6.97840508154729,14.9691259667611,4.70291570785058));
#42770=CARTESIAN_POINT('Ctrl Pts',(-6.97143143614919,14.9948834812303,4.6705691487042));
#42771=CARTESIAN_POINT('Ctrl Pts',(-6.96343343703202,15.0199262617575,4.63966369249073));
#42772=CARTESIAN_POINT('Ctrl Pts',(-6.95719888415003,15.0394474616503,4.61557245438453));
#42773=CARTESIAN_POINT('Ctrl Pts',(-6.95034087929794,15.0585349151722,4.5923562821223));
#42774=CARTESIAN_POINT('Ctrl Pts',(-6.94298351534871,15.0771558467909,4.57001569283416));
#42775=CARTESIAN_POINT('Ctrl Pts',(-6.93534008828234,15.0965007825202,4.5468064746927));
#42776=CARTESIAN_POINT('Ctrl Pts',(-6.9271576586673,15.1153422373258,4.52454227767355));
#42777=CARTESIAN_POINT('Ctrl Pts',(-6.91856206152671,15.1336516857214,4.50321362637874));
#42778=CARTESIAN_POINT('Ctrl Pts',(-6.9082791173002,15.1555553456522,4.47769808300178));
#42779=CARTESIAN_POINT('Ctrl Pts',(-6.89740589527407,15.1766974510516,4.4535212602693));
#42780=CARTESIAN_POINT('Ctrl Pts',(-6.88615352910444,15.1970443255629,4.43063595944498));
#42781=CARTESIAN_POINT('Ctrl Pts',(-6.87582437358577,15.215721822187,4.40962830401121));
#42782=CARTESIAN_POINT('Ctrl Pts',(-6.86517521076683,15.2337294687443,4.3897087262134));
#42783=CARTESIAN_POINT('Ctrl Pts',(-6.85434931457902,15.2510499793023,4.37083284180152));
#42784=CARTESIAN_POINT('Ctrl Pts',(-6.84893636648512,15.2597102345813,4.36139489959558));
#42785=CARTESIAN_POINT('Ctrl Pts',(-6.84347895561017,15.2681988269856,4.35221777101534));
#42786=CARTESIAN_POINT('Ctrl Pts',(-6.83799341138776,15.2765142688728,4.34329529706221));
#42787=CARTESIAN_POINT('Ctrl Pts',(-6.83525063927656,15.2806719898164,4.33883406008565));
#42788=CARTESIAN_POINT('Ctrl Pts',(-6.83250082545977,15.2847864234481,4.33443649226567));
#42789=CARTESIAN_POINT('Ctrl Pts',(-6.82974591181241,15.2888574285857,4.33010177679098));
#42790=CARTESIAN_POINT('Ctrl Pts',(-6.82836845498873,15.2908929311545,4.32793441905364));
#42791=CARTESIAN_POINT('Ctrl Pts',(-6.82698972268906,15.2929175766191,4.32578277473141));
#42792=CARTESIAN_POINT('Ctrl Pts',(-6.82560995332809,15.2949313485221,4.32364674161949));
#42793=CARTESIAN_POINT('Ctrl Pts',(-6.82452960127801,15.2965081211809,4.32197423908626));
#42794=CARTESIAN_POINT('Ctrl Pts',(-6.82391451566205,15.2974032632247,4.32102605564055));
#42795=CARTESIAN_POINT('Ctrl Pts',(-6.82267100370107,15.2992022745916,4.31912276492142));
#42796=CARTESIAN_POINT('Ctrl Pts',(-6.82232636696216,15.299700866829,4.31859527187976));
#42797=CARTESIAN_POINT('Ctrl Pts',(-6.82193326309863,15.3002688772549,4.3179945640952));
#42798=CARTESIAN_POINT('Ctrl Pts',(-6.82146776975955,15.3009400278368,4.31728537373772));
#42799=CARTESIAN_POINT('Ctrl Pts',(-6.81268226478646,15.3136070120445,4.30390044448221));
#42800=CARTESIAN_POINT('Ctrl Pts',(-6.80362640832164,15.3261903141844,4.29077930911651));
#42801=CARTESIAN_POINT('Ctrl Pts',(-6.79431173496066,15.338683927426,4.27793151564932));
#42802=CARTESIAN_POINT('Ctrl Pts',(-6.76482331619401,15.3782362428857,4.23725793544894));
#42803=CARTESIAN_POINT('Ctrl Pts',(-6.73274514991914,15.4168880037098,4.19932321819618));
#42804=CARTESIAN_POINT('Ctrl Pts',(-6.69853334234179,15.4544725960513,4.16431783527236));
#42805=CARTESIAN_POINT('Ctrl Pts',(-6.67146117751713,15.4842136810974,4.13661770589096));
#42806=CARTESIAN_POINT('Ctrl Pts',(-6.64305164022627,15.5132870161513,4.11075217063323));
#42807=CARTESIAN_POINT('Ctrl Pts',(-6.61350997411101,15.5416193773585,4.08681697858153));
#42808=CARTESIAN_POINT('Ctrl Pts',(-6.57430874914484,15.57921587788,4.05505543728706));
#42809=CARTESIAN_POINT('Ctrl Pts',(-6.533116155595,15.615507019943,4.02669216937345));
#42810=CARTESIAN_POINT('Ctrl Pts',(-6.49047955248457,15.6503524602336,4.00181647924621));
#42811=CARTESIAN_POINT('Ctrl Pts',(-6.45748266623747,15.6773196889905,3.98256493813914));
#42812=CARTESIAN_POINT('Ctrl Pts',(-6.42361968093473,15.7034214727792,3.96540262136043));
#42813=CARTESIAN_POINT('Ctrl Pts',(-6.38912480969674,15.7286009735068,3.95037176693883));
#42814=CARTESIAN_POINT('Ctrl Pts',(-6.34811700052793,15.7585345875121,3.93250295376041));
#42815=CARTESIAN_POINT('Ctrl Pts',(-6.30621724569481,15.7871646914559,3.91764573687081));
#42816=CARTESIAN_POINT('Ctrl Pts',(-6.26385533697638,15.8144219674758,3.90575676779332));
#42817=CARTESIAN_POINT('Ctrl Pts',(-6.22266866665511,14.5714076353156,3.97375061095509));
#42818=CARTESIAN_POINT('Ctrl Pts',(-6.22400419724087,14.9771431331047,3.92718914139647));
#42819=CARTESIAN_POINT('Ctrl Pts',(-6.22726378222481,16.0460292266971,3.85976019567651));
#42820=CARTESIAN_POINT('Ctrl Pts',(-6.23205231075792,17.7794228547352,3.98190952387196));
#42821=CARTESIAN_POINT('Ctrl Pts',(-6.23570613836487,19.7179580001375,4.44990387151557));
#42822=CARTESIAN_POINT('Ctrl Pts',(-6.23759530667989,21.5545938411779,5.23225344908634));
#42823=CARTESIAN_POINT('Ctrl Pts',(-6.23804249999508,23.235159518522,6.30682982345941));
#42824=CARTESIAN_POINT('Ctrl Pts',(-6.23649564902418,24.5993878927371,7.54006348689315));
#42825=CARTESIAN_POINT('Ctrl Pts',(-6.2349078630626,25.3447858427874,8.4442579151259));
#42826=CARTESIAN_POINT('Ctrl Pts',(-6.23413257076684,25.6421045126576,8.85534255591597));
#42827=CARTESIAN_POINT('Ctrl Pts',(-6.71589047216739,14.5843361710878,4.08565974143756));
#42828=CARTESIAN_POINT('Ctrl Pts',(-6.71707918947188,14.9863176706671,4.04021329281028));
#42829=CARTESIAN_POINT('Ctrl Pts',(-6.7199337157726,16.0451894970697,3.9750781528678));
#42830=CARTESIAN_POINT('Ctrl Pts',(-6.72416456955626,17.7615686381462,4.09849148251139));
#42831=CARTESIAN_POINT('Ctrl Pts',(-6.72736824236877,19.6804267269655,4.56367690614212));
#42832=CARTESIAN_POINT('Ctrl Pts',(-6.7290242968866,21.4982088429253,5.33903867080659));
#42833=CARTESIAN_POINT('Ctrl Pts',(-6.7294192912941,23.1617872950511,6.40303091018955));
#42834=CARTESIAN_POINT('Ctrl Pts',(-6.72805175754339,24.5127355742067,7.62318968102802));
#42835=CARTESIAN_POINT('Ctrl Pts',(-6.72668348409556,25.25139899912,8.51793670641239));
#42836=CARTESIAN_POINT('Ctrl Pts',(-6.72599033859008,25.546099410539,8.92472526281053));
#42837=CARTESIAN_POINT('Ctrl Pts',(-7.02184867857606,14.6305390034327,4.4855963187998));
#42838=CARTESIAN_POINT('Ctrl Pts',(-7.02249163139255,15.0188751615543,4.4421515223094));
#42839=CARTESIAN_POINT('Ctrl Pts',(-7.02397829285082,16.041918560353,4.38032091134352));
#42840=CARTESIAN_POINT('Ctrl Pts',(-7.02622833236719,17.6995247916472,4.5011327717638));
#42841=CARTESIAN_POINT('Ctrl Pts',(-7.02790168554062,19.5522386343259,4.95159427705417));
#42842=CARTESIAN_POINT('Ctrl Pts',(-7.0287662253155,21.3070968346045,5.70076931983152));
#42843=CARTESIAN_POINT('Ctrl Pts',(-7.02897614364903,22.9136327574069,6.72847832494041));
#42844=CARTESIAN_POINT('Ctrl Pts',(-7.02824784119134,24.2181471728286,7.90599723975289));
#42845=CARTESIAN_POINT('Ctrl Pts',(-7.0275628969235,24.9320746794641,8.76993207383052));
#42846=CARTESIAN_POINT('Ctrl Pts',(-7.02718421281456,25.216900126262,9.16263740321616));
#42847=CARTESIAN_POINT('Ctrl Pts',(-6.99898915447974,14.6884801945479,4.98714299553211));
#42848=CARTESIAN_POINT('Ctrl Pts',(-6.99894179717708,15.0596401640139,4.94565491848551));
#42849=CARTESIAN_POINT('Ctrl Pts',(-6.99873531515279,16.0377412527625,4.88660281634937));
#42850=CARTESIAN_POINT('Ctrl Pts',(-6.99850468378134,17.6222097431878,5.00216549828158));
#42851=CARTESIAN_POINT('Ctrl Pts',(-6.99828080391387,19.3931400914782,5.43285456754646));
#42852=CARTESIAN_POINT('Ctrl Pts',(-6.99816433649053,21.0703308732033,6.14885094481258));
#42853=CARTESIAN_POINT('Ctrl Pts',(-6.99814256766934,22.6063548077465,7.13148873843438));
#42854=CARTESIAN_POINT('Ctrl Pts',(-6.99821545499553,23.8529244713798,8.25667503834028));
#42855=CARTESIAN_POINT('Ctrl Pts',(-6.99835921852923,24.5356449909404,9.08279284373535));
#42856=CARTESIAN_POINT('Ctrl Pts',(-6.99838071935911,24.8079420348425,9.45819131628623));
#42857=CARTESIAN_POINT('',(-7.00000355772625,24.7867164860195,9.33251602987461));
#42858=CARTESIAN_POINT('Ctrl Pts',(-7.00001601631107,14.7967990005468,4.92966193771618));
#42859=CARTESIAN_POINT('Ctrl Pts',(-7.00002088955923,15.0161850300475,4.90663940958755));
#42860=CARTESIAN_POINT('Ctrl Pts',(-7.00001598262228,15.234292636829,4.89043247358986));
#42861=CARTESIAN_POINT('Ctrl Pts',(-7.00000988116101,15.4506299520445,4.88069443524321));
#42862=CARTESIAN_POINT('Ctrl Pts',(-7.00000652438984,15.5696497787099,4.87533697005084));
#42863=CARTESIAN_POINT('Ctrl Pts',(-7.0000027908345,15.6881347163888,4.87193754799028));
#42864=CARTESIAN_POINT('Ctrl Pts',(-6.99999999965563,15.8060095355692,4.87043898594988));
#42865=CARTESIAN_POINT('Ctrl Pts',(-6.99999455429069,16.0359738046019,4.86751541222465));
#42866=CARTESIAN_POINT('Ctrl Pts',(-6.99999266088648,16.2636130581478,4.87182596258862));
#42867=CARTESIAN_POINT('Ctrl Pts',(-6.99999257352081,16.4885162719136,4.88291846826979));
#42868=CARTESIAN_POINT('Ctrl Pts',(-6.99999248489009,16.7166760665194,4.89417159256048));
#42869=CARTESIAN_POINT('Ctrl Pts',(-6.99999425322404,16.9420200637692,4.91240447412795));
#42870=CARTESIAN_POINT('Ctrl Pts',(-6.99999619758454,17.1641720473477,4.9371555976089));
#42871=CARTESIAN_POINT('Ctrl Pts',(-6.99999754424877,17.3180345277597,4.95429822757969));
#42872=CARTESIAN_POINT('Ctrl Pts',(-6.99999897835572,17.4703669255095,4.97456784638868));
#42873=CARTESIAN_POINT('Ctrl Pts',(-6.99999998662298,17.6210585491081,4.99781411503021));
#42874=CARTESIAN_POINT('Ctrl Pts',(-7.00000143707717,17.8378376785165,5.03125529615071));
#42875=CARTESIAN_POINT('Ctrl Pts',(-7.00000201440455,18.0512192734557,5.07085505278939));
#42876=CARTESIAN_POINT('Ctrl Pts',(-7.00000210874309,18.2609089454417,5.11608568204281));
#42877=CARTESIAN_POINT('Ctrl Pts',(-7.00000220459579,18.4739641816515,5.1620422725999));
#42878=CARTESIAN_POINT('Ctrl Pts',(-7.00000180216121,18.6832080881582,5.21381192541017));
#42879=CARTESIAN_POINT('Ctrl Pts',(-7.00000129011671,18.8883807481865,5.27086478685517));
#42880=CARTESIAN_POINT('Ctrl Pts',(-7.00000086166942,19.06005658805,5.31860310590722));
#42881=CARTESIAN_POINT('Ctrl Pts',(-7.0000003561918,19.2288829378954,5.37004079520996));
#42882=CARTESIAN_POINT('Ctrl Pts',(-6.99999998816664,19.3947325989926,5.42487991583199));
#42883=CARTESIAN_POINT('Ctrl Pts',(-6.99999970373584,19.522910661253,5.46726271101465));
#42884=CARTESIAN_POINT('Ctrl Pts',(-6.99999950020159,19.6493112372598,5.51167738494756));
#42885=CARTESIAN_POINT('Ctrl Pts',(-6.99999936067768,19.77389027009,5.55798424211543));
#42886=CARTESIAN_POINT('Ctrl Pts',(-6.99999924479276,19.8773623632287,5.5964455090637));
#42887=CARTESIAN_POINT('Ctrl Pts',(-6.99999917321856,19.9795779919129,5.63621218780983));
#42888=CARTESIAN_POINT('Ctrl Pts',(-6.99999913936882,20.0805155479599,5.67720660818328));
#42889=CARTESIAN_POINT('Ctrl Pts',(-6.99999912244395,20.1309843259834,5.69770381837001));
#42890=CARTESIAN_POINT('Ctrl Pts',(-6.99999911499155,20.1811335858475,5.71850796396357));
#42891=CARTESIAN_POINT('Ctrl Pts',(-6.99999911640457,20.230960984313,5.7396095727455));
#42892=CARTESIAN_POINT('Ctrl Pts',(-6.99999911711109,20.2558746835458,5.75016037713646));
#42893=CARTESIAN_POINT('Ctrl Pts',(-6.99999912003616,20.2807079174289,5.76078554732452));
#42894=CARTESIAN_POINT('Ctrl Pts',(-6.99999912511612,20.3054604023376,5.77148390561387));
#42895=CARTESIAN_POINT('Ctrl Pts',(-6.9999991276561,20.3178366447919,5.77683308475855));
#42896=CARTESIAN_POINT('Ctrl Pts',(-6.99999913073492,20.3301927000026,5.78220056092855));
#42897=CARTESIAN_POINT('Ctrl Pts',(-6.99999913434533,20.3425285337603,5.78758618774242));
#42898=CARTESIAN_POINT('Ctrl Pts',(-6.99999913750155,20.3533125335665,5.792294308787));
#42899=CARTESIAN_POINT('Ctrl Pts',(-6.99999914057199,20.3627040147974,5.79641054922249));
#42900=CARTESIAN_POINT('Ctrl Pts',(-6.99999914483718,20.3743145448473,5.80152324163118));
#42901=CARTESIAN_POINT('Ctrl Pts',(-6.99999914545094,20.3759853177563,5.80225896583424));
#42902=CARTESIAN_POINT('Ctrl Pts',(-6.99999914609139,20.3777020071407,5.80301540343862));
#42903=CARTESIAN_POINT('Ctrl Pts',(-6.99999914676447,20.3794753368333,5.80379737398191));
#42904=CARTESIAN_POINT('Ctrl Pts',(-6.99999923697432,20.6171488623564,5.90860230487248));
#42905=CARTESIAN_POINT('Ctrl Pts',(-6.9999995214451,20.8492787949593,6.02101278100693));
#42906=CARTESIAN_POINT('Ctrl Pts',(-6.99999999018436,21.0754662943573,6.14041872107596));
#42907=CARTESIAN_POINT('Ctrl Pts',(-7.00000044364517,21.2942812687163,6.25593265435725));
#42908=CARTESIAN_POINT('Ctrl Pts',(-7.00000106797362,21.5075354204105,6.37799275859144));
#42909=CARTESIAN_POINT('Ctrl Pts',(-7.0000014259355,21.7149354690259,6.50595994064156));
#42910=CARTESIAN_POINT('Ctrl Pts',(-7.00000178766081,21.9245160164487,6.6352725046707));
#42911=CARTESIAN_POINT('Ctrl Pts',(-7.00000187627579,22.128118760899,6.7706170178974));
#42912=CARTESIAN_POINT('Ctrl Pts',(-7.00000131558895,22.3254829787871,6.91136700483684));
#42913=CARTESIAN_POINT('Ctrl Pts',(-7.00000103872953,22.4229387019167,6.98086740315849));
#42914=CARTESIAN_POINT('Ctrl Pts',(-7.00000060480684,22.5188739540238,7.0516862930617));
#42915=CARTESIAN_POINT('Ctrl Pts',(-6.99999997635786,22.6132610013232,7.12375115262203));
#42916=CARTESIAN_POINT('Ctrl Pts',(-6.99999887928546,22.7780308196262,7.24955351804758));
#42917=CARTESIAN_POINT('Ctrl Pts',(-6.99999719588015,22.9380818114236,7.37915178801838));
#42918=CARTESIAN_POINT('Ctrl Pts',(-6.99999590265512,23.0933374636584,7.51215857756211));
#42919=CARTESIAN_POINT('Ctrl Pts',(-6.99999568173278,23.11985987192,7.53488020040196));
#42920=CARTESIAN_POINT('Ctrl Pts',(-6.99999546003951,23.147696016291,7.55895210223158));
#42921=CARTESIAN_POINT('Ctrl Pts',(-6.99999525390297,23.1758122701074,7.58352676073225));
#42922=CARTESIAN_POINT('Ctrl Pts',(-6.9999951203152,23.194033142726,7.59945248558547));
#42923=CARTESIAN_POINT('Ctrl Pts',(-6.9999949932545,23.2123722852666,7.61558859099952));
#42924=CARTESIAN_POINT('Ctrl Pts',(-6.99999487632491,23.230556080559,7.63169544081873));
#42925=CARTESIAN_POINT('Ctrl Pts',(-6.99999457896369,23.2767989164085,7.67265643934869));
#42926=CARTESIAN_POINT('Ctrl Pts',(-6.99999434329156,23.3225495030913,7.71387570898918));
#42927=CARTESIAN_POINT('Ctrl Pts',(-6.99999419421933,23.3678080626012,7.75533994626581));
#42928=CARTESIAN_POINT('Ctrl Pts',(-6.99999365475981,23.5315888152958,7.9053898829985));
#42929=CARTESIAN_POINT('Ctrl Pts',(-6.99999426200986,23.6889267660997,8.05864857927771));
#42930=CARTESIAN_POINT('Ctrl Pts',(-6.99999708873464,23.8398716778354,8.21453805486139));
#42931=CARTESIAN_POINT('Ctrl Pts',(-6.99999738651599,23.8557729713616,8.23096023352509));
#42932=CARTESIAN_POINT('Ctrl Pts',(-6.99999770877531,23.8716033460782,8.24741164560196));
#42933=CARTESIAN_POINT('Ctrl Pts',(-6.99999805665875,23.8873628800275,8.26389164217577));
#42934=CARTESIAN_POINT('Ctrl Pts',(-6.99999863110266,23.9133858732566,8.29110430218429));
#42935=CARTESIAN_POINT('Ctrl Pts',(-6.99999927542236,23.939215707693,8.31839489993074));
#42936=CARTESIAN_POINT('Ctrl Pts',(-6.99999999465542,23.96485275711,8.34576054451061));
#42937=CARTESIAN_POINT('Ctrl Pts',(-7.0000039334845,24.1052522486671,8.49562656546484));
#42938=CARTESIAN_POINT('Ctrl Pts',(-7.00001006472447,24.2398678374837,8.64773959093446));
#42939=CARTESIAN_POINT('Ctrl Pts',(-7.00001375742669,24.3687624704118,8.80155051150861));
#42940=CARTESIAN_POINT('Ctrl Pts',(-7.00001750461739,24.4995590368591,8.95763102344457));
#42941=CARTESIAN_POINT('Ctrl Pts',(-7.0000187420762,24.624464636053,9.11545995264843));
#42942=CARTESIAN_POINT('Ctrl Pts',(-7.00001328590555,24.7435704048451,9.27451056188657));
#42943=CARTESIAN_POINT('Ctrl Pts',(-7.00001262320432,24.7580368766487,9.29382869548516));
#42944=CARTESIAN_POINT('Ctrl Pts',(-7.00001186252464,24.7724178171665,9.31316490733289));
#42945=CARTESIAN_POINT('Ctrl Pts',(-7.00001099700064,24.7867134139178,9.33251829944914));
#42946=CARTESIAN_POINT('',(-6.271594443024,25.5608538793675,8.76071211955143));
#42947=CARTESIAN_POINT('Origin',(-5.9999836234388,24.786713751936,9.3325281284206));
#42948=CARTESIAN_POINT('Ctrl Pts',(-6.26386059990525,15.8144217561051,3.90573753015588));
#42949=CARTESIAN_POINT('Ctrl Pts',(-6.26455152016216,16.0555038764713,3.90327937513647));
#42950=CARTESIAN_POINT('Ctrl Pts',(-6.26520985635303,16.2942788050406,3.90810430739374));
#42951=CARTESIAN_POINT('Ctrl Pts',(-6.26583560901963,16.530319704722,3.91978341537098));
#42952=CARTESIAN_POINT('Ctrl Pts',(-6.26647066279415,16.7698690862652,3.9316361201213));
#42953=CARTESIAN_POINT('Ctrl Pts',(-6.26707215721086,17.0066026034232,3.95054824892746));
#42954=CARTESIAN_POINT('Ctrl Pts',(-6.26764009283606,17.2401276173167,3.97607977054762));
#42955=CARTESIAN_POINT('Ctrl Pts',(-6.26812468264228,17.4393823148746,3.99786448445814));
#42956=CARTESIAN_POINT('Ctrl Pts',(-6.2685848405825,17.6363020702729,4.02446846271191));
#42957=CARTESIAN_POINT('Ctrl Pts',(-6.2690205670085,17.8306725455159,4.05562321069526));
#42958=CARTESIAN_POINT('Ctrl Pts',(-6.26953467303182,18.0600068849417,4.09238215538481));
#42959=CARTESIAN_POINT('Ctrl Pts',(-6.27001476738415,18.285791451733,4.13547485945373));
#42960=CARTESIAN_POINT('Ctrl Pts',(-6.27046085064331,18.5077359124598,4.1843574442804));
#42961=CARTESIAN_POINT('Ctrl Pts',(-6.27062083311881,18.5873336636003,4.20188860414532));
#42962=CARTESIAN_POINT('Ctrl Pts',(-6.27077644104249,18.6664379326915,4.22016468855067));
#42963=CARTESIAN_POINT('Ctrl Pts',(-6.27092767444099,18.7450367717596,4.23916134866817));
#42964=CARTESIAN_POINT('Ctrl Pts',(-6.27136815468887,18.9739626337642,4.29449075103807));
#42965=CARTESIAN_POINT('Ctrl Pts',(-6.27177152427923,19.1985970272609,4.35593090616152));
#42966=CARTESIAN_POINT('Ctrl Pts',(-6.27213778321205,19.4186800525206,4.42289861655494));
#42967=CARTESIAN_POINT('Ctrl Pts',(-6.27250404214487,19.6387630777802,4.48986632694836));
#42968=CARTESIAN_POINT('Ctrl Pts',(-6.27283319042016,19.8542949414132,4.56236165257248));
#42969=CARTESIAN_POINT('Ctrl Pts',(-6.27312522803792,20.0650658349331,4.63982809189077));
#42970=CARTESIAN_POINT('Ctrl Pts',(-6.27334042116275,20.2203761252606,4.69691061870571));
#42971=CARTESIAN_POINT('Ctrl Pts',(-6.27353526359634,20.3728239686049,4.75658573628156));
#42972=CARTESIAN_POINT('Ctrl Pts',(-6.27370997702005,20.5226551340267,4.81874475540076));
#42973=CARTESIAN_POINT('Ctrl Pts',(-6.27388469044377,20.6724862994485,4.88090377451995));
#42974=CARTESIAN_POINT('Ctrl Pts',(-6.27403927485761,20.819701119167,4.94554696496691));
#42975=CARTESIAN_POINT('Ctrl Pts',(-6.27417395194295,20.9645377628287,5.01262254882458));
#42976=CARTESIAN_POINT('Ctrl Pts',(-6.27427013710073,21.0679787853766,5.06052732490076));
#42977=CARTESIAN_POINT('Ctrl Pts',(-6.2743561681526,21.1702066478841,5.1096739270377));
#42978=CARTESIAN_POINT('Ctrl Pts',(-6.27443212585409,21.2713094630014,5.16004914532015));
#42979=CARTESIAN_POINT('Ctrl Pts',(-6.27457884491625,21.4665985505298,5.25735336381305));
#42980=CARTESIAN_POINT('Ctrl Pts',(-6.27469165472654,21.6616525046637,5.36122061383588));
#42981=CARTESIAN_POINT('Ctrl Pts',(-6.27477055528495,21.8559695030929,5.47186397511221));
#42982=CARTESIAN_POINT('Ctrl Pts',(-6.27484862841344,22.0482486997179,5.58134701977672));
#42983=CARTESIAN_POINT('Ctrl Pts',(-6.27489349977326,22.2398063968557,5.6974648751496));
#42984=CARTESIAN_POINT('Ctrl Pts',(-6.27490516936443,22.4301093886222,5.82040615118908));
#42985=CARTESIAN_POINT('Ctrl Pts',(-6.27491664536542,22.6172553899414,5.94130791943928));
#42986=CARTESIAN_POINT('Ctrl Pts',(-6.27489601204765,22.8031879940715,6.06880864561297));
#42987=CARTESIAN_POINT('Ctrl Pts',(-6.27484326941112,22.987353699931,6.20306946046052));
#42988=CARTESIAN_POINT('Ctrl Pts',(-6.27479056684953,23.171379472867,6.33722826115602));
#42989=CARTESIAN_POINT('Ctrl Pts',(-6.27470580374529,23.3536411785372,6.47813698009458));
#42990=CARTESIAN_POINT('Ctrl Pts',(-6.27458898009839,23.5335384062425,6.6259368247621));
#42991=CARTESIAN_POINT('Ctrl Pts',(-6.27454781389771,23.5969304126883,6.67801838724844));
#42992=CARTESIAN_POINT('Ctrl Pts',(-6.27450266675486,23.6600283703807,6.73095544150738));
#42993=CARTESIAN_POINT('Ctrl Pts',(-6.27445353865773,23.7228045290992,6.78475355170387));
#42994=CARTESIAN_POINT('Ctrl Pts',(-6.27431624105701,23.8982441751895,6.9351023721139));
#42995=CARTESIAN_POINT('Ctrl Pts',(-6.27414785113122,24.0711732188781,7.09217876505726));
#42996=CARTESIAN_POINT('Ctrl Pts',(-6.2739483686162,24.2410354064908,7.25599610010402));
#42997=CARTESIAN_POINT('Ctrl Pts',(-6.27375072715775,24.4093299083587,7.41830153833311));
#42998=CARTESIAN_POINT('Ctrl Pts',(-6.27352256437881,24.5746139498349,7.58722414933204));
#42999=CARTESIAN_POINT('Ctrl Pts',(-6.27326388002248,24.7363078687583,7.76274427820177));
#43000=CARTESIAN_POINT('Ctrl Pts',(-6.27300884363477,24.8957215788977,7.93578922097746));
#43001=CARTESIAN_POINT('Ctrl Pts',(-6.27272414043095,25.0516457201638,8.11524696640679));
#43002=CARTESIAN_POINT('Ctrl Pts',(-6.27240977016483,25.2034866584683,8.30106585433031));
#43003=CARTESIAN_POINT('Ctrl Pts',(-6.27215746702584,25.3253491546767,8.45019792488959));
#43004=CARTESIAN_POINT('Ctrl Pts',(-6.27188605493237,25.4445809018636,8.60342669609818));
#43005=CARTESIAN_POINT('Ctrl Pts',(-6.27159553375718,25.5608567073971,8.76070944735613));
#43006=CARTESIAN_POINT('Origin',(-5.999994993362,24.7867196013936,9.33250915082854));
#43007=CARTESIAN_POINT('',(-5.988522466616,25.7188096067786,9.69456809159626));
#43008=CARTESIAN_POINT('Origin',(-5.999994993362,24.7867196013936,9.33250915082854));
#43009=CARTESIAN_POINT('Origin',(-6.,24.7867243682982,9.33251101023601));
#43010=CARTESIAN_POINT('Ctrl Pts',(-5.9884183314302,25.7189877484754,9.69410640762213));
#43011=CARTESIAN_POINT('Ctrl Pts',(-5.98810627261414,25.6713270178884,9.81679904137616));
#43012=CARTESIAN_POINT('Ctrl Pts',(-5.98726405067268,25.5029619480015,10.2439466058636));
#43013=CARTESIAN_POINT('Ctrl Pts',(-5.98726405067174,25.2768814416824,10.7897532303017));
#43014=CARTESIAN_POINT('Ctrl Pts',(-5.98810627263415,25.093894583665,11.2108442548557));
#43015=CARTESIAN_POINT('Ctrl Pts',(-5.98841833146804,25.0408390141729,11.331302278264));
#43016=CARTESIAN_POINT('Ctrl Pts',(-6.58019637231563,25.7253769308084,9.69658812202776));
#43017=CARTESIAN_POINT('Ctrl Pts',(-6.57988216494696,25.6778801590244,9.81936871653832));
#43018=CARTESIAN_POINT('Ctrl Pts',(-6.57903377367882,25.5099484810601,10.2467760957568));
#43019=CARTESIAN_POINT('Ctrl Pts',(-6.57903377367798,25.283822418076,10.7926927037156));
#43020=CARTESIAN_POINT('Ctrl Pts',(-6.57988216496595,25.1003453889219,11.213660990656));
#43021=CARTESIAN_POINT('Ctrl Pts',(-6.58019637235286,25.047111685395,11.3340652753282));
#43022=CARTESIAN_POINT('Ctrl Pts',(-7.0007967699024,25.3372908820844,9.54584601718842));
#43023=CARTESIAN_POINT('Ctrl Pts',(-7.00061248525782,25.2904141391226,9.6673928911595));
#43024=CARTESIAN_POINT('Ctrl Pts',(-7.00011448478284,25.1245686183319,10.0904742410697));
#43025=CARTESIAN_POINT('Ctrl Pts',(-7.0001144847828,24.90079560249,10.6307100907232));
#43026=CARTESIAN_POINT('Ctrl Pts',(-7.00061248526902,24.7189024021122,11.0471442770885));
#43027=CARTESIAN_POINT('Ctrl Pts',(-7.00079676992375,24.6661026441675,11.1662377629661));
#43028=CARTESIAN_POINT('Ctrl Pts',(-6.99999917319424,24.7856430606076,9.33157252305582));
#43029=CARTESIAN_POINT('Ctrl Pts',(-6.99999957777252,24.7394735071848,9.45129807054518));
#43030=CARTESIAN_POINT('Ctrl Pts',(-7.00000004362271,24.576125663887,9.86804157212209));
#43031=CARTESIAN_POINT('Ctrl Pts',(-7.00000004362353,24.3557042217843,10.4001860069831));
#43032=CARTESIAN_POINT('Ctrl Pts',(-6.99999957777277,24.1765264322708,10.8103725330858));
#43033=CARTESIAN_POINT('Ctrl Pts',(-6.99999917319347,24.124514488149,10.9276780880777));
#43034=CARTESIAN_POINT('Origin',(-5.98852353411271,-11.4730434368695,-4.75229019548653));
#43035=CARTESIAN_POINT('Origin',(-7.00021006967891,-11.450461588713,-4.74293652086132));
#43036=CARTESIAN_POINT('Ctrl Pts',(-6.05501399426344,25.843213493296,9.37211836695523));
#43037=CARTESIAN_POINT('Ctrl Pts',(-4.03667599617529,26.0304542939164,8.81551147064258));
#43038=CARTESIAN_POINT('Ctrl Pts',(7.59696559070322E-7,26.2482747367075,
8.27054054754906));
#43039=CARTESIAN_POINT('Ctrl Pts',(4.03667751556894,26.030454211933,8.81551167576954));
#43040=CARTESIAN_POINT('Ctrl Pts',(6.05501627335339,25.8432132818694,9.37211899547316));
#43041=CARTESIAN_POINT('Ctrl Pts',(-6.05501399426344,25.5527964585656,10.139984230889));
#43042=CARTESIAN_POINT('Ctrl Pts',(-4.03667599617529,25.6069283663818,9.95057478849123));
#43043=CARTESIAN_POINT('Ctrl Pts',(7.59696559070322E-7,25.7965044905289,
9.81338314348819));
#43044=CARTESIAN_POINT('Ctrl Pts',(4.03667751556894,25.6069282950242,9.95057484012904));
#43045=CARTESIAN_POINT('Ctrl Pts',(6.05501627335339,25.5527963974361,10.1399844447668));
#43046=CARTESIAN_POINT('Ctrl Pts',(-6.05501399426344,25.238357418666,10.8990899687285));
#43047=CARTESIAN_POINT('Ctrl Pts',(-4.03667599617529,25.1425814619013,11.0715782717953));
#43048=CARTESIAN_POINT('Ctrl Pts',(7.59696559951561E-7,25.1794745731306,
11.3029082164588));
#43049=CARTESIAN_POINT('Ctrl Pts',(4.03667751556894,25.1425814480204,11.0715781847256));
#43050=CARTESIAN_POINT('Ctrl Pts',(6.05501627335339,25.2383575268156,10.8990897739563));
#43051=CARTESIAN_POINT('Ctrl Pts',(-6.05501399426344,24.9007381290703,11.6474034030455));
#43052=CARTESIAN_POINT('Ctrl Pts',(-4.03667599617529,24.639428484335,12.17365751233));
#43053=CARTESIAN_POINT('Ctrl Pts',(7.59696559951561E-7,24.4078900068987,
12.7132715562852));
#43054=CARTESIAN_POINT('Ctrl Pts',(4.03667751556894,24.6394285714926,12.1736573092234));
#43055=CARTESIAN_POINT('Ctrl Pts',(6.05501627335339,24.9007384241377,11.647402808804));
#43056=CARTESIAN_POINT('Ctrl Pts',(-5.98852262876833,25.7188097475182,9.69456765113316));
#43057=CARTESIAN_POINT('Ctrl Pts',(-5.94974655199935,25.7233178563395,9.68173306451428));
#43058=CARTESIAN_POINT('Ctrl Pts',(-5.90268839887375,25.7287701868352,9.66624531862473));
#43059=CARTESIAN_POINT('Ctrl Pts',(-5.84725019936459,25.7351158736154,9.64828911090958));
#43060=CARTESIAN_POINT('Ctrl Pts',(-5.7979319987961,25.7407610398751,9.63231514600116));
#43061=CARTESIAN_POINT('Ctrl Pts',(-5.74198182700145,25.7471137839668,9.61438660928848));
#43062=CARTESIAN_POINT('Ctrl Pts',(-5.67933070964221,25.7541280730545,9.59466621125991));
#43063=CARTESIAN_POINT('Ctrl Pts',(-5.62086563255419,25.7606737017603,9.57626343347167));
#43064=CARTESIAN_POINT('Ctrl Pts',(-5.55656514377058,25.7677957313199,9.55629965427607));
#43065=CARTESIAN_POINT('Ctrl Pts',(-5.48637319134976,25.7754414992881,9.53494806705986));
#43066=CARTESIAN_POINT('Ctrl Pts',(-5.42062866343296,25.782602824601,9.51494933539061));
#43067=CARTESIAN_POINT('Ctrl Pts',(-5.34971559674257,25.7902237362974,9.49373286447064));
#43068=CARTESIAN_POINT('Ctrl Pts',(-5.27358793301862,25.7982443243501,9.47148357427303));
#43069=CARTESIAN_POINT('Ctrl Pts',(-5.23094196658891,25.8027373786763,9.45901974133193));
#43070=CARTESIAN_POINT('Ctrl Pts',(-5.18665959187008,25.8073555411599,9.44623259643214));
#43071=CARTESIAN_POINT('Ctrl Pts',(-5.14073271205297,25.8120856159465,9.43316140505069));
#43072=CARTESIAN_POINT('Ctrl Pts',(-5.08889805695584,25.8174241409263,9.41840880919258));
#43073=CARTESIAN_POINT('Ctrl Pts',(-5.03496462672037,25.8229086383713,9.40328537750376));
#43074=CARTESIAN_POINT('Ctrl Pts',(-4.97891809315243,25.8285213367152,9.38784391926512));
#43075=CARTESIAN_POINT('Ctrl Pts',(-4.97191227645643,25.8292229240082,9.38591373698529));
#43076=CARTESIAN_POINT('Ctrl Pts',(-4.9648734425235,25.8299265142188,9.38397858545359));
#43077=CARTESIAN_POINT('Ctrl Pts',(-4.95780155881135,25.8306320663123,9.38203858387997));
#43078=CARTESIAN_POINT('Ctrl Pts',(-4.9507296750992,25.8313376184058,9.38009858230635));
#43079=CARTESIAN_POINT('Ctrl Pts',(-4.9496889160187,25.8314409551873,9.37981464399015));
#43080=CARTESIAN_POINT('Ctrl Pts',(-4.94641136834185,25.8317672566037,9.37891770500492));
#43081=CARTESIAN_POINT('Ctrl Pts',(-4.93985627298814,25.8324198594365,9.37712382703444));
#43082=CARTESIAN_POINT('Ctrl Pts',(-4.93317299793578,25.8330840043494,9.37529867940669));
#43083=CARTESIAN_POINT('Ctrl Pts',(-4.9263614142535,25.8337595501923,9.37344269718707));
#43084=CARTESIAN_POINT('Ctrl Pts',(-4.91273824688894,25.8351106418783,9.36973073274782));
#43085=CARTESIAN_POINT('Ctrl Pts',(-4.8986018450049,25.8365073369903,9.36589542983153));
#43086=CARTESIAN_POINT('Ctrl Pts',(-4.88395128477203,25.837948712664,9.36193973840303));
#43087=CARTESIAN_POINT('Ctrl Pts',(-4.82888918203459,25.8433659236218,9.34707281970699));
#43088=CARTESIAN_POINT('Ctrl Pts',(-4.76656444809351,25.8494139952152,9.33050591088874));
#43089=CARTESIAN_POINT('Ctrl Pts',(-4.69691511772529,25.8560232547324,9.3124519712463));
#43090=CARTESIAN_POINT('Ctrl Pts',(-4.6924371148455,25.8564481875063,9.31129121932976));
#43091=CARTESIAN_POINT('Ctrl Pts',(-4.68792883456788,25.8568754337939,9.31012433765358));
#43092=CARTESIAN_POINT('Ctrl Pts',(-4.68339026042408,25.8573049723977,9.30895139010649));
#43093=CARTESIAN_POINT('Ctrl Pts',(-4.61719980893437,25.8635693526232,9.29184515249631));
#43094=CARTESIAN_POINT('Ctrl Pts',(-4.54456608448041,25.8703224212848,9.27344578850706));
#43095=CARTESIAN_POINT('Ctrl Pts',(-4.46543031231668,25.8774900621148,9.2539735216352));
#43096=CARTESIAN_POINT('Ctrl Pts',(-4.45474238385238,25.8784581101966,9.25134363391598));
#43097=CARTESIAN_POINT('Ctrl Pts',(-4.44393585351717,25.8794336924479,9.24869424872019));
#43098=CARTESIAN_POINT('Ctrl Pts',(-4.4330105765163,25.8804165993201,9.24602597882123));
#43099=CARTESIAN_POINT('Ctrl Pts',(-4.38710136156029,25.8845468820467,9.23481361538715));
#43100=CARTESIAN_POINT('Ctrl Pts',(-4.33909519627864,25.8888067385631,9.22326717421519));
#43101=CARTESIAN_POINT('Ctrl Pts',(-4.28898061558176,25.8931797976848,9.21143417068796));
#43102=CARTESIAN_POINT('Ctrl Pts',(-4.26392332523332,25.8953663272456,9.20551766892434));
#43103=CARTESIAN_POINT('Ctrl Pts',(-4.23833893103118,25.8975811559212,9.19952952600431));
#43104=CARTESIAN_POINT('Ctrl Pts',(-4.2122259637705,25.8998220365003,9.19347619099659));
#43105=CARTESIAN_POINT('Ctrl Pts',(-4.19916948014016,25.9009424767899,9.19044952349273));
#43106=CARTESIAN_POINT('Ctrl Pts',(-4.18598085324542,25.9020694299378,9.18740655792294));
#43107=CARTESIAN_POINT('Ctrl Pts',(-4.17265989938065,25.9032026087186,9.18434811514538));
#43108=CARTESIAN_POINT('Ctrl Pts',(-4.16599942244827,25.903769198109,9.1828188937566));
#43109=CARTESIAN_POINT('Ctrl Pts',(-4.15930586377339,25.9043373438988,9.18128580306261));
#43110=CARTESIAN_POINT('Ctrl Pts',(-4.15257920030619,25.9049070094453,9.17974894750905));
#43111=CARTESIAN_POINT('Ctrl Pts',(-4.14585253683899,25.9054766749918,9.17821209195549));
#43112=CARTESIAN_POINT('Ctrl Pts',(-4.13787834766994,25.906150240868,9.17639538792558));
#43113=CARTESIAN_POINT('Ctrl Pts',(-4.13229987245998,25.9066205284662,9.1751271912668));
#43114=CARTESIAN_POINT('Ctrl Pts',(-4.01426668864598,25.9165711942729,9.14829382126812));
#43115=CARTESIAN_POINT('Ctrl Pts',(-3.89866246388149,25.9259487436324,9.12310703016633));
#43116=CARTESIAN_POINT('Ctrl Pts',(-3.78553933773529,25.9347866014893,9.09944311733136));
#43117=CARTESIAN_POINT('Ctrl Pts',(-3.72757713767392,25.9393149565894,9.08731816554915));
#43118=CARTESIAN_POINT('Ctrl Pts',(-3.67026631241337,25.9437019885214,9.07559218649405));
#43119=CARTESIAN_POINT('Ctrl Pts',(-3.61361387566397,25.9479542173353,9.06424377037705));
#43120=CARTESIAN_POINT('Ctrl Pts',(-3.53000420754008,25.954229806883,9.04749537684419));
#43121=CARTESIAN_POINT('Ctrl Pts',(-3.4478280117861,25.9602100184249,9.03157413172856));
#43122=CARTESIAN_POINT('Ctrl Pts',(-3.36710459947149,25.9659121181529,9.01642319069318));
#43123=CARTESIAN_POINT('Ctrl Pts',(-3.32674289331419,25.9687631680169,9.00884772017549));
#43124=CARTESIAN_POINT('Ctrl Pts',(-3.28674438304887,25.9715446997034,9.00146482919276));
#43125=CARTESIAN_POINT('Ctrl Pts',(-3.24711124803021,25.974258874849,8.99426757532993));
#43126=CARTESIAN_POINT('Ctrl Pts',(-3.21205403583497,25.976659679478,8.98790129479791));
#43127=CARTESIAN_POINT('Ctrl Pts',(-3.17869659599589,25.9789135456954,8.98192974330363));
#43128=CARTESIAN_POINT('Ctrl Pts',(-3.1432884761785,25.9812721261275,8.97568591217661));
#43129=CARTESIAN_POINT('Ctrl Pts',(-3.13866675033491,25.9815799852342,8.97487092183452));
#43130=CARTESIAN_POINT('Ctrl Pts',(-3.13401008629195,25.9818896040878,8.97405136081079));
#43131=CARTESIAN_POINT('Ctrl Pts',(-3.12931014363594,25.9822015197303,8.97322580890466));
#43132=CARTESIAN_POINT('Ctrl Pts',(-2.96648094475864,25.9930078162983,8.94462461834892));
#43133=CARTESIAN_POINT('Ctrl Pts',(-2.80321460460901,26.0030636630445,8.91812930485928));
#43134=CARTESIAN_POINT('Ctrl Pts',(-2.63956869903528,26.0123437147697,8.89376779891749));
#43135=CARTESIAN_POINT('Ctrl Pts',(-2.55774574624841,26.0169837406323,8.8815870459466));
#43136=CARTESIAN_POINT('Ctrl Pts',(-2.47582807006182,26.0214299518029,8.86993939926748));
#43137=CARTESIAN_POINT('Ctrl Pts',(-2.39382320408785,26.0256794517738,8.85882768855804));
#43138=CARTESIAN_POINT('Ctrl Pts',(-2.35282077110086,26.0278042017593,8.85327183320332));
#43139=CARTESIAN_POINT('Ctrl Pts',(-2.3117965406663,26.0298797740671,8.84784996190035));
#43140=CARTESIAN_POINT('Ctrl Pts',(-2.27075145561285,26.0319058064775,8.8425624289481));
#43141=CARTESIAN_POINT('Ctrl Pts',(-2.23483700619109,26.0336785848366,8.83793583761487));
#43142=CARTESIAN_POINT('Ctrl Pts',(-2.19890658995167,26.0354134342236,8.83341209908647));
#43143=CARTESIAN_POINT('Ctrl Pts',(-2.16296083870261,26.0371101115458,8.82899145069237));
#43144=CARTESIAN_POINT('Ctrl Pts',(-2.15782573138132,26.0373524940204,8.82835992949322));
#43145=CARTESIAN_POINT('Ctrl Pts',(-2.15064935712902,26.0376898014891,8.82748121634172));
#43146=CARTESIAN_POINT('Ctrl Pts',(-2.14755457971219,26.0378349211905,8.82710319943079));
#43147=CARTESIAN_POINT('Ctrl Pts',(-2.07171079200998,26.0413913733493,8.81783912952246));
#43148=CARTESIAN_POINT('Ctrl Pts',(-1.98853406425259,26.0450892765804,8.80823185855688));
#43149=CARTESIAN_POINT('Ctrl Pts',(-1.8979985584707,26.0488171805511,8.79857761323498));
#43150=CARTESIAN_POINT('Ctrl Pts',(-1.80788627983242,26.0525276576555,8.78896849870057));
#43151=CARTESIAN_POINT('Ctrl Pts',(-1.71048386265067,26.0562679429853,8.77931284001457));
#43152=CARTESIAN_POINT('Ctrl Pts',(-1.60576582961983,26.0599077783493,8.76995031000074));
#43153=CARTESIAN_POINT('Ctrl Pts',(-1.54093858753986,26.0621610720891,8.76415429777514));
#43154=CARTESIAN_POINT('Ctrl Pts',(-1.47330770039573,26.064375462622,8.7584715702553));
#43155=CARTESIAN_POINT('Ctrl Pts',(-1.40286712366898,26.066515890114,8.75299183003445));
#43156=CARTESIAN_POINT('Ctrl Pts',(-1.2874083954114,26.0700242520217,8.74401002059333));
#43157=CARTESIAN_POINT('Ctrl Pts',(-1.16440227620838,26.0733352030884,8.73557112794578));
#43158=CARTESIAN_POINT('Ctrl Pts',(-1.03383834675618,26.0762729138799,8.72811511444));
#43159=CARTESIAN_POINT('Ctrl Pts',(-0.99560026387569,26.0771332772988,8.72593148176605));
#43160=CARTESIAN_POINT('Ctrl Pts',(-0.956713932107611,26.0779614672454,
8.72383245646009));
#43161=CARTESIAN_POINT('Ctrl Pts',(-0.917179089719602,26.0787526642074,
8.72182982586604));
#43162=CARTESIAN_POINT('Ctrl Pts',(-0.829915811207326,26.0804990336547,
8.71740951960627));
#43163=CARTESIAN_POINT('Ctrl Pts',(-0.739493573310718,26.0820653851727,
8.71345864444578));
#43164=CARTESIAN_POINT('Ctrl Pts',(-0.645913650094968,26.0833957874964,
8.71011175662346));
#43165=CARTESIAN_POINT('Ctrl Pts',(-0.599123688487095,26.0840609886583,
8.70843831271229));
#43166=CARTESIAN_POINT('Ctrl Pts',(-0.551544305404433,26.0846671724655,
8.70691585554372));
#43167=CARTESIAN_POINT('Ctrl Pts',(-0.503176822052515,26.0852068326966,
8.70556207661074));
#43168=CARTESIAN_POINT('Ctrl Pts',(-0.478993080376557,26.0854766628122,
8.70488518714424));
#43169=CARTESIAN_POINT('Ctrl Pts',(-0.454612313630426,26.0857298598239,
8.70425046650503));
#43170=CARTESIAN_POINT('Ctrl Pts',(-0.430034769117113,26.0859654658729,
8.70366013802557));
#43171=CARTESIAN_POINT('Ctrl Pts',(-0.417745996860458,26.0860832688974,
8.70336497378585));
#43172=CARTESIAN_POINT('Ctrl Pts',(-0.405408030162496,26.0861966740309,
8.70308090753664));
#43173=CARTESIAN_POINT('Ctrl Pts',(-0.393020899242947,26.0863055592071,
8.70280822111152));
#43174=CARTESIAN_POINT('Ctrl Pts',(-0.386827333783172,26.0863600017952,
8.70267187789895));
#43175=CARTESIAN_POINT('Ctrl Pts',(-0.38062147726803,26.0864133143842,8.70253837963916));
#43176=CARTESIAN_POINT('Ctrl Pts',(-0.374403333723082,26.0864654815839,
8.70240776175677));
#43177=CARTESIAN_POINT('Ctrl Pts',(-0.368185190178134,26.0865176487837,
8.70227714387437));
#43178=CARTESIAN_POINT('Ctrl Pts',(-0.359951179343043,26.086584673328,8.70210934521882));
#43179=CARTESIAN_POINT('Ctrl Pts',(-0.355712046080956,26.0866185315618,
8.70202458472192));
#43180=CARTESIAN_POINT('Ctrl Pts',(-0.236619695465579,26.087569729932,8.69964336049719));
#43181=CARTESIAN_POINT('Ctrl Pts',(-0.118036481380672,26.0880468078157,
8.69845862330752));
#43182=CARTESIAN_POINT('Ctrl Pts',(8.84627652694544E-13,26.0880528188531,
8.69844059746301));
#43183=CARTESIAN_POINT('Ctrl Pts',(0.150862669520566,26.0880605015723,8.69841755859408));
#43184=CARTESIAN_POINT('Ctrl Pts',(0.300832226640068,26.0872987295697,8.70030104109582));
#43185=CARTESIAN_POINT('Ctrl Pts',(0.449830176676706,26.0858123671823,8.70402388189702));
#43186=CARTESIAN_POINT('Ctrl Pts',(0.582617904676077,26.0844877134917,8.70734169648153));
#43187=CARTESIAN_POINT('Ctrl Pts',(0.714638268422484,26.0825864011306,8.71212360418822));
#43188=CARTESIAN_POINT('Ctrl Pts',(0.845857312319287,26.0801350899488,8.71832934841613));
#43189=CARTESIAN_POINT('Ctrl Pts',(0.911466834267689,26.0789094343579,8.72143222053008));
#43190=CARTESIAN_POINT('Ctrl Pts',(0.976876025877581,26.0775462469279,8.72489104102562));
#43191=CARTESIAN_POINT('Ctrl Pts',(1.04208087423999,26.0760486783595,8.72870073181513));
#43192=CARTESIAN_POINT('Ctrl Pts',(1.0746832984212,26.0752998940752,8.73060557720988));
#43193=CARTESIAN_POINT('Ctrl Pts',(1.10723463677122,26.0745175128011,8.73259813958272));
#43194=CARTESIAN_POINT('Ctrl Pts',(1.13973439403713,26.0737019184225,8.73467778118198));
#43195=CARTESIAN_POINT('Ctrl Pts',(1.15598427267008,26.0732941212332,8.73571760198161));
#43196=CARTESIAN_POINT('Ctrl Pts',(1.17222125603092,26.0728780206698,8.73677919255257));
#43197=CARTESIAN_POINT('Ctrl Pts',(1.18844528299769,26.0724536641226,8.73786247301944));
#43198=CARTESIAN_POINT('Ctrl Pts',(1.19655729648108,26.072241485849,8.73840411325288));
#43199=CARTESIAN_POINT('Ctrl Pts',(1.20466607086589,26.0720272435736,8.73895117595814));
#43200=CARTESIAN_POINT('Ctrl Pts',(1.21277159856042,26.0718109431763,8.73950365116429));
#43201=CARTESIAN_POINT('Ctrl Pts',(1.21682436240769,26.0717027929776,8.73977988876737));
#43202=CARTESIAN_POINT('Ctrl Pts',(1.22087631458238,26.0715941282481,8.74005747949553));
#43203=CARTESIAN_POINT('Ctrl Pts',(1.22492745414149,26.0714849497653,8.74033642196936));
#43204=CARTESIAN_POINT('Ctrl Pts',(1.22695302392105,26.0714303605238,8.74047589320627));
#43205=CARTESIAN_POINT('Ctrl Pts',(1.2289783905467,26.071375642844,8.7406157023796));
#43206=CARTESIAN_POINT('Ctrl Pts',(1.23100355390154,26.0713207968345,8.74075584928271));
#43207=CARTESIAN_POINT('Ctrl Pts',(1.23302871725637,26.0712659508249,8.74089599618582));
#43208=CARTESIAN_POINT('Ctrl Pts',(1.2364307874484,26.071173499238,8.74113225907129));
#43209=CARTESIAN_POINT('Ctrl Pts',(1.23707843403604,26.071155873915,8.74117730300421));
#43210=CARTESIAN_POINT('Ctrl Pts',(1.27880640238213,26.070020271669,8.74407949046734));
#43211=CARTESIAN_POINT('Ctrl Pts',(1.32947418621204,26.0685956982891,8.74772049868581));
#43212=CARTESIAN_POINT('Ctrl Pts',(1.38903588177794,26.0667850967465,8.75236099222838));
#43213=CARTESIAN_POINT('Ctrl Pts',(1.4502568344543,26.0649240558492,8.75713075965802));
#43214=CARTESIAN_POINT('Ctrl Pts',(1.52087413046551,26.0626550531865,8.76295665858922));
#43215=CARTESIAN_POINT('Ctrl Pts',(1.600837921869,26.0598523531197,8.77017538872663));
#43216=CARTESIAN_POINT('Ctrl Pts',(1.68763018423549,26.0568103177776,8.7780105589836));
#43217=CARTESIAN_POINT('Ctrl Pts',(1.78543337805792,26.0531393882259,8.78748663714181));
#43218=CARTESIAN_POINT('Ctrl Pts',(1.89418376361909,26.0486569411145,8.79909572979417));
#43219=CARTESIAN_POINT('Ctrl Pts',(1.97507224561918,26.0453228992109,8.80773056706121));
#43220=CARTESIAN_POINT('Ctrl Pts',(2.06201712669602,26.041539334321,8.81754695154596));
#43221=CARTESIAN_POINT('Ctrl Pts',(2.1549921780888,26.0372258146777,8.82876497934841));
#43222=CARTESIAN_POINT('Ctrl Pts',(2.28380967502505,26.0312494070811,8.84430762482615));
#43223=CARTESIAN_POINT('Ctrl Pts',(2.42418374813402,26.0242460016502,8.86256856411004));
#43224=CARTESIAN_POINT('Ctrl Pts',(2.57592901329186,26.0159217123473,8.88437768472368));
#43225=CARTESIAN_POINT('Ctrl Pts',(2.68639479746009,26.0098618913404,8.90025403913974));
#43226=CARTESIAN_POINT('Ctrl Pts',(2.80288661117011,26.0031018901479,8.9180112218424));
#43227=CARTESIAN_POINT('Ctrl Pts',(2.92533293723364,25.9955370736535,8.93795304949481));
#43228=CARTESIAN_POINT('Ctrl Pts',(3.04038694421305,25.9884289596111,8.95669095084035));
#43229=CARTESIAN_POINT('Ctrl Pts',(3.16069314161519,25.9806061163848,8.97736950665797));
#43230=CARTESIAN_POINT('Ctrl Pts',(3.28616263495456,25.9719648496818,9.00029786548505));
#43231=CARTESIAN_POINT('Ctrl Pts',(3.31917347192997,25.969691345272,9.00633028257074));
#43232=CARTESIAN_POINT('Ctrl Pts',(3.35254171651977,25.9673612973124,9.01251818453037));
#43233=CARTESIAN_POINT('Ctrl Pts',(3.38626574978679,25.9649730755069,9.01886661871804));
#43234=CARTESIAN_POINT('Ctrl Pts',(3.46721789189222,25.9592403190049,9.03410558324042));
#43235=CARTESIAN_POINT('Ctrl Pts',(3.55021941013772,25.9531711026084,9.05027288491658));
#43236=CARTESIAN_POINT('Ctrl Pts',(3.63524343812244,25.9467396041628,9.06744908937538));
#43237=CARTESIAN_POINT('Ctrl Pts',(3.6777554521148,25.94352385494,9.07603719160478));
#43238=CARTESIAN_POINT('Ctrl Pts',(3.72077309357543,25.9402175474073,9.08487752393684));
#43239=CARTESIAN_POINT('Ctrl Pts',(3.76429262432316,25.936817427614,9.09398048718069));
#43240=CARTESIAN_POINT('Ctrl Pts',(3.78605238969703,25.9351173677173,9.09853196880261));
#43241=CARTESIAN_POINT('Ctrl Pts',(3.80793762739503,25.9333938556752,9.10314910848554));
#43242=CARTESIAN_POINT('Ctrl Pts',(3.82994785785757,25.9316464880811,9.10783321552209));
#43243=CARTESIAN_POINT('Ctrl Pts',(3.84095297308885,25.930772804284,9.11017526904036));
#43244=CARTESIAN_POINT('Ctrl Pts',(3.85198933651134,25.9298931566631,9.11253406442057));
#43245=CARTESIAN_POINT('Ctrl Pts',(3.86305688682359,25.9290074948405,9.11490976643313));
#43246=CARTESIAN_POINT('Ctrl Pts',(3.86859066197971,25.9285646639292,9.11609761743942));
#43247=CARTESIAN_POINT('Ctrl Pts',(3.87413223385828,25.9281203294717,9.11728969510533));
#43248=CARTESIAN_POINT('Ctrl Pts',(3.87968159470531,25.9276744851742,9.11848602009804));
#43249=CARTESIAN_POINT('Ctrl Pts',(3.88523095555234,25.9272286408767,9.11968234509074));
#43250=CARTESIAN_POINT('Ctrl Pts',(3.8929759297363,25.9266048156772,9.12135659426671));
#43251=CARTESIAN_POINT('Ctrl Pts',(3.8963530363699,25.9263324164788,9.12208775774814));
#43252=CARTESIAN_POINT('Ctrl Pts',(4.05455254536718,25.9135719608254,9.15633888343296));
#43253=CARTESIAN_POINT('Ctrl Pts',(4.20702422262898,25.9005572533943,9.19143330092842));
#43254=CARTESIAN_POINT('Ctrl Pts',(4.35383997724603,25.8874577523657,9.22692824483611));
#43255=CARTESIAN_POINT('Ctrl Pts',(4.49776644086422,25.8746160456759,9.26172465865618));
#43256=CARTESIAN_POINT('Ctrl Pts',(4.63625740514875,25.861692914023,9.29690585548952));
#43257=CARTESIAN_POINT('Ctrl Pts',(4.76938061674201,25.8488288553367,9.33210103938896));
#43258=CARTESIAN_POINT('Ctrl Pts',(4.90003547357203,25.8362033204973,9.36664363837266));
#43259=CARTESIAN_POINT('Ctrl Pts',(5.02551978873465,25.823634734847,9.40119967260459));
#43260=CARTESIAN_POINT('Ctrl Pts',(5.14589760986401,25.8112364690961,9.43546490646807));
#43261=CARTESIAN_POINT('Ctrl Pts',(5.26549547828554,25.7989185342637,9.46950812882075));
#43262=CARTESIAN_POINT('Ctrl Pts',(5.38005281035675,25.7867687802875,9.5032642479009));
#43263=CARTESIAN_POINT('Ctrl Pts',(5.48963241682708,25.7748781427592,9.53648188896845));
#43264=CARTESIAN_POINT('Ctrl Pts',(5.59870644662265,25.7630423660685,9.56954627100308));
#43265=CARTESIAN_POINT('Ctrl Pts',(5.70284857716153,25.7514633579738,9.60207711615654));
#43266=CARTESIAN_POINT('Ctrl Pts',(5.80212075381237,25.740209928981,9.63387378843652));
#43267=CARTESIAN_POINT('Ctrl Pts',(5.86628467072857,25.7329363493409,9.65442535794184));
#43268=CARTESIAN_POINT('Ctrl Pts',(5.92841411668111,25.7257983564541,9.67467118186661));
#43269=CARTESIAN_POINT('Ctrl Pts',(5.98852581792878,25.7188097818106,9.69456766392382));
#43270=CARTESIAN_POINT('Ctrl Pts',(-6.39567215327757,25.5334667771464,8.78352120081293));
#43271=CARTESIAN_POINT('Ctrl Pts',(-6.35564925405008,25.5378748203104,8.77012420775373));
#43272=CARTESIAN_POINT('Ctrl Pts',(-5.98524856644197,25.5783538673712,8.64740144178755));
#43273=CARTESIAN_POINT('Ctrl Pts',(-5.25616414720834,25.6522250604739,8.42856302669376));
#43274=CARTESIAN_POINT('Ctrl Pts',(-4.17575802099697,25.7436220847966,8.16491184754273));
#43275=CARTESIAN_POINT('Ctrl Pts',(-3.01936659774181,25.8195373983552,7.95089063936762));
#43276=CARTESIAN_POINT('Ctrl Pts',(-1.83578627573155,25.872533317112,7.80508001376507));
#43277=CARTESIAN_POINT('Ctrl Pts',(-0.697926096812265,25.8989853856378,
7.73463115189508));
#43278=CARTESIAN_POINT('Ctrl Pts',(0.331404301561069,25.9017876014486,7.72744126775874));
#43279=CARTESIAN_POINT('Ctrl Pts',(1.24580220706962,25.8874720952612,7.76509235812669));
#43280=CARTESIAN_POINT('Ctrl Pts',(2.07029186482381,25.8615915973225,7.83520238948189));
#43281=CARTESIAN_POINT('Ctrl Pts',(2.81705936567024,25.8276643504536,7.92875394935922));
#43282=CARTESIAN_POINT('Ctrl Pts',(3.49017608565394,25.7886689674746,8.03787750825027));
#43283=CARTESIAN_POINT('Ctrl Pts',(4.0949642222784,25.747012346068,8.15592090125258));
#43284=CARTESIAN_POINT('Ctrl Pts',(4.65004649453019,25.7034080434421,8.28092688614671));
#43285=CARTESIAN_POINT('Ctrl Pts',(5.18049690519974,25.6570345557263,8.4154495605664));
#43286=CARTESIAN_POINT('Ctrl Pts',(5.70541816431205,25.6067236205178,8.56333260888681));
#43287=CARTESIAN_POINT('Ctrl Pts',(6.10978031431405,25.5646825181694,8.6889091565671));
#43288=CARTESIAN_POINT('Ctrl Pts',(6.34031508653319,25.5395632352113,8.76499188397675));
#43289=CARTESIAN_POINT('Ctrl Pts',(6.39541676950722,25.5334956939384,8.78343681303983));
#43290=CARTESIAN_POINT('Ctrl Pts',(-6.33011139739059,25.7770025828591,9.06768825330065));
#43291=CARTESIAN_POINT('Ctrl Pts',(-6.29056321231621,25.7814432939444,9.05437271194277));
#43292=CARTESIAN_POINT('Ctrl Pts',(-5.92452857218488,25.8222252643026,8.93238597022711));
#43293=CARTESIAN_POINT('Ctrl Pts',(-5.203572845008,25.8966944951544,8.71469357563352));
#43294=CARTESIAN_POINT('Ctrl Pts',(-4.13461175586402,25.9888994695799,8.45222824130109));
#43295=CARTESIAN_POINT('Ctrl Pts',(-2.99009397812991,26.065525690553,8.23905800812465));
#43296=CARTESIAN_POINT('Ctrl Pts',(-1.81832922019448,26.1190305753704,8.09376643352996));
#43297=CARTESIAN_POINT('Ctrl Pts',(-0.69152146876971,26.1457315728714,8.0235405665061));
#43298=CARTESIAN_POINT('Ctrl Pts',(0.328402059247375,26.1485587633991,8.01637067248625));
#43299=CARTESIAN_POINT('Ctrl Pts',(1.23408499126555,26.1341108596132,8.05390746812353));
#43300=CARTESIAN_POINT('Ctrl Pts',(2.05049313694551,26.1079833265253,8.12378170806464));
#43301=CARTESIAN_POINT('Ctrl Pts',(2.78979399169512,26.0737316581453,8.21699609755371));
#43302=CARTESIAN_POINT('Ctrl Pts',(3.45606870546097,26.0343678285272,8.32569987339932));
#43303=CARTESIAN_POINT('Ctrl Pts',(4.05461471067682,25.992326080533,8.44325998325948));
#43304=CARTESIAN_POINT('Ctrl Pts',(4.60387478654295,25.9483298974354,8.56772132367673));
#43305=CARTESIAN_POINT('Ctrl Pts',(5.12865373396191,25.9015538253764,8.70161770703905));
#43306=CARTESIAN_POINT('Ctrl Pts',(5.64781964556615,25.8508244104092,8.84875802217962));
#43307=CARTESIAN_POINT('Ctrl Pts',(6.04758703599702,25.8084521556453,8.9736427631715));
#43308=CARTESIAN_POINT('Ctrl Pts',(6.27541106185641,25.783144228056,9.04927164235629));
#43309=CARTESIAN_POINT('Ctrl Pts',(6.32985871986087,25.7770316774931,9.06760427361747));
#43310=CARTESIAN_POINT('Ctrl Pts',(-6.21909462086777,25.836782154238,9.42601905314513));
#43311=CARTESIAN_POINT('Ctrl Pts',(-6.18025121921535,25.8412519032068,9.41291697690927));
#43312=CARTESIAN_POINT('Ctrl Pts',(-5.82072605323139,25.8823021492172,9.29288098658681));
#43313=CARTESIAN_POINT('Ctrl Pts',(-5.11236921245908,25.9572845750022,9.07859409021145));
#43314=CARTESIAN_POINT('Ctrl Pts',(-4.06204085296457,26.0501633515562,8.82020853397432));
#43315=CARTESIAN_POINT('Ctrl Pts',(-2.93762065843339,26.1273686052668,8.61036402280483));
#43316=CARTESIAN_POINT('Ctrl Pts',(-1.78654232977251,26.1812753445501,8.46734625508623));
#43317=CARTESIAN_POINT('Ctrl Pts',(-0.679604906611716,26.2081619982703,
8.39820999068061));
#43318=CARTESIAN_POINT('Ctrl Pts',(0.322775234770271,26.2110063243669,8.39114887629604));
#43319=CARTESIAN_POINT('Ctrl Pts',(1.21259995864587,26.1964622439816,8.42810733714285));
#43320=CARTESIAN_POINT('Ctrl Pts',(2.01460907267051,26.1701446088356,8.49689116067258));
#43321=CARTESIAN_POINT('Ctrl Pts',(2.74086259740854,26.1356362294652,8.58864802757013));
#43322=CARTESIAN_POINT('Ctrl Pts',(3.39541033252112,26.0959750883794,8.6956538995844));
#43323=CARTESIAN_POINT('Ctrl Pts',(3.98346188127814,26.0536180912027,8.81138170964562));
#43324=CARTESIAN_POINT('Ctrl Pts',(4.52312475530119,26.0092972283702,8.93390626645097));
#43325=CARTESIAN_POINT('Ctrl Pts',(5.0387516314274,25.9621835641126,9.06571874387191));
#43326=CARTESIAN_POINT('Ctrl Pts',(5.54885320623593,25.9110981985056,9.21056117041002));
#43327=CARTESIAN_POINT('Ctrl Pts',(5.94159337987235,25.8684387281626,9.33347708049541));
#43328=CARTESIAN_POINT('Ctrl Pts',(6.16536922502574,25.8429639688667,9.40789773397969));
#43329=CARTESIAN_POINT('Ctrl Pts',(6.21884615353447,25.8368113937589,9.42593631502812));
#43330=CARTESIAN_POINT('Ctrl Pts',(-6.09442352525463,25.6959141203215,9.75594787349936));
#43331=CARTESIAN_POINT('Ctrl Pts',(-6.05631315053983,25.7004009763365,9.74313007698199));
#43332=CARTESIAN_POINT('Ctrl Pts',(-5.70357677499405,25.7416081622015,9.62570029038551));
#43333=CARTESIAN_POINT('Ctrl Pts',(-5.00868072692758,25.8168722610937,9.41610186799907));
#43334=CARTESIAN_POINT('Ctrl Pts',(-3.97883577951549,25.9100981342311,9.16351996697486));
#43335=CARTESIAN_POINT('Ctrl Pts',(-2.87697998757772,25.9875850899881,8.95852199803055));
#43336=CARTESIAN_POINT('Ctrl Pts',(-1.74953270103721,26.0416717614473,8.81888051999469));
#43337=CARTESIAN_POINT('Ctrl Pts',(-0.665590719017744,26.0686277716833,
8.75138786955641));
#43338=CARTESIAN_POINT('Ctrl Pts',(0.316136038747394,26.071476502194,8.74449311396111));
#43339=CARTESIAN_POINT('Ctrl Pts',(1.18750276603807,26.0568999322397,8.78057512315524));
#43340=CARTESIAN_POINT('Ctrl Pts',(1.97292052610175,26.0305034336769,8.84772672103612));
#43341=CARTESIAN_POINT('Ctrl Pts',(2.68428382255083,25.9958793975116,8.93732381873537));
#43342=CARTESIAN_POINT('Ctrl Pts',(3.32557899277926,25.9560770317247,9.04184069738195));
#43343=CARTESIAN_POINT('Ctrl Pts',(3.90188993653773,25.913564745964,9.15491273886181));
#43344=CARTESIAN_POINT('Ctrl Pts',(4.43092963053144,25.8690791874711,9.27466385145588));
#43345=CARTESIAN_POINT('Ctrl Pts',(4.93654521767831,25.8217894019311,9.40353243689169));
#43346=CARTESIAN_POINT('Ctrl Pts',(5.43686957263409,25.7705123468464,9.54518075650168));
#43347=CARTESIAN_POINT('Ctrl Pts',(5.82216258062757,25.727691692376,9.665415326738));
#43348=CARTESIAN_POINT('Ctrl Pts',(6.04171208841764,25.7021196038088,9.73821977413358));
#43349=CARTESIAN_POINT('Ctrl Pts',(6.09417956627165,25.6959434303745,9.75586685440467));
#43350=CARTESIAN_POINT('',(6.27159454904157,25.5608537658352,8.76071457497584));
#43351=CARTESIAN_POINT('Origin',(5.999999949017,24.7867247244415,9.33250966431025));
#43352=CARTESIAN_POINT('Ctrl Pts',(-6.27159387327992,25.5608571664729,8.76070928018854));
#43353=CARTESIAN_POINT('Ctrl Pts',(-6.13239664953756,25.575965649089,8.71504798308059));
#43354=CARTESIAN_POINT('Ctrl Pts',(-5.98564492700752,25.5914802261018,8.66855402651474));
#43355=CARTESIAN_POINT('Ctrl Pts',(-5.83132864915275,25.607227821856,8.62173960560949));
#43356=CARTESIAN_POINT('Ctrl Pts',(-5.67907411117793,25.6227650221378,8.57555064794039));
#43357=CARTESIAN_POINT('Ctrl Pts',(-5.51945550480999,25.638529241025,8.52904987089545));
#43358=CARTESIAN_POINT('Ctrl Pts',(-5.35247247516796,25.6543232268546,8.48276842591158));
#43359=CARTESIAN_POINT('Ctrl Pts',(-5.3256661092757,25.6568586902724,8.47533870475417));
#43360=CARTESIAN_POINT('Ctrl Pts',(-5.2986699799632,25.6593948516824,8.46791471659402));
#43361=CARTESIAN_POINT('Ctrl Pts',(-5.27148411637426,25.6619308142419,8.46049875106702));
#43362=CARTESIAN_POINT('Ctrl Pts',(-5.14595239295794,25.6736407144837,8.42625525792378));
#43363=CARTESIAN_POINT('Ctrl Pts',(-5.01637482827605,25.6853470111082,8.39218170988391));
#43364=CARTESIAN_POINT('Ctrl Pts',(-4.88275739379448,25.6969639517451,8.35851824340345));
#43365=CARTESIAN_POINT('Ctrl Pts',(-4.71106409288832,25.7118912768514,8.31526197447118));
#43366=CARTESIAN_POINT('Ctrl Pts',(-4.53269553687205,25.7266725079885,8.27268032221235));
#43367=CARTESIAN_POINT('Ctrl Pts',(-4.34764553912031,25.7411115944755,8.23131618958215));
#43368=CARTESIAN_POINT('Ctrl Pts',(-4.2958392354979,25.7451539382077,8.21973595267237));
#43369=CARTESIAN_POINT('Ctrl Pts',(-4.24350936371134,25.7491693140107,8.20825139413575));
#43370=CARTESIAN_POINT('Ctrl Pts',(-4.19065603668935,25.7531530590042,8.19687502119264));
#43371=CARTESIAN_POINT('Ctrl Pts',(-4.14338231791793,25.7567162488938,8.18669962665356));
#43372=CARTESIAN_POINT('Ctrl Pts',(-4.0956898294982,25.7602541303974,8.17661078502605));
#43373=CARTESIAN_POINT('Ctrl Pts',(-4.04757899994192,25.7637634416522,8.16661761900435));
#43374=CARTESIAN_POINT('Ctrl Pts',(-3.90056248231458,25.7744871544776,8.13608061762375));
#43375=CARTESIAN_POINT('Ctrl Pts',(-3.74963598155595,25.7849451003172,8.10643537283319));
#43376=CARTESIAN_POINT('Ctrl Pts',(-3.59479967329023,25.7950405852558,8.07795017762525));
#43377=CARTESIAN_POINT('Ctrl Pts',(-3.51738151915737,25.8000883277252,8.06370758002128));
#43378=CARTESIAN_POINT('Ctrl Pts',(-3.43898590453603,25.8050453456782,8.04975523934115));
#43379=CARTESIAN_POINT('Ctrl Pts',(-3.35961280206576,25.8098988457103,8.03612821259867));
#43380=CARTESIAN_POINT('Ctrl Pts',(-3.31992625083063,25.8123255957263,8.02931469922742));
#43381=CARTESIAN_POINT('Ctrl Pts',(-3.27999532524208,25.8147264537992,8.02258252424152));
#43382=CARTESIAN_POINT('Ctrl Pts',(-3.23982002132918,25.8170997774362,8.01593617638247));
#43383=CARTESIAN_POINT('Ctrl Pts',(-3.21973236937273,25.8182864392547,8.01261300245294));
#43384=CARTESIAN_POINT('Ctrl Pts',(-3.1995836226854,25.8194662166494,8.00931128595365));
#43385=CARTESIAN_POINT('Ctrl Pts',(-3.17937378027931,25.8206389002878,8.00603159320849));
#43386=CARTESIAN_POINT('Ctrl Pts',(-3.16169016817398,25.8216649984714,8.00316186205647));
#43387=CARTESIAN_POINT('Ctrl Pts',(-3.14395977965026,25.8226856654494,8.00030899287969));
#43388=CARTESIAN_POINT('Ctrl Pts',(-3.12618261395312,25.8237007595066,7.99747336763182));
#43389=CARTESIAN_POINT('Ctrl Pts',(-3.12364301885352,25.8238457729434,7.9970682783107));
#43390=CARTESIAN_POINT('Ctrl Pts',(-3.11986204430108,25.8240613377268,7.99646617419699));
#43391=CARTESIAN_POINT('Ctrl Pts',(-3.11856096474827,25.824135458209,7.99625915656741));
#43392=CARTESIAN_POINT('Ctrl Pts',(-3.09161192020686,25.8256707034384,7.99197123481171));
#43393=CARTESIAN_POINT('Ctrl Pts',(-3.06343761503096,25.8272573707004,7.98754567947991));
#43394=CARTESIAN_POINT('Ctrl Pts',(-3.03403807605523,25.8288897798103,7.98299838251482));
#43395=CARTESIAN_POINT('Ctrl Pts',(-2.96197169591088,25.8328912648526,7.97185170324256));
#43396=CARTESIAN_POINT('Ctrl Pts',(-2.88254322638795,25.8371688494462,7.95997012655567));
#43397=CARTESIAN_POINT('Ctrl Pts',(-2.79575230181482,25.8416266619309,7.9476214331184));
#43398=CARTESIAN_POINT('Ctrl Pts',(-2.70929163338439,25.8460675115826,7.93531972883216));
#43399=CARTESIAN_POINT('Ctrl Pts',(-2.61552418771846,25.8506872657355,7.92255446105429));
#43400=CARTESIAN_POINT('Ctrl Pts',(-2.51445069720308,25.855372905854,7.90963877170834));
#43401=CARTESIAN_POINT('Ctrl Pts',(-2.50259151428056,25.8559226826846,7.90812334445098));
#43402=CARTESIAN_POINT('Ctrl Pts',(-2.4906317538322,25.8564733453643,7.90660590131109));
#43403=CARTESIAN_POINT('Ctrl Pts',(-2.47857142058778,25.8570246943066,7.90508699199917));
#43404=CARTESIAN_POINT('Ctrl Pts',(-2.37688555907985,25.8616733545927,7.89228041370609));
#43405=CARTESIAN_POINT('Ctrl Pts',(-2.26804970880952,25.8663725677609,7.8793659892952));
#43406=CARTESIAN_POINT('Ctrl Pts',(-2.15206266310375,25.8709939097392,7.86670049242327));
#43407=CARTESIAN_POINT('Ctrl Pts',(-2.11969726318713,25.8722834639335,7.86316627126169));
#43408=CARTESIAN_POINT('Ctrl Pts',(-2.08677508025734,25.8735668397906,7.85965171818127));
#43409=CARTESIAN_POINT('Ctrl Pts',(-2.05329620826432,25.8748409764783,7.85616525032574));
#43410=CARTESIAN_POINT('Ctrl Pts',(-1.97656808888935,25.8777610901518,7.84817483410527));
#43411=CARTESIAN_POINT('Ctrl Pts',(-1.89691549423532,25.8806329596912,7.84033139016118));
#43412=CARTESIAN_POINT('Ctrl Pts',(-1.81433837908348,25.8834176187708,7.83274216046773));
#43413=CARTESIAN_POINT('Ctrl Pts',(-1.81240130548538,25.8834829406166,7.8325641341896));
#43414=CARTESIAN_POINT('Ctrl Pts',(-1.81046262264534,25.8835482142048,7.8323862480318));
#43415=CARTESIAN_POINT('Ctrl Pts',(-1.80852233054424,25.8836134390365,7.83220850346248));
#43416=CARTESIAN_POINT('Ctrl Pts',(-1.76910546295402,25.8849384758959,7.82859763778417));
#43417=CARTESIAN_POINT('Ctrl Pts',(-1.72902444752696,25.8862434067418,7.82504517372945));
#43418=CARTESIAN_POINT('Ctrl Pts',(-1.6882793075523,25.8875239410946,7.82156332312573));
#43419=CARTESIAN_POINT('Ctrl Pts',(-1.66690389946438,25.8881957253707,7.81973670091749));
#43420=CARTESIAN_POINT('Ctrl Pts',(-1.64534571114051,25.8888607903948,7.81792951642983));
#43421=CARTESIAN_POINT('Ctrl Pts',(-1.62360474343983,25.889518493133,7.81614356880621));
#43422=CARTESIAN_POINT('Ctrl Pts',(-1.6127342595895,25.8898473445022,7.81525059499439));
#43423=CARTESIAN_POINT('Ctrl Pts',(-1.60181808086,25.8901743549559,7.8143629306771));
#43424=CARTESIAN_POINT('Ctrl Pts',(-1.59085620735388,25.8904994430688,7.81348080371653));
#43425=CARTESIAN_POINT('Ctrl Pts',(-1.58537527060083,25.8906619871253,7.81303974023625));
#43426=CARTESIAN_POINT('Ctrl Pts',(-1.57988291015145,25.8908240505749,7.81260006111269));
#43427=CARTESIAN_POINT('Ctrl Pts',(-1.57437912601871,25.8909856231766,7.81216179501871));
#43428=CARTESIAN_POINT('Ctrl Pts',(-1.56887534188597,25.8911471957783,7.81172352892473));
#43429=CARTESIAN_POINT('Ctrl Pts',(-1.56205961599394,25.8913460650961,7.81118421557168));
#43430=CARTESIAN_POINT('Ctrl Pts',(-1.55783350257863,25.89146885813,7.81085126459434));
#43431=CARTESIAN_POINT('Ctrl Pts',(-1.33210010952135,25.8980277185939,7.79306703912503));
#43432=CARTESIAN_POINT('Ctrl Pts',(-1.11005333250434,25.9030589041166,7.7794380791357));
#43433=CARTESIAN_POINT('Ctrl Pts',(-0.89169622994583,25.906695435275,7.76958900504006));
#43434=CARTESIAN_POINT('Ctrl Pts',(-0.848420263737139,25.907416155589,7.7676370273267));
#43435=CARTESIAN_POINT('Ctrl Pts',(-0.805289118208011,25.9080820825321,
7.76583364434555));
#43436=CARTESIAN_POINT('Ctrl Pts',(-0.762302665091636,25.9086942316615,
7.76417611739813));
#43437=CARTESIAN_POINT('Ctrl Pts',(-0.724717141794447,25.9092294687816,
7.76272684644923));
#43438=CARTESIAN_POINT('Ctrl Pts',(-0.68724222102171,25.9097235717933,7.76138905797346));
#43439=CARTESIAN_POINT('Ctrl Pts',(-0.649878100577331,25.9101771201779,
7.76016085477969));
#43440=CARTESIAN_POINT('Ctrl Pts',(-0.558066277942419,25.911291587837,7.75714289068888));
#43441=CARTESIAN_POINT('Ctrl Pts',(-0.466923505753704,25.9121612114512,
7.75478652107046));
#43442=CARTESIAN_POINT('Ctrl Pts',(-0.376449018564199,25.9127967453162,
7.7530636364847));
#43443=CARTESIAN_POINT('Ctrl Pts',(-0.312801838539285,25.9132438319986,
7.75185161806052));
#43444=CARTESIAN_POINT('Ctrl Pts',(-0.249485544181297,25.913575012163,7.75095306737938));
#43445=CARTESIAN_POINT('Ctrl Pts',(-0.186500135809807,25.9137938238034,
7.75035834235737));
#43446=CARTESIAN_POINT('Ctrl Pts',(-0.155007431624062,25.9139032296236,
7.75006097984637));
#43447=CARTESIAN_POINT('Ctrl Pts',(-0.123597448811888,25.9139845409445,
7.74983957568175));
#43448=CARTESIAN_POINT('Ctrl Pts',(-0.0922701869944179,25.9140381879309,
7.74969293815496));
#43449=CARTESIAN_POINT('Ctrl Pts',(-0.0647192837063548,25.9140853680178,
7.74956397711321));
#43450=CARTESIAN_POINT('Ctrl Pts',(-0.0383381534770102,25.9141107435395,
7.74949397605362));
#43451=CARTESIAN_POINT('Ctrl Pts',(-0.0102093113128477,25.9141157540723,
7.74947894090337));
#43452=CARTESIAN_POINT('Ctrl Pts',(-0.00635373562016292,25.9141164408581,
7.74947688005921));
#43453=CARTESIAN_POINT('Ctrl Pts',(-0.00246532424755673,25.9141167168094,
7.74947592639803));
#43454=CARTESIAN_POINT('Ctrl Pts',(0.00146343592704603,25.9141165580605,
7.74947614237112));
#43455=CARTESIAN_POINT('Ctrl Pts',(0.123996040186545,25.9141116069004,7.74948287827353));
#43456=CARTESIAN_POINT('Ctrl Pts',(0.246525247851146,25.9136952230428,7.75063924297031));
#43457=CARTESIAN_POINT('Ctrl Pts',(0.369056161634649,25.9128591689236,7.75293700917956));
#43458=CARTESIAN_POINT('Ctrl Pts',(0.64487089222353,25.9109772271792,7.75810923672925));
#43459=CARTESIAN_POINT('Ctrl Pts',(0.920694080572269,25.9069699675977,7.76906155340267));
#43460=CARTESIAN_POINT('Ctrl Pts',(1.19651513952632,25.9008591996694,7.78581189746439));
#43461=CARTESIAN_POINT('Ctrl Pts',(1.22211216209444,25.9002921020549,7.78736637969499));
#43462=CARTESIAN_POINT('Ctrl Pts',(1.24770916810565,25.8997068763829,7.7889708319627));
#43463=CARTESIAN_POINT('Ctrl Pts',(1.27330614986382,25.8991035329777,7.79062529025566));
#43464=CARTESIAN_POINT('Ctrl Pts',(1.37082342231014,25.8968049649756,7.7969283091674));
#43465=CARTESIAN_POINT('Ctrl Pts',(1.46834034405745,25.8942434560884,7.80395705460546));
#43466=CARTESIAN_POINT('Ctrl Pts',(1.56585686824688,25.89141831084,7.81170938455013));
#43467=CARTESIAN_POINT('Ctrl Pts',(1.74017752234041,25.8863680778491,7.82556745873741));
#43468=CARTESIAN_POINT('Ctrl Pts',(1.91449856142016,25.880476413635,7.84173859307239));
#43469=CARTESIAN_POINT('Ctrl Pts',(2.08881914766684,25.8737425938397,7.86022312559126));
#43470=CARTESIAN_POINT('Ctrl Pts',(2.17523066091776,25.8704046085162,7.86938599304761));
#43471=CARTESIAN_POINT('Ctrl Pts',(2.26164204568451,25.8668596485272,7.87911743613203));
#43472=CARTESIAN_POINT('Ctrl Pts',(2.34805359304106,25.863107937854,7.88941699556841));
#43473=CARTESIAN_POINT('Ctrl Pts',(2.47841969424383,25.8574478622245,7.90495558327923));
#43474=CARTESIAN_POINT('Ctrl Pts',(2.60878583457507,25.8513174294346,7.92178731779572));
#43475=CARTESIAN_POINT('Ctrl Pts',(2.73915198671474,25.8447165662376,7.93991205144734));
#43476=CARTESIAN_POINT('Ctrl Pts',(2.77254322425417,25.8430258590459,7.94455441663774));
#43477=CARTESIAN_POINT('Ctrl Pts',(2.80593446849372,25.8413042753965,7.94928160882464));
#43478=CARTESIAN_POINT('Ctrl Pts',(2.83932570100359,25.8395518100846,7.95409365064916));
#43479=CARTESIAN_POINT('Ctrl Pts',(2.87111753474536,25.8378832856951,7.95867520161762));
#43480=CARTESIAN_POINT('Ctrl Pts',(2.90290935782796,25.836186767153,7.96333366859984));
#43481=CARTESIAN_POINT('Ctrl Pts',(2.93470118626495,25.8344622609784,7.96806902210271));
#43482=CARTESIAN_POINT('Ctrl Pts',(2.98358847779635,25.8318104337559,7.97535072367763));
#43483=CARTESIAN_POINT('Ctrl Pts',(3.03247576585934,25.829092441693,7.98281424533809));
#43484=CARTESIAN_POINT('Ctrl Pts',(3.08136305634897,25.8263083276583,7.9904595402296));
#43485=CARTESIAN_POINT('Ctrl Pts',(3.09765881984551,25.8253802896468,7.99300797186011));
#43486=CARTESIAN_POINT('Ctrl Pts',(3.11203761009798,25.8245558039489,7.99527206090195));
#43487=CARTESIAN_POINT('Ctrl Pts',(3.13025034766616,25.8235021731655,7.99816542552789));
#43488=CARTESIAN_POINT('Ctrl Pts',(3.25876974095643,25.8160671575057,8.0185826453391));
#43489=CARTESIAN_POINT('Ctrl Pts',(3.38586955214421,25.8083003352541,8.04008423985018));
#43490=CARTESIAN_POINT('Ctrl Pts',(3.51153601864061,25.8002315699843,8.06258511763896));
#43491=CARTESIAN_POINT('Ctrl Pts',(3.71379593233212,25.7872449092419,8.09880023314611));
#43492=CARTESIAN_POINT('Ctrl Pts',(3.9123420147794,25.7734766580682,8.13760300891054));
#43493=CARTESIAN_POINT('Ctrl Pts',(4.1071405034411,25.75904847144,8.17864699109328));
#43494=CARTESIAN_POINT('Ctrl Pts',(4.29249186418904,25.7453200075127,8.21770046630425));
#43495=CARTESIAN_POINT('Ctrl Pts',(4.47445059164769,25.7309940292942,8.25878319076582));
#43496=CARTESIAN_POINT('Ctrl Pts',(4.65300686532189,25.7161712833696,8.30161093596719));
#43497=CARTESIAN_POINT('Ctrl Pts',(4.83064737870333,25.7014245587568,8.34421903081588));
#43498=CARTESIAN_POINT('Ctrl Pts',(5.00492039797542,25.6861862006155,8.3885543902908));
#43499=CARTESIAN_POINT('Ctrl Pts',(5.17583188151053,25.6705523550977,8.43435430849758));
#43500=CARTESIAN_POINT('Ctrl Pts',(5.35320454352684,25.6543274839557,8.48188565773427));
#43501=CARTESIAN_POINT('Ctrl Pts',(5.52695678568221,25.6376768256315,8.53099447907734));
#43502=CARTESIAN_POINT('Ctrl Pts',(5.69711015110884,25.6207054195578,8.58141011157052));
#43503=CARTESIAN_POINT('Ctrl Pts',(5.87744252567627,25.6027187406029,8.63484173603484));
#43504=CARTESIAN_POINT('Ctrl Pts',(6.05373257749037,25.5843721248016,8.68974139055599));
#43505=CARTESIAN_POINT('Ctrl Pts',(6.2260191449712,25.5657894695239,8.74581872722904));
#43506=CARTESIAN_POINT('Ctrl Pts',(6.24124268425681,25.5641474739418,8.75077381775268));
#43507=CARTESIAN_POINT('Ctrl Pts',(6.25643497131818,25.5625036240469,8.75573811142633));
#43508=CARTESIAN_POINT('Ctrl Pts',(6.27159604048006,25.5608580129971,8.7607114336902));
#43509=CARTESIAN_POINT('Origin',(5.999999999061,24.7867247845918,9.33250979146072));
#43510=CARTESIAN_POINT('Origin',(5.99996968669486,24.786693647859,9.33251391748345));
#43511=CARTESIAN_POINT('Ctrl Pts',(6.2417693835149,15.8394371419482,3.89966763071918));
#43512=CARTESIAN_POINT('Ctrl Pts',(6.29480660013804,15.8210003804235,3.91290159518924));
#43513=CARTESIAN_POINT('Ctrl Pts',(6.43873775859606,15.7672282165569,3.96076091853584));
#43514=CARTESIAN_POINT('Ctrl Pts',(6.6574605393883,15.6678516583381,4.08940826000748));
#43515=CARTESIAN_POINT('Ctrl Pts',(6.86734070593742,15.5432497310862,4.30355889900136));
#43516=CARTESIAN_POINT('Ctrl Pts',(7.01531432749514,15.4204361246427,4.56089237217717));
#43517=CARTESIAN_POINT('Ctrl Pts',(7.09527320778199,15.3106118534239,4.83061809734207));
#43518=CARTESIAN_POINT('Ctrl Pts',(7.10994677008608,15.2460735777555,5.0132274309249));
#43519=CARTESIAN_POINT('Ctrl Pts',(7.10820127775525,15.2174916046755,5.10034196570805));
#43520=CARTESIAN_POINT('Ctrl Pts',(7.10813648779779,15.2165799927952,5.10312736513287));
#43521=CARTESIAN_POINT('Ctrl Pts',(6.04288609483464,15.2236247505278,3.8631163616068));
#43522=CARTESIAN_POINT('Ctrl Pts',(6.08960513438832,15.2073416533561,3.87444417175601));
#43523=CARTESIAN_POINT('Ctrl Pts',(6.21669065164213,15.1597345425427,3.91554209118234));
#43524=CARTESIAN_POINT('Ctrl Pts',(6.41097421036258,15.0712598304035,4.02691979479796));
#43525=CARTESIAN_POINT('Ctrl Pts',(6.59849709551467,14.9599216454064,4.21386278649374));
#43526=CARTESIAN_POINT('Ctrl Pts',(6.73122625671432,14.8501808036311,4.43977189790894));
#43527=CARTESIAN_POINT('Ctrl Pts',(6.80304009224872,14.7524265349867,4.67721487713722));
#43528=CARTESIAN_POINT('Ctrl Pts',(6.81617737917041,14.6954476818957,4.83787645047658));
#43529=CARTESIAN_POINT('Ctrl Pts',(6.81461541449534,14.6703824924246,4.91434573780175));
#43530=CARTESIAN_POINT('Ctrl Pts',(6.81455743808829,14.6695832352687,4.91679057943266));
#43531=CARTESIAN_POINT('Ctrl Pts',(6.02645463242452,14.8077937469123,3.36555058259603));
#43532=CARTESIAN_POINT('Ctrl Pts',(6.0909048021779,14.7857891518488,3.38107551335727));
#43533=CARTESIAN_POINT('Ctrl Pts',(6.26494841949978,14.7221064653423,3.43708239772331));
#43534=CARTESIAN_POINT('Ctrl Pts',(6.52611209862578,14.6065921781731,3.58601226673634));
#43535=CARTESIAN_POINT('Ctrl Pts',(6.77358742595278,14.4642384951137,3.83063358124898));
#43536=CARTESIAN_POINT('Ctrl Pts',(6.94658414411926,14.3254403906868,4.12182395730633));
#43537=CARTESIAN_POINT('Ctrl Pts',(7.03979999596078,14.2018202245916,4.4257862610867));
#43538=CARTESIAN_POINT('Ctrl Pts',(7.05702527180377,14.1289362505915,4.63206598706388));
#43539=CARTESIAN_POINT('Ctrl Pts',(7.05497400841223,14.0964786467982,4.73097960482542));
#43540=CARTESIAN_POINT('Ctrl Pts',(7.05489786501909,14.0954432215508,4.73414280665572));
#43541=CARTESIAN_POINT('Ctrl Pts',(6.20434274665245,14.8765684418783,2.74504865258545));
#43542=CARTESIAN_POINT('Ctrl Pts',(6.29855278522411,14.84484558641,2.76803006088607));
#43543=CARTESIAN_POINT('Ctrl Pts',(6.55152406662262,14.7537433506342,2.85051411109445));
#43544=CARTESIAN_POINT('Ctrl Pts',(6.92554893952471,14.5915746583482,3.06637382200757));
#43545=CARTESIAN_POINT('Ctrl Pts',(7.27464606008605,14.3949448866597,3.41448089961097));
#43546=CARTESIAN_POINT('Ctrl Pts',(7.51612671900243,14.2046487813112,3.82343069258363));
#43547=CARTESIAN_POINT('Ctrl Pts',(7.64578429976314,14.0347520877583,4.24764907618302));
#43548=CARTESIAN_POINT('Ctrl Pts',(7.66995071774345,13.9332743711703,4.53620693589844));
#43549=CARTESIAN_POINT('Ctrl Pts',(7.66706900976556,13.8875235981543,4.67544806374864));
#43550=CARTESIAN_POINT('Ctrl Pts',(7.66696203369115,13.8860634885015,4.67990184251473));
#43551=CARTESIAN_POINT('',(6.9999997358383,14.7967908123979,4.92966736370966));
#43552=CARTESIAN_POINT('',(7.00000022915846,14.5427406233569,3.16613333521326));
#43553=CARTESIAN_POINT('Ctrl Pts',(7.,14.7967908124046,4.92966736369987));
#43554=CARTESIAN_POINT('Ctrl Pts',(7.,14.7551697581394,4.82500542408383));
#43555=CARTESIAN_POINT('Ctrl Pts',(7.,14.7202719475865,4.7308289607362));
#43556=CARTESIAN_POINT('Ctrl Pts',(7.,14.6923688673053,4.64894777974916));
#43557=CARTESIAN_POINT('Ctrl Pts',(7.,14.6784173271647,4.60800718925564));
#43558=CARTESIAN_POINT('Ctrl Pts',(7.,14.666162916251,4.57015546746193));
#43559=CARTESIAN_POINT('Ctrl Pts',(7.,14.655417087011,4.53564364192123));
#43560=CARTESIAN_POINT('Ctrl Pts',(7.,14.650044172391,4.51838772915088));
#43561=CARTESIAN_POINT('Ctrl Pts',(7.,14.6450467875392,4.50196675534175));
#43562=CARTESIAN_POINT('Ctrl Pts',(7.,14.6403945300219,4.48641068966369));
#43563=CARTESIAN_POINT('Ctrl Pts',(7.,14.6380684012632,4.47863265682467));
#43564=CARTESIAN_POINT('Ctrl Pts',(7.,14.6358285543382,4.47107085101841));
#43565=CARTESIAN_POINT('Ctrl Pts',(7.,14.6336709343289,4.46372880000887));
#43566=CARTESIAN_POINT('Ctrl Pts',(7.,14.6325921243242,4.46005777450411));
#43567=CARTESIAN_POINT('Ctrl Pts',(7.,14.6315338710485,4.45644168769852));
#43568=CARTESIAN_POINT('Ctrl Pts',(7.,14.6304956715052,4.45288096933233));
#43569=CARTESIAN_POINT('Ctrl Pts',(7.,14.6294574719619,4.44932025096614));
#43570=CARTESIAN_POINT('Ctrl Pts',(7.,14.6289382246372,4.4475382963016));
#43571=CARTESIAN_POINT('Ctrl Pts',(7.,14.6274407295948,4.44236534461973));
#43572=CARTESIAN_POINT('Ctrl Pts',(7.,14.603480808917,4.35959811770983));
#43573=CARTESIAN_POINT('Ctrl Pts',(7.,14.5830120743208,4.27935669050358));
#43574=CARTESIAN_POINT('Ctrl Pts',(7.,14.5661204867627,4.20226777656473));
#43575=CARTESIAN_POINT('Ctrl Pts',(7.,14.5492288992046,4.12517886262588));
#43576=CARTESIAN_POINT('Ctrl Pts',(7.,14.5361235670877,4.05275636196388));
#43577=CARTESIAN_POINT('Ctrl Pts',(7.,14.5256463779026,3.98125693906969));
#43578=CARTESIAN_POINT('Ctrl Pts',(7.,14.5046919995326,3.8382580932813));
#43579=CARTESIAN_POINT('Ctrl Pts',(7.,14.4945143427946,3.69578853863727));
#43580=CARTESIAN_POINT('Ctrl Pts',(7.,14.4974004966839,3.55817078061321));
#43581=CARTESIAN_POINT('Ctrl Pts',(7.,14.5002866505733,3.42055302258915));
#43582=CARTESIAN_POINT('Ctrl Pts',(7.,14.5162046706628,3.28801013281503));
#43583=CARTESIAN_POINT('Ctrl Pts',(7.,14.5427403138302,3.1661340810964));
#43584=CARTESIAN_POINT('',(6.2499447585205,14.859388404893,2.76546247674145));
#43585=CARTESIAN_POINT('Ctrl Pts',(6.24994458389757,14.8593878111664,2.76546236623351));
#43586=CARTESIAN_POINT('Ctrl Pts',(6.29980716926801,14.8422034238441,2.77899714130872));
#43587=CARTESIAN_POINT('Ctrl Pts',(6.34865165736493,14.8247500216694,2.79442084961687));
#43588=CARTESIAN_POINT('Ctrl Pts',(6.39650063437509,14.8070371392973,2.81164832003518));
#43589=CARTESIAN_POINT('Ctrl Pts',(6.42315488865876,14.7971701849684,2.82124487582145));
#43590=CARTESIAN_POINT('Ctrl Pts',(6.44950007514397,14.787222497999,2.83140207154089));
#43591=CARTESIAN_POINT('Ctrl Pts',(6.4755382818578,14.7771943490334,2.8421117724326));
#43592=CARTESIAN_POINT('Ctrl Pts',(6.52301982831677,14.7589076818199,2.86164127252605));
#43593=CARTESIAN_POINT('Ctrl Pts',(6.56948212852928,14.740353824833,2.88300539426928));
#43594=CARTESIAN_POINT('Ctrl Pts',(6.61495863330414,14.7215228869671,2.90616780645185));
#43595=CARTESIAN_POINT('Ctrl Pts',(6.62617146692926,14.7168798702195,2.91187880547091));
#43596=CARTESIAN_POINT('Ctrl Pts',(6.63732425001315,14.7122199768811,2.9176993436247));
#43597=CARTESIAN_POINT('Ctrl Pts',(6.6484172330222,14.7075430018446,2.92362928654739));
#43598=CARTESIAN_POINT('Ctrl Pts',(6.69398623825065,14.6883303969287,2.94798897409292));
#43599=CARTESIAN_POINT('Ctrl Pts',(6.73852982859227,14.6688362321768,2.9741895171999));
#43600=CARTESIAN_POINT('Ctrl Pts',(6.78203884617526,14.6490475988644,3.00223984763589));
#43601=CARTESIAN_POINT('Ctrl Pts',(6.82408097367041,14.629926131847,3.0293444717801));
#43602=CARTESIAN_POINT('Ctrl Pts',(6.86515740984907,14.6105295250194,3.05817677588614));
#43603=CARTESIAN_POINT('Ctrl Pts',(6.90522597828194,14.5908446770955,3.08877620005188));
#43604=CARTESIAN_POINT('Ctrl Pts',(6.93747899216091,14.5749994473275,3.11340706885768));
#43605=CARTESIAN_POINT('Ctrl Pts',(6.96907832380679,14.5589674064224,3.13918361820505));
#43606=CARTESIAN_POINT('Ctrl Pts',(7.00000068579859,14.5427398601927,3.16613235169124));
#43607=CARTESIAN_POINT('',(6.26385811009516,15.8144409652449,3.90573611874549));
#43608=CARTESIAN_POINT('Origin',(6.52771826980506,15.8038104576537,2.94124750390268));
#43609=CARTESIAN_POINT('Ctrl Pts',(6.26385556519314,15.8144410677384,3.90574542181138));
#43610=CARTESIAN_POINT('Ctrl Pts',(6.30364984979714,15.7888354137076,3.91691345720727));
#43611=CARTESIAN_POINT('Ctrl Pts',(6.34303406289391,15.7620196111154,3.9307005085015));
#43612=CARTESIAN_POINT('Ctrl Pts',(6.3816518889474,15.7340505126519,3.94714461691159));
#43613=CARTESIAN_POINT('Ctrl Pts',(6.4267935123979,15.7013565306203,3.96636666604505));
#43614=CARTESIAN_POINT('Ctrl Pts',(6.47088863867637,15.667085953782,3.98922019532522));
#43615=CARTESIAN_POINT('Ctrl Pts',(6.51341066571092,15.6313661843138,4.01561497269632));
#43616=CARTESIAN_POINT('Ctrl Pts',(6.53319158177353,15.6147496255347,4.02789361772057));
#43617=CARTESIAN_POINT('Ctrl Pts',(6.55263143917655,15.5978197383494,4.040938560204));
#43618=CARTESIAN_POINT('Ctrl Pts',(6.57167361680582,15.5805908621124,4.05474088366913));
#43619=CARTESIAN_POINT('Ctrl Pts',(6.58329053398495,15.570080171989,4.06316116267796));
#43620=CARTESIAN_POINT('Ctrl Pts',(6.59475941100498,15.5594582226939,4.0718633354495));
#43621=CARTESIAN_POINT('Ctrl Pts',(6.60606691947575,15.5487284531784,4.08084546649594));
#43622=CARTESIAN_POINT('Ctrl Pts',(6.64408869308806,15.5126493409245,4.11104810168181));
#43623=CARTESIAN_POINT('Ctrl Pts',(6.68028910165754,15.4753495562228,4.14441625586059));
#43624=CARTESIAN_POINT('Ctrl Pts',(6.71423321238755,15.4369829533116,4.18075365161009));
#43625=CARTESIAN_POINT('Ctrl Pts',(6.73210524393638,15.4167824200556,4.1998857799608));
#43626=CARTESIAN_POINT('Ctrl Pts',(6.74935110305278,15.3962864909449,4.21984101266869));
#43627=CARTESIAN_POINT('Ctrl Pts',(6.76590188515017,15.3755200500137,4.24059109905349));
#43628=CARTESIAN_POINT('Ctrl Pts',(6.77350227475515,15.3659837609818,4.2501198778105));
#43629=CARTESIAN_POINT('Ctrl Pts',(6.78095602918618,15.3563904507545,4.25981628327801));
#43630=CARTESIAN_POINT('Ctrl Pts',(6.78825615479716,15.3467426609164,4.26967762130588));
#43631=CARTESIAN_POINT('Ctrl Pts',(6.790134185423,15.3442606700914,4.27221454954726));
#43632=CARTESIAN_POINT('Ctrl Pts',(6.79200204735593,15.3417750740821,4.27476239367609));
#43633=CARTESIAN_POINT('Ctrl Pts',(6.79385965046825,15.3392859192095,4.27732107911455));
#43634=CARTESIAN_POINT('Ctrl Pts',(6.79839881275779,15.333203523107,4.2835733772379));
#43635=CARTESIAN_POINT('Ctrl Pts',(6.80287673363183,15.3270998599874,4.28989042541093));
#43636=CARTESIAN_POINT('Ctrl Pts',(6.80729206658171,15.3209756341991,4.2962711170141));
#43637=CARTESIAN_POINT('Ctrl Pts',(6.80949973305664,15.317913521305,4.29946146281569));
#43638=CARTESIAN_POINT('Ctrl Pts',(6.81169175208366,15.3148462677536,4.30266771930985));
#43639=CARTESIAN_POINT('Ctrl Pts',(6.81386795551184,15.3117739591357,4.30588975184288));
#43640=CARTESIAN_POINT('Ctrl Pts',(6.81548498418286,15.3094910792096,4.30828388417325));
#43641=CARTESIAN_POINT('Ctrl Pts',(6.81751779611187,15.3065994703175,4.31132427339662));
#43642=CARTESIAN_POINT('Ctrl Pts',(6.81901903291707,15.3044498470018,4.3135904229623));
#43643=CARTESIAN_POINT('Ctrl Pts',(6.8195381664,15.3037064989604,4.31437406623084));
#43644=CARTESIAN_POINT('Ctrl Pts',(6.81999417601719,15.303051900134,4.31506478744318));
#43645=CARTESIAN_POINT('Ctrl Pts',(6.82034894851834,15.3025419553618,4.31560304213719));
#43646=CARTESIAN_POINT('Ctrl Pts',(6.83460303192456,15.2820533456421,4.33722909059689));
#43647=CARTESIAN_POINT('Ctrl Pts',(6.84880149062183,15.2603765087782,4.36053116336644));
#43648=CARTESIAN_POINT('Ctrl Pts',(6.86266115088873,15.2375350020463,4.38562159480448));
#43649=CARTESIAN_POINT('Ctrl Pts',(6.87577607619647,15.2159208607949,4.409363817046));
#43650=CARTESIAN_POINT('Ctrl Pts',(6.88858775800522,15.1932637307109,4.43470749378823));
#43651=CARTESIAN_POINT('Ctrl Pts',(6.90081536935772,15.1696006099861,4.46173298293594));
#43652=CARTESIAN_POINT('Ctrl Pts',(6.90556277146064,15.1604133414468,4.47222569981362));
#43653=CARTESIAN_POINT('Ctrl Pts',(6.91022166644203,15.1510746283178,4.48297175954424));
#43654=CARTESIAN_POINT('Ctrl Pts',(6.91477373620808,15.1415874471195,4.49397515925285));
#43655=CARTESIAN_POINT('Ctrl Pts',(6.92451241417757,15.1212906135304,4.51751578403212));
#43656=CARTESIAN_POINT('Ctrl Pts',(6.93376334490682,15.1003134238407,4.54223534254804));
#43657=CARTESIAN_POINT('Ctrl Pts',(6.94234872663041,15.0786949537686,4.56814999140341));
#43658=CARTESIAN_POINT('Ctrl Pts',(6.95179572114869,15.0549068946186,4.59666538577509));
#43659=CARTESIAN_POINT('Ctrl Pts',(6.96043775178613,15.0303418978765,4.62662830347885));
#43660=CARTESIAN_POINT('Ctrl Pts',(6.96800702070548,15.0050707208775,4.65803766375443));
#43661=CARTESIAN_POINT('Ctrl Pts',(6.97344665173649,14.9869096699149,4.68060990060317));
#43662=CARTESIAN_POINT('Ctrl Pts',(6.97833162733887,14.9683843006087,4.70392867568163));
#43663=CARTESIAN_POINT('Ctrl Pts',(6.98254997944005,14.9495281509576,4.72798518062679));
#43664=CARTESIAN_POINT('Ctrl Pts',(6.98802445617009,14.9250570897451,4.75920513888767));
#43665=CARTESIAN_POINT('Ctrl Pts',(6.99237688658608,14.9000279909683,4.79166907499824));
#43666=CARTESIAN_POINT('Ctrl Pts',(6.99536960101161,14.8745360686185,4.82531024797829));
#43667=CARTESIAN_POINT('Ctrl Pts',(6.99836231543714,14.8490441462688,4.85895142095833));
#43668=CARTESIAN_POINT('Ctrl Pts',(6.99999594670264,14.8230891465946,4.89377001753077));
#43669=CARTESIAN_POINT('Ctrl Pts',(6.99999920776373,14.7967908123851,4.92966736373478));
#43670=CARTESIAN_POINT('Ctrl Pts',(6.99990231846403,14.6847031578439,4.95610625002928));
#43671=CARTESIAN_POINT('Ctrl Pts',(6.99990231846403,15.0109940548522,4.91841598752362));
#43672=CARTESIAN_POINT('Ctrl Pts',(6.99990231846403,15.8988757041253,4.85614479764408));
#43673=CARTESIAN_POINT('Ctrl Pts',(6.99990231846403,17.351727469812,4.9299863360756));
#43674=CARTESIAN_POINT('Ctrl Pts',(6.99990231846403,19.0057080032784,5.27368461013775));
#43675=CARTESIAN_POINT('Ctrl Pts',(6.99990231846403,20.590268079334,5.86659846405635));
#43676=CARTESIAN_POINT('Ctrl Pts',(6.99990231846403,22.0651422307797,6.69608016041579));
#43677=CARTESIAN_POINT('Ctrl Pts',(6.99990231846403,23.3944809544711,7.73956615459866));
#43678=CARTESIAN_POINT('Ctrl Pts',(6.99990231846403,24.2870583744167,8.6952955923328));
#43679=CARTESIAN_POINT('Ctrl Pts',(6.99990231846403,24.7366539504827,9.28611088916545));
#43680=CARTESIAN_POINT('Ctrl Pts',(6.99990231846403,24.8428619070666,9.43307698115495));
#43681=CARTESIAN_POINT('Ctrl Pts',(7.00658755380489,14.6298084473363,4.48100446307126));
#43682=CARTESIAN_POINT('Ctrl Pts',(7.00658755380489,14.9703697746716,4.44166427685036));
#43683=CARTESIAN_POINT('Ctrl Pts',(7.00658755380489,15.8968450849154,4.37670040150181));
#43684=CARTESIAN_POINT('Ctrl Pts',(7.00658755380489,17.4127705149432,4.45373854384782));
#43685=CARTESIAN_POINT('Ctrl Pts',(7.00658755380489,19.1391934374833,4.81245484156605));
#43686=CARTESIAN_POINT('Ctrl Pts',(7.00658755380489,20.7926967961888,5.43122447964866));
#43687=CARTESIAN_POINT('Ctrl Pts',(7.00658755380489,22.3317396202352,6.29673482166948));
#43688=CARTESIAN_POINT('Ctrl Pts',(7.00658755380489,23.7192732848802,7.38594521460744));
#43689=CARTESIAN_POINT('Ctrl Pts',(7.00658755380489,24.6505400754064,8.38311665741879));
#43690=CARTESIAN_POINT('Ctrl Pts',(7.00658755380489,25.1196657073454,8.99958310836095));
#43691=CARTESIAN_POINT('Ctrl Pts',(7.00658755380489,25.2304959439334,9.15294401871312));
#43692=CARTESIAN_POINT('Ctrl Pts',(6.71725767899343,14.5860721993496,4.10247674370146));
#43693=CARTESIAN_POINT('Ctrl Pts',(6.71725767899343,14.9380032028224,4.06182201420451));
#43694=CARTESIAN_POINT('Ctrl Pts',(6.71725767899343,15.8952272302191,3.99471279628271));
#43695=CARTESIAN_POINT('Ctrl Pts',(6.71725767899343,17.4614053239266,4.07429776800594));
#43696=CARTESIAN_POINT('Ctrl Pts',(6.71725767899343,19.2455452516906,4.44497937168528));
#43697=CARTESIAN_POINT('Ctrl Pts',(6.71725767899343,20.953977773508,5.08434908175678));
#43698=CARTESIAN_POINT('Ctrl Pts',(6.71725767899343,22.5441456868779,5.97856451697804));
#43699=CARTESIAN_POINT('Ctrl Pts',(6.71725767899343,23.9780449912323,7.10420489788168));
#43700=CARTESIAN_POINT('Ctrl Pts',(6.71725767899343,24.9401367536043,8.13439441828645));
#43701=CARTESIAN_POINT('Ctrl Pts',(6.71725767899343,25.4248225617206,8.77129790636529));
#43702=CARTESIAN_POINT('Ctrl Pts',(6.71725767899343,25.5393355062252,8.92975375864079));
#43703=CARTESIAN_POINT('Ctrl Pts',(6.25443113011109,14.5720960327223,3.98151605950182));
#43704=CARTESIAN_POINT('Ctrl Pts',(6.25443113011109,14.9276602808206,3.94044126022634));
#43705=CARTESIAN_POINT('Ctrl Pts',(6.25443113011109,15.8947102355587,3.87264648589394));
#43706=CARTESIAN_POINT('Ctrl Pts',(6.25443113011109,17.4769468535728,3.95304531142131));
#43707=CARTESIAN_POINT('Ctrl Pts',(6.25443113011109,19.2795305784078,4.32755049662825));
#43708=CARTESIAN_POINT('Ctrl Pts',(6.25443113011109,21.0055160264994,4.97350307678813));
#43709=CARTESIAN_POINT('Ctrl Pts',(6.25443113011109,22.6120212527427,5.8768913876941));
#43710=CARTESIAN_POINT('Ctrl Pts',(6.25443113011109,24.0607369607973,7.01417317831217));
#43711=CARTESIAN_POINT('Ctrl Pts',(6.25443113011109,25.0326790181266,8.05491381308084));
#43712=CARTESIAN_POINT('Ctrl Pts',(6.25443113011109,25.5223371689888,8.69834807253971));
#43713=CARTESIAN_POINT('Ctrl Pts',(6.25443113011109,25.6380269437365,8.85843204246403));
#43714=CARTESIAN_POINT('Ctrl Pts',(6.99999999975116,14.796790812404,4.92966736369432));
#43715=CARTESIAN_POINT('Ctrl Pts',(6.99999999975279,14.9628120942143,4.9122434544952));
#43716=CARTESIAN_POINT('Ctrl Pts',(6.99999999939315,15.1287094965253,4.89864382129396));
#43717=CARTESIAN_POINT('Ctrl Pts',(6.99999999870943,15.294561887614,4.88880665018259));
#43718=CARTESIAN_POINT('Ctrl Pts',(6.99999999819716,15.4188238238608,4.88143632575454));
#43719=CARTESIAN_POINT('Ctrl Pts',(6.99999999754782,15.5430607645851,4.87617913713079));
#43720=CARTESIAN_POINT('Ctrl Pts',(6.99999999746715,15.667307619498,4.87302815224969));
#43721=CARTESIAN_POINT('Ctrl Pts',(6.99999999735909,15.8337151132274,4.86880794484717));
#43722=CARTESIAN_POINT('Ctrl Pts',(6.99999999919074,16.0001407341898,4.86836394895551));
#43723=CARTESIAN_POINT('Ctrl Pts',(6.99999999987887,16.166701195129,4.87172626796587));
#43724=CARTESIAN_POINT('Ctrl Pts',(6.99999999995352,16.1847696360791,4.87209101156799));
#43725=CARTESIAN_POINT('Ctrl Pts',(6.99999999999963,16.2028396593029,4.8725005976837));
#43726=CARTESIAN_POINT('Ctrl Pts',(6.99999999999963,16.2209114099307,4.87295510148193));
#43727=CARTESIAN_POINT('Ctrl Pts',(6.99999999999963,16.4297965262892,4.8782085537198));
#43728=CARTESIAN_POINT('Ctrl Pts',(6.9999999954667,16.6388913988277,4.88938135116946));
#43729=CARTESIAN_POINT('Ctrl Pts',(6.99999999503575,16.8476333268867,4.90651885872368));
#43730=CARTESIAN_POINT('Ctrl Pts',(6.99999999469175,17.0142564616812,4.92019845466208));
#43731=CARTESIAN_POINT('Ctrl Pts',(6.9999999963588,17.1806544793605,4.93767756116664));
#43732=CARTESIAN_POINT('Ctrl Pts',(6.99999999805313,17.3465410238682,4.95895540149735));
#43733=CARTESIAN_POINT('Ctrl Pts',(6.99999999906359,17.4454726952585,4.97164511249072));
#43734=CARTESIAN_POINT('Ctrl Pts',(6.99999999999963,17.544222462615,4.98568551449838));
#43735=CARTESIAN_POINT('Ctrl Pts',(6.99999999999963,17.6427305436046,5.00106284970836));
#43736=CARTESIAN_POINT('Ctrl Pts',(6.99999999999963,17.9064996520793,5.04223780670992));
#43737=CARTESIAN_POINT('Ctrl Pts',(6.99999999769782,18.1685324379956,5.09308743825919));
#43738=CARTESIAN_POINT('Ctrl Pts',(6.99999999858912,18.4283218652711,5.15338940372302));
#43739=CARTESIAN_POINT('Ctrl Pts',(6.9999999992438,18.619142849646,5.19768250883596));
#43740=CARTESIAN_POINT('Ctrl Pts',(6.99999999995071,18.808753796749,5.24707643234085));
#43741=CARTESIAN_POINT('Ctrl Pts',(6.99999999999527,18.9969552178462,5.30150090629035));
#43742=CARTESIAN_POINT('Ctrl Pts',(6.99999999999829,19.0096808723613,5.30518093723065));
#43743=CARTESIAN_POINT('Ctrl Pts',(6.99999999999963,19.0224000823289,5.30888397401697));
#43744=CARTESIAN_POINT('Ctrl Pts',(6.99999999999963,19.0351127865529,5.3126099921686));
#43745=CARTESIAN_POINT('Ctrl Pts',(6.99999999999963,19.3842397982826,5.41493704705863));
#43746=CARTESIAN_POINT('Ctrl Pts',(6.99999999999433,19.7284570030457,5.53457218802795));
#43747=CARTESIAN_POINT('Ctrl Pts',(6.99999999997183,20.0659266389262,5.67102983958899));
#43748=CARTESIAN_POINT('Ctrl Pts',(6.9999999999649,20.169893191372,5.71306927093113));
#43749=CARTESIAN_POINT('Ctrl Pts',(6.99999999999963,20.2732191475457,5.75670501823988));
#43750=CARTESIAN_POINT('Ctrl Pts',(6.99999999999963,20.3758503571618,5.80192197800648));
#43751=CARTESIAN_POINT('Ctrl Pts',(6.99999999999963,20.4434628840057,5.83171050839074));
#43752=CARTESIAN_POINT('Ctrl Pts',(6.99999999997007,20.5107752122269,5.86218302328723));
#43753=CARTESIAN_POINT('Ctrl Pts',(6.99999999992877,20.5777722436876,5.89333439996507));
#43754=CARTESIAN_POINT('Ctrl Pts',(6.99999999970392,20.9425747082302,6.06295533298561));
#43755=CARTESIAN_POINT('Ctrl Pts',(6.99999999999963,21.2980259815938,6.25270726283353));
#43756=CARTESIAN_POINT('Ctrl Pts',(6.99999999999963,21.6419501727056,6.4612030800231));
#43757=CARTESIAN_POINT('Ctrl Pts',(6.99999999999963,21.7796572872,6.5446847254302));
#43758=CARTESIAN_POINT('Ctrl Pts',(6.9999999996197,21.9155159097578,6.63117290946998));
#43759=CARTESIAN_POINT('Ctrl Pts',(6.99999999912184,22.0494139576794,6.72060682878888));
#43760=CARTESIAN_POINT('Ctrl Pts',(6.99999999824605,22.2849549618095,6.8779306694769));
#43761=CARTESIAN_POINT('Ctrl Pts',(6.99999999886115,22.5144315343706,7.04436836788122));
#43762=CARTESIAN_POINT('Ctrl Pts',(6.99999999981795,22.7372440058527,7.21957770321878));
#43763=CARTESIAN_POINT('Ctrl Pts',(6.99999999992514,22.7622055678981,7.23920631137463));
#43764=CARTESIAN_POINT('Ctrl Pts',(6.99999999999963,22.7870834467616,7.25894503891287));
#43765=CARTESIAN_POINT('Ctrl Pts',(6.99999999999963,22.8118767647635,7.27879342661068));
#43766=CARTESIAN_POINT('Ctrl Pts',(6.99999999999963,22.9845622066237,7.41703743249722));
#43767=CARTESIAN_POINT('Ctrl Pts',(6.99999999634261,23.1531796781679,7.56056973529903));
#43768=CARTESIAN_POINT('Ctrl Pts',(6.99999999541923,23.3172464672391,7.70901269845457));
#43769=CARTESIAN_POINT('Ctrl Pts',(6.99999999530942,23.3367573752257,7.72666561292783));
#43770=CARTESIAN_POINT('Ctrl Pts',(6.99999999523431,23.3562039693901,7.7443879310535));
#43771=CARTESIAN_POINT('Ctrl Pts',(6.99999999519885,23.3755854729976,7.76217898327269));
#43772=CARTESIAN_POINT('Ctrl Pts',(6.99999999489031,23.5442323268772,7.91698663105599));
#43773=CARTESIAN_POINT('Ctrl Pts',(6.99999999999963,23.7079469955236,8.07700145659367));
#43774=CARTESIAN_POINT('Ctrl Pts',(6.99999999999963,23.8663282356994,8.24167851093918));
#43775=CARTESIAN_POINT('Ctrl Pts',(6.99999999999963,23.9843305537447,8.36437154024027));
#43776=CARTESIAN_POINT('Ctrl Pts',(6.9999999974146,24.0993266000013,8.48968650811308));
#43777=CARTESIAN_POINT('Ctrl Pts',(6.99999999745781,24.2114124198125,8.61766946000518));
#43778=CARTESIAN_POINT('Ctrl Pts',(6.99999999749905,24.318376059481,8.73980375293336));
#43779=CARTESIAN_POINT('Ctrl Pts',(6.99999999865126,24.4226893685616,8.86436824503144));
#43780=CARTESIAN_POINT('Ctrl Pts',(6.99999999924035,24.5244042559699,8.99143397814575));
#43781=CARTESIAN_POINT('Ctrl Pts',(6.99999999975839,24.6138515921833,9.10317466469306));
#43782=CARTESIAN_POINT('Ctrl Pts',(6.99999999990826,24.7012891768634,9.21685021183985));
#43783=CARTESIAN_POINT('Ctrl Pts',(6.9999999998936,24.7867157008319,9.33251047980519));
#43784=CARTESIAN_POINT('Ctrl Pts',(6.26386081936141,15.8144408559214,3.90572621533164));
#43785=CARTESIAN_POINT('Ctrl Pts',(6.2646071571378,16.0736401969478,3.90306654962963));
#43786=CARTESIAN_POINT('Ctrl Pts',(6.26531568508263,16.3306804620868,3.90881650033525));
#43787=CARTESIAN_POINT('Ctrl Pts',(6.26598638626061,16.5850686264647,3.92256316414692));
#43788=CARTESIAN_POINT('Ctrl Pts',(6.2666647366093,16.8423580210206,3.93646660504761));
#43789=CARTESIAN_POINT('Ctrl Pts',(6.26730439248674,17.0969345331479,3.95855018426228));
#43790=CARTESIAN_POINT('Ctrl Pts',(6.2679053397188,17.3483408478098,3.98839324939858));
#43791=CARTESIAN_POINT('Ctrl Pts',(6.26800176544167,17.3886805554093,3.99318175490248));
#43792=CARTESIAN_POINT('Ctrl Pts',(6.26809719457051,17.4289387505187,3.99817005148869));
#43793=CARTESIAN_POINT('Ctrl Pts',(6.26819162705404,17.4691136669068,4.00335641724054));
#43794=CARTESIAN_POINT('Ctrl Pts',(6.26876871455366,17.7146270875046,4.03505088012148));
#43795=CARTESIAN_POINT('Ctrl Pts',(6.26930858144218,17.9570264035881,4.07414071626594));
#43796=CARTESIAN_POINT('Ctrl Pts',(6.26981121749717,18.1959031194725,4.12010910859023));
#43797=CARTESIAN_POINT('Ctrl Pts',(6.27017912394857,18.37074987786,4.15375585543381));
#43798=CARTESIAN_POINT('Ctrl Pts',(6.27052708379087,18.5437104294303,4.19108825682538));
#43799=CARTESIAN_POINT('Ctrl Pts',(6.27085509380364,18.7146409206978,4.2319103480927));
#43800=CARTESIAN_POINT('Ctrl Pts',(6.27121137830344,18.9003056327786,4.27625130660444));
#43801=CARTESIAN_POINT('Ctrl Pts',(6.27154412415377,19.0835749911811,4.3247094130082));
#43802=CARTESIAN_POINT('Ctrl Pts',(6.27185332727448,19.2642823708993,4.37704091251744));
#43803=CARTESIAN_POINT('Ctrl Pts',(6.27227096880013,19.5083643374345,4.44772521623471));
#43804=CARTESIAN_POINT('Ctrl Pts',(6.27264565893848,19.7477705540641,4.5254749182099));
#43805=CARTESIAN_POINT('Ctrl Pts',(6.27297738975663,19.9821808854897,4.60968099294868));
#43806=CARTESIAN_POINT('Ctrl Pts',(6.27330912057479,20.2165912169153,4.69388706768746));
#43807=CARTESIAN_POINT('Ctrl Pts',(6.27359789209192,20.4460058483219,4.78454958019296));
#43808=CARTESIAN_POINT('Ctrl Pts',(6.27384369851774,20.6701561188015,4.88108731632356));
#43809=CARTESIAN_POINT('Ctrl Pts',(6.27395596467506,20.7725313494162,4.92517859927516));
#43810=CARTESIAN_POINT('Ctrl Pts',(6.274059268442,20.8738091329866,4.97049582165233));
#43811=CARTESIAN_POINT('Ctrl Pts',(6.27415361644308,20.9739672996456,5.01698549278479));
#43812=CARTESIAN_POINT('Ctrl Pts',(6.27415652008545,20.9770497549524,5.01841625313386));
#43813=CARTESIAN_POINT('Ctrl Pts',(6.27415941518457,20.9801311498554,5.01984812399059));
#43814=CARTESIAN_POINT('Ctrl Pts',(6.27416230174624,20.9832114837509,5.02128110381964));
#43815=CARTESIAN_POINT('Ctrl Pts',(6.27420631168368,21.0301757676948,5.04312901831916));
#43816=CARTESIAN_POINT('Ctrl Pts',(6.27424833704542,21.0768934073318,5.0652347129111));
#43817=CARTESIAN_POINT('Ctrl Pts',(6.27428839844132,21.1233627191961,5.08759195320009));
#43818=CARTESIAN_POINT('Ctrl Pts',(6.27431785052249,21.1575257310999,5.10402840632335));
#43819=CARTESIAN_POINT('Ctrl Pts',(6.2743467018383,21.1921534486782,5.12089383929234));
#43820=CARTESIAN_POINT('Ctrl Pts',(6.27437398824107,21.2260047646262,5.13758092935802));
#43821=CARTESIAN_POINT('Ctrl Pts',(6.27438625179811,21.2412188456975,5.14508074831611));
#43822=CARTESIAN_POINT('Ctrl Pts',(6.27439819925053,21.2562764111607,5.15254389876329));
#43823=CARTESIAN_POINT('Ctrl Pts',(6.27440974306803,21.2710663093239,5.15991218758797));
#43824=CARTESIAN_POINT('Ctrl Pts',(6.27456064722751,21.4644041849283,5.25623261471226));
#43825=CARTESIAN_POINT('Ctrl Pts',(6.27467736526253,21.6577059358034,5.35907904466896));
#43826=CARTESIAN_POINT('Ctrl Pts',(6.27475989543337,21.8504727943955,5.46870199605282));
#43827=CARTESIAN_POINT('Ctrl Pts',(6.27484107212138,22.0400783044643,5.57652714693292));
#43828=CARTESIAN_POINT('Ctrl Pts',(6.27488917310781,22.2291663735341,5.69090844126615));
#43829=CARTESIAN_POINT('Ctrl Pts',(6.27490419770935,22.4172141919104,5.81206904072998));
#43830=CARTESIAN_POINT('Ctrl Pts',(6.27490863155076,22.4727081231324,5.84782419083762));
#43831=CARTESIAN_POINT('Ctrl Pts',(6.2749101848683,22.5281111352571,5.88416962570433));
#43832=CARTESIAN_POINT('Ctrl Pts',(6.27490885766006,22.5834089609015,5.92111080776558));
#43833=CARTESIAN_POINT('Ctrl Pts',(6.27490450925621,22.7645842052217,6.04214319208507));
#43834=CARTESIAN_POINT('Ctrl Pts',(6.27486923980178,22.9446338346503,6.16957223798428));
#43835=CARTESIAN_POINT('Ctrl Pts',(6.2748030497645,23.1230233225777,6.30354224822262));
#43836=CARTESIAN_POINT('Ctrl Pts',(6.27475277111024,23.258529869426,6.40530728875025));
#43837=CARTESIAN_POINT('Ctrl Pts',(6.27468465104014,23.3930775980555,6.51084612431001));
#43838=CARTESIAN_POINT('Ctrl Pts',(6.27459869008054,23.5264138891986,6.62021363206385));
#43839=CARTESIAN_POINT('Ctrl Pts',(6.27448994557249,23.6950903378017,6.7585684838625));
#43840=CARTESIAN_POINT('Ctrl Pts',(6.27435264847565,23.8618295446342,6.90305124022513));
#43841=CARTESIAN_POINT('Ctrl Pts',(6.27418680127018,24.026082061508,7.05375519723077));
#43842=CARTESIAN_POINT('Ctrl Pts',(6.27401315139378,24.1980622234404,7.21154937550556));
#43843=CARTESIAN_POINT('Ctrl Pts',(6.27380820178873,24.3673155362908,7.37616474895342));
#43844=CARTESIAN_POINT('Ctrl Pts',(6.2735719562331,24.5332726200832,7.54763344678315));
#43845=CARTESIAN_POINT('Ctrl Pts',(6.27333930371878,24.6967056747693,7.71649428977333));
#43846=CARTESIAN_POINT('Ctrl Pts',(6.27307629996608,24.8569420194823,7.89200164036484));
#43847=CARTESIAN_POINT('Ctrl Pts',(6.2727829495743,25.0133992150722,8.07415384833901));
#43848=CARTESIAN_POINT('Ctrl Pts',(6.27261681774183,25.1020049280167,8.17731130422409));
#43849=CARTESIAN_POINT('Ctrl Pts',(6.27244095301194,25.1893978688721,8.28259933546736));
#43850=CARTESIAN_POINT('Ctrl Pts',(6.27225535637375,25.2754665765764,8.39001281171685));
#43851=CARTESIAN_POINT('Ctrl Pts',(6.27204648360049,25.3723293745519,8.51089727864247));
#43852=CARTESIAN_POINT('Ctrl Pts',(6.27182528484287,25.46751518399,8.63447390404182));
#43853=CARTESIAN_POINT('Ctrl Pts',(6.27159176169396,25.5608443101225,8.76072155999657));
#43854=CARTESIAN_POINT('Ctrl Pts',(-6.390310997207,15.4599632088997,3.94962478603215));
#43855=CARTESIAN_POINT('Ctrl Pts',(-4.260207331471,16.2180720984124,3.32898409023249));
#43856=CARTESIAN_POINT('Ctrl Pts',(0.0001535202166307,16.9761997022964,
2.70679304528151));
#43857=CARTESIAN_POINT('Ctrl Pts',(4.260514371904,16.2180174588604,3.32902893260671));
#43858=CARTESIAN_POINT('Ctrl Pts',(6.390771557857,15.4597992883758,3.9497589827666));
#43859=CARTESIAN_POINT('Ctrl Pts',(-6.390310997207,16.2401119443479,3.91822480441049));
#43860=CARTESIAN_POINT('Ctrl Pts',(-4.260207331471,16.9588864514405,3.34432399295645));
#43861=CARTESIAN_POINT('Ctrl Pts',(0.0001535202166307,17.6776685616714,
2.76847544297843));
#43862=CARTESIAN_POINT('Ctrl Pts',(4.260514371904,16.9588346475797,3.34436549534545));
#43863=CARTESIAN_POINT('Ctrl Pts',(6.390771557857,16.2399565288181,3.91834889490668));
#43864=CARTESIAN_POINT('Ctrl Pts',(-6.390310997207,18.1257229797427,4.02649557071453));
#43865=CARTESIAN_POINT('Ctrl Pts',(-4.260207331471,18.7393790303087,3.53810403696184));
#43866=CARTESIAN_POINT('Ctrl Pts',(0.0001535202166307,19.3530131910523,
3.05102600446442));
#43867=CARTESIAN_POINT('Ctrl Pts',(4.260514371904,18.7393348046511,3.53813914151219));
#43868=CARTESIAN_POINT('Ctrl Pts',(6.390771557857,18.125590293236,4.02660117217093));
#43869=CARTESIAN_POINT('Ctrl Pts',(-6.390310997207,21.0044951210711,4.89945800148705));
#43870=CARTESIAN_POINT('Ctrl Pts',(-4.260207331471,21.442483951078,4.44478850538388));
#43871=CARTESIAN_POINT('Ctrl Pts',(0.0001535202166307,21.8807678511965,
3.98943347064864));
#43872=CARTESIAN_POINT('Ctrl Pts',(4.260514371904,21.4424523632066,4.44482132360082));
#43873=CARTESIAN_POINT('Ctrl Pts',(6.390771557857,21.0044004178526,4.89955631145292));
#43874=CARTESIAN_POINT('Ctrl Pts',(-6.390310997207,23.7052293934154,6.63374483550749));
#43875=CARTESIAN_POINT('Ctrl Pts',(-4.260207331471,23.9981328584314,6.09525951521535));
#43876=CARTESIAN_POINT('Ctrl Pts',(0.000153520216631,24.2900557545739,5.55782195886724));
#43877=CARTESIAN_POINT('Ctrl Pts',(4.260514371904,23.9981118190468,6.09529824925896));
#43878=CARTESIAN_POINT('Ctrl Pts',(6.390771557857,23.7051660609652,6.63386126838838));
#43879=CARTESIAN_POINT('Ctrl Pts',(-6.390310997207,25.1149841603859,8.1839487906061));
#43880=CARTESIAN_POINT('Ctrl Pts',(-4.260207331471,25.3660581844935,7.53598959785924));
#43881=CARTESIAN_POINT('Ctrl Pts',(0.0001535202166303,25.6190363056788,
6.88615830217486));
#43882=CARTESIAN_POINT('Ctrl Pts',(4.260514371904,25.3660399519323,7.53603643231476));
#43883=CARTESIAN_POINT('Ctrl Pts',(6.390771557857,25.1149298724386,8.18408889422398));
#43884=CARTESIAN_POINT('Ctrl Pts',(-6.390310997207,25.680737599168,8.98426054544063));
#43885=CARTESIAN_POINT('Ctrl Pts',(-4.260207331471,25.9287994959116,8.27687328339766));
#43886=CARTESIAN_POINT('Ctrl Pts',(0.0001535202166303,26.1774666691521,
7.56887710148171));
#43887=CARTESIAN_POINT('Ctrl Pts',(4.260514371904,25.9287815740455,8.27692430989529));
#43888=CARTESIAN_POINT('Ctrl Pts',(6.390771557857,25.6806839625015,8.98441349877858));
#43889=CARTESIAN_POINT('Ctrl Pts',(-6.26386059984685,15.8144217559904,3.90573753014116));
#43890=CARTESIAN_POINT('Ctrl Pts',(-5.97539333098954,15.9103760885445,3.82576732795924));
#43891=CARTESIAN_POINT('Ctrl Pts',(-5.68507999445153,15.9990640254287,3.75075426795588));
#43892=CARTESIAN_POINT('Ctrl Pts',(-5.39340845737568,16.0805744084132,3.68097248655366));
#43893=CARTESIAN_POINT('Ctrl Pts',(-5.11949030830525,16.1571234383974,3.61543816465115));
#43894=CARTESIAN_POINT('Ctrl Pts',(-4.84437426792527,16.2273417544319,3.55451825621326));
#43895=CARTESIAN_POINT('Ctrl Pts',(-4.5684644297166,16.2913404726591,3.49841824263205));
#43896=CARTESIAN_POINT('Ctrl Pts',(-4.31194165949948,16.3508422598971,3.44626015002287));
#43897=CARTESIAN_POINT('Ctrl Pts',(-4.05473272615563,16.4049677060134,3.39826866251004));
#43898=CARTESIAN_POINT('Ctrl Pts',(-3.79716238633167,16.453842265351,3.35458408540851));
#43899=CARTESIAN_POINT('Ctrl Pts',(-3.57726994290746,16.4955673579271,3.31728977424918));
#43900=CARTESIAN_POINT('Ctrl Pts',(-3.35711409398038,16.5334658330865,3.28313426378421));
#43901=CARTESIAN_POINT('Ctrl Pts',(-3.13689690935008,16.5676399602686,3.25218673091632));
#43902=CARTESIAN_POINT('Ctrl Pts',(-2.89863169006324,16.6046148490387,3.21870287397966));
#43903=CARTESIAN_POINT('Ctrl Pts',(-2.6602852319021,16.6372510250138,3.18897493478523));
#43904=CARTESIAN_POINT('Ctrl Pts',(-2.42210555319733,16.6655736606144,3.16305553873815));
#43905=CARTESIAN_POINT('Ctrl Pts',(-2.18716847768624,16.6935107088753,3.13748901207462));
#43906=CARTESIAN_POINT('Ctrl Pts',(-1.95239367143694,16.7172508562373,3.11562807350144));
#43907=CARTESIAN_POINT('Ctrl Pts',(-1.71801916041739,16.7368573333217,3.09749090364961));
#43908=CARTESIAN_POINT('Ctrl Pts',(-1.48507356908385,16.7563442748775,3.07946431134709));
#43909=CARTESIAN_POINT('Ctrl Pts',(-1.25252340686986,16.7717477586243,3.06511627751505));
#43910=CARTESIAN_POINT('Ctrl Pts',(-1.02060237268687,16.7831691638654,3.05443172704252));
#43911=CARTESIAN_POINT('Ctrl Pts',(-0.790162778168551,16.7945176127108,
3.04381542616591));
#43912=CARTESIAN_POINT('Ctrl Pts',(-0.560344300001652,16.8019346801216,
3.03681598687228));
#43913=CARTESIAN_POINT('Ctrl Pts',(-0.331376187254698,16.8055591055299,
3.03338536086241));
#43914=CARTESIAN_POINT('Ctrl Pts',(-0.220817153790872,16.8073091875182,
3.03172885642048));
#43915=CARTESIAN_POINT('Ctrl Pts',(-0.110456384411538,16.8081755976358,
3.0309039262618));
#43916=CARTESIAN_POINT('Ctrl Pts',(-0.000319687765395044,16.8081772730686,
3.03090233350032));
#43917=CARTESIAN_POINT('Ctrl Pts',(-0.000213125382396117,16.8081772746896,
3.03090233195925));
#43918=CARTESIAN_POINT('Ctrl Pts',(-0.000106562793408779,16.8081772755014,
3.03090233118879));
#43919=CARTESIAN_POINT('Ctrl Pts',(1.54364816055824E-12,16.8081772755037,
3.03090233118895));
#43920=CARTESIAN_POINT('Ctrl Pts',(0.229814767883462,16.8081772805917,3.03090233154421));
#43921=CARTESIAN_POINT('Ctrl Pts',(0.460587477671531,16.8044096604372,3.03448931169225));
#43922=CARTESIAN_POINT('Ctrl Pts',(0.692092742459731,16.7967144780101,3.04172791113162));
#43923=CARTESIAN_POINT('Ctrl Pts',(0.92542107169346,16.7889586973348,3.04902351330604));
#43924=CARTESIAN_POINT('Ctrl Pts',(1.15949353884638,16.7772132495556,3.06002845784822));
#43925=CARTESIAN_POINT('Ctrl Pts',(1.39407939032145,16.7613548321441,3.07477450403601));
#43926=CARTESIAN_POINT('Ctrl Pts',(1.63013438285027,16.7453970982055,3.08961290030245));
#43927=CARTESIAN_POINT('Ctrl Pts',(1.86670921018194,16.7252747476301,3.10823935315465));
#43928=CARTESIAN_POINT('Ctrl Pts',(2.10356875608892,16.7009027147165,3.13065201869609));
#43929=CARTESIAN_POINT('Ctrl Pts',(2.34326327402721,16.6762389729281,3.15333294144335));
#43930=CARTESIAN_POINT('Ctrl Pts',(2.5832493669223,16.647223228046,3.17989120946434));
#43931=CARTESIAN_POINT('Ctrl Pts',(2.82328337477861,16.6138084331694,3.21029066606775));
#43932=CARTESIAN_POINT('Ctrl Pts',(2.92752592620592,16.599296974962,3.22349261585247));
#43933=CARTESIAN_POINT('Ctrl Pts',(3.03177751445368,16.5839563689886,3.23741858935517));
#43934=CARTESIAN_POINT('Ctrl Pts',(3.13601818225799,16.567785112841,3.2520636894151));
#43935=CARTESIAN_POINT('Ctrl Pts',(3.39880739691305,16.5270176101711,3.28898377467892));
#43936=CARTESIAN_POINT('Ctrl Pts',(3.66152138150451,16.4809439402936,3.33047470854717));
#43937=CARTESIAN_POINT('Ctrl Pts',(3.92381607763906,16.4293925584389,3.37641707163315));
#43938=CARTESIAN_POINT('Ctrl Pts',(4.19336645804413,16.3764151448881,3.42363030784813));
#43939=CARTESIAN_POINT('Ctrl Pts',(4.46247403215353,16.3176531431208,3.47554420302421));
#43940=CARTESIAN_POINT('Ctrl Pts',(4.73076539208801,16.2529691538375,3.53199295300502));
#43941=CARTESIAN_POINT('Ctrl Pts',(5.02425998648815,16.182208764075,3.59374448680043));
#43942=CARTESIAN_POINT('Ctrl Pts',(5.31677781390168,16.1043615550116,3.66092253642902));
#43943=CARTESIAN_POINT('Ctrl Pts',(5.60783003770296,16.0193026037346,3.73327326415423));
#43944=CARTESIAN_POINT('Ctrl Pts',(5.82741016918173,15.9551311108633,3.78785722197113));
#43945=CARTESIAN_POINT('Ctrl Pts',(6.04615611875628,15.886856153891,3.84538443185739));
#43946=CARTESIAN_POINT('Ctrl Pts',(6.26385797789322,15.8144409706466,3.9057366018783));
#43947=CARTESIAN_POINT('Ctrl Pts',(-6.38267922172612,15.7738523078598,3.93899334286503));
#43948=CARTESIAN_POINT('Ctrl Pts',(-6.32178394100786,15.7957619893123,3.92177794388969));
#43949=CARTESIAN_POINT('Ctrl Pts',(-5.68007566712876,16.0226513783196,3.74296990775899));
#43950=CARTESIAN_POINT('Ctrl Pts',(-4.3405628786162,16.4113546400769,3.42585487548982));
#43951=CARTESIAN_POINT('Ctrl Pts',(-2.26159155672449,16.7779842233051,3.11137634163404));
#43952=CARTESIAN_POINT('Ctrl Pts',(-0.000322645265903455,16.9116027729772,
2.99296782877783));
#43953=CARTESIAN_POINT('Ctrl Pts',(2.26104630018457,16.7780550953811,3.11131422928351));
#43954=CARTESIAN_POINT('Ctrl Pts',(4.34024112533146,16.4114385643274,3.42578519270288));
#43955=CARTESIAN_POINT('Ctrl Pts',(5.67995509241135,16.0226928958199,3.74293703686325));
#43956=CARTESIAN_POINT('Ctrl Pts',(6.32176875644207,15.7957675033798,3.92177361735684));
#43957=CARTESIAN_POINT('Ctrl Pts',(6.38269140808456,15.7738479232639,3.93899678720638));
#43958=CARTESIAN_POINT('Ctrl Pts',(-6.17947932752834,15.1606870779192,3.89075783424522));
#43959=CARTESIAN_POINT('Ctrl Pts',(-6.12049144092706,15.1819034727368,3.87432042702319));
#43960=CARTESIAN_POINT('Ctrl Pts',(-5.49889172536448,15.4016154015587,3.70358699318366));
#43961=CARTESIAN_POINT('Ctrl Pts',(-4.20155201647089,15.7780515103907,3.40068046498789));
#43962=CARTESIAN_POINT('Ctrl Pts',(-2.18881221307725,16.1330771577479,3.10022483933076));
#43963=CARTESIAN_POINT('Ctrl Pts',(-0.000312236874671785,16.2624448571322,
2.98709891979729));
#43964=CARTESIAN_POINT('Ctrl Pts',(2.18828441451265,16.1331457801785,3.10016549602611));
#43965=CARTESIAN_POINT('Ctrl Pts',(4.2012404201408,15.7781327862976,3.40061389543627));
#43966=CARTESIAN_POINT('Ctrl Pts',(5.49877493126362,15.4016556064113,3.70355560477545));
#43967=CARTESIAN_POINT('Ctrl Pts',(6.12047673185723,15.18190881228,3.87431629610783));
#43968=CARTESIAN_POINT('Ctrl Pts',(6.17949113217087,15.1606828320346,3.89076112296309));
#43969=CARTESIAN_POINT('Ctrl Pts',(-6.17606942198722,14.7511100720048,3.39035617507167));
#43970=CARTESIAN_POINT('Ctrl Pts',(-6.11724876379497,14.7720723442377,3.37412570862358));
#43971=CARTESIAN_POINT('Ctrl Pts',(-5.49737410508965,14.9891714302522,3.20552395379427));
#43972=CARTESIAN_POINT('Ctrl Pts',(-4.20278204043645,15.3615316584505,2.90602013925078));
#43973=CARTESIAN_POINT('Ctrl Pts',(-2.19095873851463,15.7134382585734,2.60822212402352));
#43974=CARTESIAN_POINT('Ctrl Pts',(-0.000312652823461832,15.841880384075,
2.4958818195532));
#43975=CARTESIAN_POINT('Ctrl Pts',(2.19043080442953,15.7135063490568,2.6081632346203));
#43976=CARTESIAN_POINT('Ctrl Pts',(4.20247098821445,15.3616121052018,2.90595426953607));
#43977=CARTESIAN_POINT('Ctrl Pts',(5.49725762526239,14.9892111622839,3.20549295254849));
#43978=CARTESIAN_POINT('Ctrl Pts',(6.11723409695662,14.77207761954,3.37412162987566));
#43979=CARTESIAN_POINT('Ctrl Pts',(6.17608119319573,14.7511058769368,3.39035942228679));
#43980=CARTESIAN_POINT('Ctrl Pts',(-6.37318055258469,14.8203254139217,2.77953975667807));
#43981=CARTESIAN_POINT('Ctrl Pts',(-6.31268764295094,14.8416410144565,2.76280981911965));
#43982=CARTESIAN_POINT('Ctrl Pts',(-5.67513346514493,15.0624217826566,2.58900295618313));
#43983=CARTESIAN_POINT('Ctrl Pts',(-4.34231715275912,15.4415875234496,2.27988148674971));
#43984=CARTESIAN_POINT('Ctrl Pts',(-2.26599033350655,15.800901109489,1.97166918135384));
#43985=CARTESIAN_POINT('Ctrl Pts',(-0.000323526748717448,15.9323422860991,
1.85512198255444));
#43986=CARTESIAN_POINT('Ctrl Pts',(2.2654449005586,15.8009707317227,1.97160814218462));
#43987=CARTESIAN_POINT('Ctrl Pts',(4.3419967397778,15.4416695062744,2.27981344950243));
#43988=CARTESIAN_POINT('Ctrl Pts',(5.67501364814971,15.0624621946197,2.58897099373883));
#43989=CARTESIAN_POINT('Ctrl Pts',(6.31267255995101,14.8416463783418,2.76280561495848));
#43990=CARTESIAN_POINT('Ctrl Pts',(6.37319265849431,14.8203211481087,2.7795431036554));
#43991=CARTESIAN_POINT('Ctrl Pts',(-6.24994620506134,14.8593873451939,2.76546786777471));
#43992=CARTESIAN_POINT('Ctrl Pts',(-6.22850662278677,14.8667761577535,2.75964861829393));
#43993=CARTESIAN_POINT('Ctrl Pts',(-6.20704358783532,14.8741272855027,2.7538527902599));
#43994=CARTESIAN_POINT('Ctrl Pts',(-6.18555718293149,14.8814406700516,2.74808058402306));
#43995=CARTESIAN_POINT('Ctrl Pts',(-5.88365929671791,14.9841984532296,2.6669773529572));
#43996=CARTESIAN_POINT('Ctrl Pts',(-5.5771472884225,15.0795079506171,2.59053465810836));
#43997=CARTESIAN_POINT('Ctrl Pts',(-5.26630871828218,15.1671888464119,2.51936495347675));
#43998=CARTESIAN_POINT('Ctrl Pts',(-5.13424536371906,15.2044410870992,2.48912768294538));
#43999=CARTESIAN_POINT('Ctrl Pts',(-5.00140109970354,15.2403158616087,2.45984266059681));
#44000=CARTESIAN_POINT('Ctrl Pts',(-4.86779840574354,15.274797334949,2.43155887951409));
#44001=CARTESIAN_POINT('Ctrl Pts',(-4.71600682495683,15.3139731718355,2.39942449873238));
#44002=CARTESIAN_POINT('Ctrl Pts',(-4.56323915278791,15.3513507651254,2.36857718708611));
#44003=CARTESIAN_POINT('Ctrl Pts',(-4.40952973635834,15.3869070844585,2.33907600634009));
#44004=CARTESIAN_POINT('Ctrl Pts',(-4.32504469211605,15.4064503062189,2.32286093885482));
#44005=CARTESIAN_POINT('Ctrl Pts',(-4.24027512903501,15.4254432749396,2.30705258251815));
#44006=CARTESIAN_POINT('Ctrl Pts',(-4.15522924912161,15.4438822756036,2.29165974001541));
#44007=CARTESIAN_POINT('Ctrl Pts',(-4.03534141761238,15.4698754431393,2.26996069345026));
#44008=CARTESIAN_POINT('Ctrl Pts',(-3.91490275773383,15.4947680749842,2.24908777917226));
#44009=CARTESIAN_POINT('Ctrl Pts',(-3.79393281020035,15.5185497764201,2.22906479297264));
#44010=CARTESIAN_POINT('Ctrl Pts',(-3.73344783643362,15.530440627138,2.21905329987282));
#44011=CARTESIAN_POINT('Ctrl Pts',(-3.67283003770224,15.5420537317391,2.20925428665817));
#44012=CARTESIAN_POINT('Ctrl Pts',(-3.61208195660669,15.5533877223801,2.19967049112853));
#44013=CARTESIAN_POINT('Ctrl Pts',(-3.58170791605892,15.5590547177007,2.19487859336371));
#44014=CARTESIAN_POINT('Ctrl Pts',(-3.55130130475809,15.5646519336992,2.1901404998973));
#44015=CARTESIAN_POINT('Ctrl Pts',(-3.52086244284463,15.5701791947916,2.18545654570334));
#44016=CARTESIAN_POINT('Ctrl Pts',(-3.5056430118879,15.5729428253378,2.18311456860636));
#44017=CARTESIAN_POINT('Ctrl Pts',(-3.49041551826924,15.5756889671052,2.18078612632016));
#44018=CARTESIAN_POINT('Ctrl Pts',(-3.47518000234777,15.578417597879,2.17847125990129));
#44019=CARTESIAN_POINT('Ctrl Pts',(-3.46756224438704,15.5797819132659,2.17731382669186));
#44020=CARTESIAN_POINT('Ctrl Pts',(-3.45994248085009,15.5811418509012,2.17615978744881));
#44021=CARTESIAN_POINT('Ctrl Pts',(-3.45232071680447,15.5824974079916,2.17500914725054));
#44022=CARTESIAN_POINT('Ctrl Pts',(-3.44469895275884,15.583852965082,2.17385850705228));
#44023=CARTESIAN_POINT('Ctrl Pts',(-3.43823529095624,15.5849992547046,2.17288527721797));
#44024=CARTESIAN_POINT('Ctrl Pts',(-3.42944942821482,15.586550934823,2.17156742885132));
#44025=CARTESIAN_POINT('Ctrl Pts',(-3.13033149385742,15.6393784561986,2.12670079562151));
#44026=CARTESIAN_POINT('Ctrl Pts',(-2.82949174433291,15.6852093579706,2.08740015843555));
#44027=CARTESIAN_POINT('Ctrl Pts',(-2.52723878681692,15.7240366908818,2.0539476436804));
#44028=CARTESIAN_POINT('Ctrl Pts',(-2.45239387379483,15.7336512481007,2.04566401735034));
#44029=CARTESIAN_POINT('Ctrl Pts',(-2.37746220520499,15.7428361780922,2.03773911348895));
#44030=CARTESIAN_POINT('Ctrl Pts',(-2.30244828060811,15.7515910036884,2.03017748529987));
#44031=CARTESIAN_POINT('Ctrl Pts',(-2.00299346058271,15.7865401779562,1.99999154288147));
#44032=CARTESIAN_POINT('Ctrl Pts',(-1.70222881863287,15.814638248534,1.97559222184925));
#44033=CARTESIAN_POINT('Ctrl Pts',(-1.40053607615597,15.8358823134265,1.95708487572244));
#44034=CARTESIAN_POINT('Ctrl Pts',(-1.10085973549657,15.8569843909093,1.93870122579747));
#44035=CARTESIAN_POINT('Ctrl Pts',(-0.800267108626436,15.871323783777,1.92613092772216));
#44036=CARTESIAN_POINT('Ctrl Pts',(-0.49912433318855,15.8788593394164,1.91951016285445));
#44037=CARTESIAN_POINT('Ctrl Pts',(-0.333015939771273,15.8830159028237,
1.91585819207822));
#44038=CARTESIAN_POINT('Ctrl Pts',(-0.166740066804234,15.8851016845639,
1.91401699144391));
#44039=CARTESIAN_POINT('Ctrl Pts',(-0.000358043406942927,15.8851047148172,
1.91401397084702));
#44040=CARTESIAN_POINT('Ctrl Pts',(-0.000345565863738448,15.8851047150445,
1.9140139706205));
#44041=CARTESIAN_POINT('Ctrl Pts',(-0.000333088319937549,15.88510471526,
1.91401397040431));
#44042=CARTESIAN_POINT('Ctrl Pts',(-0.000320610775539605,15.8851047154638,
1.91401397019847));
#44043=CARTESIAN_POINT('Ctrl Pts',(0.29646157639871,15.8851095633514,1.91400907409693));
#44044=CARTESIAN_POINT('Ctrl Pts',(0.592899678854785,15.878495752609,1.91980212803821));
#44045=CARTESIAN_POINT('Ctrl Pts',(0.888657766029018,15.8653161400331,1.93130344475154));
#44046=CARTESIAN_POINT('Ctrl Pts',(1.16839169566267,15.8528505981704,1.94218162073286));
#44047=CARTESIAN_POINT('Ctrl Pts',(1.44751760548253,15.8345110681381,1.95816672185245));
#44048=CARTESIAN_POINT('Ctrl Pts',(1.72573998854356,15.8103111796674,1.97921018196904));
#44049=CARTESIAN_POINT('Ctrl Pts',(1.91823927201675,15.7935675189328,1.99376994150266));
#44050=CARTESIAN_POINT('Ctrl Pts',(2.11031101581594,15.7740195872836,2.01073408711409));
#44051=CARTESIAN_POINT('Ctrl Pts',(2.30185594488252,15.7516674948778,2.03006063174667));
#44052=CARTESIAN_POINT('Ctrl Pts',(2.39508333324716,15.7407884431084,2.03946711037802));
#44053=CARTESIAN_POINT('Ctrl Pts',(2.48818591806944,15.7292450158588,2.04943330100437));
#44054=CARTESIAN_POINT('Ctrl Pts',(2.58115534057936,15.7170382210193,2.05994866323696));
#44055=CARTESIAN_POINT('Ctrl Pts',(2.7231475081323,15.6983947873899,2.07600877241801));
#44056=CARTESIAN_POINT('Ctrl Pts',(2.86482602552771,15.6782037050381,2.09335491489588));
#44057=CARTESIAN_POINT('Ctrl Pts',(3.00615411766162,15.6564670213138,2.11195842960335));
#44058=CARTESIAN_POINT('Ctrl Pts',(3.07681816372858,15.6455986794516,2.12126018695709));
#44059=CARTESIAN_POINT('Ctrl Pts',(3.14739460189104,15.6343439150781,2.13087628464253));
#44060=CARTESIAN_POINT('Ctrl Pts',(3.21787891819181,15.6227029013609,2.14080264019682));
#44061=CARTESIAN_POINT('Ctrl Pts',(3.25312107634219,15.6168823945023,2.14576581797396));
#44062=CARTESIAN_POINT('Ctrl Pts',(3.28834020388962,15.6109653238857,2.15080656003985));
#44063=CARTESIAN_POINT('Ctrl Pts',(3.3235357385418,15.6049517039844,2.15592434168264));
#44064=CARTESIAN_POINT('Ctrl Pts',(3.34113350586789,15.6019448940338,2.15848323250403));
#44065=CARTESIAN_POINT('Ctrl Pts',(3.35872537495863,15.5989139466725,2.16106138320784));
#44066=CARTESIAN_POINT('Ctrl Pts',(3.37631127579107,15.595858863346,2.16365872650413));
#44067=CARTESIAN_POINT('Ctrl Pts',(3.38510422620729,15.5943313216828,2.16495739815227));
#44068=CARTESIAN_POINT('Ctrl Pts',(3.39389568455815,15.5927977460227,2.16626086794778));
#44069=CARTESIAN_POINT('Ctrl Pts',(3.40268564210845,15.5912581365241,2.16756912736822));
#44070=CARTESIAN_POINT('Ctrl Pts',(3.41147559965875,15.5897185270255,2.16887738678867));
#44071=CARTESIAN_POINT('Ctrl Pts',(3.42142413678522,15.5879680264099,2.17036441991536));
#44072=CARTESIAN_POINT('Ctrl Pts',(3.42905100362602,15.586621206652,2.17150826594686));
#44073=CARTESIAN_POINT('Ctrl Pts',(3.74300305951125,15.5311807694804,2.21859350038224));
#44074=CARTESIAN_POINT('Ctrl Pts',(4.05359391333256,15.468300785322,2.27151445346201));
#44075=CARTESIAN_POINT('Ctrl Pts',(4.36044446898295,15.398179554136,2.32979150920995));
#44076=CARTESIAN_POINT('Ctrl Pts',(4.37670544692025,15.3944636091189,2.33287979404541));
#44077=CARTESIAN_POINT('Ctrl Pts',(4.39295592218156,15.3907273205417,2.33598312911675));
#44078=CARTESIAN_POINT('Ctrl Pts',(4.40919583866862,15.3869707151934,2.33910144596573));
#44079=CARTESIAN_POINT('Ctrl Pts',(4.72500831061156,15.3139172101386,2.39974235832286));
#44080=CARTESIAN_POINT('Ctrl Pts',(5.0368280494556,15.233183625842,2.46604569521785));
#44081=CARTESIAN_POINT('Ctrl Pts',(5.34437472290267,15.1449662897124,2.53746220440449));
#44082=CARTESIAN_POINT('Ctrl Pts',(5.62846729561695,15.0634765772789,2.60343235326581));
#44083=CARTESIAN_POINT('Ctrl Pts',(5.90891387849274,14.9756005513054,2.67376622484032));
#44084=CARTESIAN_POINT('Ctrl Pts',(6.18548847091395,14.8814648070078,2.74805806744846));
#44085=CARTESIAN_POINT('Ctrl Pts',(6.20699738299684,14.8741439702301,2.75383566508368));
#44086=CARTESIAN_POINT('Ctrl Pts',(6.22848287378777,14.8667852614923,2.75963721232427));
#44087=CARTESIAN_POINT('Ctrl Pts',(6.24994485533833,14.8593887340788,2.76546253801171));
#44088=CARTESIAN_POINT('Ctrl Pts',(7.10864015771174,15.2168666636805,-5.10578634035435));
#44089=CARTESIAN_POINT('Ctrl Pts',(7.1087319511891,15.2180649748934,-5.10211992456215));
#44090=CARTESIAN_POINT('Ctrl Pts',(7.11056295212648,15.2469376143842,-5.01406836458424));
#44091=CARTESIAN_POINT('Ctrl Pts',(7.0957532833273,15.3118408147158,-4.83046555613198));
#44092=CARTESIAN_POINT('Ctrl Pts',(7.0156532801071,15.4217311620991,-4.56064291735805));
#44093=CARTESIAN_POINT('Ctrl Pts',(6.86753478365422,15.544577900644,-4.30331374819862));
#44094=CARTESIAN_POINT('Ctrl Pts',(6.6575660839203,15.6691709072268,-4.08925365825966));
#44095=CARTESIAN_POINT('Ctrl Pts',(6.43827728684127,15.7687690204722,-3.96037917188944));
#44096=CARTESIAN_POINT('Ctrl Pts',(6.29372110804464,15.8227148621946,-3.91249915664003));
#44097=CARTESIAN_POINT('Ctrl Pts',(6.24006896070876,15.8413292732832,-3.89922637230209));
#44098=CARTESIAN_POINT('Ctrl Pts',(6.81411419638977,14.6698658120206,-4.91911214345852));
#44099=CARTESIAN_POINT('Ctrl Pts',(6.81419627724694,14.6709155403628,-4.91589643867816));
#44100=CARTESIAN_POINT('Ctrl Pts',(6.81583363952186,14.6962160679811,-4.83866110954873));
#44101=CARTESIAN_POINT('Ctrl Pts',(6.80258371972187,14.7534790973455,-4.67723688479289));
#44102=CARTESIAN_POINT('Ctrl Pts',(6.73069215177584,14.8512303729355,-4.43987215280684));
#44103=CARTESIAN_POINT('Ctrl Pts',(6.59792592232803,14.9609312319686,-4.21412828271034));
#44104=CARTESIAN_POINT('Ctrl Pts',(6.41046232976571,15.0721874407856,-4.02740669878977));
#44105=CARTESIAN_POINT('Ctrl Pts',(6.21582985009401,15.1607955045741,-3.91592435843964));
#44106=CARTESIAN_POINT('Ctrl Pts',(6.08830244040965,15.2085177762748,-3.87484710507141));
#44107=CARTESIAN_POINT('Ctrl Pts',(6.04108479571608,15.2249435030192,-3.86349736250906));
#44108=CARTESIAN_POINT('Ctrl Pts',(7.05418145170486,14.0948107036104,-4.73681539781006));
#44109=CARTESIAN_POINT('Ctrl Pts',(7.05428926420662,14.0961709987801,-4.73265407124799));
#44110=CARTESIAN_POINT('Ctrl Pts',(7.05643951699901,14.128938155199,-4.63273942242313));
#44111=CARTESIAN_POINT('Ctrl Pts',(7.03906591768119,14.2021863569183,-4.42547524588522));
#44112=CARTESIAN_POINT('Ctrl Pts',(6.94574281226092,14.3258056483014,-4.12160094983398));
#44113=CARTESIAN_POINT('Ctrl Pts',(6.77268165673607,14.4645602505892,-3.83060449371117));
#44114=CARTESIAN_POINT('Ctrl Pts',(6.52525480627982,14.6068210786327,-3.5862501007206));
#44115=CARTESIAN_POINT('Ctrl Pts',(6.26358456623248,14.7225229339098,-3.43716301885407));
#44116=CARTESIAN_POINT('Ctrl Pts',(6.08889668303178,14.7863755199405,-3.38117016334174));
#44117=CARTESIAN_POINT('Ctrl Pts',(6.0237377980366,14.8085815309694,-3.36561061007094));
#44118=CARTESIAN_POINT('Ctrl Pts',(7.66687013418301,13.8848570640408,-4.68358416887574));
#44119=CARTESIAN_POINT('Ctrl Pts',(7.66702167141007,13.8867765789514,-4.67772182071597));
#44120=CARTESIAN_POINT('Ctrl Pts',(7.67004350207725,13.9329883534776,-4.53700409028155));
#44121=CARTESIAN_POINT('Ctrl Pts',(7.64565945806534,14.0350125684346,-4.24694992517504));
#44122=CARTESIAN_POINT('Ctrl Pts',(7.51579920588202,14.2049730951923,-3.82267498432891));
#44123=CARTESIAN_POINT('Ctrl Pts',(7.27412333436781,14.3952858296309,-3.41381360895691));
#44124=CARTESIAN_POINT('Ctrl Pts',(6.92493243269211,14.5918721258049,-3.06591857353932));
#44125=CARTESIAN_POINT('Ctrl Pts',(6.54999799178159,14.7543797728273,-2.84972017330276));
#44126=CARTESIAN_POINT('Ctrl Pts',(6.29594778184491,14.8457775466123,-2.76720426236357));
#44127=CARTESIAN_POINT('Ctrl Pts',(6.20064104407826,14.8778126539731,-2.74415575802351));
#44128=CARTESIAN_POINT('',(6.26385988960052,15.8144313888753,-3.90573722891367));
#44129=CARTESIAN_POINT('',(6.24994527935227,14.8593853006947,-2.7654652932868));
#44130=CARTESIAN_POINT('Ctrl Pts',(6.26385592206845,15.8144315483309,-3.90575173238593));
#44131=CARTESIAN_POINT('Ctrl Pts',(6.25433095299875,15.7850306577855,-3.90346957258091));
#44132=CARTESIAN_POINT('Ctrl Pts',(6.24498623106511,15.7550023461302,-3.89974836247239));
#44133=CARTESIAN_POINT('Ctrl Pts',(6.23592367023207,15.7245194976627,-3.8944382562731));
#44134=CARTESIAN_POINT('Ctrl Pts',(6.22708767499122,15.6947987256923,-3.88926090364951));
#44135=CARTESIAN_POINT('Ctrl Pts',(6.21852020190849,15.6646461666652,-3.88257242852675));
#44136=CARTESIAN_POINT('Ctrl Pts',(6.21032175097156,15.6342621779096,-3.87426193331965));
#44137=CARTESIAN_POINT('Ctrl Pts',(6.20224971554734,15.60434669321,-3.86607958128502));
#44138=CARTESIAN_POINT('Ctrl Pts',(6.19453573488545,15.5742073104456,-3.8563242268315));
#44139=CARTESIAN_POINT('Ctrl Pts',(6.18727712052749,15.5440691681782,-3.84492712821924));
#44140=CARTESIAN_POINT('Ctrl Pts',(6.18014610180885,15.5144608096051,-3.83373037364125));
#44141=CARTESIAN_POINT('Ctrl Pts',(6.17345491813546,15.4848542830761,-3.82094865417076));
#44142=CARTESIAN_POINT('Ctrl Pts',(6.1672922922867,15.4554880016809,-3.8065606166512));
#44143=CARTESIAN_POINT('Ctrl Pts',(6.16649545488218,15.4516908944052,-3.80470022032753));
#44144=CARTESIAN_POINT('Ctrl Pts',(6.16570744531893,15.4478978303577,-3.80281303398504));
#44145=CARTESIAN_POINT('Ctrl Pts',(6.16492844635537,15.4441093467659,-3.80089907131186));
#44146=CARTESIAN_POINT('Ctrl Pts',(6.15899613680071,15.4152589137602,-3.78632367444429));
#44147=CARTESIAN_POINT('Ctrl Pts',(6.15358732682031,15.3866735129082,-3.77019140006747));
#44148=CARTESIAN_POINT('Ctrl Pts',(6.14877660702489,15.3585961452695,-3.75253620676512));
#44149=CARTESIAN_POINT('Ctrl Pts',(6.14402751803451,15.3308784807199,-3.73510719661675));
#44150=CARTESIAN_POINT('Ctrl Pts',(6.13986156567779,15.303656721696,-3.71619405950193));
#44151=CARTESIAN_POINT('Ctrl Pts',(6.13633724632498,15.2771655770841,-3.69587843831654));
#44152=CARTESIAN_POINT('Ctrl Pts',(6.13283362286278,15.2508299966468,-3.67568211672677));
#44153=CARTESIAN_POINT('Ctrl Pts',(6.12996433857516,15.2252172805214,-3.65409994594118));
#44154=CARTESIAN_POINT('Ctrl Pts',(6.12776996862142,15.2005469106632,-3.63125919646604));
#44155=CARTESIAN_POINT('Ctrl Pts',(6.12558304479817,15.175960254489,-3.60849595224508));
#44156=CARTESIAN_POINT('Ctrl Pts',(6.12406660150077,15.1523103055953,-3.58448308507558));
#44157=CARTESIAN_POINT('Ctrl Pts',(6.12324126585957,15.1297915883043,-3.55938867220841));
#44158=CARTESIAN_POINT('Ctrl Pts',(6.12241667337202,15.1072931474515,-3.5343168550026));
#44159=CARTESIAN_POINT('Ctrl Pts',(6.12228198917389,15.0859245249791,-3.50816605444565));
#44160=CARTESIAN_POINT('Ctrl Pts',(6.12283685496085,15.0658466643614,-3.48113814715521));
#44161=CARTESIAN_POINT('Ctrl Pts',(6.12339442435247,15.045670973604,-3.45397854535823));
#44162=CARTESIAN_POINT('Ctrl Pts',(6.12464823653243,15.0267991299266,-3.4259340178237));
#44163=CARTESIAN_POINT('Ctrl Pts',(6.12657673909308,15.0093526625765,-3.39723372259577));
#44164=CARTESIAN_POINT('Ctrl Pts',(6.12851270268902,14.9918386979301,-3.36842239100202));
#44165=CARTESIAN_POINT('Ctrl Pts',(6.13112843575211,14.9757613988018,-3.33895105166633));
#44166=CARTESIAN_POINT('Ctrl Pts',(6.13438231594651,14.9611962896866,-3.30906387764939));
#44167=CARTESIAN_POINT('Ctrl Pts',(6.13767358391751,14.9464638243649,-3.27883329363622));
#44168=CARTESIAN_POINT('Ctrl Pts',(6.14161752502853,14.9332785492476,-3.24817813040878));
#44169=CARTESIAN_POINT('Ctrl Pts',(6.14615364579537,14.9216678928345,-3.21735064817516));
#44170=CARTESIAN_POINT('Ctrl Pts',(6.14945760802415,14.9132110698768,-3.1948969168607));
#44171=CARTESIAN_POINT('Ctrl Pts',(6.1530753447366,14.905588505734,-3.17235178720936));
#44172=CARTESIAN_POINT('Ctrl Pts',(6.15697894263873,14.8987944830744,-3.14980875965272));
#44173=CARTESIAN_POINT('Ctrl Pts',(6.16243384140003,14.889300496573,-3.11830706911547));
#44174=CARTESIAN_POINT('Ctrl Pts',(6.16844711444727,14.8814260469965,-3.08681083225173));
#44175=CARTESIAN_POINT('Ctrl Pts',(6.17493398303811,14.8751150572397,-3.05555548377661));
#44176=CARTESIAN_POINT('Ctrl Pts',(6.18156924645999,14.8686596960893,-3.02358513204668));
#44177=CARTESIAN_POINT('Ctrl Pts',(6.18869966876894,14.8638396372848,-2.99186745460911));
#44178=CARTESIAN_POINT('Ctrl Pts',(6.19622900740018,14.8605521153216,-2.96062094277275));
#44179=CARTESIAN_POINT('Ctrl Pts',(6.20386986944998,14.8572158990831,-2.92891161235574));
#44180=CARTESIAN_POINT('Ctrl Pts',(6.21192119906387,14.855457238923,-2.89768789040987));
#44181=CARTESIAN_POINT('Ctrl Pts',(6.22028226351325,14.8551347288596,-2.8671362186537));
#44182=CARTESIAN_POINT('Ctrl Pts',(6.22884385259857,14.8548044839899,-2.83585182166933));
#44183=CARTESIAN_POINT('Ctrl Pts',(6.23772988449376,14.8559793294473,-2.80527231272382));
#44184=CARTESIAN_POINT('Ctrl Pts',(6.24683732091203,14.8584834957687,-2.77554952450875));
#44185=CARTESIAN_POINT('Ctrl Pts',(6.24787065150557,14.8587676187153,-2.77217717415927));
#44186=CARTESIAN_POINT('Ctrl Pts',(6.24890684053132,14.8590688368182,-2.76881580100156));
#44187=CARTESIAN_POINT('Ctrl Pts',(6.2499457442485,14.8593868813717,-2.76546558747461));
#44188=CARTESIAN_POINT('',(7.0000012282179,14.5427401407676,-3.16613547811813));
#44189=CARTESIAN_POINT('Ctrl Pts',(7.0000013293211,14.5427391135065,-3.16613474352585));
#44190=CARTESIAN_POINT('Ctrl Pts',(6.96887877241648,14.5590716998195,-3.1390116407485));
#44191=CARTESIAN_POINT('Ctrl Pts',(6.93707072944916,14.5752060957849,-3.11307622335859));
#44192=CARTESIAN_POINT('Ctrl Pts',(6.90460103412709,14.591151148044,-3.088301430666));
#44193=CARTESIAN_POINT('Ctrl Pts',(6.86312143260867,14.6115207390531,-3.05665196434374));
#44194=CARTESIAN_POINT('Ctrl Pts',(6.82056330189585,14.6315814111164,-3.02689528556155));
#44195=CARTESIAN_POINT('Ctrl Pts',(6.77697278425567,14.6513476542579,-2.99898817181636));
#44196=CARTESIAN_POINT('Ctrl Pts',(6.73506789076836,14.6703495463742,-2.9721602126101));
#44197=CARTESIAN_POINT('Ctrl Pts',(6.69220820290542,14.6890795109183,-2.9470414160688));
#44198=CARTESIAN_POINT('Ctrl Pts',(6.64840148543268,14.7075489660477,-2.92362425330318));
#44199=CARTESIAN_POINT('Ctrl Pts',(6.60341126352853,14.7265174013165,-2.89957444062669));
#44200=CARTESIAN_POINT('Ctrl Pts',(6.55744029917543,14.7452050310169,-2.87732107588973));
#44201=CARTESIAN_POINT('Ctrl Pts',(6.5104615664701,14.7636233772941,-2.85688934585874));
#44202=CARTESIAN_POINT('Ctrl Pts',(6.49869810258092,14.7682353269754,-2.85177324534746));
#44203=CARTESIAN_POINT('Ctrl Pts',(6.48687132345982,14.7728303613784,-2.84677157921616));
#44204=CARTESIAN_POINT('Ctrl Pts',(6.47498056272099,14.7774085926902,-2.84188519222801));
#44205=CARTESIAN_POINT('Ctrl Pts',(6.4282311540271,14.7954082490111,-2.8226739989862));
#44206=CARTESIAN_POINT('Ctrl Pts',(6.38049398200554,14.813148909004,-2.80524099676269));
#44207=CARTESIAN_POINT('Ctrl Pts',(6.3317535215381,14.8306268924779,-2.78964392165212));
#44208=CARTESIAN_POINT('Ctrl Pts',(6.30479293140245,14.8402947689059,-2.78101646213824));
#44209=CARTESIAN_POINT('Ctrl Pts',(6.27752507085231,14.8498821142477,-2.77295157353707));
#44210=CARTESIAN_POINT('Ctrl Pts',(6.2499457442485,14.8593868813717,-2.76546558747461));
#44211=CARTESIAN_POINT('',(6.99999966028507,14.7967844361631,-4.92965368890365));
#44212=CARTESIAN_POINT('Ctrl Pts',(6.999999755579,14.7967844361721,-4.92965368889445));
#44213=CARTESIAN_POINT('Ctrl Pts',(7.,14.7621585949968,-4.84258385989647));
#44214=CARTESIAN_POINT('Ctrl Pts',(7.,14.7150197661553,-4.71637142925406));
#44215=CARTESIAN_POINT('Ctrl Pts',(7.,14.6750808366962,-4.59674746789346));
#44216=CARTESIAN_POINT('Ctrl Pts',(7.,14.6500548613639,-4.51846226460458));
#44217=CARTESIAN_POINT('Ctrl Pts',(7.,14.6389243780002,-4.4820629208109));
#44218=CARTESIAN_POINT('Ctrl Pts',(7.,14.581446750461,-4.28361440547124));
#44219=CARTESIAN_POINT('Ctrl Pts',(7.,14.5473159321849,-4.12816776072898));
#44220=CARTESIAN_POINT('Ctrl Pts',(7.,14.4827629958402,-3.68737187183234));
#44221=CARTESIAN_POINT('Ctrl Pts',(7.,14.4884102191812,-3.41567190515103));
#44222=CARTESIAN_POINT('Ctrl Pts',(7.000002769616,14.5427399567595,-3.1661358977195));
#44223=CARTESIAN_POINT('Ctrl Pts',(6.99999922604844,14.7967844361462,-4.92965368893157));
#44224=CARTESIAN_POINT('Ctrl Pts',(6.99999541671933,14.8231421321045,-4.89367483326372));
#44225=CARTESIAN_POINT('Ctrl Pts',(6.99835381523207,14.8491523793382,-4.85878351348419));
#44226=CARTESIAN_POINT('Ctrl Pts',(6.99534856867432,14.8746944704123,-4.8250788148475));
#44227=CARTESIAN_POINT('Ctrl Pts',(6.99234332211657,14.9002365614864,-4.79137411621081));
#44228=CARTESIAN_POINT('Ctrl Pts',(6.98797378878021,14.925310754538,-4.7588558475189));
#44229=CARTESIAN_POINT('Ctrl Pts',(6.98248006879472,14.9498211812681,-4.7275907396323));
#44230=CARTESIAN_POINT('Ctrl Pts',(6.976606994457,14.976024110907,-4.69416670213496));
#44231=CARTESIAN_POINT('Ctrl Pts',(6.9694499941618,15.0015828464119,-4.66217424815261));
#44232=CARTESIAN_POINT('Ctrl Pts',(6.96130496289058,15.0264106533835,-4.63163259429477));
#44233=CARTESIAN_POINT('Ctrl Pts',(6.9554290502691,15.0443216987178,-4.60959951874131));
#44234=CARTESIAN_POINT('Ctrl Pts',(6.94903793998474,15.0618528940018,-4.58832087951969));
#44235=CARTESIAN_POINT('Ctrl Pts',(6.94223029564817,15.0789789048149,-4.56779549245821));
#44236=CARTESIAN_POINT('Ctrl Pts',(6.93362365721347,15.1006306503541,-4.54184604850422));
#44237=CARTESIAN_POINT('Ctrl Pts',(6.92435173065237,15.1216344536675,-4.51710097836386));
#44238=CARTESIAN_POINT('Ctrl Pts',(6.91459418292409,15.1419510597054,-4.49354340341939));
#44239=CARTESIAN_POINT('Ctrl Pts',(6.90513607886576,15.1616441813144,-4.47070877310125));
#44240=CARTESIAN_POINT('Ctrl Pts',(6.89522187554574,15.1806918465391,-4.4489893294753));
#44241=CARTESIAN_POINT('Ctrl Pts',(6.88501113930072,15.1990697417936,-4.4283466567952));
#44242=CARTESIAN_POINT('Ctrl Pts',(6.87463876704942,15.2177385592226,-4.40737721050242));
#44243=CARTESIAN_POINT('Ctrl Pts',(6.86396024783996,15.2357163136807,-4.38751882899225));
#44244=CARTESIAN_POINT('Ctrl Pts',(6.85312289688962,15.2529860247726,-4.36872385762821));
#44245=CARTESIAN_POINT('Ctrl Pts',(6.84770422141445,15.2616208803185,-4.35932637194619));
#44246=CARTESIAN_POINT('Ctrl Pts',(6.84224554360595,15.2700788492252,-4.3501946305685));
#44247=CARTESIAN_POINT('Ctrl Pts',(6.83676361365584,15.2783584971853,-4.34132207858134));
#44248=CARTESIAN_POINT('Ctrl Pts',(6.83402264868079,15.2824983211654,-4.33688580258776));
#44249=CARTESIAN_POINT('Ctrl Pts',(6.83127586167704,15.2865935652506,-4.33251432988044));
#44250=CARTESIAN_POINT('Ctrl Pts',(6.82852524201499,15.2906440957321,-4.32820679498813));
#44251=CARTESIAN_POINT('Ctrl Pts',(6.82714993218396,15.2926693609729,-4.32605302754197));
#44252=CARTESIAN_POINT('Ctrl Pts',(6.82577366363104,15.2946834478336,-4.32391524490488));
#44253=CARTESIAN_POINT('Ctrl Pts',(6.82439668045042,15.2966863408067,-4.32179333891745));
#44254=CARTESIAN_POINT('Ctrl Pts',(6.82331719383298,15.2982565097028,-4.32012986971237));
#44255=CARTESIAN_POINT('Ctrl Pts',(6.82270592634273,15.2991431246873,-4.31919185825726));
#44256=CARTESIAN_POINT('Ctrl Pts',(6.82146136389623,15.3009376438913,-4.31729558962247));
#44257=CARTESIAN_POINT('Ctrl Pts',(6.82111837395589,15.3014321968456,-4.31677299546278));
#44258=CARTESIAN_POINT('Ctrl Pts',(6.82072709014987,15.3019956963768,-4.31617776831686));
#44259=CARTESIAN_POINT('Ctrl Pts',(6.82026382823309,15.3026614233177,-4.31547514285564));
#44260=CARTESIAN_POINT('Ctrl Pts',(6.80986979753839,15.3175980844322,-4.299710603734));
#44261=CARTESIAN_POINT('Ctrl Pts',(6.79910042356942,15.3324180675512,-4.28431332886537));
#44262=CARTESIAN_POINT('Ctrl Pts',(6.7879747741671,15.3471115832376,-4.26929879229707));
#44263=CARTESIAN_POINT('Ctrl Pts',(6.75802588351796,15.3866647345756,-4.22888149191573));
#44264=CARTESIAN_POINT('Ctrl Pts',(6.72549937877864,15.4252998951193,-4.19123691311024));
#44265=CARTESIAN_POINT('Ctrl Pts',(6.69085593483662,15.4628507430421,-4.15655350064428));
#44266=CARTESIAN_POINT('Ctrl Pts',(6.66371764858482,15.4922665731088,-4.12938390465188));
#44267=CARTESIAN_POINT('Ctrl Pts',(6.63527895641645,15.5210174947097,-4.10403176413252));
#44268=CARTESIAN_POINT('Ctrl Pts',(6.60574127218368,15.5490325526764,-4.08058907629517));
#44269=CARTESIAN_POINT('Ctrl Pts',(6.5661772022082,15.5865571502388,-4.04918891185774));
#44270=CARTESIAN_POINT('Ctrl Pts',(6.52464362824406,15.6227609185537,-4.02121368452812));
#44271=CARTESIAN_POINT('Ctrl Pts',(6.4816917575019,15.6575041340452,-3.99674950069069));
#44272=CARTESIAN_POINT('Ctrl Pts',(6.44899681926555,15.6839506488303,-3.97812737863299));
#44273=CARTESIAN_POINT('Ctrl Pts',(6.41547886115081,15.7095513225518,-3.96154001705578));
#44274=CARTESIAN_POINT('Ctrl Pts',(6.3813625699735,15.7342522525339,-3.94702624011616));
#44275=CARTESIAN_POINT('Ctrl Pts',(6.34283814181153,15.7621447686835,-3.93063715039466));
#44276=CARTESIAN_POINT('Ctrl Pts',(6.30355144644052,15.7888900196305,-3.9168915304846));
#44277=CARTESIAN_POINT('Ctrl Pts',(6.26385592214248,15.8144315483213,-3.90575173240628));
#44278=CARTESIAN_POINT('Ctrl Pts',(6.99933866928551,24.8246602696117,-9.44604681568958));
#44279=CARTESIAN_POINT('Ctrl Pts',(6.99933866928551,24.8024268424346,-9.41529029807104));
#44280=CARTESIAN_POINT('Ctrl Pts',(6.99933866928551,24.437915482051,-8.91650381238244));
#44281=CARTESIAN_POINT('Ctrl Pts',(6.99933866928551,23.6489684573882,-8.00787919366893));
#44282=CARTESIAN_POINT('Ctrl Pts',(6.99933866928551,22.3090668585326,-6.88744611042101));
#44283=CARTESIAN_POINT('Ctrl Pts',(6.99933866928551,20.8065036616784,-5.99155840174367));
#44284=CARTESIAN_POINT('Ctrl Pts',(6.99933866928551,19.1801233637513,-5.34582278160595));
#44285=CARTESIAN_POINT('Ctrl Pts',(6.99933866928551,17.4735480440587,-4.9657269191405));
#44286=CARTESIAN_POINT('Ctrl Pts',(6.99933866928551,15.9617905172726,-4.87591919715298));
#44287=CARTESIAN_POINT('Ctrl Pts',(6.99933866928551,15.0338141052518,-4.93831842762876));
#44288=CARTESIAN_POINT('Ctrl Pts',(6.99933866928551,14.6872933691311,-4.97834430560805));
#44289=CARTESIAN_POINT('Ctrl Pts',(7.01704756088437,25.2191171808218,-9.16096594701436));
#44290=CARTESIAN_POINT('Ctrl Pts',(7.01704756088437,25.1958971300538,-9.12884521302238));
#44291=CARTESIAN_POINT('Ctrl Pts',(7.01704756088437,24.8152197698719,-8.60794384395676));
#44292=CARTESIAN_POINT('Ctrl Pts',(7.01704756088437,23.9915399790218,-7.65928052454269));
#44293=CARTESIAN_POINT('Ctrl Pts',(7.01704756088437,22.5916670864478,-6.48867427937066));
#44294=CARTESIAN_POINT('Ctrl Pts',(7.01704756088437,21.0226414798408,-5.55321290417034));
#44295=CARTESIAN_POINT('Ctrl Pts',(7.01704756088437,19.3239067410746,-4.87868204962013));
#44296=CARTESIAN_POINT('Ctrl Pts',(7.01704756088437,17.5412802279475,-4.48169569382117));
#44297=CARTESIAN_POINT('Ctrl Pts',(7.01704756088437,15.9624851498432,-4.38790582987388));
#44298=CARTESIAN_POINT('Ctrl Pts',(7.01704756088437,14.9934038436444,-4.45305428473393));
#44299=CARTESIAN_POINT('Ctrl Pts',(7.01704756088437,14.631431596948,-4.49486766018024));
#44300=CARTESIAN_POINT('Ctrl Pts',(6.7271181571115,25.5371657468869,-8.93110671799271));
#44301=CARTESIAN_POINT('Ctrl Pts',(6.7271181571115,25.5131501866105,-8.89788602339486));
#44302=CARTESIAN_POINT('Ctrl Pts',(6.7271181571115,25.1194382644694,-8.35915353832037));
#44303=CARTESIAN_POINT('Ctrl Pts',(6.7271181571115,24.2677536239904,-7.37820722173647));
#44304=CARTESIAN_POINT('Ctrl Pts',(6.7271181571115,22.8195261876635,-6.16714661578266));
#44305=CARTESIAN_POINT('Ctrl Pts',(6.7271181571115,21.1969122840431,-5.19977719806063));
#44306=CARTESIAN_POINT('Ctrl Pts',(6.7271181571115,19.439838534086,-4.50202889503887));
#44307=CARTESIAN_POINT('Ctrl Pts',(6.7271181571115,17.5958923372774,-4.09142382187531));
#44308=CARTESIAN_POINT('Ctrl Pts',(6.7271181571115,15.9630452284889,-3.99442317746496));
#44309=CARTESIAN_POINT('Ctrl Pts',(6.7271181571115,14.9608212588499,-4.06178831772415));
#44310=CARTESIAN_POINT('Ctrl Pts',(6.7271181571115,14.58639053915,-4.10504294312414));
#44311=CARTESIAN_POINT('Ctrl Pts',(6.25441317383083,25.6379536448148,-8.85826555162297));
#44312=CARTESIAN_POINT('Ctrl Pts',(6.25441317383083,25.6136859918143,-8.82469628537189));
#44313=CARTESIAN_POINT('Ctrl Pts',(6.25441317383083,25.215843486348,-8.28031321452375));
#44314=CARTESIAN_POINT('Ctrl Pts',(6.25441317383083,24.3552842580777,-7.28913658795351));
#44315=CARTESIAN_POINT('Ctrl Pts',(6.25441317383083,22.8917335241628,-6.06525621036345));
#44316=CARTESIAN_POINT('Ctrl Pts',(6.25441317383083,21.2521377744256,-5.08777530378322));
#44317=CARTESIAN_POINT('Ctrl Pts',(6.25441317383083,19.4765767022983,-4.3826695148969));
#44318=CARTESIAN_POINT('Ctrl Pts',(6.25441317383083,17.613198624076,-3.96774874268206));
#44319=CARTESIAN_POINT('Ctrl Pts',(6.25441317383083,15.9632227144307,-3.86973061903417));
#44320=CARTESIAN_POINT('Ctrl Pts',(6.25441317383083,14.9504960111262,-3.9377982151014));
#44321=CARTESIAN_POINT('Ctrl Pts',(6.25441317383083,14.5721172676417,-3.98150956493884));
#44322=CARTESIAN_POINT('',(7.00000000000001,24.7867247203242,-9.3325097692458));
#44323=CARTESIAN_POINT('Ctrl Pts',(7.00000000000006,24.7867247293774,-9.3325097625576));
#44324=CARTESIAN_POINT('Ctrl Pts',(7.00000000000006,24.6891826006153,-9.20047562542689));
#44325=CARTESIAN_POINT('Ctrl Pts',(7.00000000006077,24.5890285233467,-9.07101755125835));
#44326=CARTESIAN_POINT('Ctrl Pts',(6.99999999867348,24.4862283239914,-8.94403306164543));
#44327=CARTESIAN_POINT('Ctrl Pts',(6.99999999728335,24.383217075292,-8.81678787221477));
#44328=CARTESIAN_POINT('Ctrl Pts',(6.99999999423,24.2775485179081,-8.69202609764112));
#44329=CARTESIAN_POINT('Ctrl Pts',(6.99999999314812,24.1691470391679,-8.56967687293844));
#44330=CARTESIAN_POINT('Ctrl Pts',(6.99999999207005,24.061127052739,-8.44775822620449));
#44331=CARTESIAN_POINT('Ctrl Pts',(6.99999999472224,23.9503930271291,-8.32823485899167));
#44332=CARTESIAN_POINT('Ctrl Pts',(6.99999999803546,23.8368340148605,-8.21107349781402));
#44333=CARTESIAN_POINT('Ctrl Pts',(6.99999999907238,23.8012943438622,-8.17440642800796));
#44334=CARTESIAN_POINT('Ctrl Pts',(7.00000000000006,23.7654777308091,-8.13797099699824));
#44335=CARTESIAN_POINT('Ctrl Pts',(7.00000000000006,23.7293801188067,-8.10176700848402));
#44336=CARTESIAN_POINT('Ctrl Pts',(7.00000000000006,23.7004840050172,-8.07278574036939));
#44337=CARTESIAN_POINT('Ctrl Pts',(6.99999999938406,23.6714110890632,-8.04394890796352));
#44338=CARTESIAN_POINT('Ctrl Pts',(6.99999999847213,23.6421641709267,-8.01526109819976));
#44339=CARTESIAN_POINT('Ctrl Pts',(6.99999999416131,23.5039094271266,-7.87964934688404));
#44340=CARTESIAN_POINT('Ctrl Pts',(6.99999998574684,23.3617631569525,-7.7473702398002));
#44341=CARTESIAN_POINT('Ctrl Pts',(6.99999998500535,23.2160542950788,-7.61879342316149));
#44342=CARTESIAN_POINT('Ctrl Pts',(6.99999998426229,23.0700374208795,-7.48994480943497));
#44343=CARTESIAN_POINT('Ctrl Pts',(6.99999998984228,22.9204431673932,-7.36481445645444));
#44344=CARTESIAN_POINT('Ctrl Pts',(6.99999999473004,22.7676413783106,-7.24373929126517));
#44345=CARTESIAN_POINT('Ctrl Pts',(6.99999999759813,22.6779788884569,-7.17269365210419));
#44346=CARTESIAN_POINT('Ctrl Pts',(7.00000000000006,22.5872126828296,-7.10304362038108));
#44347=CARTESIAN_POINT('Ctrl Pts',(7.00000000000006,22.4954230550847,-7.03485104061892));
#44348=CARTESIAN_POINT('Ctrl Pts',(7.00000000000006,22.4321186731275,-6.98782079088417));
#44349=CARTESIAN_POINT('Ctrl Pts',(6.99999999890231,22.3683242960228,-6.94148920194487));
#44350=CARTESIAN_POINT('Ctrl Pts',(6.99999999758229,22.3040492398655,-6.8958618643371));
#44351=CARTESIAN_POINT('Ctrl Pts',(6.999999993463,22.1034710548579,-6.75347616899528));
#44352=CARTESIAN_POINT('Ctrl Pts',(6.99999998925884,21.8982142893946,-6.61794558861433));
#44353=CARTESIAN_POINT('Ctrl Pts',(6.99999999152164,21.6886162028712,-6.48945459759717));
#44354=CARTESIAN_POINT('Ctrl Pts',(6.99999999354313,21.5013710088194,-6.37466671500727));
#44355=CARTESIAN_POINT('Ctrl Pts',(7.00000000000006,21.3106603646735,-6.26549734902331));
#44356=CARTESIAN_POINT('Ctrl Pts',(7.00000000000006,21.1167056938803,-6.16210761400783));
#44357=CARTESIAN_POINT('Ctrl Pts',(7.00000000000006,21.0129457950191,-6.10679722419038));
#44358=CARTESIAN_POINT('Ctrl Pts',(6.99999999803041,20.9082630701657,-6.05312590552218));
#44359=CARTESIAN_POINT('Ctrl Pts',(6.99999999636328,20.8027238129362,-6.00113898290814));
#44360=CARTESIAN_POINT('Ctrl Pts',(6.99999999271544,20.5717938321343,-5.88738662803697));
#44361=CARTESIAN_POINT('Ctrl Pts',(6.99999999204991,20.336761374834,-5.78170184011558));
#44362=CARTESIAN_POINT('Ctrl Pts',(6.99999999506639,20.0983777911221,-5.68438505777925));
#44363=CARTESIAN_POINT('Ctrl Pts',(6.99999999705719,19.941050119291,-5.62015822404906));
#44364=CARTESIAN_POINT('Ctrl Pts',(7.00000000000006,19.7822633753942,-5.55957532148921));
#44365=CARTESIAN_POINT('Ctrl Pts',(7.00000000000006,19.6222386409051,-5.50271137547352));
#44366=CARTESIAN_POINT('Ctrl Pts',(7.00000000000006,19.4747046058049,-5.45028593365543));
#44367=CARTESIAN_POINT('Ctrl Pts',(6.99999999722485,19.3261163406549,-5.40103443266753));
#44368=CARTESIAN_POINT('Ctrl Pts',(6.99999999446477,19.1765618936819,-5.35498993307642));
#44369=CARTESIAN_POINT('Ctrl Pts',(6.99999999008284,18.9391276998962,-5.28188920715386));
#44370=CARTESIAN_POINT('Ctrl Pts',(6.99999998784252,18.6992583715269,-5.21686912534717));
#44371=CARTESIAN_POINT('Ctrl Pts',(6.99999999262696,18.4573223660356,-5.16006800350815));
#44372=CARTESIAN_POINT('Ctrl Pts',(6.99999999531402,18.3214448864838,-5.12816703343334));
#44373=CARTESIAN_POINT('Ctrl Pts',(7.00000000000006,18.1849153998852,-5.09885944130387));
#44374=CARTESIAN_POINT('Ctrl Pts',(7.00000000000006,18.0477988670123,-5.07217694339681));
#44375=CARTESIAN_POINT('Ctrl Pts',(7.00000000000006,17.856393082599,-5.03492990735382));
#44376=CARTESIAN_POINT('Ctrl Pts',(6.99999999014824,17.663843855679,-5.00273444785686));
#44377=CARTESIAN_POINT('Ctrl Pts',(6.99999998525267,17.4706055436115,-4.97570140054251));
#44378=CARTESIAN_POINT('Ctrl Pts',(6.99999998003395,17.2646116456454,-4.94688391227839));
#44379=CARTESIAN_POINT('Ctrl Pts',(6.99999998145014,17.0578350753082,-4.92393341763544));
#44380=CARTESIAN_POINT('Ctrl Pts',(6.99999998835951,16.8508303905368,-4.9068403931192));
#44381=CARTESIAN_POINT('Ctrl Pts',(6.9999999930865,16.7092102037236,-4.89514637118021));
#44382=CARTESIAN_POINT('Ctrl Pts',(7.00000000000006,16.5674833559243,-4.8861928324609));
#44383=CARTESIAN_POINT('Ctrl Pts',(7.00000000000006,16.4258270758153,-4.8799626811172));
#44384=CARTESIAN_POINT('Ctrl Pts',(7.00000000000006,16.2592199746816,-4.87263517361665));
#44385=CARTESIAN_POINT('Ctrl Pts',(6.99999999283356,16.0927257552284,-4.86914728796146));
#44386=CARTESIAN_POINT('Ctrl Pts',(6.99999999157262,15.9262294991414,-4.86944988962922));
#44387=CARTESIAN_POINT('Ctrl Pts',(6.99999999107899,15.8610504983776,-4.86956835039703));
#44388=CARTESIAN_POINT('Ctrl Pts',(6.99999999110876,15.7958711098815,-4.87026827073992));
#44389=CARTESIAN_POINT('Ctrl Pts',(6.99999999149986,15.7306842246115,-4.87154886618109));
#44390=CARTESIAN_POINT('Ctrl Pts',(6.99999999249462,15.5648782176151,-4.8748061228486));
#44391=CARTESIAN_POINT('Ctrl Pts',(6.99999999551031,15.3990235687409,-4.88181651104614));
#44392=CARTESIAN_POINT('Ctrl Pts',(6.9999999971705,15.2330389193309,-4.89260183864214));
#44393=CARTESIAN_POINT('Ctrl Pts',(6.99999999862381,15.0877376989017,-4.90204320125004));
#44394=CARTESIAN_POINT('Ctrl Pts',(6.99999999923222,14.9423366411189,-4.91437806045602));
#44395=CARTESIAN_POINT('Ctrl Pts',(6.99999999922778,14.7967844361711,-4.92965368888493));
#44396=CARTESIAN_POINT('',(6.27159471697229,25.5608579993301,-8.76071062884084));
#44397=CARTESIAN_POINT('Origin',(5.999999877385,24.7867246592848,-9.33250977407517));
#44398=CARTESIAN_POINT('Ctrl Pts',(6.27159470456983,25.5608577604478,-8.76071047658685));
#44399=CARTESIAN_POINT('Ctrl Pts',(6.27193966904855,25.4228903724782,-8.57412213201062));
#44400=CARTESIAN_POINT('Ctrl Pts',(6.2722578257596,25.2809101921298,-8.39339826441702));
#44401=CARTESIAN_POINT('Ctrl Pts',(6.2725491704145,25.1354917489078,-8.21861674188987));
#44402=CARTESIAN_POINT('Ctrl Pts',(6.27284515835287,24.9877557102086,-8.04104965202243));
#44403=CARTESIAN_POINT('Ctrl Pts',(6.27311347279902,24.8364709296681,-7.86961577203008));
#44404=CARTESIAN_POINT('Ctrl Pts',(6.27335411019051,24.6822005300308,-7.70435939028142));
#44405=CARTESIAN_POINT('Ctrl Pts',(6.27354178826528,24.5618818571093,-7.57547252286843));
#44406=CARTESIAN_POINT('Ctrl Pts',(6.27371263106456,24.4397462990353,-7.4503425101875));
#44407=CARTESIAN_POINT('Ctrl Pts',(6.27386663725764,24.3160449568949,-7.32897538004301));
#44408=CARTESIAN_POINT('Ctrl Pts',(6.27406868762992,24.1537534169881,-7.16974623907808));
#44409=CARTESIAN_POINT('Ctrl Pts',(6.27424175803524,23.9887687648483,-7.01699414752484));
#44410=CARTESIAN_POINT('Ctrl Pts',(6.27438584622067,23.8216789740255,-6.87062073725345));
#44411=CARTESIAN_POINT('Ctrl Pts',(6.27447251943017,23.7211696338436,-6.78257289893794));
#44412=CARTESIAN_POINT('Ctrl Pts',(6.2745487058153,23.6198976557413,-6.69683263130532));
#44413=CARTESIAN_POINT('Ctrl Pts',(6.27461440502469,23.5179829393777,-6.61337445203782));
#44414=CARTESIAN_POINT('Ctrl Pts',(6.27472591407379,23.3450065334529,-6.47172370315872));
#44415=CARTESIAN_POINT('Ctrl Pts',(6.27480721254685,23.1701811200194,-6.33664821756605));
#44416=CARTESIAN_POINT('Ctrl Pts',(6.27485829938236,22.994054627927,-6.20800456804343));
#44417=CARTESIAN_POINT('Ctrl Pts',(6.27487121302793,22.9495336652978,-6.17548623962592));
#44418=CARTESIAN_POINT('Ctrl Pts',(6.27488219624781,22.9049293331402,-6.14337877177348));
#44419=CARTESIAN_POINT('Ctrl Pts',(6.27489124903292,22.8602500105278,-6.11167962116953));
#44420=CARTESIAN_POINT('Ctrl Pts',(6.27492812717343,22.6782407926702,-5.98254745732212));
#44421=CARTESIAN_POINT('Ctrl Pts',(6.27493296994929,22.4949911250344,-5.86019253913393));
#44422=CARTESIAN_POINT('Ctrl Pts',(6.27490577729413,22.3110440760799,-5.7443888087212));
#44423=CARTESIAN_POINT('Ctrl Pts',(6.2748825782446,22.1541121151202,-5.64559240723818));
#44424=CARTESIAN_POINT('Ctrl Pts',(6.27483606247482,21.9966716419835,-5.55156390696271));
#44425=CARTESIAN_POINT('Ctrl Pts',(6.27476623045072,21.839031356596,-5.46215383379084));
#44426=CARTESIAN_POINT('Ctrl Pts',(6.27472435246144,21.7444950995172,-5.40853496573288));
#44427=CARTESIAN_POINT('Ctrl Pts',(6.27467408920095,21.6498864864855,-5.35657689080563));
#44428=CARTESIAN_POINT('Ctrl Pts',(6.27461544218262,21.5552677453534,-5.30624603899135));
#44429=CARTESIAN_POINT('Ctrl Pts',(6.27458611867346,21.5079583747874,-5.28108061308421));
#44430=CARTESIAN_POINT('Ctrl Pts',(6.27455469659286,21.4606464679072,-5.25632200111359));
#44431=CARTESIAN_POINT('Ctrl Pts',(6.27452117938581,21.4133394548803,-5.23196589211826));
#44432=CARTESIAN_POINT('Ctrl Pts',(6.27450442078228,21.3896859483668,-5.2197878376206));
#44433=CARTESIAN_POINT('Ctrl Pts',(6.27448713821938,21.36603366502,-5.20771040941384));
#44434=CARTESIAN_POINT('Ctrl Pts',(6.27446933169767,21.3423835227119,-5.19573306711981));
#44435=CARTESIAN_POINT('Ctrl Pts',(6.27445391976996,21.3219138156338,-5.18536641963247));
#44436=CARTESIAN_POINT('Ctrl Pts',(6.27443873000482,21.3022159979294,-5.17546006316596));
#44437=CARTESIAN_POINT('Ctrl Pts',(6.27442216616428,21.2812906867064,-5.16501291099337));
#44438=CARTESIAN_POINT('Ctrl Pts',(6.27441959259438,21.2780394629953,-5.16338970795018));
#44439=CARTESIAN_POINT('Ctrl Pts',(6.27441698585337,21.2747585611155,-5.16175354057576));
#44440=CARTESIAN_POINT('Ctrl Pts',(6.27441433995409,21.2714404304069,-5.16010075684977));
#44441=CARTESIAN_POINT('Ctrl Pts',(6.27440279826912,21.2569664027134,-5.15289114411244));
#44442=CARTESIAN_POINT('Ctrl Pts',(6.27439106676851,21.2424686881078,-5.14570647248201));
#44443=CARTESIAN_POINT('Ctrl Pts',(6.27437914545323,21.227947341887,-5.13854692036595));
#44444=CARTESIAN_POINT('Ctrl Pts',(6.27420011328074,21.0098683714745,-5.03102605209729));
#44445=CARTESIAN_POINT('Ctrl Pts',(6.27397827112255,20.786455912684,-4.9291684238133));
#44446=CARTESIAN_POINT('Ctrl Pts',(6.27371362325632,20.5579728151575,-4.8335167029945));
#44447=CARTESIAN_POINT('Ctrl Pts',(6.27345239736455,20.3324440710385,-4.73910178695646));
#44448=CARTESIAN_POINT('Ctrl Pts',(6.27314946557812,20.1019749203303,-4.65073332519588));
#44449=CARTESIAN_POINT('Ctrl Pts',(6.27280483384928,19.8668624230668,-4.5689577857274));
#44450=CARTESIAN_POINT('Ctrl Pts',(6.27260798841794,19.7325717670888,-4.52224954619952));
#44451=CARTESIAN_POINT('Ctrl Pts',(6.27239753873934,19.5967670728685,-4.47769264806433));
#44452=CARTESIAN_POINT('Ctrl Pts',(6.27217348622092,19.4595104125741,-4.43539260233193));
#44453=CARTESIAN_POINT('Ctrl Pts',(6.271770138192,19.2124156520413,-4.35924242026889));
#44454=CARTESIAN_POINT('Ctrl Pts',(6.27132270510958,18.9606118600149,-4.2904051057413));
#44455=CARTESIAN_POINT('Ctrl Pts',(6.27083119717597,18.7045322088994,-4.22947050840681));
#44456=CARTESIAN_POINT('Ctrl Pts',(6.27036732795719,18.4628525541364,-4.17196241519141));
#44457=CARTESIAN_POINT('Ctrl Pts',(6.26986420294061,18.2173647726219,-4.12149341735369));
#44458=CARTESIAN_POINT('Ctrl Pts',(6.26932183185764,17.9684809537258,-4.07857938281827));
#44459=CARTESIAN_POINT('Ctrl Pts',(6.26905885439899,17.847805578052,-4.0577718137999));
#44460=CARTESIAN_POINT('Ctrl Pts',(6.26878665041033,17.7263325216401,-4.03874067682215));
#44461=CARTESIAN_POINT('Ctrl Pts',(6.26850522122231,17.6041128540969,-4.02154646483739));
#44462=CARTESIAN_POINT('Ctrl Pts',(6.26791730047585,17.3487893793731,-3.98562682901008));
#44463=CARTESIAN_POINT('Ctrl Pts',(6.26728911939944,17.090204297127,-3.95772366469815));
#44464=CARTESIAN_POINT('Ctrl Pts',(6.26662069240957,16.8288425750066,-3.93824718398145));
#44465=CARTESIAN_POINT('Ctrl Pts',(6.26595957850088,16.5703403416834,-3.91898379023849));
#44466=CARTESIAN_POINT('Ctrl Pts',(6.26525909447508,16.3091218449081,-3.90796371321164));
#44467=CARTESIAN_POINT('Ctrl Pts',(6.26451925764027,16.0457069788102,-3.90559012140761));
#44468=CARTESIAN_POINT('Ctrl Pts',(6.26430324653886,15.968797405406,-3.9048971007904));
#44469=CARTESIAN_POINT('Ctrl Pts',(6.26408388074319,15.8917009326381,-3.90494120951631));
#44470=CARTESIAN_POINT('Ctrl Pts',(6.26386116074403,15.8144313374826,-3.90573258244604));
#44471=CARTESIAN_POINT('Ctrl Pts',(6.99999999998952,24.1259274560584,-10.9278021978677));
#44472=CARTESIAN_POINT('Ctrl Pts',(6.99999999998952,24.1259309537943,-10.9277942569083));
#44473=CARTESIAN_POINT('Ctrl Pts',(6.99999999998952,24.2426228977018,-10.6628666420065));
#44474=CARTESIAN_POINT('Ctrl Pts',(6.99999999998952,24.4687752087452,-10.1334777511239));
#44475=CARTESIAN_POINT('Ctrl Pts',(6.99999999998952,24.6831190611286,-9.59922082304237));
#44476=CARTESIAN_POINT('Ctrl Pts',(6.99999999998952,24.7867214499965,-9.33250574074716));
#44477=CARTESIAN_POINT('Ctrl Pts',(7.00000270565606,24.6668575635222,-11.166064437851));
#44478=CARTESIAN_POINT('Ctrl Pts',(7.00000270565606,24.6668611144483,-11.1660563761331));
#44479=CARTESIAN_POINT('Ctrl Pts',(7.00000270565606,24.7853275969941,-10.8970999979764));
#44480=CARTESIAN_POINT('Ctrl Pts',(7.00000270565606,25.0149154772904,-10.3596688248218));
#44481=CARTESIAN_POINT('Ctrl Pts',(7.00000270565606,25.23251564032,-9.81729560136332));
#44482=CARTESIAN_POINT('Ctrl Pts',(7.00000270565606,25.3376935135728,-9.54652457482602));
#44483=CARTESIAN_POINT('Ctrl Pts',(6.57967197777265,25.0472372157118,-11.3336093881521));
#44484=CARTESIAN_POINT('Ctrl Pts',(6.57967197777265,25.047240804041,-11.3336012415174));
#44485=CARTESIAN_POINT('Ctrl Pts',(6.57967197777265,25.1669551342874,-11.0618118549112));
#44486=CARTESIAN_POINT('Ctrl Pts',(6.57967197777265,25.3989588916405,-10.5187253845367));
#44487=CARTESIAN_POINT('Ctrl Pts',(6.57967197777265,25.6188488778711,-9.97064481817619));
#44488=CARTESIAN_POINT('Ctrl Pts',(6.57967197777265,25.7251346247603,-9.69702166963551));
#44489=CARTESIAN_POINT('Ctrl Pts',(5.98852435812717,25.0410285650909,-11.3308746780969));
#44490=CARTESIAN_POINT('Ctrl Pts',(5.98852435812717,25.0410321528096,-11.3308665328482));
#44491=CARTESIAN_POINT('Ctrl Pts',(5.98852435812717,25.1607261153798,-11.0591233873078));
#44492=CARTESIAN_POINT('Ctrl Pts',(5.98852435812717,25.3926904401917,-10.5161292240906));
#44493=CARTESIAN_POINT('Ctrl Pts',(5.98852435812717,25.6125430513673,-9.9681418143915));
#44494=CARTESIAN_POINT('Ctrl Pts',(5.98852435812717,25.7188107152653,-9.69456521889174));
#44495=CARTESIAN_POINT('',(6.99999999994009,24.1259366383783,-10.9277762175416));
#44496=CARTESIAN_POINT('',(5.98852583812712,25.0410393194101,-11.3308502415527));
#44497=CARTESIAN_POINT('Origin',(5.999999999061,24.1259421376201,-10.9277802195584));
#44498=CARTESIAN_POINT('',(5.98852581355276,25.7188095579036,-9.6945673613816));
#44499=CARTESIAN_POINT('Origin',(5.98846856209437,-11.4751154482372,4.75314848444354));
#44500=CARTESIAN_POINT('Origin',(6.,24.7867247762541,-9.33250981979305));
#44501=CARTESIAN_POINT('Origin',(6.99999997873566,-11.466399908179,4.74964876109848));
#44502=CARTESIAN_POINT('Origin',(5.999999877385,24.7867246592848,-9.33250977407517));
#44503=CARTESIAN_POINT('Origin',(5.99999764422236,24.7867226423257,-9.33250908125501));
#44504=CARTESIAN_POINT('Ctrl Pts',(-6.09415743644224,25.695632913879,-9.75660475861075));
#44505=CARTESIAN_POINT('Ctrl Pts',(-6.05606588786886,25.7001327750303,-9.74375762209026));
#44506=CARTESIAN_POINT('Ctrl Pts',(-5.71207088669795,25.7404909054814,-9.62883157111345));
#44507=CARTESIAN_POINT('Ctrl Pts',(-5.02599367437364,25.8158751281454,-9.41914130782388));
#44508=CARTESIAN_POINT('Ctrl Pts',(-3.98564775819421,25.9128460400099,-9.15673704498941));
#44509=CARTESIAN_POINT('Ctrl Pts',(-2.8121347216154,25.9981089845718,-8.93130224440336));
#44510=CARTESIAN_POINT('Ctrl Pts',(-1.52041606181854,26.0598653167182,-8.77189810582769));
#44511=CARTESIAN_POINT('Ctrl Pts',(-0.189383689790614,26.0855142661398,
-8.70820319779262));
#44512=CARTESIAN_POINT('Ctrl Pts',(1.08604876871579,26.0712746006462,-8.7432758938014));
#44513=CARTESIAN_POINT('Ctrl Pts',(2.24115591648484,26.0279846764949,-8.85386421781817));
#44514=CARTESIAN_POINT('Ctrl Pts',(3.27282426553086,25.9662680371191,-9.01516003136025));
#44515=CARTESIAN_POINT('Ctrl Pts',(4.19977149261964,25.8933059518543,-9.20943322947018));
#44516=CARTESIAN_POINT('Ctrl Pts',(5.05677934805222,25.8119848641214,-9.43016103454035));
#44517=CARTESIAN_POINT('Ctrl Pts',(5.68020727836871,25.7440091973074,-9.61906168812787));
#44518=CARTESIAN_POINT('Ctrl Pts',(6.02208888516753,25.7041476094482,-9.73229018312302));
#44519=CARTESIAN_POINT('Ctrl Pts',(6.09402271407761,25.6956511769004,-9.75655051851992));
#44520=CARTESIAN_POINT('Ctrl Pts',(-6.21832045083748,25.8362000143657,-9.42811502690297));
#44521=CARTESIAN_POINT('Ctrl Pts',(-6.17949927537105,25.8406700578237,-9.41497942109277));
#44522=CARTESIAN_POINT('Ctrl Pts',(-5.82891139971618,25.8807305423587,-9.29745967126212));
#44523=CARTESIAN_POINT('Ctrl Pts',(-5.12960176788881,25.9550321339388,-9.08280837935187));
#44524=CARTESIAN_POINT('Ctrl Pts',(-4.06864373258683,26.0495433651156,-8.81368358460258));
#44525=CARTESIAN_POINT('Ctrl Pts',(-2.87116826723681,26.1317341015626,-8.58205154196733));
#44526=CARTESIAN_POINT('Ctrl Pts',(-1.55239219357112,26.1905177359622,-8.41796833305674));
#44527=CARTESIAN_POINT('Ctrl Pts',(-0.193327228883218,26.2144487869133,
-8.3522524468396));
#44528=CARTESIAN_POINT('Ctrl Pts',(1.10884029567984,26.2012168234477,-8.38845432061946));
#44529=CARTESIAN_POINT('Ctrl Pts',(2.28827733632914,26.1602360331969,-8.50236336342224));
#44530=CARTESIAN_POINT('Ctrl Pts',(3.3413059591683,26.1011009640294,-8.66824165694523));
#44531=CARTESIAN_POINT('Ctrl Pts',(4.28702500024961,26.0305268774016,-8.86774343384528));
#44532=CARTESIAN_POINT('Ctrl Pts',(5.16096421564057,25.9511658454649,-9.09407335380042));
#44533=CARTESIAN_POINT('Ctrl Pts',(5.79643509995807,25.8842029429415,-9.28746110921518));
#44534=CARTESIAN_POINT('Ctrl Pts',(6.1448711748215,25.8446561037839,-9.40325337755369));
#44535=CARTESIAN_POINT('Ctrl Pts',(6.2181830809188,25.8362155442671,-9.42805839472418));
#44536=CARTESIAN_POINT('Ctrl Pts',(-6.32908148192128,25.7777118953252,-9.07101154408849));
#44537=CARTESIAN_POINT('Ctrl Pts',(-6.28955536356086,25.7821394193768,-9.05766430847315));
#44538=CARTESIAN_POINT('Ctrl Pts',(-5.93260993993696,25.8217847285637,-8.9382614968994));
#44539=CARTESIAN_POINT('Ctrl Pts',(-5.22075534859015,25.8947242064414,-8.7203448381954));
#44540=CARTESIAN_POINT('Ctrl Pts',(-4.14076534441269,25.9863193807797,-8.44741153118032));
#44541=CARTESIAN_POINT('Ctrl Pts',(-2.92177802350408,26.0649719169936,-8.21276332196714));
#44542=CARTESIAN_POINT('Ctrl Pts',(-1.57939308857452,26.1204058329895,-8.04679377181448));
#44543=CARTESIAN_POINT('Ctrl Pts',(-0.196603179973188,26.1424404003294,
-7.98050294385007));
#44544=CARTESIAN_POINT('Ctrl Pts',(1.12799353753121,26.1303178461725,-8.01700054852035));
#44545=CARTESIAN_POINT('Ctrl Pts',(2.32845047101542,26.0919206097672,-8.13213550603907));
#44546=CARTESIAN_POINT('Ctrl Pts',(3.40035685415087,26.0357243654915,-8.30005701232116));
#44547=CARTESIAN_POINT('Ctrl Pts',(4.36306687249998,25.9679208707662,-8.50222900241744));
#44548=CARTESIAN_POINT('Ctrl Pts',(5.25267862910245,25.890893519041,-8.7317891343879));
#44549=CARTESIAN_POINT('Ctrl Pts',(5.89955400277617,25.8251984299464,-8.92811103922429));
#44550=CARTESIAN_POINT('Ctrl Pts',(6.25429750722298,25.7860851791503,-9.04574939358607));
#44551=CARTESIAN_POINT('Ctrl Pts',(6.32894084680062,25.7777244435615,-9.07095421174326));
#44552=CARTESIAN_POINT('Ctrl Pts',(-6.39488356528743,25.5363210844092,-8.78685862136819));
#44553=CARTESIAN_POINT('Ctrl Pts',(-6.35487788319777,25.5407054572845,-8.77343701804182));
#44554=CARTESIAN_POINT('Ctrl Pts',(-5.99362024485588,25.5799359332653,-8.65339948326985));
#44555=CARTESIAN_POINT('Ctrl Pts',(-5.27348028270466,25.6516207929835,-8.43484668262279));
#44556=CARTESIAN_POINT('Ctrl Pts',(-4.18145907208881,25.7406723417186,-8.1621080481356));
#44557=CARTESIAN_POINT('Ctrl Pts',(-2.949539041277,25.8163265374911,-7.92849107071696));
#44558=CARTESIAN_POINT('Ctrl Pts',(-1.59372167497793,25.8689861431572,-7.7639717081696));
#44559=CARTESIAN_POINT('Ctrl Pts',(-0.198277517924796,25.8894849573124,
-7.69871919628221));
#44560=CARTESIAN_POINT('Ctrl Pts',(1.13804826103157,25.8782580228526,-7.73459284944474));
#44561=CARTESIAN_POINT('Ctrl Pts',(2.35022440052859,25.8419841352125,-7.84850481328988));
#44562=CARTESIAN_POINT('Ctrl Pts',(3.43314706915597,25.7882484371947,-8.01534244688904));
#44563=CARTESIAN_POINT('Ctrl Pts',(4.40622700504305,25.7228105380502,-8.21685996825643));
#44564=CARTESIAN_POINT('Ctrl Pts',(5.3057887963983,25.6478272285819,-8.44635317423841));
#44565=CARTESIAN_POINT('Ctrl Pts',(5.96018277702732,25.5832948021266,-8.64321733490893));
#44566=CARTESIAN_POINT('Ctrl Pts',(6.31919090099219,25.5446108704843,-8.76145689273703));
#44567=CARTESIAN_POINT('Ctrl Pts',(6.39473997509298,25.5363312504338,-8.78680248425463));
#44568=CARTESIAN_POINT('',(-5.98852245733802,25.7188096065183,-9.69456809190458));
#44569=CARTESIAN_POINT('Ctrl Pts',(-5.98852261949295,25.7188097472649,-9.69456765143577));
#44570=CARTESIAN_POINT('Ctrl Pts',(-5.87207793470072,25.7323476875087,-9.65602540128857));
#44571=CARTESIAN_POINT('Ctrl Pts',(-5.74893720685401,25.7463673807796,-9.61639632705623));
#44572=CARTESIAN_POINT('Ctrl Pts',(-5.61909817687992,25.7607399809517,-9.57606535652041));
#44573=CARTESIAN_POINT('Ctrl Pts',(-5.51159709928282,25.7726398696575,-9.54267306458784));
#44574=CARTESIAN_POINT('Ctrl Pts',(-5.39950421817578,25.7847813042434,-9.50880032892854));
#44575=CARTESIAN_POINT('Ctrl Pts',(-5.28282127149538,25.7970760121566,-9.47468790985182));
#44576=CARTESIAN_POINT('Ctrl Pts',(-5.21054205117668,25.8046919657068,-9.45355698091836));
#44577=CARTESIAN_POINT('Ctrl Pts',(-5.13650113477044,25.8123654142613,-9.4323371784525));
#44578=CARTESIAN_POINT('Ctrl Pts',(-5.06069864646586,25.8200697754248,-9.41109682695929));
#44579=CARTESIAN_POINT('Ctrl Pts',(-5.00141638195798,25.8260950654459,-9.39448554989407));
#44580=CARTESIAN_POINT('Ctrl Pts',(-4.94105673135458,25.8321392021902,-9.37786175899752));
#44581=CARTESIAN_POINT('Ctrl Pts',(-4.8796195626138,25.838189572322,-9.36125999719662));
#44582=CARTESIAN_POINT('Ctrl Pts',(-4.8096220277546,25.8450829725697,-9.34234502399392));
#44583=CARTESIAN_POINT('Ctrl Pts',(-4.73822586607673,25.8519843749472,-9.32345890387002));
#44584=CARTESIAN_POINT('Ctrl Pts',(-4.6654310767679,25.8588734261793,-9.30465633951433));
#44585=CARTESIAN_POINT('Ctrl Pts',(-4.62903368211348,25.8623179517954,-9.29525505733649));
#44586=CARTESIAN_POINT('Ctrl Pts',(-4.5922866305945,25.8657593845531,-9.28587466213729));
#44587=CARTESIAN_POINT('Ctrl Pts',(-4.55518992227452,25.8691950184334,-9.27652232790471));
#44588=CARTESIAN_POINT('Ctrl Pts',(-4.53664156811452,25.8709128353735,-9.27184616078842));
#44589=CARTESIAN_POINT('Ctrl Pts',(-4.5180057997557,25.8726292022635,-9.267177008788));
#44590=CARTESIAN_POINT('Ctrl Pts',(-4.49928261721151,25.8743437757585,-9.2625157760302));
#44591=CARTESIAN_POINT('Ctrl Pts',(-4.48992102593942,25.875201062506,-9.26018515965129));
#44592=CARTESIAN_POINT('Ctrl Pts',(-4.48053758112102,25.8760579008829,-9.25785652307483));
#44593=CARTESIAN_POINT('Ctrl Pts',(-4.47113228275811,25.8769142474015,-9.25552998043822));
#44594=CARTESIAN_POINT('Ctrl Pts',(-4.4617269843952,25.8777705939201,-9.2532034378016));
#44595=CARTESIAN_POINT('Ctrl Pts',(-4.45105740216065,25.8787389127704,-9.25057364239245));
#44596=CARTESIAN_POINT('Ctrl Pts',(-4.44285082703765,25.8794817676788,-9.24855674879096));
#44597=CARTESIAN_POINT('Ctrl Pts',(-4.30874234741994,25.8916211974477,-9.21559750204138));
#44598=CARTESIAN_POINT('Ctrl Pts',(-4.17030708094963,25.9036878750233,-9.1829900567557));
#44599=CARTESIAN_POINT('Ctrl Pts',(-4.02753713403268,25.9155537376321,-9.15105856413114));
#44600=CARTESIAN_POINT('Ctrl Pts',(-3.89073584476344,25.9269235345553,-9.12046200334463));
#44601=CARTESIAN_POINT('Ctrl Pts',(-3.74995452272013,25.9381087315707,-9.09048623610026));
#44602=CARTESIAN_POINT('Ctrl Pts',(-3.60520088627223,25.9489924261705,-9.06143417695892));
#44603=CARTESIAN_POINT('Ctrl Pts',(-3.45728944004113,25.9601135492601,-9.03174834530014));
#44604=CARTESIAN_POINT('Ctrl Pts',(-3.30522643331322,25.9709195633236,-9.00302795442544));
#44605=CARTESIAN_POINT('Ctrl Pts',(-3.14901186622847,25.9812763843197,-8.97561339885051));
#44606=CARTESIAN_POINT('Ctrl Pts',(-3.07090458268609,25.9864547948178,-8.96190612106305));
#44607=CARTESIAN_POINT('Ctrl Pts',(-2.99175940894427,25.9915207744709,-8.9485255226544));
#44608=CARTESIAN_POINT('Ctrl Pts',(-2.91157634414655,25.9964568067801,-8.93551526360204));
#44609=CARTESIAN_POINT('Ctrl Pts',(-2.89518327496918,25.9974659565215,-8.932855374295));
#44610=CARTESIAN_POINT('Ctrl Pts',(-2.87874682707864,25.9984696751547,-8.93021096065387));
#44611=CARTESIAN_POINT('Ctrl Pts',(-2.86226699500748,25.9994678077459,-8.92758240669926));
#44612=CARTESIAN_POINT('Ctrl Pts',(-2.83844310394662,26.000910747335,-8.92378246609356));
#44613=CARTESIAN_POINT('Ctrl Pts',(-2.81452854512119,26.0023420130239,-8.92001566975204));
#44614=CARTESIAN_POINT('Ctrl Pts',(-2.79052332849145,26.0037611565803,-8.91628315123654));
#44615=CARTESIAN_POINT('Ctrl Pts',(-2.77021808947114,26.0049615643735,-8.91312593412936));
#44616=CARTESIAN_POINT('Ctrl Pts',(-2.74984798224947,26.0061532976401,-8.90999324600946));
#44617=CARTESIAN_POINT('Ctrl Pts',(-2.72941300683531,26.0073360817096,-8.90688578004086));
#44618=CARTESIAN_POINT('Ctrl Pts',(-2.71919551912823,26.0079274737443,-8.90533204705655));
#44619=CARTESIAN_POINT('Ctrl Pts',(-2.70896181437299,26.008516628468,-8.90378461960582));
#44620=CARTESIAN_POINT('Ctrl Pts',(-2.69871189257079,26.0091035113992,-8.90224358452302));
#44621=CARTESIAN_POINT('Ctrl Pts',(-2.68846197076859,26.0096903943305,-8.90070254944022));
#44622=CARTESIAN_POINT('Ctrl Pts',(-2.67679403336959,26.0103543913698,-8.89895957144287));
#44623=CARTESIAN_POINT('Ctrl Pts',(-2.66791347602445,26.0108573102655,-8.89763974325157));
#44624=CARTESIAN_POINT('Ctrl Pts',(-2.48215217967096,26.0213772430126,-8.87003190443557));
#44625=CARTESIAN_POINT('Ctrl Pts',(-2.29149550040864,26.031141594686,-8.84454323782441));
#44626=CARTESIAN_POINT('Ctrl Pts',(-2.09593759637921,26.0399567757891,-8.82164664478182));
#44627=CARTESIAN_POINT('Ctrl Pts',(-1.99233080418927,26.0446270684126,-8.80951600465763));
#44628=CARTESIAN_POINT('Ctrl Pts',(-1.8873486414055,26.0490305925451,-8.79811362071221));
#44629=CARTESIAN_POINT('Ctrl Pts',(-1.78099278798611,26.0531361167612,-8.78751463948269));
#44630=CARTESIAN_POINT('Ctrl Pts',(-1.70012356651363,26.0562578118669,-8.77945554980521));
#44631=CARTESIAN_POINT('Ctrl Pts',(-1.61846022886176,26.0592076248522,-8.77185973311662));
#44632=CARTESIAN_POINT('Ctrl Pts',(-1.5360013136412,26.0619722371313,-8.76475833345694));
#44633=CARTESIAN_POINT('Ctrl Pts',(-1.46189047434314,26.0644569622309,-8.75837587393073));
#44634=CARTESIAN_POINT('Ctrl Pts',(-1.38713697991105,26.0667920820591,-8.75239281551445));
#44635=CARTESIAN_POINT('Ctrl Pts',(-1.3117420899921,26.0689671301156,-8.74683140022213));
#44636=CARTESIAN_POINT('Ctrl Pts',(-1.23210084237991,26.0712646802682,-8.7409567573538));
#44637=CARTESIAN_POINT('Ctrl Pts',(-1.15174319397122,26.0733836147045,-8.73555262591372));
#44638=CARTESIAN_POINT('Ctrl Pts',(-1.07066914321278,26.0753115011317,-8.73064468619408));
#44639=CARTESIAN_POINT('Ctrl Pts',(-1.03013211783356,26.0762754443453,-8.72819071633426));
#44640=CARTESIAN_POINT('Ctrl Pts',(-0.989415991865598,26.077191621347,-8.72586079302465));
#44641=CARTESIAN_POINT('Ctrl Pts',(-0.948520765211829,26.0780584628039,
-8.72365808622068));
#44642=CARTESIAN_POINT('Ctrl Pts',(-0.928073151884945,26.0784918835323,
-8.72255673281869));
#44643=CARTESIAN_POINT('Ctrl Pts',(-0.907580763387053,26.0789129700991,
-8.72148718345254));
#44644=CARTESIAN_POINT('Ctrl Pts',(-0.887043599715693,26.0793215255028,
-8.72044983132777));
#44645=CARTESIAN_POINT('Ctrl Pts',(-0.876775017880014,26.0795258032047,
-8.71993115526538));
#44646=CARTESIAN_POINT('Ctrl Pts',(-0.866495242251005,26.0797269480983,
-8.71942052850753));
#44647=CARTESIAN_POINT('Ctrl Pts',(-0.856204272829031,26.0799249355149,
-8.718917999984));
#44648=CARTESIAN_POINT('Ctrl Pts',(-0.845913303407058,26.0801229229315,
-8.71841547146047));
#44649=CARTESIAN_POINT('Ctrl Pts',(-0.833923452093846,26.0803491142949,
-8.71784146531518));
#44650=CARTESIAN_POINT('Ctrl Pts',(-0.825297783184885,26.0805094006148,
-8.71743475796202));
#44651=CARTESIAN_POINT('Ctrl Pts',(-0.603448600533726,26.084631908612,-8.70697438731385));
#44652=CARTESIAN_POINT('Ctrl Pts',(-0.379486899971072,26.0871467845146,
-8.70066381320836));
#44653=CARTESIAN_POINT('Ctrl Pts',(-0.153407990999127,26.0879157525049,
-8.6987153874091));
#44654=CARTESIAN_POINT('Ctrl Pts',(-0.0982029332275835,26.0881035228835,
-8.69823961123299));
#44655=CARTESIAN_POINT('Ctrl Pts',(-0.0428716692110073,26.0881870787357,
-8.69802412669697));
#44656=CARTESIAN_POINT('Ctrl Pts',(0.0125852468759724,26.0881662678656,
-8.69807058298918));
#44657=CARTESIAN_POINT('Ctrl Pts',(0.153868871692206,26.088113249498,-8.69818893636729));
#44658=CARTESIAN_POINT('Ctrl Pts',(0.295970722828568,26.0873812607907,-8.70001209002015));
#44659=CARTESIAN_POINT('Ctrl Pts',(0.438890814456262,26.0859637557959,-8.70357996189666));
#44660=CARTESIAN_POINT('Ctrl Pts',(0.510350860270108,26.0852550032984,-8.70536389783492));
#44661=CARTESIAN_POINT('Ctrl Pts',(0.582015465730846,26.0843748755081,-8.70758401484754));
#44662=CARTESIAN_POINT('Ctrl Pts',(0.653884630802583,26.0833230375972,-8.71024397464699));
#44663=CARTESIAN_POINT('Ctrl Pts',(0.689819213338452,26.0827971186417,-8.71157395454672));
#44664=CARTESIAN_POINT('Ctrl Pts',(0.725804935763038,26.0822282726436,-8.71301389529905));
#44665=CARTESIAN_POINT('Ctrl Pts',(0.761841798001913,26.0816164748928,-8.71456421474941));
#44666=CARTESIAN_POINT('Ctrl Pts',(0.77986022912135,26.0813105760174,-8.71533937447459));
#44667=CARTESIAN_POINT('Ctrl Pts',(0.797891445193713,26.0809939392436,-8.71614212888663));
#44668=CARTESIAN_POINT('Ctrl Pts',(0.815935446207505,26.080666563389,-8.71697252537766));
#44669=CARTESIAN_POINT('Ctrl Pts',(0.833979447221296,26.0803391875343,-8.71780292186869));
#44670=CARTESIAN_POINT('Ctrl Pts',(0.853658583946665,26.0799697510364,-8.71874048460496));
#44671=CARTESIAN_POINT('Ctrl Pts',(0.870105804060285,26.0796522180939,-8.71954668702734));
#44672=CARTESIAN_POINT('Ctrl Pts',(0.954941294048503,26.0780143691095,-8.72370511483821));
#44673=CARTESIAN_POINT('Ctrl Pts',(1.03915646093526,26.0761553385722,-8.72843526314769));
#44674=CARTESIAN_POINT('Ctrl Pts',(1.12274548012097,26.0740873004632,-8.73371107518766));
#44675=CARTESIAN_POINT('Ctrl Pts',(1.34023153458158,26.068706576378,-8.74743794452801));
#44676=CARTESIAN_POINT('Ctrl Pts',(1.5534774917799,26.0619126838085,-8.76485554934346));
#44677=CARTESIAN_POINT('Ctrl Pts',(1.76248314120672,26.0539184363475,-8.78549176678133));
#44678=CARTESIAN_POINT('Ctrl Pts',(1.93916409665569,26.0471605746181,-8.80293639865504));
#44679=CARTESIAN_POINT('Ctrl Pts',(2.11281537719476,26.039544475079,-8.82268188960559));
#44680=CARTESIAN_POINT('Ctrl Pts',(2.28344819734372,26.0311859009393,-8.84446642487241));
#44681=CARTESIAN_POINT('Ctrl Pts',(2.31468206953677,26.0296558867476,-8.84845402461854));
#44682=CARTESIAN_POINT('Ctrl Pts',(2.34581483023983,26.0281009648234,-8.85251000041726));
#44683=CARTESIAN_POINT('Ctrl Pts',(2.37684657615407,26.0265218157015,-8.85663275222822));
#44684=CARTESIAN_POINT('Ctrl Pts',(2.47767146807603,26.0213910202901,-8.87002793814233));
#44685=CARTESIAN_POINT('Ctrl Pts',(2.57829977349914,26.0159614000799,-8.88424000732834));
#44686=CARTESIAN_POINT('Ctrl Pts',(2.67796170055171,26.0102878204125,-8.89913258066258));
#44687=CARTESIAN_POINT('Ctrl Pts',(2.7797715277508,26.0044919645363,-8.91434611668933));
#44688=CARTESIAN_POINT('Ctrl Pts',(2.88057272493239,25.9984415859338,-8.93026972198904));
#44689=CARTESIAN_POINT('Ctrl Pts',(2.97955492182406,25.9922130910505,-8.94670742513009));
#44690=CARTESIAN_POINT('Ctrl Pts',(3.01344853266624,25.9900803218422,-8.95233604452729));
#44691=CARTESIAN_POINT('Ctrl Pts',(3.04712895851175,25.9879268149008,-8.95802452155688));
#44692=CARTESIAN_POINT('Ctrl Pts',(3.08056397548561,25.9857560785503,-8.96376371145562));
#44693=CARTESIAN_POINT('Ctrl Pts',(3.15906127951969,25.980659716511,-8.97723793624046));
#44694=CARTESIAN_POINT('Ctrl Pts',(3.23641909108672,25.9754553795562,-8.99102598292456));
#44695=CARTESIAN_POINT('Ctrl Pts',(3.31263593449704,25.970160509038,-9.00508309829586));
#44696=CARTESIAN_POINT('Ctrl Pts',(3.4564951477893,25.9601664463986,-9.03161588905429));
#44697=CARTESIAN_POINT('Ctrl Pts',(3.59628912015428,25.9498505824851,-9.0591058921734));
#44698=CARTESIAN_POINT('Ctrl Pts',(3.73202210285664,25.9393266493449,-9.08726369510383));
#44699=CARTESIAN_POINT('Ctrl Pts',(3.83584437087129,25.9312768843925,-9.10880162129055));
#44700=CARTESIAN_POINT('Ctrl Pts',(3.93728959599926,25.9231052112615,-9.13073051857037));
#44701=CARTESIAN_POINT('Ctrl Pts',(4.03635777759006,25.9148586837289,-9.15292779425468));
#44702=CARTESIAN_POINT('Ctrl Pts',(4.06112482298776,25.9127970518458,-9.15847711317576));
#44703=CARTESIAN_POINT('Ctrl Pts',(4.08675526254168,25.9106474134483,-9.16426728241562));
#44704=CARTESIAN_POINT('Ctrl Pts',(4.11470923701844,25.9082794988606,-9.17065119655818));
#44705=CARTESIAN_POINT('Ctrl Pts',(4.14266321149521,25.9059115842728,-9.17703511070074));
#44706=CARTESIAN_POINT('Ctrl Pts',(4.17043865126593,25.9035366069139,-9.18344354837801));
#44707=CARTESIAN_POINT('Ctrl Pts',(4.1980355563503,25.9011555857014,-9.18987381165783));
#44708=CARTESIAN_POINT('Ctrl Pts',(4.20574811720379,25.9004901570623,-9.19167088986997));
#44709=CARTESIAN_POINT('Ctrl Pts',(4.21344673427636,25.899824256114,-9.19346967337576));
#44710=CARTESIAN_POINT('Ctrl Pts',(4.221131407003,25.8991579044704,-9.1952701047956));
#44711=CARTESIAN_POINT('Ctrl Pts',(4.26844096715695,25.8950556083431,-9.20635419667437));
#44712=CARTESIAN_POINT('Ctrl Pts',(4.31522201712048,25.8909362468103,-9.21750071746783));
#44713=CARTESIAN_POINT('Ctrl Pts',(4.36147457089465,25.886805009107,-9.22869641509208));
#44714=CARTESIAN_POINT('Ctrl Pts',(4.51942902568656,25.8726966551718,-9.26693020263357));
#44715=CARTESIAN_POINT('Ctrl Pts',(4.67122070891271,25.858452365169,-9.30573242780717));
#44716=CARTESIAN_POINT('Ctrl Pts',(4.81684736679282,25.8442592310686,-9.34461209392482));
#44717=CARTESIAN_POINT('Ctrl Pts',(4.86949798770537,25.8391277713897,-9.3586688510582));
#44718=CARTESIAN_POINT('Ctrl Pts',(4.92134287243755,25.8340027593491,-9.37273615127393));
#44719=CARTESIAN_POINT('Ctrl Pts',(4.97238230340753,25.8288922459384,-9.38679219881856));
#44720=CARTESIAN_POINT('Ctrl Pts',(5.00462682864208,25.8256636425723,-9.39567220729706));
#44721=CARTESIAN_POINT('Ctrl Pts',(5.03654983724056,25.8224411457875,-9.40454687349655));
#44722=CARTESIAN_POINT('Ctrl Pts',(5.06815129371359,25.8192264788938,-9.41341144578933));
#44723=CARTESIAN_POINT('Ctrl Pts',(5.21039120874781,25.804757084225,-9.45331137922485));
#44724=CARTESIAN_POINT('Ctrl Pts',(5.34611635893376,25.7904487595192,-9.49300344357613));
#44725=CARTESIAN_POINT('Ctrl Pts',(5.4753262897967,25.7764523083133,-9.53208482760559));
#44726=CARTESIAN_POINT('Ctrl Pts',(5.60705266934046,25.7621832669828,-9.57192734738235));
#44727=CARTESIAN_POINT('Ctrl Pts',(5.73200777546778,25.748238173852,-9.61113514909158));
#44728=CARTESIAN_POINT('Ctrl Pts',(5.85019315497047,25.7347467326449,-9.64932598153051));
#44729=CARTESIAN_POINT('Ctrl Pts',(5.86232961570843,25.7333612960774,-9.65324779944399));
#44730=CARTESIAN_POINT('Ctrl Pts',(5.87439468823684,25.7319806192149,-9.65715893133953));
#44731=CARTESIAN_POINT('Ctrl Pts',(5.88638837412529,25.7306048262631,-9.66105898934999));
#44732=CARTESIAN_POINT('Ctrl Pts',(5.92102986644089,25.7266311086411,-9.67232356896765));
#44733=CARTESIAN_POINT('Ctrl Pts',(5.95507582044836,25.7226981505854,-9.68349575279175));
#44734=CARTESIAN_POINT('Ctrl Pts',(5.98852582161055,25.7188089328326,-9.6945670296992));
#44735=CARTESIAN_POINT('',(-6.27159361731479,25.5608563036375,-8.7607097378382));
#44736=CARTESIAN_POINT('Origin',(-5.999994980806,24.7867195890732,-9.33250914740904));
#44737=CARTESIAN_POINT('Ctrl Pts',(-6.2715938630759,25.5608571679648,-8.76070927462916));
#44738=CARTESIAN_POINT('Ctrl Pts',(-6.19708063874005,25.5689447885943,-8.73626652810999));
#44739=CARTESIAN_POINT('Ctrl Pts',(-6.1154389227446,25.577703521834,-8.70997409232932));
#44740=CARTESIAN_POINT('Ctrl Pts',(-6.02658468262738,25.58705204236,-8.68208171992035));
#44741=CARTESIAN_POINT('Ctrl Pts',(-5.93855991568889,25.5963132924639,-8.65444972872418));
#44742=CARTESIAN_POINT('Ctrl Pts',(-5.84345650339964,25.6061534772221,-8.62524745250685));
#44743=CARTESIAN_POINT('Ctrl Pts',(-5.74118376542963,25.6164754182921,-8.59476438981034));
#44744=CARTESIAN_POINT('Ctrl Pts',(-5.64049526630337,25.62663746905,-8.56475351992844));
#44745=CARTESIAN_POINT('Ctrl Pts',(-5.53285766337119,25.6372665650423,-8.53350118952672));
#44746=CARTESIAN_POINT('Ctrl Pts',(-5.41817807236923,25.6482508460994,-8.50132996802472));
#44747=CARTESIAN_POINT('Ctrl Pts',(-5.37925228009582,25.6519792500723,-8.49041006262196));
#44748=CARTESIAN_POINT('Ctrl Pts',(-5.33951511383068,25.6557484047636,-8.47938469052703));
#44749=CARTESIAN_POINT('Ctrl Pts',(-5.29896282541383,25.6595533901367,-8.46826772471874));
#44750=CARTESIAN_POINT('Ctrl Pts',(-5.21821391750951,25.6671299887815,-8.44613129584444));
#44751=CARTESIAN_POINT('Ctrl Pts',(-5.13423305843698,25.6748488767625,-8.42363096906741));
#44752=CARTESIAN_POINT('Ctrl Pts',(-5.04699090211752,25.6826701546544,-8.40088618232919));
#44753=CARTESIAN_POINT('Ctrl Pts',(-4.92201156784759,25.6938745785857,-8.36830298603306));
#44754=CARTESIAN_POINT('Ctrl Pts',(-4.79033921223311,25.7052898942599,-8.33521583496531));
#44755=CARTESIAN_POINT('Ctrl Pts',(-4.65188791926913,25.7167846607454,-8.30201798427405));
#44756=CARTESIAN_POINT('Ctrl Pts',(-4.51343662630514,25.728279427231,-8.26882013358279));
#44757=CARTESIAN_POINT('Ctrl Pts',(-4.36820619844028,25.7398537430577,-8.23551131174542));
#44758=CARTESIAN_POINT('Ctrl Pts',(-4.21611372757936,25.7513582417137,-8.20253791990527));
#44759=CARTESIAN_POINT('Ctrl Pts',(-4.07083064345331,25.7623476683212,-8.17104079165483));
#44760=CARTESIAN_POINT('Ctrl Pts',(-3.9192856518954,25.7732731892018,-8.13984997581947));
#44761=CARTESIAN_POINT('Ctrl Pts',(-3.76142356347455,25.7839926998624,-8.10940008417812));
#44762=CARTESIAN_POINT('Ctrl Pts',(-3.73054864169615,25.7860892390407,-8.10344464527578));
#44763=CARTESIAN_POINT('Ctrl Pts',(-3.69943211321045,25.7881778519993,-8.09751769687057));
#44764=CARTESIAN_POINT('Ctrl Pts',(-3.66807362047968,25.7902574078451,-8.09162270996234));
#44765=CARTESIAN_POINT('Ctrl Pts',(-3.58017497373741,25.7960864553775,-8.07509891284474));
#44766=CARTESIAN_POINT('Ctrl Pts',(-3.49037512731969,25.801844445983,-8.05882589668978));
#44767=CARTESIAN_POINT('Ctrl Pts',(-3.39866710747283,25.8075055236016,-8.04288325163617));
#44768=CARTESIAN_POINT('Ctrl Pts',(-3.3528130975494,25.8103360624109,-8.03491192910937));
#44769=CARTESIAN_POINT('Ctrl Pts',(-3.30648203531614,25.8131423275125,-8.0270232354011));
#44770=CARTESIAN_POINT('Ctrl Pts',(-3.25967321929016,25.8159209780059,-8.01922760696347));
#44771=CARTESIAN_POINT('Ctrl Pts',(-3.23626881127717,25.8173103032525,-8.01532979274466));
#44772=CARTESIAN_POINT('Ctrl Pts',(-3.21274496422015,25.8186927219388,-8.01145524714368));
#44773=CARTESIAN_POINT('Ctrl Pts',(-3.18910159440111,25.8200678037302,-8.00760529675011));
#44774=CARTESIAN_POINT('Ctrl Pts',(-3.17727990949158,25.8207553446259,-8.00568032155332));
#44775=CARTESIAN_POINT('Ctrl Pts',(-3.16542834385686,25.8214410511118,-8.00376149530634));
#44776=CARTESIAN_POINT('Ctrl Pts',(-3.15354688766476,25.8221248688895,-8.00184898569553));
#44777=CARTESIAN_POINT('Ctrl Pts',(-3.14166543147266,25.8228086866673,-7.99993647608473));
#44778=CARTESIAN_POINT('Ctrl Pts',(-3.12814004114031,25.8235825261987,-7.99777350825232));
#44779=CARTESIAN_POINT('Ctrl Pts',(-3.11781283770829,25.8241706012354,-7.9961305753528));
#44780=CARTESIAN_POINT('Ctrl Pts',(-3.07662183306222,25.8265161928305,-7.9895775857518));
#44781=CARTESIAN_POINT('Ctrl Pts',(-3.03569007114915,25.8288015738271,-7.98319701218292));
#44782=CARTESIAN_POINT('Ctrl Pts',(-2.99501928700432,25.8310283058371,-7.97698426024937));
#44783=CARTESIAN_POINT('Ctrl Pts',(-2.79740326302321,25.8418478151123,-7.94679700517417));
#44784=CARTESIAN_POINT('Ctrl Pts',(-2.60595262121096,25.8512834386195,-7.92057031856116));
#44785=CARTESIAN_POINT('Ctrl Pts',(-2.42086041250325,25.8595189574556,-7.89776639789247));
#44786=CARTESIAN_POINT('Ctrl Pts',(-2.23093226301904,25.8679696473226,-7.87436667467437));
#44787=CARTESIAN_POINT('Ctrl Pts',(-2.04769882625,25.8751567868988,-7.85457054853199));
#44788=CARTESIAN_POINT('Ctrl Pts',(-1.87131987055302,25.8812683271939,-7.83782008293064));
#44789=CARTESIAN_POINT('Ctrl Pts',(-1.78117209159126,25.8843919525803,-7.82925887298034));
#44790=CARTESIAN_POINT('Ctrl Pts',(-1.69281413701159,25.8872344267731,-7.8214936708302));
#44791=CARTESIAN_POINT('Ctrl Pts',(-1.60626302542332,25.8898197051797,-7.81445268897836));
#44792=CARTESIAN_POINT('Ctrl Pts',(-1.43906925792771,25.8948137766467,-7.80085138148414));
#44793=CARTESIAN_POINT('Ctrl Pts',(-1.27862000666068,25.898849112208,-7.78995007340322));
#44794=CARTESIAN_POINT('Ctrl Pts',(-1.12501483003616,25.9020960343758,-7.78123950576144));
#44795=CARTESIAN_POINT('Ctrl Pts',(-0.969937933891774,25.9053740659037,
-7.77244548056499));
#44796=CARTESIAN_POINT('Ctrl Pts',(-0.821836496383836,25.9078485158435,
-7.76588420567675));
#44797=CARTESIAN_POINT('Ctrl Pts',(-0.680780588800408,25.9096791291633,
-7.76107116675371));
#44798=CARTESIAN_POINT('Ctrl Pts',(-0.538386308398421,25.9115271117883,
-7.75621246054469));
#44799=CARTESIAN_POINT('Ctrl Pts',(-0.403171507814499,25.9127190007761,
-7.7531351475061));
#44800=CARTESIAN_POINT('Ctrl Pts',(-0.275181335910393,25.9134031565432,
-7.75138350697485));
#44801=CARTESIAN_POINT('Ctrl Pts',(-0.23621669182446,25.9136114372695,-7.75085024689049));
#44802=CARTESIAN_POINT('Ctrl Pts',(-0.197921464321872,25.9137725488857,
-7.75044015773775));
#44803=CARTESIAN_POINT('Ctrl Pts',(-0.160296520144296,25.9138903830244,
-7.7501411945641));
#44804=CARTESIAN_POINT('Ctrl Pts',(-0.153989050215633,25.9139101368154,
-7.75009107618468));
#44805=CARTESIAN_POINT('Ctrl Pts',(-0.147700417129246,25.9139286740498,
-7.75004408169272));
#44806=CARTESIAN_POINT('Ctrl Pts',(-0.14143062418855,25.9139460125369,-7.75000015385425));
#44807=CARTESIAN_POINT('Ctrl Pts',(-0.103047756247163,25.9140521565302,
-7.74973123326331));
#44808=CARTESIAN_POINT('Ctrl Pts',(-0.0662555242699623,25.9141126179072,
-7.74957970085559));
#44809=CARTESIAN_POINT('Ctrl Pts',(-0.0289807896640162,25.9141334369677,
-7.74952611301502));
#44810=CARTESIAN_POINT('Ctrl Pts',(-0.0185588351444299,25.9141392579428,
-7.74951112994289));
#44811=CARTESIAN_POINT('Ctrl Pts',(-0.00809915958435751,25.9141418859072,
-7.74950410082371));
#44812=CARTESIAN_POINT('Ctrl Pts',(0.00244355159823323,25.9141412341181,
-7.74950529176633));
#44813=CARTESIAN_POINT('Ctrl Pts',(0.127127936130238,25.9141335256725,-7.74951937656334));
#44814=CARTESIAN_POINT('Ctrl Pts',(0.258986331532658,25.9136690001181,-7.75068425796915));
#44815=CARTESIAN_POINT('Ctrl Pts',(0.397985519236686,25.9126040414671,-7.75344426483185));
#44816=CARTESIAN_POINT('Ctrl Pts',(0.535666549793538,25.9115491820323,-7.75617809799646));
#44817=CARTESIAN_POINT('Ctrl Pts',(0.680353904295599,25.9099052023948,-7.76047708456449));
#44818=CARTESIAN_POINT('Ctrl Pts',(0.831993346520431,25.9075172238835,-7.76681627110057));
#44819=CARTESIAN_POINT('Ctrl Pts',(0.942271910387529,25.9057805857312,-7.77142639348712));
#44820=CARTESIAN_POINT('Ctrl Pts',(1.0562268708477,25.9036501454434,-7.77711643635547));
#44821=CARTESIAN_POINT('Ctrl Pts',(1.17382842543845,25.9010612483794,-7.78408308820957));
#44822=CARTESIAN_POINT('Ctrl Pts',(1.33438952198139,25.8975266339528,-7.79359463986226));
#44823=CARTESIAN_POINT('Ctrl Pts',(1.50174979691909,25.8931378133859,-7.8054850775063));
#44824=CARTESIAN_POINT('Ctrl Pts',(1.6757982372772,25.8877230536469,-7.82026951813892));
#44825=CARTESIAN_POINT('Ctrl Pts',(1.84379921682465,25.8824964343315,-7.83454026083119));
#44826=CARTESIAN_POINT('Ctrl Pts',(2.0180318933548,25.876313850564,-7.85150771899027));
#44827=CARTESIAN_POINT('Ctrl Pts',(2.19835974785299,25.8690099500942,-7.87166082959492));
#44828=CARTESIAN_POINT('Ctrl Pts',(2.26108749901612,25.8664692596809,-7.87867116812908));
#44829=CARTESIAN_POINT('Ctrl Pts',(2.32455243103844,25.8637927933555,-7.88606718978257));
#44830=CARTESIAN_POINT('Ctrl Pts',(2.38874762164454,25.8609732905271,-7.8938701297493));
#44831=CARTESIAN_POINT('Ctrl Pts',(2.47500693013271,25.8571847144366,-7.90435496824498));
#44832=CARTESIAN_POINT('Ctrl Pts',(2.56258480514964,25.8531378845742,-7.91557450655615));
#44833=CARTESIAN_POINT('Ctrl Pts',(2.65146458196224,25.848815666565,-7.92757930467197));
#44834=CARTESIAN_POINT('Ctrl Pts',(2.72897715732554,25.8450462348541,-7.93804875961486));
#44835=CARTESIAN_POINT('Ctrl Pts',(2.80747992813828,25.8410673768089,-7.9491155169345));
#44836=CARTESIAN_POINT('Ctrl Pts',(2.88696060599889,25.8368674947661,-7.96081344720335));
#44837=CARTESIAN_POINT('Ctrl Pts',(2.9267009449292,25.8347675537447,-7.96666241233777));
#44838=CARTESIAN_POINT('Ctrl Pts',(2.96668575943288,25.8326123506864,-7.97266917549959));
#44839=CARTESIAN_POINT('Ctrl Pts',(3.00691339244417,25.8304004308499,-7.97883801236851));
#44840=CARTESIAN_POINT('Ctrl Pts',(3.02702720894982,25.8292944709316,-7.98192243080296));
#44841=CARTESIAN_POINT('Ctrl Pts',(3.0472017300277,25.8281743314571,-7.98504736795455));
#44842=CARTESIAN_POINT('Ctrl Pts',(3.06743674395561,25.8270398286313,-7.98821335935204));
#44843=CARTESIAN_POINT('Ctrl Pts',(3.07755425091957,25.8264725772184,-7.98979635505079));
#44844=CARTESIAN_POINT('Ctrl Pts',(3.0876868810919,25.825901734945,-7.99138961432908));
#44845=CARTESIAN_POINT('Ctrl Pts',(3.09783460752958,25.8253272787821,-7.99299320423445));
#44846=CARTESIAN_POINT('Ctrl Pts',(3.10798233396726,25.8247528226193,-7.99459679413982));
#44847=CARTESIAN_POINT('Ctrl Pts',(3.11649242506835,25.8242692127508,-7.99594695059774));
#44848=CARTESIAN_POINT('Ctrl Pts',(3.12832304853956,25.82359304553,-7.99783503294886));
#44849=CARTESIAN_POINT('Ctrl Pts',(3.24396953136902,25.8169833887294,-8.01629137920404));
#44850=CARTESIAN_POINT('Ctrl Pts',(3.35682435864532,25.8101922685851,-8.03535487522875));
#44851=CARTESIAN_POINT('Ctrl Pts',(3.46689563034231,25.8032667769389,-8.05487934571839));
#44852=CARTESIAN_POINT('Ctrl Pts',(3.6391333436612,25.7924298816586,-8.08543091561534));
#44853=CARTESIAN_POINT('Ctrl Pts',(3.80455492699797,25.7812649336087,-8.11710823621666));
#44854=CARTESIAN_POINT('Ctrl Pts',(3.96321661982111,25.7699421395512,-8.14939090713435));
#44855=CARTESIAN_POINT('Ctrl Pts',(4.12187831264424,25.7586193454937,-8.18167357805204));
#44856=CARTESIAN_POINT('Ctrl Pts',(4.27378038615049,25.7471386169463,-8.21456188766466));
#44857=CARTESIAN_POINT('Ctrl Pts',(4.41899134481302,25.7356523279005,-8.24759224460065));
#44858=CARTESIAN_POINT('Ctrl Pts',(4.56352096949038,25.7242199328525,-8.28046762215402));
#44859=CARTESIAN_POINT('Ctrl Pts',(4.70142263449432,25.7127820946714,-8.31348398400438));
#44860=CARTESIAN_POINT('Ctrl Pts',(4.83277716227932,25.701475689374,-8.34623545712527));
#44861=CARTESIAN_POINT('Ctrl Pts',(4.90532510903957,25.6952310893333,-8.364324305438));
#44862=CARTESIAN_POINT('Ctrl Pts',(4.97587596872295,25.6890262679304,-8.38233324870066));
#44863=CARTESIAN_POINT('Ctrl Pts',(5.04444366156708,25.6828820630984,-8.40020029227818));
#44864=CARTESIAN_POINT('Ctrl Pts',(5.13538873989178,25.6747326684417,-8.42389832863012));
#44865=CARTESIAN_POINT('Ctrl Pts',(5.22284501849858,25.6666900645241,-8.44734628553018));
#44866=CARTESIAN_POINT('Ctrl Pts',(5.30684506809983,25.6587988385195,-8.47041118653151));
#44867=CARTESIAN_POINT('Ctrl Pts',(5.42689981782459,25.6475205218101,-8.50337605893679));
#44868=CARTESIAN_POINT('Ctrl Pts',(5.5398950614998,25.6365523282452,-8.53555660222992));
#44869=CARTESIAN_POINT('Ctrl Pts',(5.64592784626714,25.626011852568,-8.56661221179925));
#44870=CARTESIAN_POINT('Ctrl Pts',(5.75378710344553,25.615289811462,-8.59820277114107));
#44871=CARTESIAN_POINT('Ctrl Pts',(5.8544421213826,25.6050102665336,-8.6286293612162));
#44872=CARTESIAN_POINT('Ctrl Pts',(5.94798770048386,25.5952770852613,-8.65758355223814));
#44873=CARTESIAN_POINT('Ctrl Pts',(6.0249647423883,25.5872678184433,-8.68140945611321));
#44874=CARTESIAN_POINT('Ctrl Pts',(6.09712761964016,25.5796281190708,-8.70423930677315));
#44875=CARTESIAN_POINT('Ctrl Pts',(6.16452450090577,25.5724066275389,-8.72592555602332));
#44876=CARTESIAN_POINT('Ctrl Pts',(6.201659121019,25.5684276994394,-8.73787433781357));
#44877=CARTESIAN_POINT('Ctrl Pts',(6.23734677867825,25.5645756133094,-8.74947634942516));
#44878=CARTESIAN_POINT('Ctrl Pts',(6.27159479316256,25.5608580129641,-8.76071029006199));
#44879=CARTESIAN_POINT('Ctrl Pts',(-6.390311350175,25.6807323022503,-8.98425322501931));
#44880=CARTESIAN_POINT('Ctrl Pts',(-4.260207566783,25.9287942543074,-8.27686643699921));
#44881=CARTESIAN_POINT('Ctrl Pts',(0.0001663376502052,26.1774622431302,
-7.56886858723369));
#44882=CARTESIAN_POINT('Ctrl Pts',(4.260540242084,25.9287748360782,-8.27692172383348));
#44883=CARTESIAN_POINT('Ctrl Pts',(6.390810363126,25.680674187269,-8.98441894883408));
#44884=CARTESIAN_POINT('Ctrl Pts',(-6.390311350175,25.1149800030297,-8.18394436969906));
#44885=CARTESIAN_POINT('Ctrl Pts',(-4.260207566783,25.3660541768592,-7.53598542510633));
#44886=CARTESIAN_POINT('Ctrl Pts',(0.0001663376502052,25.6190332007536,
-6.88615243075911));
#44887=CARTESIAN_POINT('Ctrl Pts',(4.260540242084,25.3660344219837,-7.53603616990792));
#44888=CARTESIAN_POINT('Ctrl Pts',(6.390810363126,25.1149211823672,-8.18409617097628));
#44889=CARTESIAN_POINT('Ctrl Pts',(-6.390311350175,23.7052267659156,-6.6337432666024));
#44890=CARTESIAN_POINT('Ctrl Pts',(-4.260207566783,23.9981304018685,-6.09525796678867));
#44891=CARTESIAN_POINT('Ctrl Pts',(0.0001663376502052,24.2900543482721,
-5.55781881254414));
#44892=CARTESIAN_POINT('Ctrl Pts',(4.260540242084,23.9981076058214,-6.09529993486804));
#44893=CARTESIAN_POINT('Ctrl Pts',(6.390810363126,23.7051581455831,-6.63386942084684));
#44894=CARTESIAN_POINT('Ctrl Pts',(-6.390311350175,21.0044950488536,-4.89945807529049));
#44895=CARTESIAN_POINT('Ctrl Pts',(-4.260207566783,21.4424839272,-4.44478852896696));
#44896=CARTESIAN_POINT('Ctrl Pts',(0.0001663376502052,21.8807691942899,
-3.98943207395094));
#44897=CARTESIAN_POINT('Ctrl Pts',(4.260540242084,21.4424497019397,-4.44482408729352));
#44898=CARTESIAN_POINT('Ctrl Pts',(6.390810363126,21.0043924385214,-4.89956459350057));
#44899=CARTESIAN_POINT('Ctrl Pts',(-6.390311350175,18.1258724665889,-4.02654101163599));
#44900=CARTESIAN_POINT('Ctrl Pts',(-4.260207566783,18.7395194568021,-3.53815117609504));
#44901=CARTESIAN_POINT('Ctrl Pts',(0.0001663376502052,19.3531464197629,
-3.05107327276496));
#44902=CARTESIAN_POINT('Ctrl Pts',(4.260540242084,18.7394715392942,-3.53818921151541));
#44903=CARTESIAN_POINT('Ctrl Pts',(6.390810363126,18.1257287037498,-4.02665542972081));
#44904=CARTESIAN_POINT('Ctrl Pts',(-6.390311350175,16.240422330399,-3.91824273036391));
#44905=CARTESIAN_POINT('Ctrl Pts',(-4.260207566783,16.9591796068581,-3.34435593602518));
#44906=CARTESIAN_POINT('Ctrl Pts',(0.0001663376502052,17.6779466440266,
-2.76852020743102));
#44907=CARTESIAN_POINT('Ctrl Pts',(4.260540242084,16.9591234790623,-3.34440090245649));
#44908=CARTESIAN_POINT('Ctrl Pts',(6.390810363126,16.2402539427348,-3.91837717831515));
#44909=CARTESIAN_POINT('Ctrl Pts',(-6.390311350175,15.4604268853052,-3.94960622933079));
#44910=CARTESIAN_POINT('Ctrl Pts',(-4.260207566783,16.2185124735635,-3.32899325071769));
#44911=CARTESIAN_POINT('Ctrl Pts',(0.0001663376502052,16.9766190503815,
-2.70682781485386));
#44912=CARTESIAN_POINT('Ctrl Pts',(4.260540242084,16.2184532737935,-3.32904183498501));
#44913=CARTESIAN_POINT('Ctrl Pts',(6.390810363126,15.4602492839623,-3.9497516241131));
#44914=CARTESIAN_POINT('',(-6.26385894387447,15.8144218171323,-3.90574358261498));
#44915=CARTESIAN_POINT('Ctrl Pts',(-6.27159552384793,25.5608567088063,-8.76070944182709));
#44916=CARTESIAN_POINT('Ctrl Pts',(-6.27195777365649,25.4158727521427,-8.56459404632321));
#44917=CARTESIAN_POINT('Ctrl Pts',(-6.27229031339005,25.2662939880144,-8.37478230713065));
#44918=CARTESIAN_POINT('Ctrl Pts',(-6.27259314329467,25.1127468329758,-8.19135361540759));
#44919=CARTESIAN_POINT('Ctrl Pts',(-6.27289863603481,24.9578495113491,-8.00631200359623));
#44920=CARTESIAN_POINT('Ctrl Pts',(-6.27317389416156,24.7989136560697,-7.82776610778095));
#44921=CARTESIAN_POINT('Ctrl Pts',(-6.27341891792754,24.6365419304632,-7.65576216835644));
#44922=CARTESIAN_POINT('Ctrl Pts',(-6.27366754313708,24.4717836094022,-7.48123005588655));
#44923=CARTESIAN_POINT('Ctrl Pts',(-6.27388503866392,24.3034876610362,-7.3134335727354));
#44924=CARTESIAN_POINT('Ctrl Pts',(-6.27407140477198,24.1322426600605,-7.15238583194492));
#44925=CARTESIAN_POINT('Ctrl Pts',(-6.27421804520854,23.997500125787,-7.02566691688459));
#44926=CARTESIAN_POINT('Ctrl Pts',(-6.27434541285329,23.8609309481042,-6.90312555205716));
#44927=CARTESIAN_POINT('Ctrl Pts',(-6.27445350783479,23.7228045338919,-6.78475354206035));
#44928=CARTESIAN_POINT('Ctrl Pts',(-6.27450263029994,23.6600346450967,-6.73096080483236));
#44929=CARTESIAN_POINT('Ctrl Pts',(-6.27454777269265,23.5969429742338,-6.67802891099079));
#44930=CARTESIAN_POINT('Ctrl Pts',(-6.27458893502498,23.5335572607895,-6.62595230104111));
#44931=CARTESIAN_POINT('Ctrl Pts',(-6.2747071268515,23.351554132648,-6.47642166710454));
#44932=CARTESIAN_POINT('Ctrl Pts',(-6.27479250388727,23.1671305121251,-6.33394416675351));
#44933=CARTESIAN_POINT('Ctrl Pts',(-6.27484506613229,22.9809077959271,-6.19837352650065));
#44934=CARTESIAN_POINT('Ctrl Pts',(-6.27489762837732,22.7946850797292,-6.0628028862478));
#44935=CARTESIAN_POINT('Ctrl Pts',(-6.27491737583159,22.6066631058893,-5.93413899916805));
#44936=CARTESIAN_POINT('Ctrl Pts',(-6.27490430849512,22.4174128626672,-5.81221513152887));
#44937=CARTESIAN_POINT('Ctrl Pts',(-6.27489476886027,22.2792532446046,-5.72320623675051));
#44938=CARTESIAN_POINT('Ctrl Pts',(-6.27486754212272,22.1401875184331,-5.63763292305786));
#44939=CARTESIAN_POINT('Ctrl Pts',(-6.27482284547966,22.0006885576582,-5.5556073289692));
#44940=CARTESIAN_POINT('Ctrl Pts',(-6.27477793189728,21.8605125256569,-5.47318361600363));
#44941=CARTESIAN_POINT('Ctrl Pts',(-6.27471537841422,21.7198993850789,-5.39434222334161));
#44942=CARTESIAN_POINT('Ctrl Pts',(-6.27463540540562,21.5793421829761,-5.31914585597933));
#44943=CARTESIAN_POINT('Ctrl Pts',(-6.27457693026747,21.4765687353424,-5.26416333066059));
#44944=CARTESIAN_POINT('Ctrl Pts',(-6.27450914207864,21.3738254880783,-5.2111284861831));
#44945=CARTESIAN_POINT('Ctrl Pts',(-6.27443212698732,21.2713080572712,-5.16004844385829));
#44946=CARTESIAN_POINT('Ctrl Pts',(-6.27435635557793,21.1704461341697,-5.10979327007536));
#44947=CARTESIAN_POINT('Ctrl Pts',(-6.2742702487733,21.0681857430153,-5.06062314250506));
#44948=CARTESIAN_POINT('Ctrl Pts',(-6.27417380657344,20.9645377930346,-5.01262251543797));
#44949=CARTESIAN_POINT('Ctrl Pts',(-6.27399075735707,20.7678119193992,-4.92151636913622));
#44950=CARTESIAN_POINT('Ctrl Pts',(-6.27377047509006,20.5660845709857,-4.83462207821818));
#44951=CARTESIAN_POINT('Ctrl Pts',(-6.27351295977241,20.359498064142,-4.75246107710196));
#44952=CARTESIAN_POINT('Ctrl Pts',(-6.27325823661086,20.155151508612,-4.67119092140055));
#44953=CARTESIAN_POINT('Ctrl Pts',(-6.2729670834335,19.946050481584,-4.59455195740143));
#44954=CARTESIAN_POINT('Ctrl Pts',(-6.27263950024032,19.7323768917561,-4.52307344733918));
#44955=CARTESIAN_POINT('Ctrl Pts',(-6.2723170042366,19.5220215369732,-4.45270495979887));
#44956=CARTESIAN_POINT('Ctrl Pts',(-6.27195920090826,19.3072344669029,-4.38733790193485));
#44957=CARTESIAN_POINT('Ctrl Pts',(-6.27156609025531,19.0882335843155,-4.3275012229039));
#44958=CARTESIAN_POINT('Ctrl Pts',(-6.27136275697641,18.9749571640432,-4.29655118872356));
#44959=CARTESIAN_POINT('Ctrl Pts',(-6.27114997760678,18.86055411936,-4.26708114042404));
#44960=CARTESIAN_POINT('Ctrl Pts',(-6.27092775214643,18.7450594689835,-4.23916684282755));
#44961=CARTESIAN_POINT('Ctrl Pts',(-6.27050608511531,18.525911373813,-4.18620018916566));
#44962=CARTESIAN_POINT('Ctrl Pts',(-6.2700504091853,18.3028302897812,-4.13883345388171));
#44963=CARTESIAN_POINT('Ctrl Pts',(-6.26956072372642,18.0760898397093,-4.09760201550297));
#44964=CARTESIAN_POINT('Ctrl Pts',(-6.26938505591299,17.9947498726805,-4.0828108133279));
#44965=CARTESIAN_POINT('Ctrl Pts',(-6.26920501136115,17.9129394062442,-4.06880939222112));
#44966=CARTESIAN_POINT('Ctrl Pts',(-6.26902059004181,17.830672539127,-4.05562321484025));
#44967=CARTESIAN_POINT('Ctrl Pts',(-6.26850854405841,17.6022584977174,-4.0190117797407));
#44968=CARTESIAN_POINT('Ctrl Pts',(-6.26796275775828,17.3703223746845,-3.98868456769828));
#44969=CARTESIAN_POINT('Ctrl Pts',(-6.2673832305189,17.1352158000369,-3.96507801654729));
#44970=CARTESIAN_POINT('Ctrl Pts',(-6.26681232023244,16.9036050097943,-3.94182246967379));
#44971=CARTESIAN_POINT('Ctrl Pts',(-6.26620866493078,16.6689173034159,-3.92508923644793));
#44972=CARTESIAN_POINT('Ctrl Pts',(-6.26557226401876,16.4315383934375,-3.91530365129545));
#44973=CARTESIAN_POINT('Ctrl Pts',(-6.26502584939568,16.2277245629199,-3.90690173558202));
#44974=CARTESIAN_POINT('Ctrl Pts',(-6.26445529483575,16.0219275203492,-3.90362173020364));
#44975=CARTESIAN_POINT('Ctrl Pts',(-6.26386059996225,15.8144217505981,-3.90573752907647));
#44976=CARTESIAN_POINT('Ctrl Pts',(6.26385988960052,15.8144313888753,-3.90573722891367));
#44977=CARTESIAN_POINT('Ctrl Pts',(5.97383890811555,15.9109016778241,-3.82533638560084));
#44978=CARTESIAN_POINT('Ctrl Pts',(5.68187770057698,16.0000524237085,-3.74992558202442));
#44979=CARTESIAN_POINT('Ctrl Pts',(5.38846872966892,16.0819645988975,-3.67979129585554));
#44980=CARTESIAN_POINT('Ctrl Pts',(5.11338321554584,16.1587613401665,-3.61403691176594));
#44981=CARTESIAN_POINT('Ctrl Pts',(4.8370251180331,16.2291950416424,-3.55292118456409));
#44982=CARTESIAN_POINT('Ctrl Pts',(4.55980027851165,16.2933699268073,-3.49665879142387));
#44983=CARTESIAN_POINT('Ctrl Pts',(4.30239166101817,16.3529575470819,-3.44441807280681));
#44984=CARTESIAN_POINT('Ctrl Pts',(4.04423578353628,16.4071490501026,-3.39636191484229));
#44985=CARTESIAN_POINT('Ctrl Pts',(3.78565753068499,16.4560640033003,-3.35263740201647));
#44986=CARTESIAN_POINT('Ctrl Pts',(3.57067796546936,16.4967314424799,-3.31628524690324));
#44987=CARTESIAN_POINT('Ctrl Pts',(3.35540644993641,16.53375215926,-3.28292688525913));
#44988=CARTESIAN_POINT('Ctrl Pts',(3.14002968425104,16.5672169853369,-3.25263029902007));
#44989=CARTESIAN_POINT('Ctrl Pts',(2.89780164180822,16.6048539109611,-3.21855660145092));
#44990=CARTESIAN_POINT('Ctrl Pts',(2.65545154831624,16.6380109389512,-3.18835920226728));
#44991=CARTESIAN_POINT('Ctrl Pts',(2.41322309383044,16.6667127080183,-3.16209554360299));
#44992=CARTESIAN_POINT('Ctrl Pts',(2.17467399151019,16.6949785088322,-3.13623081928184));
#44993=CARTESIAN_POINT('Ctrl Pts',(1.93624286096661,16.7189233572091,-3.11418128167405));
#44994=CARTESIAN_POINT('Ctrl Pts',(1.69816245541642,16.7386097374021,-3.09596954709885));
#44995=CARTESIAN_POINT('Ctrl Pts',(1.46175003732677,16.7581581951347,-3.07788540364077));
#44996=CARTESIAN_POINT('Ctrl Pts',(1.22568344709819,16.7735076019663,-3.06358553975951));
#44997=CARTESIAN_POINT('Ctrl Pts',(0.990190580144821,16.7847583353012,-3.05305920629704));
#44998=CARTESIAN_POINT('Ctrl Pts',(0.756490769869116,16.7959234048841,-3.04261302096284));
#44999=CARTESIAN_POINT('Ctrl Pts',(0.523355979403398,16.8030519622097,-3.03588315603065));
#45000=CARTESIAN_POINT('Ctrl Pts',(0.291008938069498,16.8062812827463,-3.0328258709267));
#45001=CARTESIAN_POINT('Ctrl Pts',(0.193862822501669,16.8076314869247,-3.03154759610845));
#45002=CARTESIAN_POINT('Ctrl Pts',(0.0968544166298517,16.8083005240372,
-3.03091093566987));
#45003=CARTESIAN_POINT('Ctrl Pts',(-5.14033260401447E-13,16.8083004872782,
-3.03091093310305));
#45004=CARTESIAN_POINT('Ctrl Pts',(-7.96995737912801E-7,16.8083004872779,
-3.03091093310303));
#45005=CARTESIAN_POINT('Ctrl Pts',(-1.59399094937538E-6,16.8083004872776,
-3.03091093310305));
#45006=CARTESIAN_POINT('Ctrl Pts',(-2.39098615129052E-6,16.8083004872772,
-3.03091093310312));
#45007=CARTESIAN_POINT('Ctrl Pts',(-0.230506131557345,16.8083003735928,
-3.03091095192717));
#45008=CARTESIAN_POINT('Ctrl Pts',(-0.461891800831802,16.8045079999109,
-3.03451929091951));
#45009=CARTESIAN_POINT('Ctrl Pts',(-0.693935583712521,16.7967708693938,
-3.04179370678685));
#45010=CARTESIAN_POINT('Ctrl Pts',(-0.928010239167388,16.7889660226639,
-3.04913178913771));
#45011=CARTESIAN_POINT('Ctrl Pts',(-1.1627545784042,16.7771470646875,-3.06020038435807));
#45012=CARTESIAN_POINT('Ctrl Pts',(-1.39793885818094,16.7611979788335,-3.07502429701105));
#45013=CARTESIAN_POINT('Ctrl Pts',(-1.63471559035675,16.7451409003871,-3.08994858361459));
#45014=CARTESIAN_POINT('Ctrl Pts',(-1.87193824099098,16.7248976083887,-3.10867916066466));
#45015=CARTESIAN_POINT('Ctrl Pts',(-2.10937236833873,16.7003903422879,-3.13120709605691));
#45016=CARTESIAN_POINT('Ctrl Pts',(-2.34982826438089,16.6755711779342,-3.1540217392223));
#45017=CARTESIAN_POINT('Ctrl Pts',(-2.59050105421909,16.6463788347557,-3.18073096523689));
#45018=CARTESIAN_POINT('Ctrl Pts',(-2.83114723065116,16.6127737269867,-3.21129121206657));
#45019=CARTESIAN_POINT('Ctrl Pts',(-2.93418537812882,16.5983849338563,-3.22437627855912));
#45020=CARTESIAN_POINT('Ctrl Pts',(-3.0372186465189,16.5831876475592,-3.23816694041524));
#45021=CARTESIAN_POINT('Ctrl Pts',(-3.14022792105303,16.5671810042051,-3.25265793254405));
#45022=CARTESIAN_POINT('Ctrl Pts',(-3.40298085139679,16.5263517442645,-3.28962111535118));
#45023=CARTESIAN_POINT('Ctrl Pts',(-3.66557290592767,16.4802294293196,-3.3311415890159));
#45024=CARTESIAN_POINT('Ctrl Pts',(-3.92766532767384,16.4286539573448,-3.37709229468276));
#45025=CARTESIAN_POINT('Ctrl Pts',(-4.19885767852042,16.3752877691976,-3.42463842291429));
#45026=CARTESIAN_POINT('Ctrl Pts',(-4.46951509946873,16.3160835074943,-3.47692733800474));
#45027=CARTESIAN_POINT('Ctrl Pts',(-4.73926230901666,16.2509126285198,-3.53378214924202));
#45028=CARTESIAN_POINT('Ctrl Pts',(-5.03507254493692,16.1794449269006,-3.59613028308734));
#45029=CARTESIAN_POINT('Ctrl Pts',(-5.32978818261875,16.1008019704071,-3.6639688704703));
#45030=CARTESIAN_POINT('Ctrl Pts',(-5.62291431247201,16.014869556307,-3.73702784181589));
#45031=CARTESIAN_POINT('Ctrl Pts',(-5.83747944819202,15.9519679647521,-3.79050621343079));
#45032=CARTESIAN_POINT('Ctrl Pts',(-6.05119291280412,15.8851618807612,-3.84678083666339));
#45033=CARTESIAN_POINT('Ctrl Pts',(-6.26386059996225,15.8144217505981,-3.90573752907647));
#45034=CARTESIAN_POINT('Ctrl Pts',(6.38247014577615,15.7729006312219,-3.93895139429922));
#45035=CARTESIAN_POINT('Ctrl Pts',(5.83981133037685,15.9681476187677,-3.78553079687121));
#45036=CARTESIAN_POINT('Ctrl Pts',(4.52590233473943,16.369552788887,-3.46059646224381));
#45037=CARTESIAN_POINT('Ctrl Pts',(2.3863676788619,16.7684714876093,-3.11895962047874));
#45038=CARTESIAN_POINT('Ctrl Pts',(0.000145921253848828,16.9128764845052,
-2.99096322074304));
#45039=CARTESIAN_POINT('Ctrl Pts',(-2.38607593148343,16.7685070072141,-3.11892840793774));
#45040=CARTESIAN_POINT('Ctrl Pts',(-4.52571177279445,16.369604017143,-3.4605539154598));
#45041=CARTESIAN_POINT('Ctrl Pts',(-5.83971599368801,15.9681816437148,-3.78550400961911));
#45042=CARTESIAN_POINT('Ctrl Pts',(-6.38246546509551,15.7729022400972,-3.93895010743252));
#45043=CARTESIAN_POINT('Ctrl Pts',(6.17792611310107,15.1551690118173,-3.88975075307634));
#45044=CARTESIAN_POINT('Ctrl Pts',(5.65238026945388,15.3441929863978,-3.74331335325337));
#45045=CARTESIAN_POINT('Ctrl Pts',(4.38005561086563,15.7328411772922,-3.43305555917197));
#45046=CARTESIAN_POINT('Ctrl Pts',(2.30906659857668,16.119049889924,-3.10675668983587));
#45047=CARTESIAN_POINT('Ctrl Pts',(0.000141183631923982,16.2588285236581,
-2.98451005281823));
#45048=CARTESIAN_POINT('Ctrl Pts',(-2.3087842620022,16.119084273518,-3.10672687830997));
#45049=CARTESIAN_POINT('Ctrl Pts',(-4.37987109836434,15.7328907786648,-3.43301492630012));
#45050=CARTESIAN_POINT('Ctrl Pts',(-5.65228794008332,15.3442259268502,-3.743287783153));
#45051=CARTESIAN_POINT('Ctrl Pts',(-6.177921579923,15.1551705696293,-3.88974952300261));
#45052=CARTESIAN_POINT('Ctrl Pts',(6.17628882186073,14.7460473480683,-3.38362402344176));
#45053=CARTESIAN_POINT('Ctrl Pts',(5.65209551729923,14.9328346346656,-3.23898800415555));
#45054=CARTESIAN_POINT('Ctrl Pts',(4.3823925489299,15.3172277280071,-2.93223668842095));
#45055=CARTESIAN_POINT('Ctrl Pts',(2.31204710154926,15.7000802439509,-2.60875661073035));
#45056=CARTESIAN_POINT('Ctrl Pts',(0.000141413130813221,15.8388906345013,
-2.48731588780259));
#45057=CARTESIAN_POINT('Ctrl Pts',(-2.31176457385417,15.7001143733183,-2.60872701329724));
#45058=CARTESIAN_POINT('Ctrl Pts',(-4.38220833686575,15.3172768284095,-2.93219647030261));
#45059=CARTESIAN_POINT('Ctrl Pts',(-5.65200342190241,14.9328671899495,-3.23896275109574));
#45060=CARTESIAN_POINT('Ctrl Pts',(-6.176284300804,14.7460488896197,-3.38362281162595));
#45061=CARTESIAN_POINT('Ctrl Pts',(6.37612500939897,14.8213329701347,-2.77073838960337));
#45062=CARTESIAN_POINT('Ctrl Pts',(5.83680124907823,15.0113419617907,-2.62156111143535));
#45063=CARTESIAN_POINT('Ctrl Pts',(4.52946237799516,15.4027707876115,-2.30490021431075));
#45064=CARTESIAN_POINT('Ctrl Pts',(2.3922729610528,15.7937874269067,-1.96995867414585));
#45065=CARTESIAN_POINT('Ctrl Pts',(0.000146391209654873,15.9359006779543,
-1.84389364375196));
#45066=CARTESIAN_POINT('Ctrl Pts',(-2.39198089092465,15.7938223457685,-1.96992797308875));
#45067=CARTESIAN_POINT('Ctrl Pts',(-4.52927258508639,15.4028208397379,-2.30485864836242));
#45068=CARTESIAN_POINT('Ctrl Pts',(-5.83670648990435,15.0113750845678,-2.62153507085255));
#45069=CARTESIAN_POINT('Ctrl Pts',(-6.376120358534,14.8213345408617,-2.77073714556678));
#45070=CARTESIAN_POINT('',(-6.24994532642006,14.8593843574536,-2.76546731080821));
#45071=CARTESIAN_POINT('Origin',(-6.52772047565603,15.803815900541,-2.9412381944653));
#45072=CARTESIAN_POINT('Ctrl Pts',(6.24994434955625,14.8593821393419,-2.76546470491022));
#45073=CARTESIAN_POINT('Ctrl Pts',(5.96223477282027,14.9585365244006,-2.68736489781825));
#45074=CARTESIAN_POINT('Ctrl Pts',(5.66971282350541,15.0511199847504,-2.613288972184));
#45075=CARTESIAN_POINT('Ctrl Pts',(5.3725988245355,15.1368745061914,-2.54385966649289));
#45076=CARTESIAN_POINT('Ctrl Pts',(5.16122334739288,15.1978827486491,-2.4944656538613));
#45077=CARTESIAN_POINT('Ctrl Pts',(4.94752407483941,15.2554341029525,-2.4474241767453));
#45078=CARTESIAN_POINT('Ctrl Pts',(4.7315875681965,15.3094273221724,-2.4029712482205));
#45079=CARTESIAN_POINT('Ctrl Pts',(4.7256242571508,15.3109184010343,-2.40174363440102));
#45080=CARTESIAN_POINT('Ctrl Pts',(4.71965924273307,15.3124067666448,-2.40051798699696));
#45081=CARTESIAN_POINT('Ctrl Pts',(4.71369252616525,15.3138924170786,-2.39929431020639));
#45082=CARTESIAN_POINT('Ctrl Pts',(4.45978012163924,15.3771139677675,-2.34722099438445));
#45083=CARTESIAN_POINT('Ctrl Pts',(4.20278480382731,15.435420451617,-2.298714158249));
#45084=CARTESIAN_POINT('Ctrl Pts',(3.94288022045684,15.4886619316243,-2.2540814333537));
#45085=CARTESIAN_POINT('Ctrl Pts',(3.80987416504048,15.5159082354349,-2.23124065615838));
#45086=CARTESIAN_POINT('Ctrl Pts',(3.67610656094729,15.541827855014,-2.20941360390684));
#45087=CARTESIAN_POINT('Ctrl Pts',(3.54160298166754,15.5663992231882,-2.18863623548886));
#45088=CARTESIAN_POINT('Ctrl Pts',(3.47435119202767,15.5786849072753,-2.17824755127986));
#45089=CARTESIAN_POINT('Ctrl Pts',(3.40691540524463,15.5906335095712,-2.16812128533049));
#45090=CARTESIAN_POINT('Ctrl Pts',(3.33929900391423,15.6022422426552,-2.15826152779633));
#45091=CARTESIAN_POINT('Ctrl Pts',(3.30549080324904,15.6080466091972,-2.15333164902926));
#45092=CARTESIAN_POINT('Ctrl Pts',(3.27163744877826,15.6137660072614,-2.14846839720879));
#45093=CARTESIAN_POINT('Ctrl Pts',(3.23773936865723,15.6194000821641,-2.14367226990373));
#45094=CARTESIAN_POINT('Ctrl Pts',(3.21152573531064,15.6237569535037,-2.13996338957158));
#45095=CARTESIAN_POINT('Ctrl Pts',(3.18421433654936,15.6282372847887,-2.13614588435894));
#45096=CARTESIAN_POINT('Ctrl Pts',(3.1582898601169,15.63243545858,-2.13256563781385));
#45097=CARTESIAN_POINT('Ctrl Pts',(3.15069017881112,15.6336661404402,-2.13151609944382));
#45098=CARTESIAN_POINT('Ctrl Pts',(3.14320976052125,15.6348728406731,-2.13048673700716));
#45099=CARTESIAN_POINT('Ctrl Pts',(3.1359113824538,15.6360459784053,-2.12948575159818));
#45100=CARTESIAN_POINT('Ctrl Pts',(2.87775719540782,15.6775415565695,-2.0940794500733));
#45101=CARTESIAN_POINT('Ctrl Pts',(2.61837526546646,15.7138739789539,-2.06281531592252));
#45102=CARTESIAN_POINT('Ctrl Pts',(2.35795007230111,15.7450248387696,-2.03590284652233));
#45103=CARTESIAN_POINT('Ctrl Pts',(2.05596056132431,15.7811474304739,-2.00469509978109));
#45104=CARTESIAN_POINT('Ctrl Pts',(1.75256804347705,15.8103033922598,-1.97933798480163));
#45105=CARTESIAN_POINT('Ctrl Pts',(1.44816290506226,15.8324815067107,-1.95997140574192));
#45106=CARTESIAN_POINT('Ctrl Pts',(1.14644744569396,15.8544636586031,-1.94077594692731));
#45107=CARTESIAN_POINT('Ctrl Pts',(0.843736620889954,15.8695907029274,-1.92746554146444));
#45108=CARTESIAN_POINT('Ctrl Pts',(0.540407879657201,15.8778133211475,-1.92020969609162));
#45109=CARTESIAN_POINT('Ctrl Pts',(0.360510778949315,15.8826899614948,-1.91590642584941));
#45110=CARTESIAN_POINT('Ctrl Pts',(0.180396322194014,15.885137313928,-1.91373342287414));
#45111=CARTESIAN_POINT('Ctrl Pts',(0.000144007191481506,15.8851386638734,
-1.91373185548263));
#45112=CARTESIAN_POINT('Ctrl Pts',(9.53315880905156E-5,15.8851386642379,
-1.91373185505937));
#45113=CARTESIAN_POINT('Ctrl Pts',(4.66559746552919E-5,15.885138664424,
-1.91373185479448));
#45114=CARTESIAN_POINT('Ctrl Pts',(-2.01964882728384E-6,15.8851386644318,
-1.91373185468797));
#45115=CARTESIAN_POINT('Ctrl Pts',(-0.298062756534573,15.8851387118627,
-1.91373120245655));
#45116=CARTESIAN_POINT('Ctrl Pts',(-0.595730756791502,15.8784609266372,
-1.91959815322724));
#45117=CARTESIAN_POINT('Ctrl Pts',(-0.892664018370692,15.8651644845163,
-1.93123666047278));
#45118=CARTESIAN_POINT('Ctrl Pts',(-1.12138444999966,15.8549225602372,-1.94020151805242));
#45119=CARTESIAN_POINT('Ctrl Pts',(-1.34966889347301,15.840752819092,-1.95259155229056));
#45120=CARTESIAN_POINT('Ctrl Pts',(-1.57735595186607,15.8226670203481,-1.96837642029373));
#45121=CARTESIAN_POINT('Ctrl Pts',(-1.8383182568047,15.8019380787905,-1.98646816238189));
#45122=CARTESIAN_POINT('Ctrl Pts',(-2.0984992486968,15.7760676159358,-2.00899841000987));
#45123=CARTESIAN_POINT('Ctrl Pts',(-2.35766799609165,15.7450658005388,-2.03581781779785));
#45124=CARTESIAN_POINT('Ctrl Pts',(-2.35834041617024,15.7449853655197,-2.03588740145126));
#45125=CARTESIAN_POINT('Ctrl Pts',(-2.3590128294376,15.7449048959452,-2.03595701398876));
#45126=CARTESIAN_POINT('Ctrl Pts',(-2.35968523589097,15.744824391816,-2.03602665540553));
#45127=CARTESIAN_POINT('Ctrl Pts',(-2.48960318705321,15.7292699135974,-2.04948231178473));
#45128=CARTESIAN_POINT('Ctrl Pts',(-2.61926666928655,15.712425704544,-2.06401477308485));
#45129=CARTESIAN_POINT('Ctrl Pts',(-2.74864747588165,15.6942949274031,-2.07959991770205));
#45130=CARTESIAN_POINT('Ctrl Pts',(-2.81333787917919,15.6852295388327,-2.08739249001066));
#45131=CARTESIAN_POINT('Ctrl Pts',(-2.87795761323466,15.675842495087,-2.09544823158194));
#45132=CARTESIAN_POINT('Ctrl Pts',(-2.94250321346813,15.6661341570901,-2.1037637162872));
#45133=CARTESIAN_POINT('Ctrl Pts',(-2.97477601358486,15.6612799880917,-2.10792145863982));
#45134=CARTESIAN_POINT('Ctrl Pts',(-3.00703028020938,15.6563454946965,-2.11214413667789));
#45135=CARTESIAN_POINT('Ctrl Pts',(-3.03926558210551,15.6513307183264,-2.11643130961707));
#45136=CARTESIAN_POINT('Ctrl Pts',(-3.064364380523,15.6474261524059,-2.11976935465006));
#45137=CARTESIAN_POINT('Ctrl Pts',(-3.08836657723838,15.6436450931043,-2.1229994894086));
#45138=CARTESIAN_POINT('Ctrl Pts',(-3.11380677381553,15.6395860007454,-2.12646439387274));
#45139=CARTESIAN_POINT('Ctrl Pts',(-3.12104034923816,15.6384318527955,-2.12744959254043));
#45140=CARTESIAN_POINT('Ctrl Pts',(-3.12839011457528,15.6372549869322,-2.1284539648356));
#45141=CARTESIAN_POINT('Ctrl Pts',(-3.13591416326753,15.6360455791301,-2.12948586516546));
#45142=CARTESIAN_POINT('Ctrl Pts',(-3.43719649088153,15.5876177695101,-2.1708058174891));
#45143=CARTESIAN_POINT('Ctrl Pts',(-3.73502117399232,15.5324414885685,-2.21754192480206));
#45144=CARTESIAN_POINT('Ctrl Pts',(-4.02908029278226,15.4707748211256,-2.26918834452949));
#45145=CARTESIAN_POINT('Ctrl Pts',(-4.25953208892564,15.4224471435727,-2.30966323352303));
#45146=CARTESIAN_POINT('Ctrl Pts',(-4.48767165484889,15.3701326152782,-2.35315478653788));
#45147=CARTESIAN_POINT('Ctrl Pts',(-4.71335824231695,15.3139426610573,-2.39943616491744));
#45148=CARTESIAN_POINT('Ctrl Pts',(-5.01356244980717,15.2391998025426,-2.46099881546688));
#45149=CARTESIAN_POINT('Ctrl Pts',(-5.3094265767787,15.1576010421758,-2.52749625938663));
#45150=CARTESIAN_POINT('Ctrl Pts',(-5.60075678418667,15.069395087537,-2.59838443704975));
#45151=CARTESIAN_POINT('Ctrl Pts',(-5.8197409198287,15.0030933301364,-2.65166894348975));
#45152=CARTESIAN_POINT('Ctrl Pts',(-6.0361635747021,14.9330577376595,-2.70743518407641));
#45153=CARTESIAN_POINT('Ctrl Pts',(-6.24994452515074,14.8593816330971,-2.76546680377027));
#45154=CARTESIAN_POINT('Ctrl Pts',(-6.2427709657445,15.8383026749575,-3.89994404666797));
#45155=CARTESIAN_POINT('Ctrl Pts',(-6.29815583222613,15.8190276923523,-3.91383371439998));
#45156=CARTESIAN_POINT('Ctrl Pts',(-6.44474178978945,15.7640294246474,-3.96332153595004));
#45157=CARTESIAN_POINT('Ctrl Pts',(-6.66526185116382,15.663015036285,-4.09559797813337));
#45158=CARTESIAN_POINT('Ctrl Pts',(-6.87369342521677,15.5379585762815,-4.31230158072116));
#45159=CARTESIAN_POINT('Ctrl Pts',(-7.01918565228154,15.4153897468304,-4.57079555903126));
#45160=CARTESIAN_POINT('Ctrl Pts',(-7.09651835747178,15.3064823826313,-4.83972908208072));
#45161=CARTESIAN_POINT('Ctrl Pts',(-7.10969900601091,15.2437103395232,-5.01815780639156));
#45162=CARTESIAN_POINT('Ctrl Pts',(-7.10784879018326,15.2163983333452,-5.10154097469548));
#45163=CARTESIAN_POINT('Ctrl Pts',(-6.04395578033757,15.2228359720061,-3.86290031537712));
#45164=CARTESIAN_POINT('Ctrl Pts',(-6.09276946335539,15.2058036729393,-3.87479654436034));
#45165=CARTESIAN_POINT('Ctrl Pts',(-6.22228199032594,15.1570815317897,-3.91732220179018));
#45166=CARTESIAN_POINT('Ctrl Pts',(-6.41829648081485,15.0670943798548,-4.03193268370061));
#45167=CARTESIAN_POINT('Ctrl Pts',(-6.60464058492451,14.9552980626184,-4.22123672601488));
#45168=CARTESIAN_POINT('Ctrl Pts',(-6.73521157215934,14.8457420429051,-4.44829710876009));
#45169=CARTESIAN_POINT('Ctrl Pts',(-6.80469367850032,14.7487886821563,-4.68514860236371));
#45170=CARTESIAN_POINT('Ctrl Pts',(-6.81649571524118,14.6933666369333,-4.84218285847006));
#45171=CARTESIAN_POINT('Ctrl Pts',(-6.81483976787885,14.6694087006988,-4.91540371267267));
#45172=CARTESIAN_POINT('Ctrl Pts',(-6.02805603627548,14.8073272184145,-3.3655266670929));
#45173=CARTESIAN_POINT('Ctrl Pts',(-6.09538291851958,14.7843156654749,-3.38182744412473));
#45174=CARTESIAN_POINT('Ctrl Pts',(-6.27265849572073,14.7191838386095,-3.43975761399766));
#45175=CARTESIAN_POINT('Ctrl Pts',(-6.53595052706497,14.6017994961237,-3.592883556401));
#45176=CARTESIAN_POINT('Ctrl Pts',(-6.78171369715551,14.4589479168646,-3.84041911230593));
#45177=CARTESIAN_POINT('Ctrl Pts',(-6.95183436314053,14.3204156154418,-4.13296218348673));
#45178=CARTESIAN_POINT('Ctrl Pts',(-7.0420260852345,14.1977825871932,-4.43614337260094));
#45179=CARTESIAN_POINT('Ctrl Pts',(-7.05751523271005,14.1268472965378,-4.63782502157415));
#45180=CARTESIAN_POINT('Ctrl Pts',(-7.05533881082366,14.0958150745125,-4.73255226145534));
#45181=CARTESIAN_POINT('Ctrl Pts',(-6.20650782976424,14.8758369048666,-2.74558929006944));
#45182=CARTESIAN_POINT('Ctrl Pts',(-6.30488567809951,14.8426759833281,-2.76970897684925));
#45183=CARTESIAN_POINT('Ctrl Pts',(-6.56239158597099,14.7495682389862,-2.85497534271012));
#45184=CARTESIAN_POINT('Ctrl Pts',(-6.93915150013541,14.584925472277,-3.07670868851015));
#45185=CARTESIAN_POINT('Ctrl Pts',(-7.28557448399626,14.3877425186133,-3.42866438866332));
#45186=CARTESIAN_POINT('Ctrl Pts',(-7.52291531247474,14.1978736014857,-3.83925449985577));
#45187=CARTESIAN_POINT('Ctrl Pts',(-7.64834332641638,14.0293214778286,-4.26225227400094));
#45188=CARTESIAN_POINT('Ctrl Pts',(-7.67008673407683,13.9305172526115,-4.54438303023317));
#45189=CARTESIAN_POINT('Ctrl Pts',(-7.66702779568007,13.8867739926947,-4.67771839241253));
#45190=CARTESIAN_POINT('',(-7.00001043090743,14.7967990244186,-4.92966193641599));
#45191=CARTESIAN_POINT('',(-7.00000027445822,14.5427414083387,-3.16613020376588));
#45192=CARTESIAN_POINT('Ctrl Pts',(-7.,14.7967990243833,-4.92966193665079));
#45193=CARTESIAN_POINT('Ctrl Pts',(-7.,14.7552771220866,-4.82520423675662));
#45194=CARTESIAN_POINT('Ctrl Pts',(-7.,14.7204230598774,-4.73114199069113));
#45195=CARTESIAN_POINT('Ctrl Pts',(-7.,14.6925169059846,-4.64926898759083));
#45196=CARTESIAN_POINT('Ctrl Pts',(-7.,14.6785638290383,-4.60833248604069));
#45197=CARTESIAN_POINT('Ctrl Pts',(-7.,14.6662969026635,-4.5704573646326));
#45198=CARTESIAN_POINT('Ctrl Pts',(-7.,14.65553053564,-4.53589212276887));
#45199=CARTESIAN_POINT('Ctrl Pts',(-7.,14.6501473521282,-4.518609501837));
#45200=CARTESIAN_POINT('Ctrl Pts',(-7.,14.6451376851526,-4.50215438545475));
#45201=CARTESIAN_POINT('Ctrl Pts',(-7.,14.6404714582614,-4.48655657212187));
#45202=CARTESIAN_POINT('Ctrl Pts',(-7.,14.6381383448158,-4.47875766545543));
#45203=CARTESIAN_POINT('Ctrl Pts',(-7.,14.6358910913914,-4.47117308455133));
#45204=CARTESIAN_POINT('Ctrl Pts',(-7.,14.6337256779967,-4.46380634029146));
#45205=CARTESIAN_POINT('Ctrl Pts',(-7.,14.6326429712994,-4.46012296816153));
#45206=CARTESIAN_POINT('Ctrl Pts',(-7.,14.6315807246095,-4.45649405519266));
#45207=CARTESIAN_POINT('Ctrl Pts',(-7.,14.6305384389577,-4.45292002921339));
#45208=CARTESIAN_POINT('Ctrl Pts',(-7.,14.6294961533059,-4.44934600323413));
#45209=CARTESIAN_POINT('Ctrl Pts',(-7.,14.6289683953982,-4.44753506389562));
#45210=CARTESIAN_POINT('Ctrl Pts',(-7.,14.6274709645299,-4.44236303548761));
#45211=CARTESIAN_POINT('Ctrl Pts',(-7.,14.6035120706366,-4.3596105809594));
#45212=CARTESIAN_POINT('Ctrl Pts',(-7.,14.5830405217098,-4.27937746873487));
#45213=CARTESIAN_POINT('Ctrl Pts',(-7.,14.5661444668209,-4.20228869892318));
#45214=CARTESIAN_POINT('Ctrl Pts',(-7.,14.5492484119319,-4.12519992911148));
#45215=CARTESIAN_POINT('Ctrl Pts',(-7.,14.5361344232984,-4.05274778190799));
#45216=CARTESIAN_POINT('Ctrl Pts',(-7.,14.5256556230562,-3.98124889454358));
#45217=CARTESIAN_POINT('Ctrl Pts',(-7.,14.5046980225716,-3.83825111981476));
#45218=CARTESIAN_POINT('Ctrl Pts',(-7.,14.4945186462401,-3.69578424712143));
#45219=CARTESIAN_POINT('Ctrl Pts',(-7.,14.4974035759029,-3.55816691131067));
#45220=CARTESIAN_POINT('Ctrl Pts',(-7.,14.5002885055657,-3.42054957549992));
#45221=CARTESIAN_POINT('Ctrl Pts',(-7.,14.516205703975,-3.28800621878016));
#45222=CARTESIAN_POINT('Ctrl Pts',(-7.,14.542741062884,-3.1661309938642));
#45223=CARTESIAN_POINT('Ctrl Pts',(-6.24994591275502,14.8593863510063,-2.76546768184339));
#45224=CARTESIAN_POINT('Ctrl Pts',(-6.299845029724,14.8421892411351,-2.77901288816629));
#45225=CARTESIAN_POINT('Ctrl Pts',(-6.34871496761958,14.8247258705584,-2.79444809502116));
#45226=CARTESIAN_POINT('Ctrl Pts',(-6.39657992132363,14.8070063190978,-2.81168411646804));
#45227=CARTESIAN_POINT('Ctrl Pts',(-6.42793513327259,14.7953986552708,-2.82297503108932));
#45228=CARTESIAN_POINT('Ctrl Pts',(-6.45885895078646,14.783680793141,-2.83503980941021));
#45229=CARTESIAN_POINT('Ctrl Pts',(-6.48935510410294,14.7718531612462,-2.8478647965535));
#45230=CARTESIAN_POINT('Ctrl Pts',(-6.53665117765749,14.7535098461971,-2.86775489642839));
#45231=CARTESIAN_POINT('Ctrl Pts',(-6.58292000167124,14.7349027780747,-2.88947137235263));
#45232=CARTESIAN_POINT('Ctrl Pts',(-6.62819541826187,14.7160216008304,-2.91297873974637));
#45233=CARTESIAN_POINT('Ctrl Pts',(-6.63503348051049,14.7131699282221,-2.91652911771402));
#45234=CARTESIAN_POINT('Ctrl Pts',(-6.64184883446373,14.7103119908072,-2.92012043062703));
#45235=CARTESIAN_POINT('Ctrl Pts',(-6.64864154341018,14.7074477408645,-2.92375264317202));
#45236=CARTESIAN_POINT('Ctrl Pts',(-6.69594095403225,14.6875032186967,-2.94904468998083));
#45237=CARTESIAN_POINT('Ctrl Pts',(-6.74212292260707,14.6672603945742,-2.97631459532374));
#45238=CARTESIAN_POINT('Ctrl Pts',(-6.78718059541533,14.6467045734034,-3.00556997718216));
#45239=CARTESIAN_POINT('Ctrl Pts',(-6.83223826822359,14.6261487522327,-3.03482535904057));
#45240=CARTESIAN_POINT('Ctrl Pts',(-6.87617231393712,14.605279683737,-3.0660666811726));
#45241=CARTESIAN_POINT('Ctrl Pts',(-6.9189314546316,14.5840807130254,-3.09934282893694));
#45242=CARTESIAN_POINT('Ctrl Pts',(-6.94644683168257,14.5704392398165,-3.12075592886526));
#45243=CARTESIAN_POINT('Ctrl Pts',(-6.97347470733396,14.5566611364393,-3.14301246594803));
#45244=CARTESIAN_POINT('Ctrl Pts',(-7.00000082163496,14.5427407797108,-3.1661291973434));
#45245=CARTESIAN_POINT('Ctrl Pts',(-6.26385534037038,15.8144219619575,-3.90575675456612));
#45246=CARTESIAN_POINT('Ctrl Pts',(-6.30612912668385,15.7872214193081,-3.91762094721362));
#45247=CARTESIAN_POINT('Ctrl Pts',(-6.34794394428928,15.7586530202396,-3.93244141861837));
#45248=CARTESIAN_POINT('Ctrl Pts',(-6.38887221657581,15.7287855297124,-3.95026172552475));
#45249=CARTESIAN_POINT('Ctrl Pts',(-6.43384338942066,15.6959677242225,-3.9698423248822));
#45250=CARTESIAN_POINT('Ctrl Pts',(-6.47774451336698,15.6615808963665,-3.99304561857202));
#45251=CARTESIAN_POINT('Ctrl Pts',(-6.52005083552343,15.6257531868192,-4.0197782938412));
#45252=CARTESIAN_POINT('Ctrl Pts',(-6.53777952313905,15.6107393960151,-4.03098076252246));
#45253=CARTESIAN_POINT('Ctrl Pts',(-6.55522760380306,15.5954728200784,-4.04280298375156));
#45254=CARTESIAN_POINT('Ctrl Pts',(-6.5723539047681,15.5799639707862,-4.05523818474512));
#45255=CARTESIAN_POINT('Ctrl Pts',(-6.58619729733292,15.5674279836271,-4.06528970546332));
#45256=CARTESIAN_POINT('Ctrl Pts',(-6.59983045220702,15.5547337111189,-4.07574174794345));
#45257=CARTESIAN_POINT('Ctrl Pts',(-6.61323081388031,15.5418870223125,-4.08659088585896));
#45258=CARTESIAN_POINT('Ctrl Pts',(-6.64590220353243,15.5105655411489,-4.11304214298688));
#45259=CARTESIAN_POINT('Ctrl Pts',(-6.67719136733343,15.4783372184194,-4.14185401750552));
#45260=CARTESIAN_POINT('Ctrl Pts',(-6.70681950123728,15.4453015233143,-4.17289744569691));
#45261=CARTESIAN_POINT('Ctrl Pts',(-6.72770964444803,15.4220087839183,-4.19478548166891));
#45262=CARTESIAN_POINT('Ctrl Pts',(-6.74777361636949,15.3983149027798,-4.2177828371642));
#45263=CARTESIAN_POINT('Ctrl Pts',(-6.76690562067418,15.3742584345528,-4.24184469883051));
#45264=CARTESIAN_POINT('Ctrl Pts',(-6.77618564902021,15.3625897821995,-4.25351596728547));
#45265=CARTESIAN_POINT('Ctrl Pts',(-6.7852463335436,15.3508358260357,-4.2654377471286));
#45266=CARTESIAN_POINT('Ctrl Pts',(-6.79407487600683,15.3390012936185,-4.27760496147909));
#45267=CARTESIAN_POINT('Ctrl Pts',(-6.79434693680216,15.33863660009,-4.27797990695021));
#45268=CARTESIAN_POINT('Ctrl Pts',(-6.79461877711129,15.338271830059,-4.27835508549851));
#45269=CARTESIAN_POINT('Ctrl Pts',(-6.79489039665138,15.3379069836732,-4.27873049688523));
#45270=CARTESIAN_POINT('Ctrl Pts',(-6.79943331814915,15.3318048141144,-4.2850093693798));
#45271=CARTESIAN_POINT('Ctrl Pts',(-6.80391448952032,15.3256812783291,-4.29135338184373));
#45272=CARTESIAN_POINT('Ctrl Pts',(-6.80833257737852,15.3195370717944,-4.29776142244535));
#45273=CARTESIAN_POINT('Ctrl Pts',(-6.81054162130762,15.3164649685271,-4.30096544274615));
#45274=CARTESIAN_POINT('Ctrl Pts',(-6.81273489404392,15.3133876975829,-4.30418547019675));
#45275=CARTESIAN_POINT('Ctrl Pts',(-6.81491222677554,15.3103053465848,-4.30742136632205));
#45276=CARTESIAN_POINT('Ctrl Pts',(-6.81652751375196,15.3080186582199,-4.30982196444484));
#45277=CARTESIAN_POINT('Ctrl Pts',(-6.8185572820015,15.3051233541833,-4.3128693695528));
#45278=CARTESIAN_POINT('Ctrl Pts',(-6.82005847796644,15.3029677319571,-4.31514418563211));
#45279=CARTESIAN_POINT('Ctrl Pts',(-6.82058082528438,15.3022176743267,-4.31593571725461));
#45280=CARTESIAN_POINT('Ctrl Pts',(-6.82103962524178,15.3015571937407,-4.31663336823083));
#45281=CARTESIAN_POINT('Ctrl Pts',(-6.82139623449801,15.3010431417636,-4.31717652240758));
#45282=CARTESIAN_POINT('Ctrl Pts',(-6.83575184522523,15.2803495395993,-4.33904165851986));
#45283=CARTESIAN_POINT('Ctrl Pts',(-6.85002639055998,15.2584767386076,-4.36258429588056));
#45284=CARTESIAN_POINT('Ctrl Pts',(-6.86393640900324,15.2354494940946,-4.38791385863263));
#45285=CARTESIAN_POINT('Ctrl Pts',(-6.87708940977073,15.2136754492946,-4.41186492380748));
#45286=CARTESIAN_POINT('Ctrl Pts',(-6.88991660004127,15.1908690825995,-4.4374138196626));
#45287=CARTESIAN_POINT('Ctrl Pts',(-6.90213804434222,15.1670684973955,-4.46463760236649));
#45288=CARTESIAN_POINT('Ctrl Pts',(-6.90769940804151,15.15623804992,-4.47702577459544));
#45289=CARTESIAN_POINT('Ctrl Pts',(-6.91313475985191,15.1452019823458,-4.48976053775622));
#45290=CARTESIAN_POINT('Ctrl Pts',(-6.91841457854223,15.1339652658698,-4.50284791920425));
#45291=CARTESIAN_POINT('Ctrl Pts',(-6.92704804648557,15.1155911819904,-4.52424817834588));
#45292=CARTESIAN_POINT('Ctrl Pts',(-6.93526620688473,15.096680157031,-4.54659190807374));
#45293=CARTESIAN_POINT('Ctrl Pts',(-6.94294163519944,15.0772610284527,-4.56988881411136));
#45294=CARTESIAN_POINT('Ctrl Pts',(-6.95237987912846,15.0533819086308,-4.5985363205382));
#45295=CARTESIAN_POINT('Ctrl Pts',(-6.96099870124445,15.0287337634886,-4.62862589435581));
#45296=CARTESIAN_POINT('Ctrl Pts',(-6.96853214143094,15.0033880804351,-4.66015381903064));
#45297=CARTESIAN_POINT('Ctrl Pts',(-6.97439397594545,14.9836663867549,-4.68468596801629));
#45298=CARTESIAN_POINT('Ctrl Pts',(-6.97959814083466,14.9635227136263,-4.71008852577051));
#45299=CARTESIAN_POINT('Ctrl Pts',(-6.98400298712196,14.9430003235828,-4.73634858810239));
#45300=CARTESIAN_POINT('Ctrl Pts',(-6.98927533274534,14.9184362125401,-4.76778036021766));
#45301=CARTESIAN_POINT('Ctrl Pts',(-6.9934029386722,14.8933287532684,-4.8004419443322));
#45302=CARTESIAN_POINT('Ctrl Pts',(-6.99614956570734,14.8677747239439,-4.83426271362839));
#45303=CARTESIAN_POINT('Ctrl Pts',(-6.99865578088694,14.8444574350024,-4.86512315602239));
#45304=CARTESIAN_POINT('Ctrl Pts',(-7.00001226509507,14.8207684317736,-4.89694850040556));
#45305=CARTESIAN_POINT('Ctrl Pts',(-7.00001530551468,14.7967990246409,-4.92966193612583));
#45306=CARTESIAN_POINT('Ctrl Pts',(-6.23412736340852,25.6421127780222,-8.85535177831017));
#45307=CARTESIAN_POINT('Ctrl Pts',(-6.23490266413302,25.3447921922583,-8.44426356616765));
#45308=CARTESIAN_POINT('Ctrl Pts',(-6.23649046053314,24.5993917002302,-7.54006523054698));
#45309=CARTESIAN_POINT('Ctrl Pts',(-6.23803731643754,23.2351603117236,-6.30682882468332));
#45310=CARTESIAN_POINT('Ctrl Pts',(-6.23759012311847,21.554594420239,-5.23225230543038));
#45311=CARTESIAN_POINT('Ctrl Pts',(-6.23570095048077,19.7179583713161,-4.44990267765729));
#45312=CARTESIAN_POINT('Ctrl Pts',(-6.23204712515177,17.7794232167923,-3.98190829741467));
#45313=CARTESIAN_POINT('Ctrl Pts',(-6.22725857217666,16.0460302754405,-3.85975908900695));
#45314=CARTESIAN_POINT('Ctrl Pts',(-6.22399902673659,14.9771463891637,-3.92718775185178));
#45315=CARTESIAN_POINT('Ctrl Pts',(-6.22266349997794,14.5714121948162,-3.97374893451381));
#45316=CARTESIAN_POINT('Ctrl Pts',(-6.72598868298147,25.5461091699583,-8.92473325230161));
#45317=CARTESIAN_POINT('Ctrl Pts',(-6.72668184133724,25.2514068069937,-8.5179410961706));
#45318=CARTESIAN_POINT('Ctrl Pts',(-6.72805010629819,24.5127407420923,-7.62319006625967));
#45319=CARTESIAN_POINT('Ctrl Pts',(-6.72941765802146,23.1617892511338,-6.40302838449347));
#45320=CARTESIAN_POINT('Ctrl Pts',(-6.72902265940225,21.4982103197369,-5.33903582949243));
#45321=CARTESIAN_POINT('Ctrl Pts',(-6.72736659887997,19.680427704485,-4.56367388117981));
#45322=CARTESIAN_POINT('Ctrl Pts',(-6.7241629162859,17.7615692934668,-4.09848834078605));
#45323=CARTESIAN_POINT('Ctrl Pts',(-6.71993204305552,16.0451905586601,-3.97507508254132));
#45324=CARTESIAN_POINT('Ctrl Pts',(-6.71707752304265,14.9863207288799,-4.04020996538142));
#45325=CARTESIAN_POINT('Ctrl Pts',(-6.71588880214766,14.5843404536859,-4.08565613536179));
#45326=CARTESIAN_POINT('Ctrl Pts',(-7.02718524992886,25.2169081072125,-9.16264615230095));
#45327=CARTESIAN_POINT('Ctrl Pts',(-7.02756394516156,24.9320808125448,-8.76993740843315));
#45328=CARTESIAN_POINT('Ctrl Pts',(-7.02824885826503,24.218150878117,-7.90599885534894));
#45329=CARTESIAN_POINT('Ctrl Pts',(-7.0289771823686,22.9136335544715,-6.72847731374345));
#45330=CARTESIAN_POINT('Ctrl Pts',(-7.02876725796423,21.3070974217811,-5.70076816462786));
#45331=CARTESIAN_POINT('Ctrl Pts',(-7.02790271803788,19.5522390185827,-4.95159305632285));
#45332=CARTESIAN_POINT('Ctrl Pts',(-7.02622935620566,17.6995251453896,-4.5011314991558));
#45333=CARTESIAN_POINT('Ctrl Pts',(-7.02397932362077,16.0419195973798,-4.38031971054423));
#45334=CARTESIAN_POINT('Ctrl Pts',(-7.02249264002466,15.018878224234,-4.44215006170692));
#45335=CARTESIAN_POINT('Ctrl Pts',(-7.02184968078489,14.6305433081597,-4.4855945803032));
#45336=CARTESIAN_POINT('Ctrl Pts',(-6.99838063092152,24.807947129522,-9.4582014980152));
#45337=CARTESIAN_POINT('Ctrl Pts',(-6.99835913541704,24.5356483926749,-9.08279986617113));
#45338=CARTESIAN_POINT('Ctrl Pts',(-6.99821532761512,23.8529257690149,-8.25667875130623));
#45339=CARTESIAN_POINT('Ctrl Pts',(-6.99814245713621,22.6063536722315,-7.13149025517221));
#45340=CARTESIAN_POINT('Ctrl Pts',(-6.9981642204857,21.0703299742658,-6.14885260427005));
#45341=CARTESIAN_POINT('Ctrl Pts',(-6.99828069521003,19.3931394797008,-5.43285637063545));
#45342=CARTESIAN_POINT('Ctrl Pts',(-6.9985045739756,17.6222095925353,-5.00216737521387));
#45343=CARTESIAN_POINT('Ctrl Pts',(-6.99873523975645,16.0377422523945,-4.88660480595007));
#45344=CARTESIAN_POINT('Ctrl Pts',(-6.99894168369694,15.0596432996674,-4.94565663341864));
#45345=CARTESIAN_POINT('Ctrl Pts',(-6.99898903543767,14.6884846232875,-4.98714443423185));
#45346=CARTESIAN_POINT('',(-7.00000308919871,24.7867179209017,-9.33251796323064));
#45347=CARTESIAN_POINT('Origin',(-5.99998370356801,24.7867138050937,-9.33252808562228));
#45348=CARTESIAN_POINT('Ctrl Pts',(-7.00001101651655,24.7867134185415,-9.33251828871336));
#45349=CARTESIAN_POINT('Ctrl Pts',(-7.00001786888999,24.6735525722877,-9.17932102897506));
#45350=CARTESIAN_POINT('Ctrl Pts',(-7.00001802523188,24.5580143029184,-9.03121154693793));
#45351=CARTESIAN_POINT('Ctrl Pts',(-7.00001556839463,24.4406111277544,-8.88816531793989));
#45352=CARTESIAN_POINT('Ctrl Pts',(-7.00001306417432,24.3209436913995,-8.74236027066983));
#45353=CARTESIAN_POINT('Ctrl Pts',(-7.0000078435676,24.199338696344,-8.60181555932676));
#45354=CARTESIAN_POINT('Ctrl Pts',(-7.00000354839009,24.0762964133774,-8.466471695584));
#45355=CARTESIAN_POINT('Ctrl Pts',(-7.00000225630901,24.0392826682261,-8.42575737234825));
#45356=CARTESIAN_POINT('Ctrl Pts',(-7.00000104345646,24.0021385728783,-8.38551347172416));
#45357=CARTESIAN_POINT('Ctrl Pts',(-6.99999999753986,23.9648770204239,-8.34573781928481));
#45358=CARTESIAN_POINT('Ctrl Pts',(-6.9999988766632,23.9249449603375,-8.30311147554537));
#45359=CARTESIAN_POINT('Ctrl Pts',(-6.9999979469053,23.8848780062048,-8.26102289425667));
#45360=CARTESIAN_POINT('Ctrl Pts',(-6.9999971808686,23.8446913133936,-8.21946684648591));
#45361=CARTESIAN_POINT('Ctrl Pts',(-6.99999462214768,23.7104594524111,-8.08066105687884));
#45362=CARTESIAN_POINT('Ctrl Pts',(-6.99999387751261,23.5748953627083,-7.94779826807436));
#45363=CARTESIAN_POINT('Ctrl Pts',(-6.99999403436151,23.4385317260012,-7.82067003236729));
#45364=CARTESIAN_POINT('Ctrl Pts',(-6.99999406718201,23.409997754318,-7.79406856026382));
#45365=CARTESIAN_POINT('Ctrl Pts',(-6.99999414004824,23.3814286057908,-7.7677181073587));
#45366=CARTESIAN_POINT('Ctrl Pts',(-6.99999424550307,23.3528288963755,-7.74161665661631));
#45367=CARTESIAN_POINT('Ctrl Pts',(-6.99999432423887,23.3314754804659,-7.72212851687852));
#45368=CARTESIAN_POINT('Ctrl Pts',(-6.99999441864844,23.3106151852605,-7.70323911051233));
#45369=CARTESIAN_POINT('Ctrl Pts',(-6.99999453140734,23.2890698406971,-7.68388257740629));
#45370=CARTESIAN_POINT('Ctrl Pts',(-6.99999463683964,23.2689244221075,-7.66578375050118));
#45371=CARTESIAN_POINT('Ctrl Pts',(-6.99999475849122,23.2481799713201,-7.64727658207253));
#45372=CARTESIAN_POINT('Ctrl Pts',(-6.99999490352849,23.2258462288783,-7.62752044062178));
#45373=CARTESIAN_POINT('Ctrl Pts',(-6.99999520368183,23.1796267491328,-7.58663528301742));
#45374=CARTESIAN_POINT('Ctrl Pts',(-6.99999556267854,23.1331494864943,-7.54621522276226));
#45375=CARTESIAN_POINT('Ctrl Pts',(-6.99999595372392,23.0864243015881,-7.5062613627382));
#45376=CARTESIAN_POINT('Ctrl Pts',(-6.99999673581468,22.9929739317757,-7.42635364269007));
#45377=CARTESIAN_POINT('Ctrl Pts',(-6.99999764539602,22.8985318728929,-7.3483107235662));
#45378=CARTESIAN_POINT('Ctrl Pts',(-6.99999847634363,22.8031748666945,-7.27213985850401));
#45379=CARTESIAN_POINT('Ctrl Pts',(-6.99999902467255,22.7402503163646,-7.22187593324709));
#45380=CARTESIAN_POINT('Ctrl Pts',(-6.99999953898535,22.6769273082929,-7.17242715339307));
#45381=CARTESIAN_POINT('Ctrl Pts',(-6.99999996276667,22.6132273489527,-7.12379520528499));
#45382=CARTESIAN_POINT('Ctrl Pts',(-7.00000126736585,22.41712876638,-6.97408308316544));
#45383=CARTESIAN_POINT('Ctrl Pts',(-7.00000171384891,22.217461340655,-6.83211389992002));
#45384=CARTESIAN_POINT('Ctrl Pts',(-7.00000170643164,22.0149178030739,-6.69789294448405));
#45385=CARTESIAN_POINT('Ctrl Pts',(-7.00000169893506,21.8102086021931,-6.56223685366578));
#45386=CARTESIAN_POINT('Ctrl Pts',(-7.00000122941368,21.6025614301284,-6.43449553455437));
#45387=CARTESIAN_POINT('Ctrl Pts',(-7.00000072342701,21.3926444044191,-6.31464932663616));
#45388=CARTESIAN_POINT('Ctrl Pts',(-7.00000046988867,21.2874597908477,-6.25459713684695));
#45389=CARTESIAN_POINT('Ctrl Pts',(-7.00000020716685,21.1817045351281,-6.19652684959421));
#45390=CARTESIAN_POINT('Ctrl Pts',(-6.9999999876654,21.0754583563051,-6.14043370312219));
#45391=CARTESIAN_POINT('Ctrl Pts',(-6.99999993928893,21.0520424943101,-6.12807119379527));
#45392=CARTESIAN_POINT('Ctrl Pts',(-6.99999989300575,21.0286027758283,-6.11580471396694));
#45393=CARTESIAN_POINT('Ctrl Pts',(-6.99999984878329,21.0051400649146,-6.10363406323595));
#45394=CARTESIAN_POINT('Ctrl Pts',(-6.99999965374504,20.9016603977064,-6.04995676686628));
#45395=CARTESIAN_POINT('Ctrl Pts',(-6.999999498637,20.7977336996679,-5.99814355137489));
#45396=CARTESIAN_POINT('Ctrl Pts',(-6.99999938184612,20.6934324619098,-5.94817675977887));
#45397=CARTESIAN_POINT('Ctrl Pts',(-6.99999932345068,20.6412818430308,-5.92319336398087));
#45398=CARTESIAN_POINT('Ctrl Pts',(-6.99999927466585,20.5890375892218,-5.8986715741567));
#45399=CARTESIAN_POINT('Ctrl Pts',(-6.99999923547398,20.5367084691644,-5.87460910041797));
#45400=CARTESIAN_POINT('Ctrl Pts',(-6.99999921587804,20.5105439091356,-5.86257786354861));
#45401=CARTESIAN_POINT('Ctrl Pts',(-6.99999919868237,20.4843581325447,-5.8506614557006));
#45402=CARTESIAN_POINT('Ctrl Pts',(-6.99999918389672,20.4581522268333,-5.83885958823657));
#45403=CARTESIAN_POINT('Ctrl Pts',(-6.9999991728316,20.4385405337695,-5.83002743395683));
#45404=CARTESIAN_POINT('Ctrl Pts',(-6.99999916268855,20.4179923363439,-5.82084769630923));
#45405=CARTESIAN_POINT('Ctrl Pts',(-6.99999915446007,20.3985848805957,-5.81224565595625));
#45406=CARTESIAN_POINT('Ctrl Pts',(-6.99999915169334,20.3920593404632,-5.80935331600849));
#45407=CARTESIAN_POINT('Ctrl Pts',(-6.99999914913303,20.3856629518266,-5.80652587657329));
#45408=CARTESIAN_POINT('Ctrl Pts',(-6.99999914678765,20.3794752048421,-5.80379731697459));
#45409=CARTESIAN_POINT('Ctrl Pts',(-6.99999907529436,20.1908565103081,-5.72062369162249));
#45410=CARTESIAN_POINT('Ctrl Pts',(-6.99999912491866,19.997467426613,-5.64168479882575));
#45411=CARTESIAN_POINT('Ctrl Pts',(-6.99999933315965,19.7994484267587,-5.56752045890149));
#45412=CARTESIAN_POINT('Ctrl Pts',(-6.99999947285736,19.6666081079875,-5.51776758385295));
#45413=CARTESIAN_POINT('Ctrl Pts',(-6.99999968443231,19.5316850177846,-5.47016399769346));
#45414=CARTESIAN_POINT('Ctrl Pts',(-6.99999998816762,19.3947326008755,-5.42487991153454));
#45415=CARTESIAN_POINT('Ctrl Pts',(-7.00000042903658,19.1959474430728,-5.3591504821735));
#45416=CARTESIAN_POINT('Ctrl Pts',(-7.00000106780694,18.9928846417257,-5.29830694871975));
#45417=CARTESIAN_POINT('Ctrl Pts',(-7.00000153331201,18.7857670354442,-5.2428642781925));
#45418=CARTESIAN_POINT('Ctrl Pts',(-7.00000199134807,18.5819726260479,-5.18831118394662));
#45419=CARTESIAN_POINT('Ctrl Pts',(-7.0000022813202,18.3742524289665,-5.13898704366274));
#45420=CARTESIAN_POINT('Ctrl Pts',(-7.0000020266282,18.1628635746473,-5.0954046588484));
#45421=CARTESIAN_POINT('Ctrl Pts',(-7.00000181209342,17.9848043394636,-5.05869389596303));
#45422=CARTESIAN_POINT('Ctrl Pts',(-7.00000121063125,17.8041428262805,-5.02605738962653));
#45423=CARTESIAN_POINT('Ctrl Pts',(-6.99999998662421,17.6210585944206,-4.99781411446671));
#45424=CARTESIAN_POINT('Ctrl Pts',(-6.99999852881455,17.4030026883872,-4.96417597484234));
#45425=CARTESIAN_POINT('Ctrl Pts',(-6.99999617286851,17.1815088161742,-4.93677017707439));
#45426=CARTESIAN_POINT('Ctrl Pts',(-6.99999449845778,16.9569202000096,-4.91605392211338));
#45427=CARTESIAN_POINT('Ctrl Pts',(-6.99999284826951,16.7355805405395,-4.89563735382567));
#45428=CARTESIAN_POINT('Ctrl Pts',(-6.99999186158928,16.5112349764961,-4.88171820714913));
#45429=CARTESIAN_POINT('Ctrl Pts',(-6.99999320068089,16.2842613693983,-4.8747443371105));
#45430=CARTESIAN_POINT('Ctrl Pts',(-6.9999941339609,16.126072094649,-4.86988389779461));
#45431=CARTESIAN_POINT('Ctrl Pts',(-6.99999620011936,15.9666072927035,-4.86839726412075));
#45432=CARTESIAN_POINT('Ctrl Pts',(-6.99999999965512,15.80600961461,-4.87043896575524));
#45433=CARTESIAN_POINT('Ctrl Pts',(-7.00000506883584,15.5917469503153,-4.87316291816286));
#45434=CARTESIAN_POINT('Ctrl Pts',(-7.00001329849009,15.3754653810258,-4.88216722490851));
#45435=CARTESIAN_POINT('Ctrl Pts',(-7.00001657716831,15.1576281619852,-4.89779630238528));
#45436=CARTESIAN_POINT('Ctrl Pts',(-7.00001838080227,15.037793710345,-4.90639401556449));
#45437=CARTESIAN_POINT('Ctrl Pts',(-7.00001867122265,14.9174893804563,-4.91699659995693));
#45438=CARTESIAN_POINT('Ctrl Pts',(-7.00001598720761,14.7967990242442,-4.92966193645403));
#45439=CARTESIAN_POINT('Origin',(-5.999994980806,24.7867195890732,-9.33250914740904));
#45440=CARTESIAN_POINT('Origin',(-6.,24.7867243677925,-9.33251101143268));
#45441=CARTESIAN_POINT('Ctrl Pts',(-7.1043551019301,14.3540695603781,-7.16139801889706));
#45442=CARTESIAN_POINT('Ctrl Pts',(-7.10505840364598,14.3262466614253,-7.2166440006466));
#45443=CARTESIAN_POINT('Ctrl Pts',(-7.09599870842687,14.250813032227,-7.37231361286277));
#45444=CARTESIAN_POINT('Ctrl Pts',(-7.02992031322268,14.1377144382614,-7.63343902919195));
#45445=CARTESIAN_POINT('Ctrl Pts',(-6.87962835847259,14.0336429995058,-7.92131943416508));
#45446=CARTESIAN_POINT('Ctrl Pts',(-6.66675658014908,13.9662230204584,-8.17059025983369));
#45447=CARTESIAN_POINT('Ctrl Pts',(-6.44849849026614,13.9438645604057,-8.33481728798434));
#45448=CARTESIAN_POINT('Ctrl Pts',(-6.30562810957406,13.9470394167763,-8.40803755460183));
#45449=CARTESIAN_POINT('Ctrl Pts',(-6.25403108440681,13.9502324530738,-8.43056626115595));
#45450=CARTESIAN_POINT('Ctrl Pts',(-6.81769315740398,13.8371643132692,-6.90501019096244));
#45451=CARTESIAN_POINT('Ctrl Pts',(-6.81832491766206,13.8126035966522,-6.95375927642177));
#45452=CARTESIAN_POINT('Ctrl Pts',(-6.81018068214544,13.7460176756343,-7.09142431241616));
#45453=CARTESIAN_POINT('Ctrl Pts',(-6.75054164470443,13.6465473839494,-7.32312337578426));
#45454=CARTESIAN_POINT('Ctrl Pts',(-6.61500606191396,13.5560338595191,-7.57861801524689));
#45455=CARTESIAN_POINT('Ctrl Pts',(-6.42374559388827,13.4986449647106,-7.79929848485672));
#45456=CARTESIAN_POINT('Ctrl Pts',(-6.2287190790081,13.4808603575806,-7.94407139582291));
#45457=CARTESIAN_POINT('Ctrl Pts',(-6.10176442006207,13.4845982242126,-8.00837466920298));
#45458=CARTESIAN_POINT('Ctrl Pts',(-6.05601366185832,13.4876931636193,-8.02813942562704));
#45459=CARTESIAN_POINT('Ctrl Pts',(-7.05994136368923,13.3052082606372,-6.63417610553049));
#45460=CARTESIAN_POINT('Ctrl Pts',(-7.06077434405811,13.2734780527966,-6.69718330261341));
#45461=CARTESIAN_POINT('Ctrl Pts',(-7.05006316137364,13.1877446689244,-6.87408086960113));
#45462=CARTESIAN_POINT('Ctrl Pts',(-6.9726777229904,13.0596165904912,-7.16954064266108));
#45463=CARTESIAN_POINT('Ctrl Pts',(-6.79632560572774,12.9411861766716,-7.4964228042818));
#45464=CARTESIAN_POINT('Ctrl Pts',(-6.5443353497334,12.8637753759665,-7.78232843918036));
#45465=CARTESIAN_POINT('Ctrl Pts',(-6.28263461591015,12.8380285719052,-7.97358623594707));
#45466=CARTESIAN_POINT('Ctrl Pts',(-6.10912624217055,12.8422479165076,-8.0601704519397));
#45467=CARTESIAN_POINT('Ctrl Pts',(-6.04615886818837,12.8462520261003,-8.08697139379655));
#45468=CARTESIAN_POINT('Ctrl Pts',(-7.66740328026631,13.1170710760981,-6.53161011949029));
#45469=CARTESIAN_POINT('Ctrl Pts',(-7.66857435637506,13.0725817013203,-6.62000105264184));
#45470=CARTESIAN_POINT('Ctrl Pts',(-7.65354730602362,12.952637211568,-6.86687204017496));
#45471=CARTESIAN_POINT('Ctrl Pts',(-7.54621409601368,12.7729199260003,-7.2762178468624));
#45472=CARTESIAN_POINT('Ctrl Pts',(-7.30103647553656,12.6039522523028,-7.73004848906578));
#45473=CARTESIAN_POINT('Ctrl Pts',(-6.94698677236901,12.4899890553448,-8.13094481283146));
#45474=CARTESIAN_POINT('Ctrl Pts',(-6.5737315426479,12.4491218575515,-8.40323327799303));
#45475=CARTESIAN_POINT('Ctrl Pts',(-6.32263787429271,12.45341638109,-8.5282493153534));
#45476=CARTESIAN_POINT('Ctrl Pts',(-6.23101741108753,12.4587230728515,-8.56713483649188));
#45477=CARTESIAN_POINT('',(-6.26386059966982,13.9442583573344,-8.42071137120996));
#45478=CARTESIAN_POINT('',(-6.24994560412829,12.4626529248953,-8.55169129771482));
#45479=CARTESIAN_POINT('Ctrl Pts',(-6.26385531438063,13.9442721684155,-8.42069786050422));
#45480=CARTESIAN_POINT('Ctrl Pts',(-6.25431876900276,13.9218692534565,-8.40152732455114));
#45481=CARTESIAN_POINT('Ctrl Pts',(-6.24496566034452,13.898005006553,-8.38292933852713));
#45482=CARTESIAN_POINT('Ctrl Pts',(-6.23589696786197,13.8726957646131,-8.36513250150588));
#45483=CARTESIAN_POINT('Ctrl Pts',(-6.22705466583233,13.8480183415111,-8.34777994396607));
#45484=CARTESIAN_POINT('Ctrl Pts',(-6.2184830520658,13.8219669051049,-8.33118973070111));
#45485=CARTESIAN_POINT('Ctrl Pts',(-6.21028187793343,13.7946047513556,-8.31558229425693));
#45486=CARTESIAN_POINT('Ctrl Pts',(-6.20220717037243,13.7676645369181,-8.3002155329823));
#45487=CARTESIAN_POINT('Ctrl Pts',(-6.19449189366985,13.7394535982295,-8.28580222594987));
#45488=CARTESIAN_POINT('Ctrl Pts',(-6.18723271225038,13.7100825577268,-8.2725504751593));
#45489=CARTESIAN_POINT('Ctrl Pts',(-6.18010114805958,13.6812278634311,-8.25953169164331));
#45490=CARTESIAN_POINT('Ctrl Pts',(-6.1734101242466,13.6512536412055,-8.24763473584261));
#45491=CARTESIAN_POINT('Ctrl Pts',(-6.16724777116303,13.6203134060684,-8.23704356365176));
#45492=CARTESIAN_POINT('Ctrl Pts',(-6.16645167093337,13.6163163082124,-8.23567531446202));
#45493=CARTESIAN_POINT('Ctrl Pts',(-6.16566438487322,13.6123031533829,-8.23432883038793));
#45494=CARTESIAN_POINT('Ctrl Pts',(-6.16488609396448,13.6082743301702,-8.2330044812538));
#45495=CARTESIAN_POINT('Ctrl Pts',(-6.15895413328033,13.5775675332214,-8.22291058588955));
#45496=CARTESIAN_POINT('Ctrl Pts',(-6.15354561085793,13.5459472765254,-8.21410500969514));
#45497=CARTESIAN_POINT('Ctrl Pts',(-6.14873512281968,13.5136094010613,-8.20673556407136));
#45498=CARTESIAN_POINT('Ctrl Pts',(-6.14398626259485,13.4816858104971,-8.19946052941302));
#45499=CARTESIAN_POINT('Ctrl Pts',(-6.13982048464334,13.4490634552977,-8.19358561892249));
#45500=CARTESIAN_POINT('Ctrl Pts',(-6.13629629272268,13.4159660304879,-8.1892190615961));
#45501=CARTESIAN_POINT('Ctrl Pts',(-6.13279279596087,13.3830629641238,-8.18487814606208));
#45502=CARTESIAN_POINT('Ctrl Pts',(-6.12992359196701,13.3496911104767,-8.18202834059126));
#45503=CARTESIAN_POINT('Ctrl Pts',(-6.12772926495945,13.3160956606706,-8.18073484260766));
#45504=CARTESIAN_POINT('Ctrl Pts',(-6.12554238394843,13.2826142101007,-8.17944573384293));
#45505=CARTESIAN_POINT('Ctrl Pts',(-6.12402594639205,13.2489115085795,-8.17970261237211));
#45506=CARTESIAN_POINT('Ctrl Pts',(-6.12320058978627,13.2152439538066,-8.18152417251487));
#45507=CARTESIAN_POINT('Ctrl Pts',(-6.12237597635794,13.181606714375,-8.18334409246671));
#45508=CARTESIAN_POINT('Ctrl Pts',(-6.12224124458969,13.1480054342186,-8.18672588281752));
#45509=CARTESIAN_POINT('Ctrl Pts',(-6.12279604741047,13.1146966651274,-8.19164059249816));
#45510=CARTESIAN_POINT('Ctrl Pts',(-6.12335355350003,13.081225599537,-8.19657924903116));
#45511=CARTESIAN_POINT('Ctrl Pts',(-6.12460728679828,13.048050768882,-8.20306560627659));
#45512=CARTESIAN_POINT('Ctrl Pts',(-6.12653570663021,13.0154201453311,-8.21102355208262));
#45513=CARTESIAN_POINT('Ctrl Pts',(-6.12847158715998,12.9826632799634,-8.21901228570164));
#45514=CARTESIAN_POINT('Ctrl Pts',(-6.13108723330755,12.9504556062705,-8.22848358864234));
#45515=CARTESIAN_POINT('Ctrl Pts',(-6.13434103434159,12.9190231830349,-8.23931820150807));
#45516=CARTESIAN_POINT('Ctrl Pts',(-6.13763222177764,12.8872295990525,-8.25027730483523));
#45517=CARTESIAN_POINT('Ctrl Pts',(-6.14157609014089,12.8562298310844,-8.26263064964509));
#45518=CARTESIAN_POINT('Ctrl Pts',(-6.14611215712109,12.8262216470255,-8.2762192495679));
#45519=CARTESIAN_POINT('Ctrl Pts',(-6.14941594017699,12.8043655918867,-8.28611632259929));
#45520=CARTESIAN_POINT('Ctrl Pts',(-6.15303348114506,12.7830347782143,-8.29666786989227));
#45521=CARTESIAN_POINT('Ctrl Pts',(-6.15693687422531,12.7622912696509,-8.30780374079499));
#45522=CARTESIAN_POINT('Ctrl Pts',(-6.16239173227345,12.7333029273786,-8.32336573872032));
#45523=CARTESIAN_POINT('Ctrl Pts',(-6.16840510191083,12.7054636338093,-8.34006900844475));
#45524=CARTESIAN_POINT('Ctrl Pts',(-6.17489262861964,12.6789001914872,-8.35770723169384));
#45525=CARTESIAN_POINT('Ctrl Pts',(-6.18152856588358,12.6517290761028,-8.37574895208775));
#45526=CARTESIAN_POINT('Ctrl Pts',(-6.18866024944796,12.6258929457347,-8.39476808136235));
#45527=CARTESIAN_POINT('Ctrl Pts',(-6.19619197334983,12.6014736028412,-8.41453721976038));
#45528=CARTESIAN_POINT('Ctrl Pts',(-6.20383525725669,12.5766925602823,-8.43459917892654));
#45529=CARTESIAN_POINT('Ctrl Pts',(-6.21189016673278,12.5533703503877,-8.45543275336067));
#45530=CARTESIAN_POINT('Ctrl Pts',(-6.22025661292607,12.5315387851256,-8.47680583653422));
#45531=CARTESIAN_POINT('Ctrl Pts',(-6.22882371433385,12.509183626296,-8.4986915173495));
#45532=CARTESIAN_POINT('Ctrl Pts',(-6.23771714857315,12.488391076784,-8.52114219668428));
#45533=CARTESIAN_POINT('Ctrl Pts',(-6.24683464861735,12.4691441717878,-8.54392588646561));
#45534=CARTESIAN_POINT('Ctrl Pts',(-6.24786889296593,12.4669608975763,-8.54651035614283));
#45535=CARTESIAN_POINT('Ctrl Pts',(-6.24890602880747,12.4647974632093,-8.54909913490104));
#45536=CARTESIAN_POINT('Ctrl Pts',(-6.24994591367904,12.4626538076691,-8.55169190342477));
#45537=CARTESIAN_POINT('',(-6.99999993308851,12.5220609673846,-8.04448262432736));
#45538=CARTESIAN_POINT('Ctrl Pts',(-6.99999979926552,12.522060623473,-8.04448240338846));
#45539=CARTESIAN_POINT('Ctrl Pts',(-6.97542285739824,12.5160357668641,-8.06874693229243));
#45540=CARTESIAN_POINT('Ctrl Pts',(-6.95040800356331,12.5104440175142,-8.092411446419));
#45541=CARTESIAN_POINT('Ctrl Pts',(-6.92495762901603,12.5052794586727,-8.11549292092594));
#45542=CARTESIAN_POINT('Ctrl Pts',(-6.88589911077916,12.4973534450368,-8.1509159042415));
#45543=CARTESIAN_POINT('Ctrl Pts',(-6.84581661617226,12.4904323745383,-8.18496704826789));
#45544=CARTESIAN_POINT('Ctrl Pts',(-6.80471668547353,12.4845032510779,-8.21769224628849));
#45545=CARTESIAN_POINT('Ctrl Pts',(-6.79363454055424,12.4829045280554,-8.2265162365194));
#45546=CARTESIAN_POINT('Ctrl Pts',(-6.78247820901056,12.4813780594646,-8.23524367399069));
#45547=CARTESIAN_POINT('Ctrl Pts',(-6.77124736772588,12.4799238936921,-8.24387511076992));
#45548=CARTESIAN_POINT('Ctrl Pts',(-6.70998521883027,12.4719916900564,-8.29095799189599));
#45549=CARTESIAN_POINT('Ctrl Pts',(-6.6465178674323,12.4661981270724,-8.33519774227364));
#45550=CARTESIAN_POINT('Ctrl Pts',(-6.5811239193887,12.4625979661439,-8.37641200247287));
#45551=CARTESIAN_POINT('Ctrl Pts',(-6.56109760139874,12.4614954487134,-8.38903350499969));
#45552=CARTESIAN_POINT('Ctrl Pts',(-6.5408902874965,12.4605987859764,-8.4013711331731));
#45553=CARTESIAN_POINT('Ctrl Pts',(-6.52050919424535,12.4599099639518,-8.41341925274955));
#45554=CARTESIAN_POINT('Ctrl Pts',(-6.51186917965474,12.4596179564393,-8.41852672797903));
#45555=CARTESIAN_POINT('Ctrl Pts',(-6.50319799142138,12.459363514444,-8.42358182730049));
#45556=CARTESIAN_POINT('Ctrl Pts',(-6.49449523374268,12.4591467968089,-8.42858461341113));
#45557=CARTESIAN_POINT('Ctrl Pts',(-6.45012191074507,12.4580418043481,-8.45409264801016));
#45558=CARTESIAN_POINT('Ctrl Pts',(-6.40492956497043,12.4579153804756,-8.47824371821814));
#45559=CARTESIAN_POINT('Ctrl Pts',(-6.35888373115315,12.458787611434,-8.50103476438739));
#45560=CARTESIAN_POINT('Ctrl Pts',(-6.32309503968703,12.4594655447467,-8.51874889076804));
#45561=CARTESIAN_POINT('Ctrl Pts',(-6.28679018132058,12.4607472817652,-8.53564077229362));
#45562=CARTESIAN_POINT('Ctrl Pts',(-6.24994591368686,12.462653807653,-8.55169190344427));
#45563=CARTESIAN_POINT('',(-7.00000699063831,13.9486956645825,-6.97707644718775));
#45564=CARTESIAN_POINT('Ctrl Pts',(-7.00000699063831,13.9486956645825,-6.97707644718775));
#45565=CARTESIAN_POINT('Ctrl Pts',(-7.00000696201984,13.9388631272801,-6.98132934556522));
#45566=CARTESIAN_POINT('Ctrl Pts',(-6.99999999999998,13.8939388286958,-7.00116680182805));
#45567=CARTESIAN_POINT('Ctrl Pts',(-6.99999999999998,13.7156828472741,-7.08002168518265));
#45568=CARTESIAN_POINT('Ctrl Pts',(-7.,13.390887431638,-7.2290274543114));
#45569=CARTESIAN_POINT('Ctrl Pts',(-7.,12.8079631824901,-7.66311431918244));
#45570=CARTESIAN_POINT('Ctrl Pts',(-7.,12.6357805654568,-7.86746450612831));
#45571=CARTESIAN_POINT('Ctrl Pts',(-7.,12.5220605681818,-8.04448236787108));
#45572=CARTESIAN_POINT('Ctrl Pts',(-7.00000698845854,13.9487142985806,-6.97711952785195));
#45573=CARTESIAN_POINT('Ctrl Pts',(-7.00000440247537,13.9417124577176,-7.02271343158893));
#45574=CARTESIAN_POINT('Ctrl Pts',(-6.9982617039689,13.9352233858386,-7.06743899796608));
#45575=CARTESIAN_POINT('Ctrl Pts',(-6.99501560109673,13.9292493585815,-7.11111644741427));
#45576=CARTESIAN_POINT('Ctrl Pts',(-6.99400447902474,13.927388520815,-7.12472144852615));
#45577=CARTESIAN_POINT('Ctrl Pts',(-6.99284724471071,13.9255776194665,-7.1382250551963));
#45578=CARTESIAN_POINT('Ctrl Pts',(-6.99155043900581,13.9238166198075,-7.15162262632134));
#45579=CARTESIAN_POINT('Ctrl Pts',(-6.98721566830246,13.9179302100688,-7.19640604961227));
#45580=CARTESIAN_POINT('Ctrl Pts',(-6.98132457884879,13.9126014783713,-7.2400021018724));
#45581=CARTESIAN_POINT('Ctrl Pts',(-6.97415403051326,13.9078036282271,-7.28229317583046));
#45582=CARTESIAN_POINT('Ctrl Pts',(-6.96663085873588,13.9027698359551,-7.32666398251757));
#45583=CARTESIAN_POINT('Ctrl Pts',(-6.95769892916249,13.8983205261988,-7.36959827165777));
#45584=CARTESIAN_POINT('Ctrl Pts',(-6.94763652196407,13.8944217247386,-7.41099935405376));
#45585=CARTESIAN_POINT('Ctrl Pts',(-6.9449082656302,13.8933646288003,-7.42222457710907));
#45586=CARTESIAN_POINT('Ctrl Pts',(-6.94209669584886,13.8923479811363,-7.43333730319684));
#45587=CARTESIAN_POINT('Ctrl Pts',(-6.93920691998523,13.891371053529,-7.4443360722963));
#45588=CARTESIAN_POINT('Ctrl Pts',(-6.93549800688392,13.8901172055586,-7.45845255770426));
#45589=CARTESIAN_POINT('Ctrl Pts',(-6.93166027951993,13.8889287888692,-7.47238130999926));
#45590=CARTESIAN_POINT('Ctrl Pts',(-6.92770413969251,13.8878042041527,-7.48611969781178));
#45591=CARTESIAN_POINT('Ctrl Pts',(-6.91583249176674,13.8844295322757,-7.52734607258448));
#45592=CARTESIAN_POINT('Ctrl Pts',(-6.90289794786343,13.8816295401607,-7.56685615963965));
#45593=CARTESIAN_POINT('Ctrl Pts',(-6.88919659010306,13.8793390685756,-7.60462800461149));
#45594=CARTESIAN_POINT('Ctrl Pts',(-6.87483949860464,13.8769389772345,-7.64420757357169));
#45595=CARTESIAN_POINT('Ctrl Pts',(-6.85964015705107,13.8750984351494,-7.68187857528357));
#45596=CARTESIAN_POINT('Ctrl Pts',(-6.84389294039583,13.8737425403749,-7.71764776642021));
#45597=CARTESIAN_POINT('Ctrl Pts',(-6.84271076881642,13.8736407509411,-7.72033302325676));
#45598=CARTESIAN_POINT('Ctrl Pts',(-6.84152549002593,13.8735416925283,-7.72300757600783));
#45599=CARTESIAN_POINT('Ctrl Pts',(-6.84033721930421,13.8734453332486,-7.72567143426748));
#45600=CARTESIAN_POINT('Ctrl Pts',(-6.83414454227264,13.8729431565244,-7.73955414092537));
#45601=CARTESIAN_POINT('Ctrl Pts',(-6.82787067434591,13.872514290194,-7.75314633620957));
#45602=CARTESIAN_POINT('Ctrl Pts',(-6.82153140754412,13.8721542004677,-7.76644977163411));
#45603=CARTESIAN_POINT('Ctrl Pts',(-6.81836177414322,13.8719741556045,-7.77310148934638));
#45604=CARTESIAN_POINT('Ctrl Pts',(-6.81517578531874,13.8718113078776,-7.77968101442203));
#45605=CARTESIAN_POINT('Ctrl Pts',(-6.81197532766753,13.8716650831134,-7.78618863946136));
#45606=CARTESIAN_POINT('Ctrl Pts',(-6.81037509884193,13.8715919707312,-7.78944245198102));
#45607=CARTESIAN_POINT('Ctrl Pts',(-6.80877125245983,13.8715230142659,-7.79267828933442));
#45608=CARTESIAN_POINT('Ctrl Pts',(-6.80716402087194,13.8714581422824,-7.79589618956667));
#45609=CARTESIAN_POINT('Ctrl Pts',(-6.80578119710739,13.8714023279733,-7.79866479425727));
#45610=CARTESIAN_POINT('Ctrl Pts',(-6.80477551129168,13.8713635671486,-7.80066840713703));
#45611=CARTESIAN_POINT('Ctrl Pts',(-6.80316743052006,13.8713054813963,-7.80384746390922));
#45612=CARTESIAN_POINT('Ctrl Pts',(-6.80290646747114,13.8712960551067,-7.80436336855941));
#45613=CARTESIAN_POINT('Ctrl Pts',(-6.80262955743476,13.871286162908,-7.80491017874213));
#45614=CARTESIAN_POINT('Ctrl Pts',(-6.80233240072437,13.8712757085966,-7.80549611779183));
#45615=CARTESIAN_POINT('Ctrl Pts',(-6.80117192980019,13.8712348819082,-7.80778435563652));
#45616=CARTESIAN_POINT('Ctrl Pts',(-6.80000721951744,13.8711961246117,-7.81006857574347));
#45617=CARTESIAN_POINT('Ctrl Pts',(-6.7988382919471,13.8711594425164,-7.81234875510117));
#45618=CARTESIAN_POINT('Ctrl Pts',(-6.76921159976319,13.8702297278157,-7.87014033575078));
#45619=CARTESIAN_POINT('Ctrl Pts',(-6.73688041703603,13.8706311177965,-7.92533559663938));
#45620=CARTESIAN_POINT('Ctrl Pts',(-6.70230805444698,13.8723877950923,-7.9776628787557));
#45621=CARTESIAN_POINT('Ctrl Pts',(-6.67499636244358,13.8737755460488,-8.0190007135321));
#45622=CARTESIAN_POINT('Ctrl Pts',(-6.64628463556096,13.8760097247121,-8.05854875323045));
#45623=CARTESIAN_POINT('Ctrl Pts',(-6.61638074962212,13.8791106998596,-8.09617745463876));
#45624=CARTESIAN_POINT('Ctrl Pts',(-6.57642476260087,13.8832540584519,-8.14645493055517));
#45625=CARTESIAN_POINT('Ctrl Pts',(-6.53434261580545,13.8889438259581,-8.19330604016633));
#45626=CARTESIAN_POINT('Ctrl Pts',(-6.49070743375913,13.8961521103861,-8.23654095029581));
#45627=CARTESIAN_POINT('Ctrl Pts',(-6.45843664964803,13.9014830607725,-8.26851570977706));
#45628=CARTESIAN_POINT('Ctrl Pts',(-6.42531520566761,13.9076451739511,-8.29851261540396));
#45629=CARTESIAN_POINT('Ctrl Pts',(-6.39155836829281,13.9146333113849,-8.32645867036084));
#45630=CARTESIAN_POINT('Ctrl Pts',(-6.3498114974705,13.9232754974849,-8.36101938270853));
#45631=CARTESIAN_POINT('Ctrl Pts',(-6.30709401505599,13.9331804020228,-8.39244392968853));
#45632=CARTESIAN_POINT('Ctrl Pts',(-6.26385531438063,13.9442721684154,-8.42069786050422));
#45633=CARTESIAN_POINT('Ctrl Pts',(-6.2226671525855,13.113406883036,-7.49367536133247));
#45634=CARTESIAN_POINT('Ctrl Pts',(-6.22400268361015,13.3673812776541,-7.81349762199499));
#45635=CARTESIAN_POINT('Ctrl Pts',(-6.22726226983453,14.0755184331267,-8.61699371744871));
#45636=CARTESIAN_POINT('Ctrl Pts',(-6.23205080008166,15.3875854737378,-9.75631552861892));
#45637=CARTESIAN_POINT('Ctrl Pts',(-6.23570462908324,17.0892588497341,-10.7961449380645));
#45638=CARTESIAN_POINT('Ctrl Pts',(-6.23759379811576,18.9411612581294,-11.5416379309798));
#45639=CARTESIAN_POINT('Ctrl Pts',(-6.23804099158829,20.889340946093,-11.9701370898467));
#45640=CARTESIAN_POINT('Ctrl Pts',(-6.23649414006684,22.7260240230269,-12.0627643382486));
#45641=CARTESIAN_POINT('Ctrl Pts',(-6.2349063534325,23.8924620138941,-11.950478265913));
#45642=CARTESIAN_POINT('Ctrl Pts',(-6.23413106088457,24.393378813603,-11.8700335727714));
#45643=CARTESIAN_POINT('Ctrl Pts',(-6.71588969012869,13.2016799428778,-7.42368590845217));
#45644=CARTESIAN_POINT('Ctrl Pts',(-6.71707840875763,13.4537883131605,-7.74006526921503));
#45645=CARTESIAN_POINT('Ctrl Pts',(-6.71993293840253,14.1564663174282,-8.53485828384865));
#45646=CARTESIAN_POINT('Ctrl Pts',(-6.72416379703351,15.4573961547951,-9.66125530951553));
#45647=CARTESIAN_POINT('Ctrl Pts',(-6.72736747360088,17.1431696324249,-10.6891572004536));
#45648=CARTESIAN_POINT('Ctrl Pts',(-6.7290235300564,18.9767994120935,-11.4262597642551));
#45649=CARTESIAN_POINT('Ctrl Pts',(-6.72941852491458,20.9054833059166,-11.8502312766459));
#45650=CARTESIAN_POINT('Ctrl Pts',(-6.72805098959961,22.7235306892769,-11.9427134310675));
#45651=CARTESIAN_POINT('Ctrl Pts',(-6.7266827144802,23.8785263901091,-11.8323456482745));
#45652=CARTESIAN_POINT('Ctrl Pts',(-6.72598956820625,24.3745540375429,-11.7530873535714));
#45653=CARTESIAN_POINT('Ctrl Pts',(-7.02184866845526,13.5171483052377,-7.17355825144612));
#45654=CARTESIAN_POINT('Ctrl Pts',(-7.02249162233139,13.7610233403838,-7.47887351087227));
#45655=CARTESIAN_POINT('Ctrl Pts',(-7.02397828640646,14.4407034652188,-8.24599533105423));
#45656=CARTESIAN_POINT('Ctrl Pts',(-7.02622832975696,15.698235042491,-9.33267312724308));
#45657=CARTESIAN_POINT('Ctrl Pts',(-7.02790168586848,17.3268260635882,-10.3242153344646));
#45658=CARTESIAN_POINT('Ctrl Pts',(-7.02876622716094,19.0974450740525,-11.0353407644723));
#45659=CARTESIAN_POINT('Ctrl Pts',(-7.02897614585137,20.9601376524492,-11.4446332304759));
#45660=CARTESIAN_POINT('Ctrl Pts',(-7.02824784215516,22.7152003710236,-11.5344326158821));
#45661=CARTESIAN_POINT('Ctrl Pts',(-7.02756289660507,23.8309176062701,-11.4283614102117));
#45662=CARTESIAN_POINT('Ctrl Pts',(-7.02718421187953,24.3100042451047,-11.352078808438));
#45663=CARTESIAN_POINT('Ctrl Pts',(-6.99898915854136,13.9127665113907,-6.85988137561707));
#45664=CARTESIAN_POINT('Ctrl Pts',(-6.9989418013608,14.1458797420746,-7.15166760754954));
#45665=CARTESIAN_POINT('Ctrl Pts',(-6.99873531963908,14.7957455165646,-7.88504566691922));
#45666=CARTESIAN_POINT('Ctrl Pts',(-6.99850468870856,15.9978490959828,-8.92371893442041));
#45667=CARTESIAN_POINT('Ctrl Pts',(-6.99828080917683,17.5546291317113,-9.87141264151665));
#45668=CARTESIAN_POINT('Ctrl Pts',(-6.99816434192788,19.2468680171176,-10.5510797293928));
#45669=CARTESIAN_POINT('Ctrl Pts',(-6.99814257314777,21.0278308193474,-10.9423828250013));
#45670=CARTESIAN_POINT('Ctrl Pts',(-6.99821546033242,22.7049155574539,-11.0282138250255));
#45671=CARTESIAN_POINT('Ctrl Pts',(-6.99835922371807,23.7718253763724,-10.9268166310602));
#45672=CARTESIAN_POINT('Ctrl Pts',(-6.99838072447693,24.2298152718707,-10.8539129111309));
#45673=CARTESIAN_POINT('',(-7.00000355772629,24.1259406808705,-10.9277699389936));
#45674=CARTESIAN_POINT('Ctrl Pts',(-7.00001601631083,13.9487142982008,-6.97711952796313));
#45675=CARTESIAN_POINT('Ctrl Pts',(-7.00002088955871,14.0875642651609,-7.14852826728832));
#45676=CARTESIAN_POINT('Ctrl Pts',(-7.00001598262134,14.2303296025025,-7.31421367370573));
#45677=CARTESIAN_POINT('Ctrl Pts',(-7.00000988115996,14.3764173564029,-7.47407309340898));
#45678=CARTESIAN_POINT('Ctrl Pts',(-7.00000652438907,14.4567887769833,-7.56202111308673));
#45679=CARTESIAN_POINT('Ctrl Pts',(-7.00000279083418,14.5381665194036,-7.6482063638788));
#45680=CARTESIAN_POINT('Ctrl Pts',(-6.9999999996556,14.6204569538272,-7.7326160850522));
#45681=CARTESIAN_POINT('Ctrl Pts',(-6.99999455429067,14.7809989736415,-7.89729266288357));
#45682=CARTESIAN_POINT('Ctrl Pts',(-6.99999266088662,14.945012257854,-8.0552099081169));
#45683=CARTESIAN_POINT('Ctrl Pts',(-6.99999257352113,15.1118864367878,-8.20639691426214));
#45684=CARTESIAN_POINT('Ctrl Pts',(-6.99999248489059,15.2811769408462,-8.35977309649074));
#45685=CARTESIAN_POINT('Ctrl Pts',(-6.99999425322475,15.4534118096271,-8.50622277538367));
#45686=CARTESIAN_POINT('Ctrl Pts',(-6.99999619758536,15.6279986773723,-8.64580626644339));
#45687=CARTESIAN_POINT('Ctrl Pts',(-6.9999975442495,15.7489175403573,-8.74248179105995));
#45688=CARTESIAN_POINT('Ctrl Pts',(-6.99999897835629,15.8709655864557,-8.83586426951038));
#45689=CARTESIAN_POINT('Ctrl Pts',(-6.99999998662344,15.9939582392987,-8.92598173680061));
#45690=CARTESIAN_POINT('Ctrl Pts',(-7.00000143707747,16.1708906990695,-9.05562122978986));
#45691=CARTESIAN_POINT('Ctrl Pts',(-7.00000201440485,16.3497755095874,-9.17850353424194));
#45692=CARTESIAN_POINT('Ctrl Pts',(-7.00000210874344,16.5300313646543,-9.29479362824702));
#45693=CARTESIAN_POINT('Ctrl Pts',(-7.0000022045962,16.7131803904388,-9.41295021970705));
#45694=CARTESIAN_POINT('Ctrl Pts',(-7.0000018021616,16.8977448553806,-9.52430133802055));
#45695=CARTESIAN_POINT('Ctrl Pts',(-7.00000129011705,17.0831663074433,-9.62903785732185));
#45696=CARTESIAN_POINT('Ctrl Pts',(-7.0000008616697,17.2383155596398,-9.7166749266387));
#45697=CARTESIAN_POINT('Ctrl Pts',(-7.000000356192,17.3940657682826,-9.7996812518257));
#45698=CARTESIAN_POINT('Ctrl Pts',(-6.99999998816679,17.5501163155923,-9.87817756443021));
#45699=CARTESIAN_POINT('Ctrl Pts',(-6.99999970373598,17.6707210515928,-9.93884397811405));
#45700=CARTESIAN_POINT('Ctrl Pts',(-6.99999950020172,17.7915056704017,-9.99681676418069));
#45701=CARTESIAN_POINT('Ctrl Pts',(-6.99999936067781,17.9123402394409,-10.052163549305));
#45702=CARTESIAN_POINT('Ctrl Pts',(-6.99999924479288,18.0127022819856,-10.0981331459818));
#45703=CARTESIAN_POINT('Ctrl Pts',(-6.99999917321868,18.1130989356455,-10.1422912225978));
#45704=CARTESIAN_POINT('Ctrl Pts',(-6.99999913936894,18.2134600000256,-10.1846774209558));
#45705=CARTESIAN_POINT('Ctrl Pts',(-6.99999912244407,18.2636405322157,-10.2058705201348));
#45706=CARTESIAN_POINT('Ctrl Pts',(-6.99999911499166,18.3138121670858,-10.2266206497493));
#45707=CARTESIAN_POINT('Ctrl Pts',(-6.99999911640469,18.3639665498459,-10.2469328507477));
#45708=CARTESIAN_POINT('Ctrl Pts',(-6.99999911711121,18.3890437412259,-10.257088951247));
#45709=CARTESIAN_POINT('Ctrl Pts',(-6.99999912003628,18.4141166195784,-10.2671355695921));
#45710=CARTESIAN_POINT('Ctrl Pts',(-6.99999912511624,18.4391841515938,-10.2770733379868));
#45711=CARTESIAN_POINT('Ctrl Pts',(-6.99999912765622,18.4517179176014,-10.2820422221842));
#45712=CARTESIAN_POINT('Ctrl Pts',(-6.99999913073504,18.4642503470248,-10.2869838938939));
#45713=CARTESIAN_POINT('Ctrl Pts',(-6.99999913434545,18.4767813121668,-10.2918984324336));
#45714=CARTESIAN_POINT('Ctrl Pts',(-6.99999913750167,18.4877358965313,-10.2961947277656));
#45715=CARTESIAN_POINT('Ctrl Pts',(-6.99999914057212,18.4972872989131,-10.2999248866138));
#45716=CARTESIAN_POINT('Ctrl Pts',(-6.9999991448373,18.5091124036526,-10.3045195519568));
#45717=CARTESIAN_POINT('Ctrl Pts',(-6.99999914545106,18.5108140535906,-10.3051807310472));
#45718=CARTESIAN_POINT('Ctrl Pts',(-6.99999914609152,18.512562817932,-10.3058597313892));
#45719=CARTESIAN_POINT('Ctrl Pts',(-6.99999914676459,18.5143696874875,-10.3065607279455));
#45720=CARTESIAN_POINT('Ctrl Pts',(-6.99999923697446,18.756538526747,-10.4005130123415));
#45721=CARTESIAN_POINT('Ctrl Pts',(-6.99999952144524,19.0001653869772,-10.4851674521453));
#45722=CARTESIAN_POINT('Ctrl Pts',(-6.9999999901845,19.2445368529083,-10.5606734172128));
#45723=CARTESIAN_POINT('Ctrl Pts',(-7.00000044364536,19.4809431068111,-10.6337182888017));
#45724=CARTESIAN_POINT('Ctrl Pts',(-7.00000106797385,19.7180461077543,-10.6982022220885));
#45725=CARTESIAN_POINT('Ctrl Pts',(-7.00000142593571,19.9551865679679,-10.7543697435462));
#45726=CARTESIAN_POINT('Ctrl Pts',(-7.00000178766101,20.1948202019461,-10.8111277816571));
#45727=CARTESIAN_POINT('Ctrl Pts',(-7.00000187627591,20.4344921235716,-10.8593936415268));
#45728=CARTESIAN_POINT('Ctrl Pts',(-7.00000131558885,20.6735749882544,-10.8994259487503));
#45729=CARTESIAN_POINT('Ctrl Pts',(-7.00000103872944,20.7916307599478,-10.9191933416507));
#45730=CARTESIAN_POINT('Ctrl Pts',(-7.00000060480682,20.9095437108038,-10.9369532860267));
#45731=CARTESIAN_POINT('Ctrl Pts',(-6.99999997635804,21.0272429493937,-10.952737451835));
#45732=CARTESIAN_POINT('Ctrl Pts',(-6.99999887928568,21.2327085093352,-10.9802916017586));
#45733=CARTESIAN_POINT('Ctrl Pts',(-6.99999719588043,21.4375214653267,-11.0018249277698));
#45734=CARTESIAN_POINT('Ctrl Pts',(-6.99999590265544,21.64135379194,-11.017557249433));
#45735=CARTESIAN_POINT('Ctrl Pts',(-6.99999568173141,21.6761748475984,-11.0202448312183));
#45736=CARTESIAN_POINT('Ctrl Pts',(-6.99999546003679,21.7128796212977,-11.0229065687753));
#45737=CARTESIAN_POINT('Ctrl Pts',(-6.99999525389925,21.7501379488206,-11.0254108675337));
#45738=CARTESIAN_POINT('Ctrl Pts',(-6.99999512031343,21.7742829151731,-11.0270337586638));
#45739=CARTESIAN_POINT('Ctrl Pts',(-6.99999499325457,21.7986602566777,-11.0285915188677));
#45740=CARTESIAN_POINT('Ctrl Pts',(-6.99999487632653,21.8229070721095,-11.0300601215468));
#45741=CARTESIAN_POINT('Ctrl Pts',(-6.99999457896569,21.8845693793482,-11.0337949390062));
#45742=CARTESIAN_POINT('Ctrl Pts',(-6.99999434329364,21.9460662483819,-11.0369990609859));
#45743=CARTESIAN_POINT('Ctrl Pts',(-6.99999419422111,22.0073884293069,-11.0396820509392));
#45744=CARTESIAN_POINT('Ctrl Pts',(-6.99999365475363,22.229302706117,-11.0493913236069));
#45745=CARTESIAN_POINT('Ctrl Pts',(-6.99999426201958,22.4489302340576,-11.052275764615));
#45746=CARTESIAN_POINT('Ctrl Pts',(-6.99999708882621,22.6658974946071,-11.0487792497662));
#45747=CARTESIAN_POINT('Ctrl Pts',(-6.99999738657651,22.6887508674568,-11.048410958452));
#45748=CARTESIAN_POINT('Ctrl Pts',(-6.99999770879897,22.7115747727124,-11.0479718660013));
#45749=CARTESIAN_POINT('Ctrl Pts',(-6.99999805663936,22.7343688068517,-11.0474624862398));
#45750=CARTESIAN_POINT('Ctrl Pts',(-6.99999863108817,22.7720125263258,-11.0466212595955));
#45751=CARTESIAN_POINT('Ctrl Pts',(-6.99999927541435,22.8095747740487,-11.0455883343058));
#45752=CARTESIAN_POINT('Ctrl Pts',(-6.99999999465569,22.8470537700766,-11.0443660188129));
#45753=CARTESIAN_POINT('Ctrl Pts',(-7.00000393353181,23.0523049357241,-11.0376720913791));
#45754=CARTESIAN_POINT('Ctrl Pts',(-7.00001006487458,23.2550551876909,-11.025299315509));
#45755=CARTESIAN_POINT('Ctrl Pts',(-7.00001375756537,23.4549607434785,-11.0076804777777));
#45756=CARTESIAN_POINT('Ctrl Pts',(-7.00001750474234,23.6578159341913,-10.9898016715884));
#45757=CARTESIAN_POINT('Ctrl Pts',(-7.00001874207268,23.8577419415626,-10.9665208647451));
#45758=CARTESIAN_POINT('Ctrl Pts',(-7.00001328548954,24.0544307360115,-10.9382749572289));
#45759=CARTESIAN_POINT('Ctrl Pts',(-7.00001262288608,24.0783150372645,-10.934845001973));
#45760=CARTESIAN_POINT('Ctrl Pts',(-7.0000118623437,24.1021516637156,-10.9313418142916));
#45761=CARTESIAN_POINT('Ctrl Pts',(-7.00001099700081,24.1259401133038,-10.9277661612309));
#45762=CARTESIAN_POINT('',(-6.271594443024,24.2690120587724,-11.8794941632625));
#45763=CARTESIAN_POINT('Origin',(-5.99998362344297,24.1259473036637,-10.9277594519388));
#45764=CARTESIAN_POINT('Ctrl Pts',(-6.26386059979505,13.9442583574626,-8.42071137129207));
#45765=CARTESIAN_POINT('Ctrl Pts',(-6.26455151948238,14.1129908023888,-8.59292016862684));
#45766=CARTESIAN_POINT('Ctrl Pts',(-6.26520985509005,14.2852417224813,-8.75834762210823));
#45767=CARTESIAN_POINT('Ctrl Pts',(-6.26583560718918,14.4604060134602,-8.91699520035935));
#45768=CARTESIAN_POINT('Ctrl Pts',(-6.26647066052081,14.6381739613785,-9.07800092972525));
#45769=CARTESIAN_POINT('Ctrl Pts',(-6.26707215449678,14.8189425471099,-9.23202378228874));
#45770=CARTESIAN_POINT('Ctrl Pts',(-6.26764008971406,15.0021229851888,-9.37909727117105));
#45771=CARTESIAN_POINT('Ctrl Pts',(-6.26812468084495,15.1584218251682,-9.50458783088976));
#45772=CARTESIAN_POINT('Ctrl Pts',(-6.26858483996506,15.3164773504787,-9.62501957376955));
#45773=CARTESIAN_POINT('Ctrl Pts',(-6.26902056744525,15.4759481442513,-9.74043079566719));
#45774=CARTESIAN_POINT('Ctrl Pts',(-6.26953467292203,15.6641043019273,-9.87660201267336));
#45775=CARTESIAN_POINT('Ctrl Pts',(-6.27001476678973,15.8542290240486,-10.0057845274972));
#45776=CARTESIAN_POINT('Ctrl Pts',(-6.27046084965745,16.0457324355046,-10.1281576247455));
#45777=CARTESIAN_POINT('Ctrl Pts',(-6.27062083269891,16.1144131682359,-10.1720454799107));
#45778=CARTESIAN_POINT('Ctrl Pts',(-6.2707764411619,16.1832716979968,-10.2150576431113));
#45779=CARTESIAN_POINT('Ctrl Pts',(-6.27092767507453,16.2522823588231,-10.2572028832353));
#45780=CARTESIAN_POINT('Ctrl Pts',(-6.27136815533791,16.4532811528737,-10.3799540978805));
#45781=CARTESIAN_POINT('Ctrl Pts',(-6.27177152493213,16.6555663660736,-10.4953498283191));
#45782=CARTESIAN_POINT('Ctrl Pts',(-6.27213778385719,16.8585418381092,-10.6036186820221));
#45783=CARTESIAN_POINT('Ctrl Pts',(-6.27250404278226,17.0615173101449,-10.7118875357251));
#45784=CARTESIAN_POINT('Ctrl Pts',(-6.27283319103817,17.2651832295118,-10.8130296163902));
#45785=CARTESIAN_POINT('Ctrl Pts',(-6.27312522862493,17.4689977328183,-10.9072900744684));
#45786=CARTESIAN_POINT('Ctrl Pts',(-6.27334042191518,17.6191822143953,-10.9767476341614));
#45787=CARTESIAN_POINT('Ctrl Pts',(-6.27353526444441,17.7691758351741,-11.042347876032));
#45788=CARTESIAN_POINT('Ctrl Pts',(-6.27370997792537,17.9190755664926,-11.1043414616088));
#45789=CARTESIAN_POINT('Ctrl Pts',(-6.27388469140633,18.0689752978111,-11.1663350471856));
#45790=CARTESIAN_POINT('Ctrl Pts',(-6.27403927583901,18.2187815654056,-11.2247220206197));
#45791=CARTESIAN_POINT('Ctrl Pts',(-6.27417395293615,18.3686262123522,-11.2797074204369));
#45792=CARTESIAN_POINT('Ctrl Pts',(-6.27427013778255,18.4756435497946,-11.3189773657205));
#45793=CARTESIAN_POINT('Ctrl Pts',(-6.27435616858698,18.5826811784756,-11.3565113915369));
#45794=CARTESIAN_POINT('Ctrl Pts',(-6.27443212611559,18.6897920788877,-11.3923811462087));
#45795=CARTESIAN_POINT('Ctrl Pts',(-6.27457884520034,18.8966868207852,-11.4616669388422));
#45796=CARTESIAN_POINT('Ctrl Pts',(-6.27469165502992,19.1080560626436,-11.5261457010041));
#45797=CARTESIAN_POINT('Ctrl Pts',(-6.2747705556043,19.323695632466,-11.5853119206409));
#45798=CARTESIAN_POINT('Ctrl Pts',(-6.27484862874894,19.5370737916784,-11.6438576645601));
#45799=CARTESIAN_POINT('Ctrl Pts',(-6.27489350012138,19.7546332935116,-11.6972017097186));
#45800=CARTESIAN_POINT('Ctrl Pts',(-6.27490516972162,19.9761304716923,-11.7448336552605));
#45801=CARTESIAN_POINT('Ctrl Pts',(-6.27491664573162,20.1939531716346,-11.7916754212218));
#45802=CARTESIAN_POINT('Ctrl Pts',(-6.27489601241902,20.4155840381427,-11.8329930159802));
#45803=CARTESIAN_POINT('Ctrl Pts',(-6.2748432697838,20.6407456233376,-11.8682811185367));
#45804=CARTESIAN_POINT('Ctrl Pts',(-6.2747905672207,20.8657361381505,-11.9035424103511));
#45805=CARTESIAN_POINT('Ctrl Pts',(-6.27470580410768,21.0942521822708,-11.9327834027245));
#45806=CARTESIAN_POINT('Ctrl Pts',(-6.27458898044473,21.3259690497801,-11.9554796923451));
#45807=CARTESIAN_POINT('Ctrl Pts',(-6.27454781417929,21.4076213266664,-11.9634773998245));
#45808=CARTESIAN_POINT('Ctrl Pts',(-6.27450266695934,21.4896706048662,-11.9706622567438));
#45809=CARTESIAN_POINT('Ctrl Pts',(-6.27445353877278,21.5721011963913,-11.9770107061708));
#45810=CARTESIAN_POINT('Ctrl Pts',(-6.27431624112677,21.8024684655282,-11.9947526018758));
#45811=CARTESIAN_POINT('Ctrl Pts',(-6.27414785115202,22.0358175823162,-12.0059621193271));
#45812=CARTESIAN_POINT('Ctrl Pts',(-6.2739483685844,22.2717646695394,-12.0102364741364));
#45813=CARTESIAN_POINT('Ctrl Pts',(-6.27375072707306,22.5055341636434,-12.0144713802468));
#45814=CARTESIAN_POINT('Ctrl Pts',(-6.2735225642374,22.7418539878509,-12.0118985196058));
#45815=CARTESIAN_POINT('Ctrl Pts',(-6.27326387982054,22.9803003608198,-12.0021219073502));
#45816=CARTESIAN_POINT('Ctrl Pts',(-6.27300884337127,23.2153841630831,-11.9924831648788));
#45817=CARTESIAN_POINT('Ctrl Pts',(-6.27272414010175,23.4525350029681,-11.975842386317));
#45818=CARTESIAN_POINT('Ctrl Pts',(-6.27240976976577,23.6912965883486,-11.9518163382874));
#45819=CARTESIAN_POINT('Ctrl Pts',(-6.27215746673689,23.8829185840646,-11.9325338424652));
#45820=CARTESIAN_POINT('Ctrl Pts',(-6.27188605477603,24.0755771621085,-11.9084943263574));
#45821=CARTESIAN_POINT('Ctrl Pts',(-6.27159553375594,24.269012168963,-11.8794980525045));
#45822=CARTESIAN_POINT('Origin',(-5.999994993362,24.1259380195517,-10.9277770074801));
#45823=CARTESIAN_POINT('',(-5.98852246661529,25.0410395152426,-11.3308498387572));
#45824=CARTESIAN_POINT('Origin',(-5.999994993362,24.1259380195517,-10.9277770074801));
#45825=CARTESIAN_POINT('Origin',(-6.,24.1259427050578,-10.9277790633915));
#45826=CARTESIAN_POINT('Ctrl Pts',(-5.98841833147186,25.040839013447,-11.3313022800101));
#45827=CARTESIAN_POINT('Ctrl Pts',(-5.98810627263551,25.0938945834088,-11.2108442555191));
#45828=CARTESIAN_POINT('Ctrl Pts',(-5.98726405067241,25.2768814426334,-10.7897532281002));
#45829=CARTESIAN_POINT('Ctrl Pts',(-5.98726405067148,25.5029619533758,-10.243946592786));
#45830=CARTESIAN_POINT('Ctrl Pts',(-5.98810627265534,25.6713270262133,-9.81679902016955));
#45831=CARTESIAN_POINT('Ctrl Pts',(-5.98841833150937,25.7189877605111,-9.69410637652636));
#45832=CARTESIAN_POINT('Ctrl Pts',(-6.58019637618801,25.0471116846997,-11.3340652770895));
#45833=CARTESIAN_POINT('Ctrl Pts',(-6.57988216879889,25.1003453887023,-11.2136609913314));
#45834=CARTESIAN_POINT('Ctrl Pts',(-6.57903377750892,25.283822419077,-10.7926927015325));
#45835=CARTESIAN_POINT('Ctrl Pts',(-6.57903377750808,25.5099484864861,-10.2467760826941));
#45836=CARTESIAN_POINT('Ctrl Pts',(-6.57988216881772,25.6778801673696,-9.81936869533563));
#45837=CARTESIAN_POINT('Ctrl Pts',(-6.58019637622491,25.7253769428462,-9.69658809092832));
#45838=CARTESIAN_POINT('Ctrl Pts',(-7.00079677429206,24.6661026394801,-11.1662377629589));
#45839=CARTESIAN_POINT('Ctrl Pts',(-7.00061248963685,24.71890239789,-11.0471442760213));
#45840=CARTESIAN_POINT('Ctrl Pts',(-7.00011448915271,24.9007955994558,-10.6307100868733));
#45841=CARTESIAN_POINT('Ctrl Pts',(-7.00011448915269,25.1245686196564,-10.0904742265064));
#45842=CARTESIAN_POINT('Ctrl Pts',(-7.00061248964794,25.2904141432989,-9.66739286858448));
#45843=CARTESIAN_POINT('Ctrl Pts',(-7.00079677431321,25.3372908898922,-9.5458459848272));
#45844=CARTESIAN_POINT('Ctrl Pts',(-6.99999917318422,24.1245144806645,-10.927678086825));
#45845=CARTESIAN_POINT('Ctrl Pts',(-6.99999957776486,24.1765264252401,-10.8103725307981));
#45846=CARTESIAN_POINT('Ctrl Pts',(-7.00000004362128,24.355704215903,-10.400186001978));
#45847=CARTESIAN_POINT('Ctrl Pts',(-7.0000000436221,24.5761256622778,-9.86804155660993));
#45848=CARTESIAN_POINT('Ctrl Pts',(-6.99999957776511,24.7394735083832,-9.45129804718199));
#45849=CARTESIAN_POINT('Ctrl Pts',(-6.99999917318346,24.7856430653761,-9.33157249006387));
#45850=CARTESIAN_POINT('Origin',(-5.98852353411045,-11.4730434473617,4.7522901952293));
#45851=CARTESIAN_POINT('Origin',(-7.00021006962827,-11.4504589303418,4.74293534796429));
#45852=CARTESIAN_POINT('Ctrl Pts',(-6.05501399426507,24.9009999601274,-11.6468230574062));
#45853=CARTESIAN_POINT('Ctrl Pts',(-4.03667599617638,24.6398186891149,-12.1728028080739));
#45854=CARTESIAN_POINT('Ctrl Pts',(7.59696227890794E-7,24.4084883660198,
-12.7121777555246));
#45855=CARTESIAN_POINT('Ctrl Pts',(4.03667751556907,24.6398187761839,-12.1728026050588));
#45856=CARTESIAN_POINT('Ctrl Pts',(6.05501627335409,24.901000255044,-11.6468224634765));
#45857=CARTESIAN_POINT('Ctrl Pts',(-6.05501399426507,25.238607264913,-10.8985040433412));
#45858=CARTESIAN_POINT('Ctrl Pts',(-4.03667599617638,25.1429516028745,-11.0707137835862));
#45859=CARTESIAN_POINT('Ctrl Pts',(7.59696227890794E-7,25.1799930233034,
-11.3017734890235));
#45860=CARTESIAN_POINT('Ctrl Pts',(4.03667751556907,25.1429515889299,-11.0707136966136));
#45861=CARTESIAN_POINT('Ctrl Pts',(6.05501627335409,25.2386073729271,-10.8985038488906));
#45862=CARTESIAN_POINT('Ctrl Pts',(-6.05501399426507,25.5530341023971,-10.1393932511011));
#45863=CARTESIAN_POINT('Ctrl Pts',(-4.03667599617638,25.6072779226778,-9.94970177382422));
#45864=CARTESIAN_POINT('Ctrl Pts',(7.59696227453643E-7,25.7969402643708,
-9.81221417039094));
#45865=CARTESIAN_POINT('Ctrl Pts',(4.03667751556907,25.6072778512807,-9.94970182557552));
#45866=CARTESIAN_POINT('Ctrl Pts',(6.05501627335409,25.5530340411425,-10.1393934652993));
#45867=CARTESIAN_POINT('Ctrl Pts',(-6.05501399426507,25.843438717122,-9.3715228581096));
#45868=CARTESIAN_POINT('Ctrl Pts',(-4.03667599617638,26.0307827446463,-8.81463118702198));
#45869=CARTESIAN_POINT('Ctrl Pts',(7.59696227453643E-7,26.2486250668438,
-8.26934400982197));
#45870=CARTESIAN_POINT('Ctrl Pts',(4.03667751556907,26.0307826626489,-8.8146313922699));
#45871=CARTESIAN_POINT('Ctrl Pts',(6.05501627335409,25.8434385055746,-9.37152348694043));
#45872=CARTESIAN_POINT('Ctrl Pts',(-5.98852262876652,25.0410393033093,-11.3308502497276));
#45873=CARTESIAN_POINT('Ctrl Pts',(-5.94974655039506,25.0351515941518,-11.3431133877847));
#45874=CARTESIAN_POINT('Ctrl Pts',(-5.9026883960913,25.0280554837042,-11.3579202581523));
#45875=CARTESIAN_POINT('Ctrl Pts',(-5.84725019583372,25.0198456055148,-11.3751042927631));
#45876=CARTESIAN_POINT('Ctrl Pts',(-5.79793199403674,25.0125420417737,-11.3903913273834));
#45877=CARTESIAN_POINT('Ctrl Pts',(-5.74198182120236,25.0043567201721,-11.4075607859964));
#45878=CARTESIAN_POINT('Ctrl Pts',(-5.6793307029936,24.9953721442677,-11.426465064784));
#45879=CARTESIAN_POINT('Ctrl Pts',(-5.62086562486345,24.9869878736077,-11.4441062524901));
#45880=CARTESIAN_POINT('Ctrl Pts',(-5.55656513515357,24.9779073852414,-11.463258811785));
#45881=CARTESIAN_POINT('Ctrl Pts',(-5.48637318192282,24.9682159074148,-11.4837630384779));
#45882=CARTESIAN_POINT('Ctrl Pts',(-5.42062865300875,24.9591384902058,-11.5029680992096));
#45883=CARTESIAN_POINT('Ctrl Pts',(-5.34971558538561,24.9495249779784,-11.5233592082409));
#45884=CARTESIAN_POINT('Ctrl Pts',(-5.27358792079333,24.9394637661138,-11.5447632446162));
#45885=CARTESIAN_POINT('Ctrl Pts',(-5.23094195729711,24.9338275749052,-11.5567535737406));
#45886=CARTESIAN_POINT('Ctrl Pts',(-5.18665958579444,24.9280512324723,-11.5690609837086));
#45887=CARTESIAN_POINT('Ctrl Pts',(-5.1407327094781,24.9221531728174,-11.5816483787659));
#45888=CARTESIAN_POINT('Ctrl Pts',(-5.08889805502216,24.9154964195459,-11.5958549463713));
#45889=CARTESIAN_POINT('Ctrl Pts',(-5.03496462552337,24.9086806638732,-11.6104269526063));
#45890=CARTESIAN_POINT('Ctrl Pts',(-4.97891809278852,24.9017306812036,-11.6253144892783));
#45891=CARTESIAN_POINT('Ctrl Pts',(-4.97191227619667,24.9008619333698,-11.6271754313623));
#45892=CARTESIAN_POINT('Ctrl Pts',(-4.96487344236937,24.8999910880212,-11.6290413035143));
#45893=CARTESIAN_POINT('Ctrl Pts',(-4.95780155876438,24.8991182004358,-11.6309119924244));
#45894=CARTESIAN_POINT('Ctrl Pts',(-4.95072967515938,24.8982453128505,-11.6327826813344));
#45895=CARTESIAN_POINT('Ctrl Pts',(-4.94968891732262,24.8981176084339,-11.6330565258536));
#45896=CARTESIAN_POINT('Ctrl Pts',(-4.94641137045497,24.8977141068387,-11.6339214872236));
#45897=CARTESIAN_POINT('Ctrl Pts',(-4.93985627671968,24.8969071036484,-11.6356514099635));
#45898=CARTESIAN_POINT('Ctrl Pts',(-4.93317300322536,24.8960861509461,-11.6374116051909));
#45899=CARTESIAN_POINT('Ctrl Pts',(-4.92636142104071,24.8952514565616,-11.6392016654597));
#45900=CARTESIAN_POINT('Ctrl Pts',(-4.91273825667142,24.8935820677926,-11.6427817859974));
#45901=CARTESIAN_POINT('Ctrl Pts',(-4.89860185754123,24.891857712009,-11.6464813665709));
#45902=CARTESIAN_POINT('Ctrl Pts',(-4.88395129397506,24.8900798204547,-11.6502976733481));
#45903=CARTESIAN_POINT('Ctrl Pts',(-4.82889198736725,24.8833982019791,-11.6646400025022));
#45904=CARTESIAN_POINT('Ctrl Pts',(-4.76657070444679,24.8759606415624,-11.6806303902859));
#45905=CARTESIAN_POINT('Ctrl Pts',(-4.69692567007587,24.8678685078306,-11.6980688734675));
#45906=CARTESIAN_POINT('Ctrl Pts',(-4.69244416228836,24.8673477964739,-11.6991910022579));
#45907=CARTESIAN_POINT('Ctrl Pts',(-4.68793232944609,24.866824382464,-11.7003191105458));
#45908=CARTESIAN_POINT('Ctrl Pts',(-4.68339015508959,24.8662982960782,-11.7014531379833));
#45909=CARTESIAN_POINT('Ctrl Pts',(-4.61719643682191,24.8586315683679,-11.7179794724683));
#45910=CARTESIAN_POINT('Ctrl Pts',(-4.54455890139893,24.8503959953999,-11.7357657894902));
#45911=CARTESIAN_POINT('Ctrl Pts',(-4.46541859029337,24.8416948429548,-11.7546040661354));
#45912=CARTESIAN_POINT('Ctrl Pts',(-4.45473449345366,24.8405201703507,-11.7571472703401));
#45913=CARTESIAN_POINT('Ctrl Pts',(-4.44393188009192,24.8393370441802,-11.7597095757516));
#45914=CARTESIAN_POINT('Ctrl Pts',(-4.43301060514178,24.8381457490915,-11.7622904018907));
#45915=CARTESIAN_POINT('Ctrl Pts',(-4.38710138739875,24.8331379614591,-11.773139291761));
#45916=CARTESIAN_POINT('Ctrl Pts',(-4.33909521834272,24.8279855675989,-11.7843160329874));
#45917=CARTESIAN_POINT('Ctrl Pts',(-4.28898063287715,24.822710589797,-11.7957754509205));
#45918=CARTESIAN_POINT('Ctrl Pts',(-4.26392334014436,24.820073100896,-11.801505159887));
#45919=CARTESIAN_POINT('Ctrl Pts',(-4.23833894330931,24.8174049645217,-11.8073055373451));
#45920=CARTESIAN_POINT('Ctrl Pts',(-4.21222597316621,24.8147091518377,-11.8131704340925));
#45921=CARTESIAN_POINT('Ctrl Pts',(-4.19916948809466,24.8133612454958,-11.8161028824662));
#45922=CARTESIAN_POINT('Ctrl Pts',(-4.18598085969634,24.8120064199622,-11.8190514606104));
#45923=CARTESIAN_POINT('Ctrl Pts',(-4.17265990426549,24.8106450525724,-11.8220153849909));
#45924=CARTESIAN_POINT('Ctrl Pts',(-4.16599942655006,24.8099643688776,-11.8234973471811));
#45925=CARTESIAN_POINT('Ctrl Pts',(-4.15930586707652,24.8092820497102,-11.8249831459266));
#45926=CARTESIAN_POINT('Ctrl Pts',(-4.15257920279502,24.8085981430141,-11.8264726814627));
#45927=CARTESIAN_POINT('Ctrl Pts',(-4.14585253851352,24.807914236318,-11.8279622169988));
#45928=CARTESIAN_POINT('Ctrl Pts',(-4.13787834775704,24.8071059154165,-11.8297231040874));
#45929=CARTESIAN_POINT('Ctrl Pts',(-4.13229987245898,24.8065417084999,-11.8309523981142));
#45930=CARTESIAN_POINT('Ctrl Pts',(-4.01426669075566,24.7946038340917,-11.8569626388121));
#45931=CARTESIAN_POINT('Ctrl Pts',(-3.89866246854569,24.7834250122886,-11.8814033178166));
#45932=CARTESIAN_POINT('Ctrl Pts',(-3.78553934540173,24.7729414085328,-11.904385539706));
#45933=CARTESIAN_POINT('Ctrl Pts',(-3.72757714111731,24.7675698031028,-11.9161612068114));
#45934=CARTESIAN_POINT('Ctrl Pts',(-3.67026631188076,24.7623803834644,-11.9275548269377));
#45935=CARTESIAN_POINT('Ctrl Pts',(-3.613613871405,24.7573626209778,-11.9385861494722));
#45936=CARTESIAN_POINT('Ctrl Pts',(-3.53000420327667,24.7499572302704,-11.9548665640205));
#45937=CARTESIAN_POINT('Ctrl Pts',(-3.44782800787335,24.7429278580583,-11.9703532324538));
#45938=CARTESIAN_POINT('Ctrl Pts',(-3.36710459626749,24.7362465183607,-11.9850985588426));
#45939=CARTESIAN_POINT('Ctrl Pts',(-3.32674289046455,24.7329058485118,-11.992471222037));
#45940=CARTESIAN_POINT('Ctrl Pts',(-3.28674438064314,24.7296521961897,-11.9996585541475));
#45941=CARTESIAN_POINT('Ctrl Pts',(-3.2471112461582,24.7264821808726,-12.0066669927124));
#45942=CARTESIAN_POINT('Ctrl Pts',(-3.21205403780241,24.7236781662796,-12.0128662573987));
#45943=CARTESIAN_POINT('Ctrl Pts',(-3.17869660210454,24.721049366133,-12.0186825053255));
#45944=CARTESIAN_POINT('Ctrl Pts',(-3.14328848633031,24.7183020793255,-12.0247653281962));
#45945=CARTESIAN_POINT('Ctrl Pts',(-3.13866675716948,24.7179434831316,-12.0255593032278));
#45946=CARTESIAN_POINT('Ctrl Pts',(-3.13401008974949,24.717582899303,-12.0263577545565));
#45947=CARTESIAN_POINT('Ctrl Pts',(-3.12931014363493,24.7172197033507,-12.0271620661654));
#45948=CARTESIAN_POINT('Ctrl Pts',(-2.9664809447597,24.7046368131405,-12.0550273675416));
#45949=CARTESIAN_POINT('Ctrl Pts',(-2.80321460461108,24.6930123547265,-12.0808729408053));
#45950=CARTESIAN_POINT('Ctrl Pts',(-2.63956869903732,24.6823481561796,-12.1046611143612));
#45951=CARTESIAN_POINT('Ctrl Pts',(-2.55774574625044,24.6770160569062,-12.1165552011391));
#45952=CARTESIAN_POINT('Ctrl Pts',(-2.47582807006359,24.6719238730238,-12.1279352771598));
#45953=CARTESIAN_POINT('Ctrl Pts',(-2.3938232040891,24.6670715572768,-12.1387972933987));
#45954=CARTESIAN_POINT('Ctrl Pts',(-2.35282077110186,24.6646453994033,-12.1442283015181));
#45955=CARTESIAN_POINT('Ctrl Pts',(-2.31179654066698,24.6622792086921,-12.1495297947366));
#45956=CARTESIAN_POINT('Ctrl Pts',(-2.27075145561316,24.6599729795422,-12.1547012663989));
#45957=CARTESIAN_POINT('Ctrl Pts',(-2.23483700619106,24.6579550290361,-12.1592263041033));
#45958=CARTESIAN_POINT('Ctrl Pts',(-2.19890658995127,24.6559829866123,-12.1636517940586));
#45959=CARTESIAN_POINT('Ctrl Pts',(-2.16296083870178,24.6540568481957,-12.1679773965549));
#45960=CARTESIAN_POINT('Ctrl Pts',(-2.15782573138042,24.6537816855648,-12.1685953397687));
#45961=CARTESIAN_POINT('Ctrl Pts',(-2.15064935716421,24.6533988539371,-12.1694551961909));
#45962=CARTESIAN_POINT('Ctrl Pts',(-2.14755457971117,24.653234170739,-12.1698251096412));
#45963=CARTESIAN_POINT('Ctrl Pts',(-2.0717107903665,24.6491982754368,-12.1788905879287));
#45964=CARTESIAN_POINT('Ctrl Pts',(-1.98853406098885,24.6450197213633,-12.1882987669993));
#45965=CARTESIAN_POINT('Ctrl Pts',(-1.89799855360911,24.6408291651433,-12.1977613756536));
#45966=CARTESIAN_POINT('Ctrl Pts',(-1.80788627331092,24.636658198551,-12.2071797493734));
#45967=CARTESIAN_POINT('Ctrl Pts',(-1.71048385448022,24.6324753978846,-12.2166521123484));
#45968=CARTESIAN_POINT('Ctrl Pts',(-1.6057658198115,24.6284288416531,-12.2258461731663));
#45969=CARTESIAN_POINT('Ctrl Pts',(-1.54093857958377,24.6259237614752,-12.2315378918009));
#45970=CARTESIAN_POINT('Ctrl Pts',(-1.47330769454403,24.6234712769607,-12.2371219973271));
#45971=CARTESIAN_POINT('Ctrl Pts',(-1.40286712017468,24.6211100263704,-12.2425102693972));
#45972=CARTESIAN_POINT('Ctrl Pts',(-1.28740839052695,24.6172397144659,-12.2513421543411));
#45973=CARTESIAN_POINT('Ctrl Pts',(-1.16440226992658,24.6136137121762,-12.2596505485663));
#45974=CARTESIAN_POINT('Ctrl Pts',(-1.0338383390704,24.6104187896776,-12.2670000215224));
#45975=CARTESIAN_POINT('Ctrl Pts',(-0.995600257807905,24.6094830970608,
-12.2691524516942));
#45976=CARTESIAN_POINT('Ctrl Pts',(-0.956713927726055,24.6085844808045,
-12.2712223053479));
#45977=CARTESIAN_POINT('Ctrl Pts',(-0.917179087092564,24.607727867909,-12.2731978396645));
#45978=CARTESIAN_POINT('Ctrl Pts',(-0.829915808871143,24.6058371090687,
-12.2775583378465));
#45979=CARTESIAN_POINT('Ctrl Pts',(-0.739493571338707,24.6041509962435,
-12.2814596062158));
#45980=CARTESIAN_POINT('Ctrl Pts',(-0.645913648560607,24.6027251256842,
-12.2847669497706));
#45981=CARTESIAN_POINT('Ctrl Pts',(-0.599123687171559,24.6020121904045,
-12.2864206215479));
#45982=CARTESIAN_POINT('Ctrl Pts',(-0.551544304326092,24.6013642873024,
-12.2879257980049));
#45983=CARTESIAN_POINT('Ctrl Pts',(-0.503176821229749,24.6007886184522,
-12.2892646616672));
#45984=CARTESIAN_POINT('Ctrl Pts',(-0.478993079681576,24.6005007840271,
-12.2899340934983));
#45985=CARTESIAN_POINT('Ctrl Pts',(-0.454612313067827,24.600231006085,-12.2905619460855));
#45986=CARTESIAN_POINT('Ctrl Pts',(-0.430034768691489,24.599980179451,-12.2911459699869));
#45987=CARTESIAN_POINT('Ctrl Pts',(-0.417745996503321,24.5998547661339,
-12.2914379819376));
#45988=CARTESIAN_POINT('Ctrl Pts',(-0.405408029874993,24.5997340905027,
-12.2917190366455));
#45989=CARTESIAN_POINT('Ctrl Pts',(-0.393020899026227,24.5996182655297,
-12.2919888485103));
#45990=CARTESIAN_POINT('Ctrl Pts',(-0.386827333601843,24.5995603530432,
-12.2921237544427));
#45991=CARTESIAN_POINT('Ctrl Pts',(-0.380621477122377,24.5995036532121,
-12.2922558496597));
#45992=CARTESIAN_POINT('Ctrl Pts',(-0.374403333613394,24.5994481802028,
-12.2923850982298));
#45993=CARTESIAN_POINT('Ctrl Pts',(-0.36818519010441,24.5993927071935,-12.2925143467999));
#45994=CARTESIAN_POINT('Ctrl Pts',(-0.359951179428822,24.5993214491376,
-12.2926803918735));
#45995=CARTESIAN_POINT('Ctrl Pts',(-0.355712046080024,24.5992854558015,
-12.2927642679839));
#45996=CARTESIAN_POINT('Ctrl Pts',(-0.236619694947637,24.5982742748198,
-12.2951206466052));
#45997=CARTESIAN_POINT('Ctrl Pts',(-0.118036480863534,24.5977738841301,
-12.2962957273024));
#45998=CARTESIAN_POINT('Ctrl Pts',(4.36983782492462E-13,24.5977653883777,
-12.296312723946));
#45999=CARTESIAN_POINT('Ctrl Pts',(0.150862673191552,24.5977545299388,-12.2963344473919));
#46000=CARTESIAN_POINT('Ctrl Pts',(0.300832233086994,24.5985476990758,-12.294463969907));
#46001=CARTESIAN_POINT('Ctrl Pts',(0.449830184999458,24.6001291281758,-12.2907805068968));
#46002=CARTESIAN_POINT('Ctrl Pts',(0.58261791299645,24.6015385057845,-12.2874977860406));
#46003=CARTESIAN_POINT('Ctrl Pts',(0.714638276046149,24.6035753943051,-12.28277203577));
#46004=CARTESIAN_POINT('Ctrl Pts',(0.845857318554737,24.6062301793636,-12.2766505732036));
#46005=CARTESIAN_POINT('Ctrl Pts',(0.911466839809031,24.6075575718929,-12.2735898419204));
#46006=CARTESIAN_POINT('Ctrl Pts',(0.97687603055194,24.6090394082341,-12.2701801674416));
#46007=CARTESIAN_POINT('Ctrl Pts',(1.04208087787506,24.6106743255165,-12.2664273684045));
#46008=CARTESIAN_POINT('Ctrl Pts',(1.07468330153662,24.6114917841576,-12.2645509688859));
#46009=CARTESIAN_POINT('Ctrl Pts',(1.10723463932392,24.6123475114073,-12.2625887874429));
#46010=CARTESIAN_POINT('Ctrl Pts',(1.1397343959841,24.6132413277545,-12.2605415464827));
#46011=CARTESIAN_POINT('Ctrl Pts',(1.15598427431419,24.6136882359282,-12.2595179260026));
#46012=CARTESIAN_POINT('Ctrl Pts',(1.17222125736142,24.6141446662819,-12.2584730405988));
#46013=CARTESIAN_POINT('Ctrl Pts',(1.18844528400384,24.6146105958455,-12.257406980262));
#46014=CARTESIAN_POINT('Ctrl Pts',(1.19655729732504,24.6148435606272,-12.2568739500935));
#46015=CARTESIAN_POINT('Ctrl Pts',(1.20466607154499,24.6150789002057,-12.2563356261892));
#46016=CARTESIAN_POINT('Ctrl Pts',(1.21277159907198,24.6153166116882,-12.2557920197572));
#46017=CARTESIAN_POINT('Ctrl Pts',(1.21682436283548,24.6154354674294,-12.2555202165412));
#46018=CARTESIAN_POINT('Ctrl Pts',(1.22087631492573,24.6155549161463,-12.2552470926931));
#46019=CARTESIAN_POINT('Ctrl Pts',(1.22492745439972,24.6156749574131,-12.2549726497381));
#46020=CARTESIAN_POINT('Ctrl Pts',(1.22695302413672,24.6157349780466,-12.2548354282606));
#46021=CARTESIAN_POINT('Ctrl Pts',(1.22897839071965,24.6157951468175,-12.2546978770064));
#46022=CARTESIAN_POINT('Ctrl Pts',(1.2310035540316,24.6158554636566,-12.2545599961983));
#46023=CARTESIAN_POINT('Ctrl Pts',(1.23302871734353,24.6159157804956,-12.2544221153902));
#46024=CARTESIAN_POINT('Ctrl Pts',(1.23643078757501,24.6160174704414,-12.2541896791548));
#46025=CARTESIAN_POINT('Ctrl Pts',(1.23707843403692,24.6160368583227,-12.2541453653075));
#46026=CARTESIAN_POINT('Ctrl Pts',(1.27880639131658,24.6172860223795,-12.2512902175771));
#46027=CARTESIAN_POINT('Ctrl Pts',(1.3294741638359,24.618853278113,-12.2477083113246));
#46028=CARTESIAN_POINT('Ctrl Pts',(1.38903584785586,24.6208543134989,-12.2431466992377));
#46029=CARTESIAN_POINT('Ctrl Pts',(1.45025678814527,24.6229110932877,-12.2384580107665));
#46030=CARTESIAN_POINT('Ctrl Pts',(1.52087407136146,24.6254261982142,-12.2327340521914));
#46031=CARTESIAN_POINT('Ctrl Pts',(1.60083784957267,24.6285488023689,-12.2256478324131));
#46032=CARTESIAN_POINT('Ctrl Pts',(1.68763009550311,24.6319380597778,-12.2179564883637));
#46033=CARTESIAN_POINT('Ctrl Pts',(1.7854332718843,24.6360429187669,-12.2086601522125));
#46034=CARTESIAN_POINT('Ctrl Pts',(1.89418363901753,24.6410822169797,-12.1972817179609));
#46035=CARTESIAN_POINT('Ctrl Pts',(1.97507214192233,24.6448304460558,-12.1888184406749));
#46036=CARTESIAN_POINT('Ctrl Pts',(2.06201704854094,24.6490962947508,-12.1792018218676));
#46037=CARTESIAN_POINT('Ctrl Pts',(2.15499213008654,24.6539785207663,-12.168219356019));
#46038=CARTESIAN_POINT('Ctrl Pts',(2.28380963126724,24.6607428725159,-12.1530030874888));
#46039=CARTESIAN_POINT('Ctrl Pts',(2.42418371072383,24.6687031512469,-12.1351384975467));
#46040=CARTESIAN_POINT('Ctrl Pts',(2.57592898429611,24.6782383673289,-12.1138309581078));
#46041=CARTESIAN_POINT('Ctrl Pts',(2.68639476604679,24.6851797044386,-12.0983197402234));
#46042=CARTESIAN_POINT('Ctrl Pts',(2.8028865775025,24.6929558858114,-12.0809834737766));
#46043=CARTESIAN_POINT('Ctrl Pts',(2.92533290147752,24.7017077540705,-12.0615333397425));
#46044=CARTESIAN_POINT('Ctrl Pts',(3.04038690825321,24.7099312554162,-12.0432574472511));
#46045=CARTESIAN_POINT('Ctrl Pts',(3.16069310575817,24.7190216168601,-12.0231039149372));
#46046=CARTESIAN_POINT('Ctrl Pts',(3.28616259950354,24.7291241165009,-12.0007808188169));
#46047=CARTESIAN_POINT('Ctrl Pts',(3.31917344125611,24.731782069498,-11.9949076446177));
#46048=CARTESIAN_POINT('Ctrl Pts',(3.3525416907452,24.7345099845977,-11.9888845436361));
#46049=CARTESIAN_POINT('Ctrl Pts',(3.38626572903287,24.737310278026,-11.9827067940583));
#46050=CARTESIAN_POINT('Ctrl Pts',(3.4672178741226,24.744032182383,-11.967877547457));
#46051=CARTESIAN_POINT('Ctrl Pts',(3.5502193955923,24.7511726072005,-11.9521539542066));
#46052=CARTESIAN_POINT('Ctrl Pts',(3.63524342703742,24.758770261966,-11.9354607867723));
#46053=CARTESIAN_POINT('Ctrl Pts',(3.67775544275998,24.7625690893488,-11.9271142030551));
#46054=CARTESIAN_POINT('Ctrl Pts',(3.72077308600985,24.7664822359632,-11.9185252313042));
#46055=CARTESIAN_POINT('Ctrl Pts',(3.76429261860533,24.7705147554021,-11.9096842161446));
#46056=CARTESIAN_POINT('Ctrl Pts',(3.78605238490307,24.7725310151215,-11.9052637085649));
#46057=CARTESIAN_POINT('Ctrl Pts',(3.80793762353956,24.7745771189329,-11.9007801905478));
#46058=CARTESIAN_POINT('Ctrl Pts',(3.82994785495516,24.7766537073945,-11.896232451032));
#46059=CARTESIAN_POINT('Ctrl Pts',(3.84095297066295,24.7776920016253,-11.8939585812741));
#46060=CARTESIAN_POINT('Ctrl Pts',(3.85198933456561,24.7787379170807,-11.8916686561703));
#46061=CARTESIAN_POINT('Ctrl Pts',(3.86305688536165,24.7797915346484,-11.8893625235876));
#46062=CARTESIAN_POINT('Ctrl Pts',(3.86859066075967,24.7803183434323,-11.8882094572963));
#46063=CARTESIAN_POINT('Ctrl Pts',(3.87413223288104,24.7808470777483,-11.8870523391372));
#46064=CARTESIAN_POINT('Ctrl Pts',(3.87968159397177,24.7813777477599,-11.885891150046));
#46065=CARTESIAN_POINT('Ctrl Pts',(3.88523095506251,24.7819084177716,-11.8847299609548));
#46066=CARTESIAN_POINT('Ctrl Pts',(3.89297592965654,24.7826511797274,-11.8831049768951));
#46067=CARTESIAN_POINT('Ctrl Pts',(3.89635303637021,24.7829755750705,-11.8823953509024));
#46068=CARTESIAN_POINT('Ctrl Pts',(4.05455253139167,24.7981717722322,-11.8491531458965));
#46069=CARTESIAN_POINT('Ctrl Pts',(4.20702419525135,24.8137844834955,-11.8151348605723));
#46070=CARTESIAN_POINT('Ctrl Pts',(4.35383993702875,24.8296204514967,-11.7807734023157));
#46071=CARTESIAN_POINT('Ctrl Pts',(4.49776638929034,24.8451447724241,-11.7470881671935));
#46072=CARTESIAN_POINT('Ctrl Pts',(4.63625734266588,24.8608835998161,-11.7130732733762));
#46073=CARTESIAN_POINT('Ctrl Pts',(4.76938054378893,24.8766740884016,-11.6790902601868));
#46074=CARTESIAN_POINT('Ctrl Pts',(4.90003539201982,24.8921717918239,-11.6457373555599));
#46075=CARTESIAN_POINT('Ctrl Pts',(5.02551969887325,24.9077192645111,-11.6124152200153));
#46076=CARTESIAN_POINT('Ctrl Pts',(5.14589751197744,24.923181544606,-11.5794191457888));
#46077=CARTESIAN_POINT('Ctrl Pts',(5.26549537339328,24.9385436415263,-11.5466368596611));
#46078=CARTESIAN_POINT('Ctrl Pts',(5.38005269865761,24.9538216475631,-11.5141765080823));
#46079=CARTESIAN_POINT('Ctrl Pts',(5.4896322985156,24.9689021151162,-11.4822801409863));
#46080=CARTESIAN_POINT('Ctrl Pts',(5.59870632316951,24.9839130048422,-11.4505309364309));
#46081=CARTESIAN_POINT('Ctrl Pts',(5.70284844862924,24.9987281898052,-11.4193405622832));
#46082=CARTESIAN_POINT('Ctrl Pts',(5.8021206202617,25.0132544553156,-11.3888995459745));
#46083=CARTESIAN_POINT('Ctrl Pts',(5.86628458488748,25.0226434187182,-11.3692241801446));
#46084=CARTESIAN_POINT('Ctrl Pts',(5.92841407534379,25.0319120614579,-11.3498608839104));
#46085=CARTESIAN_POINT('Ctrl Pts',(5.98852581792881,25.0410393365977,-11.3308502649318));
#46086=CARTESIAN_POINT('Ctrl Pts',(-6.39567215432545,24.265774903146,-11.8440001019888));
#46087=CARTESIAN_POINT('Ctrl Pts',(-6.35564925509037,24.2594187557205,-11.8565901638456));
#46088=CARTESIAN_POINT('Ctrl Pts',(-5.98524856741148,24.2012636643636,-11.9719912725476));
#46089=CARTESIAN_POINT('Ctrl Pts',(-5.25616414804593,24.0987563586202,-12.1789682214255));
#46090=CARTESIAN_POINT('Ctrl Pts',(-4.17575802164877,23.9769542776332,-12.4300252137512));
#46091=CARTESIAN_POINT('Ctrl Pts',(-3.01936659820269,23.8792986630108,-12.635041294384));
#46092=CARTESIAN_POINT('Ctrl Pts',(-1.83578627600257,23.8136687543955,-12.7756187500438));
#46093=CARTESIAN_POINT('Ctrl Pts',(-0.697926096906866,23.7825583234657,
-12.8441380550359));
#46094=CARTESIAN_POINT('Ctrl Pts',(0.331404301616038,23.779455773439,-12.8512035366654));
#46095=CARTESIAN_POINT('Ctrl Pts',(1.24580220726389,23.7959565232568,-12.8144576038436));
#46096=CARTESIAN_POINT('Ctrl Pts',(2.07029186514626,23.8272315262671,-12.7465820496497));
#46097=CARTESIAN_POINT('Ctrl Pts',(2.81705936611203,23.869392282327,-12.6564409209412));
#46098=CARTESIAN_POINT('Ctrl Pts',(3.49017608620424,23.9189803910815,-12.5517050127182));
#46099=CARTESIAN_POINT('Ctrl Pts',(4.09496422292832,23.972993995276,-12.4387800495708));
#46100=CARTESIAN_POINT('Ctrl Pts',(4.65004649527303,24.0305536768163,-12.3195545718887));
#46101=CARTESIAN_POINT('Ctrl Pts',(5.18049690603252,24.0928845644996,-12.1916416689504));
#46102=CARTESIAN_POINT('Ctrl Pts',(5.70541816523766,24.1618784673525,-12.051497359207));
#46103=CARTESIAN_POINT('Ctrl Pts',(6.1097803153111,24.2209469472287,-11.9329737822134));
#46104=CARTESIAN_POINT('Ctrl Pts',(6.34031508757241,24.2569835443928,-11.8614131544149));
#46105=CARTESIAN_POINT('Ctrl Pts',(6.39541677055505,24.2657356792402,-11.8440802204204));
#46106=CARTESIAN_POINT('Ctrl Pts',(-6.33011139869697,24.6389171751212,-11.8152694738916));
#46107=CARTESIAN_POINT('Ctrl Pts',(-6.2905632136143,24.6326417224546,-11.827825040408));
#46108=CARTESIAN_POINT('Ctrl Pts',(-5.92452857340538,24.5752212779463,-11.9429199004965));
#46109=CARTESIAN_POINT('Ctrl Pts',(-5.20357284607826,24.4739472076042,-12.149509367077));
#46110=CARTESIAN_POINT('Ctrl Pts',(-4.13461175671286,24.3535549525084,-12.4002991475077));
#46111=CARTESIAN_POINT('Ctrl Pts',(-2.99009397874043,24.2570037555148,-12.6052161854276));
#46112=CARTESIAN_POINT('Ctrl Pts',(-1.81832922056056,24.1921007647318,-12.7457865099649));
#46113=CARTESIAN_POINT('Ctrl Pts',(-0.691521468902351,24.1613240343279,
-12.814324153161));
#46114=CARTESIAN_POINT('Ctrl Pts',(0.328402059320489,24.1582532792487,-12.821393159439));
#46115=CARTESIAN_POINT('Ctrl Pts',(1.23408499152528,24.1745795912403,-12.7846344259474));
#46116=CARTESIAN_POINT('Ctrl Pts',(2.0504931373738,24.2055131843259,-12.7167509212318));
#46117=CARTESIAN_POINT('Ctrl Pts',(2.78979399227695,24.2472061242734,-12.6266188073296));
#46118=CARTESIAN_POINT('Ctrl Pts',(3.45606870618063,24.2962368704784,-12.5219191994195));
#46119=CARTESIAN_POINT('Ctrl Pts',(4.05461471151914,24.3496364162726,-12.4090636434254));
#46120=CARTESIAN_POINT('Ctrl Pts',(4.60387478749737,24.4065338746757,-12.2899461861913));
#46121=CARTESIAN_POINT('Ctrl Pts',(5.12865373502468,24.4681372375982,-12.1621914677793));
#46122=CARTESIAN_POINT('Ctrl Pts',(5.64781964673563,24.5363100389222,-12.022276439811));
#46123=CARTESIAN_POINT('Ctrl Pts',(6.04758703724719,24.5946551774785,-11.9040078838942));
#46124=CARTESIAN_POINT('Ctrl Pts',(6.27541106315239,24.6302374636023,-11.832634783351));
#46125=CARTESIAN_POINT('Ctrl Pts',(6.3298587211672,24.6388783655307,-11.8153494295136));
#46126=CARTESIAN_POINT('Ctrl Pts',(-6.21909462167523,24.9345658565175,-11.6041618753865));
#46127=CARTESIAN_POINT('Ctrl Pts',(-6.18025122001806,24.9284618793619,-11.616587032151));
#46128=CARTESIAN_POINT('Ctrl Pts',(-5.82072605398916,24.8726105239354,-11.7304922022284));
#46129=CARTESIAN_POINT('Ctrl Pts',(-5.11236921312775,24.7741073881107,-11.9350365015387));
#46130=CARTESIAN_POINT('Ctrl Pts',(-4.06204085349769,24.6570764218307,-12.1834178932697));
#46131=CARTESIAN_POINT('Ctrl Pts',(-2.9376206588192,24.563286303404,-12.386392728577));
#46132=CARTESIAN_POINT('Ctrl Pts',(-1.78654233000432,24.5002752909014,-12.5256393828724));
#46133=CARTESIAN_POINT('Ctrl Pts',(-0.679604906695004,24.4704003046752,
-12.5935378394357));
#46134=CARTESIAN_POINT('Ctrl Pts',(0.322775234820087,24.4674185850898,-12.6005420435692));
#46135=CARTESIAN_POINT('Ctrl Pts',(1.21259995881462,24.48326794551,-12.5641242474114));
#46136=CARTESIAN_POINT('Ctrl Pts',(2.01460907294657,24.5132960752993,-12.4968773610704));
#46137=CARTESIAN_POINT('Ctrl Pts',(2.74086259778098,24.5537768690484,-12.4075943492003));
#46138=CARTESIAN_POINT('Ctrl Pts',(3.39541033297856,24.6013967849816,-12.3038851096544));
#46139=CARTESIAN_POINT('Ctrl Pts',(3.98346188181152,24.6532777843204,-12.1921022704338));
#46140=CARTESIAN_POINT('Ctrl Pts',(4.52312475590325,24.7085761466578,-12.0741247427906));
#46141=CARTESIAN_POINT('Ctrl Pts',(5.03875163209351,24.7684672518194,-11.9476048546621));
#46142=CARTESIAN_POINT('Ctrl Pts',(5.54885320696534,24.8347635054044,-11.8090629842029));
#46143=CARTESIAN_POINT('Ctrl Pts',(5.94159338064799,24.8915133781883,-11.6919835098928));
#46144=CARTESIAN_POINT('Ctrl Pts',(6.16536922582763,24.9261233518869,-11.6213467860975));
#46145=CARTESIAN_POINT('Ctrl Pts',(6.2188461543419,24.9345280272955,-11.6042410555399));
#46146=CARTESIAN_POINT('Ctrl Pts',(-6.0944235252482,25.0682520215298,-11.2712582249933));
#46147=CARTESIAN_POINT('Ctrl Pts',(-6.05631315053343,25.0623611570049,-11.2834944621479));
#46148=CARTESIAN_POINT('Ctrl Pts',(-5.703576774987,25.0084636391483,-11.3956677411211));
#46149=CARTESIAN_POINT('Ctrl Pts',(-5.00868072692008,24.9134749280578,-11.5970959616219));
#46150=CARTESIAN_POINT('Ctrl Pts',(-3.97883577950606,24.8007932001164,-11.8416189837205));
#46151=CARTESIAN_POINT('Ctrl Pts',(-2.87697998756759,24.7106292980149,-12.0413659895638));
#46152=CARTESIAN_POINT('Ctrl Pts',(-1.74953270102815,24.6501329141197,-12.1783524777748));
#46153=CARTESIAN_POINT('Ctrl Pts',(-0.665590719009689,24.6214691809497,
-12.2451377662104));
#46154=CARTESIAN_POINT('Ctrl Pts',(0.316136038753768,24.6186082091784,-12.252027451311));
#46155=CARTESIAN_POINT('Ctrl Pts',(1.18750276604363,24.6338148510926,-12.2162064264699));
#46156=CARTESIAN_POINT('Ctrl Pts',(1.9729205261056,24.662633058189,-12.1500579331026));
#46157=CARTESIAN_POINT('Ctrl Pts',(2.68428382255306,24.7015048827846,-12.0622203269822));
#46158=CARTESIAN_POINT('Ctrl Pts',(3.32557899278067,24.7472649536685,-11.9601712105928));
#46159=CARTESIAN_POINT('Ctrl Pts',(3.90188993653852,24.7971582354132,-11.8501564777456));
#46160=CARTESIAN_POINT('Ctrl Pts',(4.43092963053168,24.8503790191096,-11.7340236139045));
#46161=CARTESIAN_POINT('Ctrl Pts',(4.93654521767705,24.9080639417193,-11.6094608352251));
#46162=CARTESIAN_POINT('Ctrl Pts',(5.43686957263232,24.9719660756905,-11.473041994514));
#46163=CARTESIAN_POINT('Ctrl Pts',(5.82216258062342,25.0267059804824,-11.3577445394207));
#46164=CARTESIAN_POINT('Ctrl Pts',(6.04171208841225,25.0601043017063,-11.2881818237279));
#46165=CARTESIAN_POINT('Ctrl Pts',(6.09417956626521,25.0682154577126,-11.2713362394887));
#46166=CARTESIAN_POINT('',(6.27159454871108,24.2690137147111,-11.8794923468356));
#46167=CARTESIAN_POINT('Origin',(5.999999949017,24.12594200518,-10.9277802669376));
#46168=CARTESIAN_POINT('Ctrl Pts',(-6.27159387328068,24.2690123753745,-11.8794984953319));
#46169=CARTESIAN_POINT('Ctrl Pts',(-6.13239664937028,24.2474082730374,-11.9224692187189));
#46170=CARTESIAN_POINT('Ctrl Pts',(-5.98564492666201,24.2255025436533,-11.9663158733557));
#46171=CARTESIAN_POINT('Ctrl Pts',(-5.83132864861891,24.2035349808948,-12.0105538996301));
#46172=CARTESIAN_POINT('Ctrl Pts',(-5.679074110429,24.1818609153628,-12.0542008845514));
#46173=CARTESIAN_POINT('Ctrl Pts',(-5.51945550383331,24.1601268866317,-12.0982288854611));
#46174=CARTESIAN_POINT('Ctrl Pts',(-5.35247247395099,24.1385689974971,-12.1421228435869));
#46175=CARTESIAN_POINT('Ctrl Pts',(-5.32566610845767,24.1351082347129,-12.1491692930692));
#46176=CARTESIAN_POINT('Ctrl Pts',(-5.29866997954998,24.1316520193249,-12.1562121822653));
#46177=CARTESIAN_POINT('Ctrl Pts',(-5.27148411637172,24.1282013361865,-12.1632492579947));
#46178=CARTESIAN_POINT('Ctrl Pts',(-5.14595239291341,24.1122676798361,-12.1957432140862));
#46179=CARTESIAN_POINT('Ctrl Pts',(-5.01637482818976,24.096451644679,-12.2281144526996));
#46180=CARTESIAN_POINT('Ctrl Pts',(-4.88275739366669,24.080862396749,-12.2601325356358));
#46181=CARTESIAN_POINT('Ctrl Pts',(-4.7110640926815,24.0608308084571,-12.3012745495516));
#46182=CARTESIAN_POINT('Ctrl Pts',(-4.53269553658461,24.0411729421543,-12.341836233405));
#46183=CARTESIAN_POINT('Ctrl Pts',(-4.34764553875065,24.0221340594359,-12.3812950680686));
#46184=CARTESIAN_POINT('Ctrl Pts',(-4.29583923524703,24.0168039640669,-12.3923419007539));
#46185=CARTESIAN_POINT('Ctrl Pts',(-4.243509363582,24.0115224543185,-12.4033020094073));
#46186=CARTESIAN_POINT('Ctrl Pts',(-4.19065603668429,24.0062950769768,-12.4141632529344));
#46187=CARTESIAN_POINT('Ctrl Pts',(-4.14338231788257,24.0016195422276,-12.423877899154));
#46188=CARTESIAN_POINT('Ctrl Pts',(-4.09568982943223,23.9969873138978,-12.4335134474914));
#46189=CARTESIAN_POINT('Ctrl Pts',(-4.04757899984503,23.9924025362211,-12.4430611407423));
#46190=CARTESIAN_POINT('Ctrl Pts',(-3.90056248222818,23.9783924255274,-12.472236871551));
#46191=CARTESIAN_POINT('Ctrl Pts',(-3.74963598148268,23.964824956328,-12.5005941095896));
#46192=CARTESIAN_POINT('Ctrl Pts',(-3.59479967323274,23.9518214674941,-12.5278747701407));
#46193=CARTESIAN_POINT('Ctrl Pts',(-3.51738151910778,23.9453197230771,-12.5415151004163));
#46194=CARTESIAN_POINT('Ctrl Pts',(-3.43898590449499,23.9389590693787,-12.5548860361321));
#46195=CARTESIAN_POINT('Ctrl Pts',(-3.35961280203394,23.9327552491476,-12.5679537419326));
#46196=CARTESIAN_POINT('Ctrl Pts',(-3.31992625080342,23.929653339032,-12.5744875948328));
#46197=CARTESIAN_POINT('Ctrl Pts',(-3.27999532521964,23.9265906354718,-12.5809456244407));
#46198=CARTESIAN_POINT('Ctrl Pts',(-3.23982002131168,23.9235691510685,-12.5873234953188));
#46199=CARTESIAN_POINT('Ctrl Pts',(-3.2197323693577,23.9220584088669,-12.5905124307578));
#46200=CARTESIAN_POINT('Ctrl Pts',(-3.19958362267288,23.920557971337,-12.5936813254797));
#46201=CARTESIAN_POINT('Ctrl Pts',(-3.17937378026934,23.9190680909098,-12.5968296310125));
#46202=CARTESIAN_POINT('Ctrl Pts',(-3.16169016816624,23.9177644455359,-12.5995843983537));
#46203=CARTESIAN_POINT('Ctrl Pts',(-3.14395977964478,23.9164688829369,-12.6023234020356));
#46204=CARTESIAN_POINT('Ctrl Pts',(-3.12618261394994,23.9151815729868,-12.6050462717683));
#46205=CARTESIAN_POINT('Ctrl Pts',(-3.12364301885068,23.9149976715654,-12.6054352531587));
#46206=CARTESIAN_POINT('Ctrl Pts',(-3.11986204396182,23.9147243469594,-12.606013432432));
#46207=CARTESIAN_POINT('Ctrl Pts',(-3.11856096474608,23.9146303745096,-12.6062122270458));
#46208=CARTESIAN_POINT('Ctrl Pts',(-3.09161192130301,23.9126839383508,-12.6103298277411));
#46209=CARTESIAN_POINT('Ctrl Pts',(-3.06343761612503,23.9106765413445,-12.6145811111119));
#46210=CARTESIAN_POINT('Ctrl Pts',(-3.03403807604731,23.9086154043005,-12.6189508233468));
#46211=CARTESIAN_POINT('Ctrl Pts',(-2.96197172541788,23.9035629910819,-12.6296621886687));
#46212=CARTESIAN_POINT('Ctrl Pts',(-2.88254328538339,23.898186158627,-12.6410884371183));
#46213=CARTESIAN_POINT('Ctrl Pts',(-2.79575239027412,23.8926064649136,-12.6529724277651));
#46214=CARTESIAN_POINT('Ctrl Pts',(-2.7092917509017,23.8870480029879,-12.6648111975845));
#46215=CARTESIAN_POINT('Ctrl Pts',(-2.61552433421982,23.8812882565591,-12.6771042612895));
#46216=CARTESIAN_POINT('Ctrl Pts',(-2.51445087260997,23.8754687341903,-12.6895502780204));
#46217=CARTESIAN_POINT('Ctrl Pts',(-2.50259165346356,23.874785914091,-12.6910106023979));
#46218=CARTESIAN_POINT('Ctrl Pts',(-2.49063185611826,23.8741022949286,-12.6924729786301));
#46219=CARTESIAN_POINT('Ctrl Pts',(-2.4785714853039,23.8734181242808,-12.693936876879));
#46220=CARTESIAN_POINT('Ctrl Pts',(-2.37688564609167,23.8676496062509,-12.7062795920612));
#46221=CARTESIAN_POINT('Ctrl Pts',(-2.2680498179562,23.8618405756023,-12.7187343126261));
#46222=CARTESIAN_POINT('Ctrl Pts',(-2.15206279422411,23.8561524998458,-12.7309579520322));
#46223=CARTESIAN_POINT('Ctrl Pts',(-2.11969736791119,23.8545652792169,-12.7343688792872));
#46224=CARTESIAN_POINT('Ctrl Pts',(-2.08677515745332,23.8529875972799,-12.7377615303618));
#46225=CARTESIAN_POINT('Ctrl Pts',(-2.05329625680072,23.8514232415302,-12.7411277890785));
#46226=CARTESIAN_POINT('Ctrl Pts',(-1.97656813203254,23.8478379958737,-12.7488426994781));
#46227=CARTESIAN_POINT('Ctrl Pts',(-1.89691553063701,23.8443225615171,-12.7564195711127));
#46228=CARTESIAN_POINT('Ctrl Pts',(-1.81433840739538,23.8409252166606,-12.7637550190458));
#46229=CARTESIAN_POINT('Ctrl Pts',(-1.81240132437288,23.840845522203,-12.7639270929943));
#46230=CARTESIAN_POINT('Ctrl Pts',(-1.81046263209235,23.8407658927029,-12.7640990337383));
#46231=CARTESIAN_POINT('Ctrl Pts',(-1.80852233053468,23.8406863288454,-12.7642708398867));
#46232=CARTESIAN_POINT('Ctrl Pts',(-1.76910546799746,23.8390700039906,-12.7677610495955));
#46233=CARTESIAN_POINT('Ctrl Pts',(-1.7290244576289,23.8374807582071,-12.7711957460505));
#46234=CARTESIAN_POINT('Ctrl Pts',(-1.68827932271826,23.8359241927331,-12.7745632603602));
#46235=CARTESIAN_POINT('Ctrl Pts',(-1.66690391227081,23.8351075989,-12.7763299007387));
#46236=CARTESIAN_POINT('Ctrl Pts',(-1.64534572150314,23.8342999983825,-12.7780780453442));
#46237=CARTESIAN_POINT('Ctrl Pts',(-1.6236047512744,23.8335022086739,-12.7798059672955));
#46238=CARTESIAN_POINT('Ctrl Pts',(-1.61273426616003,23.8331033138196,-12.7806699282712));
#46239=CARTESIAN_POINT('Ctrl Pts',(-1.60181808614543,23.8327068716212,-12.7815288331432));
#46240=CARTESIAN_POINT('Ctrl Pts',(-1.59085621133314,23.8323129856253,-12.7823824632121));
#46241=CARTESIAN_POINT('Ctrl Pts',(-1.585375273927,23.8321160426274,-12.7828092782465));
#46242=CARTESIAN_POINT('Ctrl Pts',(-1.57988291281928,23.8319197386772,-12.7832347745525));
#46243=CARTESIAN_POINT('Ctrl Pts',(-1.57437912802292,23.8317240868079,-12.7836589246136));
#46244=CARTESIAN_POINT('Ctrl Pts',(-1.56887534322656,23.8315284349386,-12.7840830746747));
#46245=CARTESIAN_POINT('Ctrl Pts',(-1.56205961728679,23.8312877046499,-12.7846050486512));
#46246=CARTESIAN_POINT('Ctrl Pts',(-1.55783350257619,23.8311391004969,-12.7849273084309));
#46247=CARTESIAN_POINT('Ctrl Pts',(-1.33210044392375,23.8232015805096,-12.8021404440734));
#46248=CARTESIAN_POINT('Ctrl Pts',(-1.11005401698134,23.8171220430774,-12.8153351438866));
#46249=CARTESIAN_POINT('Ctrl Pts',(-0.89169728020786,23.8127291140289,-12.8248709020606));
#46250=CARTESIAN_POINT('Ctrl Pts',(-0.848420918716724,23.8118584745958,
-12.8267608044466));
#46251=CARTESIAN_POINT('Ctrl Pts',(-0.805289381652995,23.8110541639786,
-12.8285068870435));
#46252=CARTESIAN_POINT('Ctrl Pts',(-0.762302540745554,23.8103149636894,
-12.8301118046048));
#46253=CARTESIAN_POINT('Ctrl Pts',(-0.724717058268129,23.8096686449804,
-12.8315150619647));
#46254=CARTESIAN_POINT('Ctrl Pts',(-0.687242178941791,23.8090720699838,
-12.8328104033074));
#46255=CARTESIAN_POINT('Ctrl Pts',(-0.649878100570094,23.8085243069343,
-12.8339995799136));
#46256=CARTESIAN_POINT('Ctrl Pts',(-0.558066241026871,23.8071783311641,
-12.836921651601));
#46257=CARTESIAN_POINT('Ctrl Pts',(-0.466923437756322,23.806127042761,-12.8392027737831));
#46258=CARTESIAN_POINT('Ctrl Pts',(-0.376448925310672,23.8053581696707,
-12.8408704275147));
#46259=CARTESIAN_POINT('Ctrl Pts',(-0.31280175564922,23.8048172814723,-12.8420435915045));
#46260=CARTESIAN_POINT('Ctrl Pts',(-0.24948547424537,23.8044160901311,-12.8429131420936));
#46261=CARTESIAN_POINT('Ctrl Pts',(-0.186500081418701,23.8041502793706,
-12.8434883990749));
#46262=CARTESIAN_POINT('Ctrl Pts',(-0.155007385005365,23.8040173739904,
-12.8437760275656));
#46263=CARTESIAN_POINT('Ctrl Pts',(-0.123597410613271,23.8039183134464,
-12.8439900796137));
#46264=CARTESIAN_POINT('Ctrl Pts',(-0.0922701578635517,23.8038525592422,
-12.8441317020657));
#46265=CARTESIAN_POINT('Ctrl Pts',(-0.0647193108532514,23.8037947315087,
-12.8442562523587));
#46266=CARTESIAN_POINT('Ctrl Pts',(-0.0383382413166024,23.8037631765259,
-12.8443236937014));
#46267=CARTESIAN_POINT('Ctrl Pts',(-0.01020945845667,23.8037560879699,-12.8443378683129));
#46268=CARTESIAN_POINT('Ctrl Pts',(-0.00635383481666235,23.8037551163386,
-12.8443398112326));
#46269=CARTESIAN_POINT('Ctrl Pts',(-0.0024653745155048,23.8037546371122,
-12.8443406807256));
#46270=CARTESIAN_POINT('Ctrl Pts',(0.00146343591164922,23.8037546775758,
-12.8443404157537));
#46271=CARTESIAN_POINT('Ctrl Pts',(0.123996040178889,23.803755939565,-12.844332151754));
#46272=CARTESIAN_POINT('Ctrl Pts',(0.246525247851222,23.8042791850219,-12.8432200505871));
#46273=CARTESIAN_POINT('Ctrl Pts',(0.369056161642459,23.8053127715422,-12.8410041049826));
#46274=CARTESIAN_POINT('Ctrl Pts',(0.644870892073421,23.8076393549214,-12.8360160540438));
#46275=CARTESIAN_POINT('Ctrl Pts',(0.920694080264234,23.8125502518664,-12.8254380362402));
#46276=CARTESIAN_POINT('Ctrl Pts',(1.19651513906033,23.8200735682843,-12.8092727889426));
#46277=CARTESIAN_POINT('Ctrl Pts',(1.22211216178672,23.8207717546452,-12.8077726054386));
#46278=CARTESIAN_POINT('Ctrl Pts',(1.2477091679562,23.8214924566863,-12.8062242693096));
#46279=CARTESIAN_POINT('Ctrl Pts',(1.27330614987264,23.8222357071553,-12.8046277624084));
#46280=CARTESIAN_POINT('Ctrl Pts',(1.37082342232289,23.8250672815464,-12.7985455219725));
#46281=CARTESIAN_POINT('Ctrl Pts',(1.4683403440741,23.8282260948037,-12.7917641881055));
#46282=CARTESIAN_POINT('Ctrl Pts',(1.56585686826745,23.8317101405147,-12.7842847836682));
#46283=CARTESIAN_POINT('Ctrl Pts',(1.74017752235782,23.8379382247521,-12.7709145914417));
#46284=CARTESIAN_POINT('Ctrl Pts',(1.91449856143439,23.8452069077848,-12.7553138369756));
#46285=CARTESIAN_POINT('Ctrl Pts',(2.0888191476779,23.8535159164419,-12.7374817690434));
#46286=CARTESIAN_POINT('Ctrl Pts',(2.17523066093796,23.8576347301014,-12.7286423312708));
#46287=CARTESIAN_POINT('Ctrl Pts',(2.26164204571388,23.8620092342545,-12.7192544966263));
#46288=CARTESIAN_POINT('Ctrl Pts',(2.34805359307956,23.8666392625227,-12.7093187482457));
#46289=CARTESIAN_POINT('Ctrl Pts',(2.47841969428531,23.8736244254112,-12.6943290296443));
#46290=CARTESIAN_POINT('Ctrl Pts',(2.60878583461951,23.8811913884393,-12.6780923254294));
#46291=CARTESIAN_POINT('Ctrl Pts',(2.73915198676214,23.889339995395,-12.6606086882267));
#46292=CARTESIAN_POINT('Ctrl Pts',(2.77254322428871,23.8914271327838,-12.6561305298008));
#46293=CARTESIAN_POINT('Ctrl Pts',(2.8059344685154,23.8935524189645,-12.6515705566779));
#46294=CARTESIAN_POINT('Ctrl Pts',(2.83932570101241,23.8957158662664,-12.6469287491679));
#46295=CARTESIAN_POINT('Ctrl Pts',(2.87111753476851,23.8977756871181,-12.642509278497));
#46296=CARTESIAN_POINT('Ctrl Pts',(2.90290935786543,23.8998701009498,-12.6380156251359));
#46297=CARTESIAN_POINT('Ctrl Pts',(2.93470118631675,23.901999091517,-12.6334478145499));
#46298=CARTESIAN_POINT('Ctrl Pts',(2.98358847784925,23.9052729070727,-12.6264237489751));
#46299=CARTESIAN_POINT('Ctrl Pts',(3.03247576591333,23.9086285032369,-12.6192243315775));
#46300=CARTESIAN_POINT('Ctrl Pts',(3.08136305640405,23.912065877191,-12.6118496258009));
#46301=CARTESIAN_POINT('Ctrl Pts',(3.09765881990095,23.913211668509,-12.6093913905421));
#46302=CARTESIAN_POINT('Ctrl Pts',(3.1120376099665,23.9142296217841,-12.6072074384278));
#46303=CARTESIAN_POINT('Ctrl Pts',(3.13025034772233,23.9155305100753,-12.6044164911794));
#46304=CARTESIAN_POINT('Ctrl Pts',(3.2587697411143,23.924710314688,-12.5847219865885));
#46305=CARTESIAN_POINT('Ctrl Pts',(3.38586955228427,23.9344222653021,-12.5640260906196));
#46306=CARTESIAN_POINT('Ctrl Pts',(3.51153601864268,23.9446273099282,-12.5424100887366));
#46307=CARTESIAN_POINT('Ctrl Pts',(3.71379593266574,23.9610523078492,-12.5076191790446));
#46308=CARTESIAN_POINT('Ctrl Pts',(3.91234201511289,23.9787543899613,-12.4704458493914));
#46309=CARTESIAN_POINT('Ctrl Pts',(4.10714050344062,23.9975745994538,-12.431221102725));
#46310=CARTESIAN_POINT('Ctrl Pts',(4.29249186451379,24.015482086699,-12.3938986355705));
#46311=CARTESIAN_POINT('Ctrl Pts',(4.47445059197192,24.0344019634126,-12.3547187661609));
#46312=CARTESIAN_POINT('Ctrl Pts',(4.65300686531934,24.0542044882689,-12.3139537130224));
#46313=CARTESIAN_POINT('Ctrl Pts',(4.83064737904963,24.0739054521314,-12.2733977311686));
#46314=CARTESIAN_POINT('Ctrl Pts',(5.00492039832214,24.0944801390872,-12.2312727514534));
#46315=CARTESIAN_POINT('Ctrl Pts',(5.17583188150985,24.1158107736013,-12.1878325206193));
#46316=CARTESIAN_POINT('Ctrl Pts',(5.35320454393151,24.137947796605,-12.1427500647448));
#46317=CARTESIAN_POINT('Ctrl Pts',(5.52695678608636,24.1608991837852,-12.096251090736));
#46318=CARTESIAN_POINT('Ctrl Pts',(5.6971101511077,24.1845478230226,-12.0486012589137));
#46319=CARTESIAN_POINT('Ctrl Pts',(5.87744252616867,24.2096111844207,-11.9981008921257));
#46320=CARTESIAN_POINT('Ctrl Pts',(6.05373257798032,24.2354580859825,-11.9463079576679));
#46321=CARTESIAN_POINT('Ctrl Pts',(6.22601914496659,24.2619708293824,-11.8935153712287));
#46322=CARTESIAN_POINT('Ctrl Pts',(6.24124268414525,24.2643135412661,-11.8888505269401));
#46323=CARTESIAN_POINT('Ctrl Pts',(6.25643497109608,24.2666614495617,-11.884177863846));
#46324=CARTESIAN_POINT('Ctrl Pts',(6.27159604014383,24.2690144967095,-11.8794975712513));
#46325=CARTESIAN_POINT('Origin',(5.999999999061,24.1259421376201,-10.9277802195584));
#46326=CARTESIAN_POINT('Origin',(5.99996968668368,24.1259230380857,-10.9277552850324));
#46327=CARTESIAN_POINT('Ctrl Pts',(6.25613331744712,13.9489619820917,-8.4284867777746));
#46328=CARTESIAN_POINT('Ctrl Pts',(6.30398162206973,13.9460624564194,-8.4074766351842));
#46329=CARTESIAN_POINT('Ctrl Pts',(6.44264536447383,13.9427640734649,-8.33682408595486));
#46330=CARTESIAN_POINT('Ctrl Pts',(6.65740687788328,13.9634937286633,-8.17768320800854));
#46331=CARTESIAN_POINT('Ctrl Pts',(6.87093031596624,14.0289047773005,-7.9319975038466));
#46332=CARTESIAN_POINT('Ctrl Pts',(7.02371352601407,14.1310161098413,-7.64667378240476));
#46333=CARTESIAN_POINT('Ctrl Pts',(7.09387171678717,14.2445990542294,-7.38242484159179));
#46334=CARTESIAN_POINT('Ctrl Pts',(7.10431447968315,14.32188980161,-7.22230334652378));
#46335=CARTESIAN_POINT('Ctrl Pts',(7.10368173933534,14.3516768211256,-7.16309324424638));
#46336=CARTESIAN_POINT('Ctrl Pts',(6.05827718003039,13.4862137568793,-8.02727938977323));
#46337=CARTESIAN_POINT('Ctrl Pts',(6.10075122454661,13.4833941800054,-8.00882735698102));
#46338=CARTESIAN_POINT('Ctrl Pts',(6.22408246292093,13.479581942238,-7.94671825031444));
#46339=CARTESIAN_POINT('Ctrl Pts',(6.41612732474395,13.4959994652657,-7.80631939831103));
#46340=CARTESIAN_POINT('Ctrl Pts',(6.6081082855051,13.5516701956529,-7.5886512718711));
#46341=CARTESIAN_POINT('Ctrl Pts',(6.74599089454977,13.6405012639782,-7.3352289873818));
#46342=CARTESIAN_POINT('Ctrl Pts',(6.80936980898649,13.7404476399642,-7.10053992025847));
#46343=CARTESIAN_POINT('Ctrl Pts',(6.81876823331771,13.8087304568116,-6.95878686654306));
#46344=CARTESIAN_POINT('Ctrl Pts',(6.81819968063314,13.8350481205052,-6.90649028682641));
#46345=CARTESIAN_POINT('Ctrl Pts',(6.04955572358106,12.8455322123978,-8.08627330790688));
#46346=CARTESIAN_POINT('Ctrl Pts',(6.1079900662572,12.8418918206761,-8.06126216610187));
#46347=CARTESIAN_POINT('Ctrl Pts',(6.27656937354435,12.8375323202349,-7.97762604596949));
#46348=CARTESIAN_POINT('Ctrl Pts',(6.53441767608495,12.861417377942,-7.79202339799651));
#46349=CARTESIAN_POINT('Ctrl Pts',(6.78749235738749,12.9366218552611,-7.50985856325181));
#46350=CARTESIAN_POINT('Ctrl Pts',(6.96695694214048,13.0529645859862,-7.18551418269103));
#46351=CARTESIAN_POINT('Ctrl Pts',(7.04916843852754,13.1817527221056,-6.8862940990644));
#46352=CARTESIAN_POINT('Ctrl Pts',(7.06151642465278,13.2696410515648,-6.70425305611641));
#46353=CARTESIAN_POINT('Ctrl Pts',(7.06076537745517,13.30363561243,-6.63667727119217));
#46354=CARTESIAN_POINT('Ctrl Pts',(6.23560916772017,12.4584536559934,-8.56519010373521));
#46355=CARTESIAN_POINT('Ctrl Pts',(6.32056751352294,12.4536453748849,-8.52892949502008));
#46356=CARTESIAN_POINT('Ctrl Pts',(6.56443955501225,12.4490736721987,-8.40822505546004));
#46357=CARTESIAN_POINT('Ctrl Pts',(6.93220306534565,12.4871642464157,-8.14398300609675));
#46358=CARTESIAN_POINT('Ctrl Pts',(7.28777720473864,12.5979902636432,-7.74834066871077));
#46359=CARTESIAN_POINT('Ctrl Pts',(7.5372435266576,12.7640653483726,-7.29812244537945));
#46360=CARTESIAN_POINT('Ctrl Pts',(7.65118970568607,12.944704829802,-6.88383897116639));
#46361=CARTESIAN_POINT('Ctrl Pts',(7.66849057114655,13.0675783364571,-6.63004784546159));
#46362=CARTESIAN_POINT('Ctrl Pts',(7.66743350755391,13.1152141901136,-6.53531350553332));
#46363=CARTESIAN_POINT('',(7.,13.9487330738339,-6.97709941346537));
#46364=CARTESIAN_POINT('',(7.00000024171084,12.5220639668164,-8.04447769320174));
#46365=CARTESIAN_POINT('Ctrl Pts',(7.,13.9487330738339,-6.97709941346537));
#46366=CARTESIAN_POINT('Ctrl Pts',(7.,13.8474233649361,-7.02089621734514));
#46367=CARTESIAN_POINT('Ctrl Pts',(7.,13.7572507680496,-7.06228070002983));
#46368=CARTESIAN_POINT('Ctrl Pts',(7.,13.6796219035787,-7.10036238057953));
#46369=CARTESIAN_POINT('Ctrl Pts',(7.,13.6408074713433,-7.11940322085437));
#46370=CARTESIAN_POINT('Ctrl Pts',(7.,13.6051028921232,-7.13758106048456));
#46371=CARTESIAN_POINT('Ctrl Pts',(7.,13.5725576246799,-7.15462107918448));
#46372=CARTESIAN_POINT('Ctrl Pts',(7.,13.5562849909583,-7.16314108853445));
#46373=CARTESIAN_POINT('Ctrl Pts',(7.,13.5408011417253,-7.17137543826938));
#46374=CARTESIAN_POINT('Ctrl Pts',(7.,13.5261067530512,-7.17928526244922));
#46375=CARTESIAN_POINT('Ctrl Pts',(7.,13.5187595587141,-7.18324017453914));
#46376=CARTESIAN_POINT('Ctrl Pts',(7.,13.5116097295168,-7.18711395524029));
#46377=CARTESIAN_POINT('Ctrl Pts',(7.,13.5046570157243,-7.19090164180328));
#46378=CARTESIAN_POINT('Ctrl Pts',(7.,13.501180658828,-7.19279548508479));
#46379=CARTESIAN_POINT('Ctrl Pts',(7.,13.497753580783,-7.19466780483175));
#46380=CARTESIAN_POINT('Ctrl Pts',(7.,13.4943757443323,-7.19651798759228));
#46381=CARTESIAN_POINT('Ctrl Pts',(7.,13.4909979078817,-7.19836817035281));
#46382=CARTESIAN_POINT('Ctrl Pts',(7.,13.4891097481019,-7.19940326285153));
#46383=CARTESIAN_POINT('Ctrl Pts',(7.,13.4843899179469,-7.20200151208179));
#46384=CARTESIAN_POINT('Ctrl Pts',(7.,13.4088726354676,-7.24357349976597));
#46385=CARTESIAN_POINT('Ctrl Pts',(7.,13.3376342766462,-7.28583253383395));
#46386=CARTESIAN_POINT('Ctrl Pts',(7.,13.2711782420073,-7.32838772409819));
#46387=CARTESIAN_POINT('Ctrl Pts',(7.,13.2047222073684,-7.37094291436244));
#46388=CARTESIAN_POINT('Ctrl Pts',(7.,13.1443064441612,-7.41284332621996));
#46389=CARTESIAN_POINT('Ctrl Pts',(7.,13.086335335477,-7.45600227764588));
#46390=CARTESIAN_POINT('Ctrl Pts',(7.,12.9703931181087,-7.54232018049772));
#46391=CARTESIAN_POINT('Ctrl Pts',(7.,12.8624564072214,-7.63587433767221));
#46392=CARTESIAN_POINT('Ctrl Pts',(7.,12.7671922400942,-7.73522621634518));
#46393=CARTESIAN_POINT('Ctrl Pts',(7.,12.6719280729671,-7.83457809501815));
#46394=CARTESIAN_POINT('Ctrl Pts',(7.,12.5894712830982,-7.93954794161539));
#46395=CARTESIAN_POINT('Ctrl Pts',(7.,12.5220642584494,-8.04447694179117));
#46396=CARTESIAN_POINT('',(6.24994426646177,12.4626501726359,-8.55169607210683));
#46397=CARTESIAN_POINT('Ctrl Pts',(6.24994458182163,12.4626510719251,-8.55169668917956));
#46398=CARTESIAN_POINT('Ctrl Pts',(6.29730962523071,12.4601998637428,-8.53106267340422));
#46399=CARTESIAN_POINT('Ctrl Pts',(6.34378299838276,12.4587800143928,-8.50904133309007));
#46400=CARTESIAN_POINT('Ctrl Pts',(6.38941189043019,12.4583505508832,-8.48566684378005));
#46401=CARTESIAN_POINT('Ctrl Pts',(6.42007369520999,12.4580619590349,-8.4699596022519));
#46402=CARTESIAN_POINT('Ctrl Pts',(6.45035395481478,12.45822117737,-8.45364039584658));
#46403=CARTESIAN_POINT('Ctrl Pts',(6.48026258827735,12.4588227609006,-8.4367093262394));
#46404=CARTESIAN_POINT('Ctrl Pts',(6.49376528155068,12.4590943546497,-8.42906554538992));
#46405=CARTESIAN_POINT('Ctrl Pts',(6.50719217244104,12.4594561861776,-8.42129694892268));
#46406=CARTESIAN_POINT('Ctrl Pts',(6.5205447379029,12.459907641538,-8.41340334926298));
#46407=CARTESIAN_POINT('Ctrl Pts',(6.58762875903047,12.4621757780263,-8.3737454716921));
#46408=CARTESIAN_POINT('Ctrl Pts',(6.65283225450676,12.4666941319735,-8.3309532994621));
#46409=CARTESIAN_POINT('Ctrl Pts',(6.71587879633085,12.4733990844445,-8.28522333652232));
#46410=CARTESIAN_POINT('Ctrl Pts',(6.73454150082755,12.4753838490804,-8.2716865942951));
#46411=CARTESIAN_POINT('Ctrl Pts',(6.75301492419843,12.4775603607654,-8.25789228705324));
#46412=CARTESIAN_POINT('Ctrl Pts',(6.77129115402012,12.4799273256629,-8.24384519251942));
#46413=CARTESIAN_POINT('Ctrl Pts',(6.81296395481405,12.4853243937466,-8.21181551364404));
#46414=CARTESIAN_POINT('Ctrl Pts',(6.85361150889779,12.4917143765242,-8.17846837699809));
#46415=CARTESIAN_POINT('Ctrl Pts',(6.89323596425004,12.4991044430277,-8.14376490312572));
#46416=CARTESIAN_POINT('Ctrl Pts',(6.89902702850173,12.5001844919411,-8.13869303412045));
#46417=CARTESIAN_POINT('Ctrl Pts',(6.90479617496775,12.5012859442648,-8.13359214701145));
#46418=CARTESIAN_POINT('Ctrl Pts',(6.91054334136795,12.5024088652269,-8.12846207329433));
#46419=CARTESIAN_POINT('Ctrl Pts',(6.94097886456702,12.5083555674127,-8.10129451509989));
#46420=CARTESIAN_POINT('Ctrl Pts',(6.97079915829075,12.5149037297071,-8.0733090443511));
#46421=CARTESIAN_POINT('Ctrl Pts',(7.00000072349027,12.5220628111649,-8.04447789421037));
#46422=CARTESIAN_POINT('',(6.26385803707234,13.9442711326918,-8.42072576609336));
#46423=CARTESIAN_POINT('Origin',(6.52771738877616,13.2547577723573,-9.09520568086109));
#46424=CARTESIAN_POINT('Ctrl Pts',(6.26385550478166,13.9442777501869,-8.42071929290311));
#46425=CARTESIAN_POINT('Ctrl Pts',(6.30452443286976,13.9338444255139,-8.39414427067733));
#46426=CARTESIAN_POINT('Ctrl Pts',(6.34473782035942,13.9244595648097,-8.36476023937334));
#46427=CARTESIAN_POINT('Ctrl Pts',(6.38412017358082,13.9161889610762,-8.33259129990798));
#46428=CARTESIAN_POINT('Ctrl Pts',(6.43028376898849,13.9064942431809,-8.29488319501582));
#46429=CARTESIAN_POINT('Ctrl Pts',(6.47530622992681,13.8983305918767,-8.25334743496533));
#46430=CARTESIAN_POINT('Ctrl Pts',(6.51863204392152,13.8917172362002,-8.20816366664338));
#46431=CARTESIAN_POINT('Ctrl Pts',(6.53236556036768,13.8896209194649,-8.19384121154941));
#46432=CARTESIAN_POINT('Ctrl Pts',(6.54592825180032,13.8876804846815,-8.17915231926784));
#46433=CARTESIAN_POINT('Ctrl Pts',(6.55930139429603,13.8858969140951,-8.16410295969278));
#46434=CARTESIAN_POINT('Ctrl Pts',(6.57612915295727,13.883652602753,-8.14516597528418));
#46435=CARTESIAN_POINT('Ctrl Pts',(6.59265686365932,13.8816566547036,-8.12565821603501));
#46436=CARTESIAN_POINT('Ctrl Pts',(6.60884596028903,13.8799115789078,-8.10559172049823));
#46437=CARTESIAN_POINT('Ctrl Pts',(6.63669630747203,13.8769094986876,-8.07107102547566));
#46438=CARTESIAN_POINT('Ctrl Pts',(6.66354508932836,13.874649698669,-8.03489647221724));
#46439=CARTESIAN_POINT('Ctrl Pts',(6.6892266606921,13.8731171640556,-7.99716821313463));
#46440=CARTESIAN_POINT('Ctrl Pts',(6.7095316520745,13.8719054740979,-7.96733857519326));
#46441=CARTESIAN_POINT('Ctrl Pts',(6.72910683801557,13.8711484558773,-7.93653778302505));
#46442=CARTESIAN_POINT('Ctrl Pts',(6.74786474749874,13.8708408971235,-7.90481678065775));
#46443=CARTESIAN_POINT('Ctrl Pts',(6.75724370224032,13.8706871177466,-7.8889562794741));
#46444=CARTESIAN_POINT('Ctrl Pts',(6.7664182828091,13.8706457384359,-7.87286569376261));
#46445=CARTESIAN_POINT('Ctrl Pts',(6.77537696952256,13.8707163362684,-7.85655154099461));
#46446=CARTESIAN_POINT('Ctrl Pts',(6.7798563128793,13.8707516351847,-7.84839446461061));
#46447=CARTESIAN_POINT('Ctrl Pts',(6.78428167880814,13.8708149310595,-7.8401814940248));
#46448=CARTESIAN_POINT('Ctrl Pts',(6.78865159456431,13.8709061873141,-7.83191343984588));
#46449=CARTESIAN_POINT('Ctrl Pts',(6.78982459935173,13.8709306829861,-7.82969406819763));
#46450=CARTESIAN_POINT('Ctrl Pts',(6.79099360851041,13.8709571933607,-7.82747072784429));
#46451=CARTESIAN_POINT('Ctrl Pts',(6.79215859333577,13.8709857178622,-7.82524343428559));
#46452=CARTESIAN_POINT('Ctrl Pts',(6.79316362759247,13.871010325995,-7.82332194459967));
#46453=CARTESIAN_POINT('Ctrl Pts',(6.79416566671888,13.8710364331518,-7.82139751272386));
#46454=CARTESIAN_POINT('Ctrl Pts',(6.79516469713977,13.8710640359232,-7.81947015226407));
#46455=CARTESIAN_POINT('Ctrl Pts',(6.79696105904224,13.8711136686128,-7.8160045551912));
#46456=CARTESIAN_POINT('Ctrl Pts',(6.79910519164567,13.8711796554962,-7.81182991997246));
#46457=CARTESIAN_POINT('Ctrl Pts',(6.80070351406485,13.8712333795176,-7.80869388659622));
#46458=CARTESIAN_POINT('Ctrl Pts',(6.80102444344323,13.8712441668384,-7.80806419809912));
#46459=CARTESIAN_POINT('Ctrl Pts',(6.80132350624074,13.871254386852,-7.80747646908176));
#46460=CARTESIAN_POINT('Ctrl Pts',(6.80159364688567,13.8712637147728,-7.80694495668783));
#46461=CARTESIAN_POINT('Ctrl Pts',(6.81852791122845,13.8718484526873,-7.77362612240944));
#46462=CARTESIAN_POINT('Ctrl Pts',(6.8351307337105,13.8728723168352,-7.73832342759663));
#46463=CARTESIAN_POINT('Ctrl Pts',(6.85111676556959,13.8744191424824,-7.7010006024349));
#46464=CARTESIAN_POINT('Ctrl Pts',(6.86624053184969,13.8758825343843,-7.66569092148123));
#46465=CARTESIAN_POINT('Ctrl Pts',(6.88081240248914,13.8778139223046,-7.62857313319346));
#46466=CARTESIAN_POINT('Ctrl Pts',(6.894553421665,13.8802837333051,-7.58964285657535));
#46467=CARTESIAN_POINT('Ctrl Pts',(6.90444958100783,13.8820624691393,-7.56160561888994));
#46468=CARTESIAN_POINT('Ctrl Pts',(6.91391408924983,13.8841204526936,-7.5326288089318));
#46469=CARTESIAN_POINT('Ctrl Pts',(6.92282868318488,13.886484152877,-7.50272017513952));
#46470=CARTESIAN_POINT('Ctrl Pts',(6.92839424746096,13.8879598594987,-7.48404760014695));
#46471=CARTESIAN_POINT('Ctrl Pts',(6.93374517006024,13.8895547576781,-7.46501194873757));
#46472=CARTESIAN_POINT('Ctrl Pts',(6.93885429742972,13.8912731958799,-7.44561960630978));
#46473=CARTESIAN_POINT('Ctrl Pts',(6.94955798596152,13.8948733463444,-7.4049923957828));
#46474=CARTESIAN_POINT('Ctrl Pts',(6.95920279168186,13.8990160099639,-7.36279719266331));
#46475=CARTESIAN_POINT('Ctrl Pts',(6.96751456368846,13.9037380721181,-7.31911914123901));
#46476=CARTESIAN_POINT('Ctrl Pts',(6.97543732765642,13.9082391320437,-7.27748531252707));
#46477=CARTESIAN_POINT('Ctrl Pts',(6.98214922820788,13.9132665333231,-7.23450421686683));
#46478=CARTESIAN_POINT('Ctrl Pts',(6.98737818945742,13.9188495108828,-7.19028269317926));
#46479=CARTESIAN_POINT('Ctrl Pts',(6.9882530277002,13.9197835782902,-7.18288415296647));
#46480=CARTESIAN_POINT('Ctrl Pts',(6.98908626773821,13.9207331924292,-7.17545096943005));
#46481=CARTESIAN_POINT('Ctrl Pts',(6.98987652405541,13.9216984850986,-7.16798373863768));
#46482=CARTESIAN_POINT('Ctrl Pts',(6.9944022584873,13.9272266386557,-7.12521950787827));
#46483=CARTESIAN_POINT('Ctrl Pts',(6.99752057952379,13.9332694552473,-7.08133542937894));
#46484=CARTESIAN_POINT('Ctrl Pts',(6.99900427208156,13.9398281691519,-7.0364929204224));
#46485=CARTESIAN_POINT('Ctrl Pts',(6.99965344019274,13.9426978390811,-7.01687273247491));
#46486=CARTESIAN_POINT('Ctrl Pts',(6.99998929454039,13.9456662025399,-6.99706957208411));
#46487=CARTESIAN_POINT('Ctrl Pts',(6.99999076617782,13.9487330740186,-6.97709941303822));
#46488=CARTESIAN_POINT('Ctrl Pts',(6.99990203904237,13.888165173065,-6.87914443466826));
#46489=CARTESIAN_POINT('Ctrl Pts',(6.99990203904237,14.0922362660489,-7.13651751059625));
#46490=CARTESIAN_POINT('Ctrl Pts',(6.99990203904237,14.6760299602152,-7.80837580698534));
#46491=CARTESIAN_POINT('Ctrl Pts',(6.99990203904237,15.7555631911401,-8.78348152161194));
#46492=CARTESIAN_POINT('Ctrl Pts',(6.99990203904237,17.1681328395499,-9.70998929655117));
#46493=CARTESIAN_POINT('Ctrl Pts',(6.99990203904237,18.707836621519,-10.4111877922339));
#46494=CARTESIAN_POINT('Ctrl Pts',(6.99990203904237,20.3372593085727,-10.8675483426642));
#46495=CARTESIAN_POINT('Ctrl Pts',(6.99990203904237,22.0150966880212,-11.0696763778178));
#46496=CARTESIAN_POINT('Ctrl Pts',(6.99990203904237,23.3220446342241,-11.0250212390944));
#46497=CARTESIAN_POINT('Ctrl Pts',(6.99990203904237,24.0577248833002,-10.9251639976814));
#46498=CARTESIAN_POINT('Ctrl Pts',(6.99990203904237,24.2367456444932,-10.8963436960955));
#46499=CARTESIAN_POINT('Ctrl Pts',(7.00657991031323,13.5143482295687,-7.17552474229237));
#46500=CARTESIAN_POINT('Ctrl Pts',(7.00657991031323,13.7273208138437,-7.44412675674585));
#46501=CARTESIAN_POINT('Ctrl Pts',(7.00657991031323,14.3364361714447,-8.14510512450419));
#46502=CARTESIAN_POINT('Ctrl Pts',(7.00657991031323,15.4627111247065,-9.16244330636057));
#46503=CARTESIAN_POINT('Ctrl Pts',(7.00657991031323,16.9369683207059,-10.1294536145601));
#46504=CARTESIAN_POINT('Ctrl Pts',(7.00657991031323,18.5435357472038,-10.8610425695369));
#46505=CARTESIAN_POINT('Ctrl Pts',(7.00657991031323,20.2436295715865,-11.3372508338949));
#46506=CARTESIAN_POINT('Ctrl Pts',(7.00657991031323,21.9947633032354,-11.5481745874969));
#46507=CARTESIAN_POINT('Ctrl Pts',(7.00657991031323,23.3582294831803,-11.5015779615709));
#46508=CARTESIAN_POINT('Ctrl Pts',(7.00657991031323,24.1257769274139,-11.3974033892945));
#46509=CARTESIAN_POINT('Ctrl Pts',(7.00657991031323,24.3125682645583,-11.3673328815837));
#46510=CARTESIAN_POINT('Ctrl Pts',(6.71852921530218,13.2161068334526,-7.41198506936298));
#46511=CARTESIAN_POINT('Ctrl Pts',(6.71852921530218,13.4361812712895,-7.68954583852755));
#46512=CARTESIAN_POINT('Ctrl Pts',(6.71852921530218,14.0654989455187,-8.41375699680662));
#46513=CARTESIAN_POINT('Ctrl Pts',(6.71852921530218,15.2290657250872,-9.46478939774906));
#46514=CARTESIAN_POINT('Ctrl Pts',(6.71852921530218,16.752538936138,-10.4641137363018));
#46515=CARTESIAN_POINT('Ctrl Pts',(6.71852921530218,18.4124520095801,-11.2199490320946));
#46516=CARTESIAN_POINT('Ctrl Pts',(6.71852921530218,20.1689292029679,-11.7119923462326));
#46517=CARTESIAN_POINT('Ctrl Pts',(6.71852921530218,21.978540771934,-11.929933564917));
#46518=CARTESIAN_POINT('Ctrl Pts',(6.71852921530218,23.3870987467495,-11.8817879673256));
#46519=CARTESIAN_POINT('Ctrl Pts',(6.71852921530218,24.180070712107,-11.7741689102501));
#46520=CARTESIAN_POINT('Ctrl Pts',(6.71852921530218,24.3730616275822,-11.7431009538378));
#46521=CARTESIAN_POINT('Ctrl Pts',(6.25703473519962,13.1199246148395,-7.48824302405876));
#46522=CARTESIAN_POINT('Ctrl Pts',(6.25703473519962,13.3422893854061,-7.7686929726366));
#46523=CARTESIAN_POINT('Ctrl Pts',(6.25703473519962,13.978122263964,-8.50039665665675));
#46524=CARTESIAN_POINT('Ctrl Pts',(6.25703473519962,15.153715578534,-9.56229537189375));
#46525=CARTESIAN_POINT('Ctrl Pts',(6.25703473519962,16.6930608502105,-10.5720409168031));
#46526=CARTESIAN_POINT('Ctrl Pts',(6.25703473519962,18.3701777818156,-11.3356956061556));
#46527=CARTESIAN_POINT('Ctrl Pts',(6.25703473519962,20.1448384922945,-11.8328456903125));
#46528=CARTESIAN_POINT('Ctrl Pts',(6.25703473519962,21.973309039948,-12.0530500266267));
#46529=CARTESIAN_POINT('Ctrl Pts',(6.25703473519962,23.3964090231084,-12.0044048889509));
#46530=CARTESIAN_POINT('Ctrl Pts',(6.25703473519962,24.197580342684,-11.895674992817));
#46531=CARTESIAN_POINT('Ctrl Pts',(6.25703473519962,24.3925706090388,-11.8642853613214));
#46532=CARTESIAN_POINT('Ctrl Pts',(6.99999999999956,13.9487330738349,-6.97709941346457));
#46533=CARTESIAN_POINT('Ctrl Pts',(6.99999999999956,14.053386251496,-7.10629498286879));
#46534=CARTESIAN_POINT('Ctrl Pts',(6.99999999999324,14.1606435018721,-7.23273587370856));
#46535=CARTESIAN_POINT('Ctrl Pts',(6.99999999940879,14.2705233076618,-7.35652129864407));
#46536=CARTESIAN_POINT('Ctrl Pts',(6.999999998967,14.3535805484897,-7.45008968253378));
#46537=CARTESIAN_POINT('Ctrl Pts',(6.99999999822953,14.4381371927886,-7.54214022916443));
#46538=CARTESIAN_POINT('Ctrl Pts',(6.99999999797983,14.5242162277568,-7.63270296562204));
#46539=CARTESIAN_POINT('Ctrl Pts',(6.99999999764853,14.6384202201537,-7.75285563775258));
#46540=CARTESIAN_POINT('Ctrl Pts',(6.99999999919476,14.7553029036892,-7.87039100103324));
#46541=CARTESIAN_POINT('Ctrl Pts',(6.99999999987613,14.8749736388849,-7.98536856617627));
#46542=CARTESIAN_POINT('Ctrl Pts',(6.99999999995181,14.8882664665725,-7.99814008428295));
#46543=CARTESIAN_POINT('Ctrl Pts',(6.99999999999965,14.9015937278416,-8.0108800022357));
#46544=CARTESIAN_POINT('Ctrl Pts',(6.99999999999965,14.9149555972393,-8.02358837040624));
#46545=CARTESIAN_POINT('Ctrl Pts',(6.99999999999965,15.0622915543763,-8.16371843247603));
#46546=CARTESIAN_POINT('Ctrl Pts',(6.99999999555913,15.2137650538499,-8.3000557814469));
#46547=CARTESIAN_POINT('Ctrl Pts',(6.99999999493045,15.3690240498991,-8.43218410937023));
#46548=CARTESIAN_POINT('Ctrl Pts',(6.99999999439676,15.50082389845,-8.54434826122432));
#46549=CARTESIAN_POINT('Ctrl Pts',(6.9999999961049,15.6353509161497,-8.65347965096803));
#46550=CARTESIAN_POINT('Ctrl Pts',(6.99999999794295,15.7723688449927,-8.75934441784532));
#46551=CARTESIAN_POINT('Ctrl Pts',(6.99999999899899,15.8510917690786,-8.82016845800282));
#46552=CARTESIAN_POINT('Ctrl Pts',(6.99999999999965,15.9306366045598,-8.87991455028249));
#46553=CARTESIAN_POINT('Ctrl Pts',(6.99999999999965,16.0109493844193,-8.9385489450054));
#46554=CARTESIAN_POINT('Ctrl Pts',(6.99999999999965,16.2224433271297,-9.09295549574484));
#46555=CARTESIAN_POINT('Ctrl Pts',(6.99999999747041,16.4393240289556,-9.23958606259355));
#46556=CARTESIAN_POINT('Ctrl Pts',(6.99999999839021,16.661113395121,-9.37826165929473));
#46557=CARTESIAN_POINT('Ctrl Pts',(6.99999999909794,16.8317700681298,-9.48496612565262));
#46558=CARTESIAN_POINT('Ctrl Pts',(6.99999999994318,17.0053339299189,-9.58696026447865));
#46559=CARTESIAN_POINT('Ctrl Pts',(6.9999999999948,17.1816030196623,-9.6841487567417));
#46560=CARTESIAN_POINT('Ctrl Pts',(6.99999999999814,17.1930137959965,-9.69044025202934));
#46561=CARTESIAN_POINT('Ctrl Pts',(6.99999999999965,17.2044359132746,-9.69671160410671));
#46562=CARTESIAN_POINT('Ctrl Pts',(6.99999999999965,17.2158693153257,-9.70296278908558));
#46563=CARTESIAN_POINT('Ctrl Pts',(6.99999999999964,17.5300710084143,-9.87475180650998));
#46564=CARTESIAN_POINT('Ctrl Pts',(7.00000000000802,17.8527744443978,-10.0313270806561));
#46565=CARTESIAN_POINT('Ctrl Pts',(6.99999999997833,18.1824069034162,-10.1717696536148));
#46566=CARTESIAN_POINT('Ctrl Pts',(6.99999999996856,18.2908723305482,-10.2179822253646));
#46567=CARTESIAN_POINT('Ctrl Pts',(6.99999999999964,18.4000875899428,-10.2624481862356));
#46568=CARTESIAN_POINT('Ctrl Pts',(6.99999999999964,18.5099955100176,-10.3051352656413));
#46569=CARTESIAN_POINT('Ctrl Pts',(6.99999999999964,18.5790288315156,-10.3319470811539));
#46570=CARTESIAN_POINT('Ctrl Pts',(6.99999999997185,18.6483347586902,-10.3580596457169));
#46571=CARTESIAN_POINT('Ctrl Pts',(6.99999999993251,18.7178989046704,-10.3834658744547));
#46572=CARTESIAN_POINT('Ctrl Pts',(6.99999999971885,19.0956724624964,-10.5214363948426));
#46573=CARTESIAN_POINT('Ctrl Pts',(6.99999999999965,19.481061546552,-10.6385715529277));
#46574=CARTESIAN_POINT('Ctrl Pts',(6.99999999999965,19.8715517335095,-10.73431644707));
#46575=CARTESIAN_POINT('Ctrl Pts',(6.99999999999965,20.0280805593397,-10.772695992472));
#46576=CARTESIAN_POINT('Ctrl Pts',(6.99999999962334,20.1854297801842,-10.8076370879262));
#46577=CARTESIAN_POINT('Ctrl Pts',(6.99999999912728,20.3434768183341,-10.8391033410566));
#46578=CARTESIAN_POINT('Ctrl Pts',(6.99999999825512,20.6213539562873,-10.8944270754608));
#46579=CARTESIAN_POINT('Ctrl Pts',(6.99999999886831,20.9013888478931,-10.9390121158806));
#46580=CARTESIAN_POINT('Ctrl Pts',(6.99999999982003,21.1829146752606,-10.9726760530095));
#46581=CARTESIAN_POINT('Ctrl Pts',(6.99999999992606,21.2142778778935,-10.9764263621426));
#46582=CARTESIAN_POINT('Ctrl Pts',(6.99999999999964,21.2456595741147,-10.9800410779504));
#46583=CARTESIAN_POINT('Ctrl Pts',(6.99999999999964,21.2770588331736,-10.9835199089928));
#46584=CARTESIAN_POINT('Ctrl Pts',(6.99999999999964,21.4969229007099,-11.0078793991896));
#46585=CARTESIAN_POINT('Ctrl Pts',(6.99999999634621,21.7176500295301,-11.0256227319415));
#46586=CARTESIAN_POINT('Ctrl Pts',(6.99999999542167,21.9386318391872,-11.036675632778));
#46587=CARTESIAN_POINT('Ctrl Pts',(6.99999999531138,21.9649927459056,-11.0379941326508));
#46588=CARTESIAN_POINT('Ctrl Pts',(6.99999999523597,21.9913572760442,-11.0392174880406));
#46589=CARTESIAN_POINT('Ctrl Pts',(6.99999999520045,22.0177243973286,-11.0403456225131));
#46590=CARTESIAN_POINT('Ctrl Pts',(6.99999999489241,22.246398142798,-11.0501295777824));
#46591=CARTESIAN_POINT('Ctrl Pts',(6.99999999999965,22.4752661616617,-11.0527466161651));
#46592=CARTESIAN_POINT('Ctrl Pts',(6.99999999999965,22.703659797635,-11.048298338829));
#46593=CARTESIAN_POINT('Ctrl Pts',(6.99999999999965,22.873857685662,-11.0449835029986));
#46594=CARTESIAN_POINT('Ctrl Pts',(6.99999999741394,23.0437838324152,-11.0376888894721));
#46595=CARTESIAN_POINT('Ctrl Pts',(6.99999999745697,23.2135387084807,-11.0264498585388));
#46596=CARTESIAN_POINT('Ctrl Pts',(6.99999999749804,23.3755780199356,-11.0157216551667));
#46597=CARTESIAN_POINT('Ctrl Pts',(6.99999999865098,23.537461613108,-11.0013990881958));
#46598=CARTESIAN_POINT('Ctrl Pts',(6.99999999924031,23.6992764926518,-10.9834686168323));
#46599=CARTESIAN_POINT('Ctrl Pts',(6.99999999975841,23.8415378782003,-10.9677048396884));
#46600=CARTESIAN_POINT('Ctrl Pts',(6.99999999990827,23.9837463384243,-10.9491517994266));
#46601=CARTESIAN_POINT('Ctrl Pts',(6.99999999989361,24.1259362011698,-10.9277733096369));
#46602=CARTESIAN_POINT('Ctrl Pts',(6.26386081918706,13.9442638622873,-8.42073287772094));
#46603=CARTESIAN_POINT('Ctrl Pts',(6.26460715582258,14.1256644813049,-8.60589482522455));
#46604=CARTESIAN_POINT('Ctrl Pts',(6.26531568264654,14.3114848731865,-8.78358359448678));
#46605=CARTESIAN_POINT('Ctrl Pts',(6.26598638276582,14.5010844523376,-8.95374253421015));
#46606=CARTESIAN_POINT('Ctrl Pts',(6.26666473223493,14.6928464189228,-9.1258421404408));
#46607=CARTESIAN_POINT('Ctrl Pts',(6.26730438727457,14.8884742964778,-9.29023923288897));
#46608=CARTESIAN_POINT('Ctrl Pts',(6.26790533375421,15.087347270408,-9.44690789015415));
#46609=CARTESIAN_POINT('Ctrl Pts',(6.2680017616388,15.1192584319309,-9.47204694614937));
#46610=CARTESIAN_POINT('Ctrl Pts',(6.26809719288439,15.1512532324775,-9.49698708152831));
#46611=CARTESIAN_POINT('Ctrl Pts',(6.26819162743985,15.1833292053893,-9.52172826496564));
#46612=CARTESIAN_POINT('Ctrl Pts',(6.26876871395664,15.3793444393205,-9.67292083744168));
#46613=CARTESIAN_POINT('Ctrl Pts',(6.26930857994914,15.5783869659425,-9.81668210430068));
#46614=CARTESIAN_POINT('Ctrl Pts',(6.26981121523602,15.7798024932585,-9.95308866259111));
#46615=CARTESIAN_POINT('Ctrl Pts',(6.27017912285584,15.9272300797869,-10.0529324529055));
#46616=CARTESIAN_POINT('Ctrl Pts',(6.27052708374744,16.0759300700406,-10.1488363157099));
#46617=CARTESIAN_POINT('Ctrl Pts',(6.27085509470647,16.22566217413,-10.2408371004955));
#46618=CARTESIAN_POINT('Ctrl Pts',(6.27121137913853,16.3883006964033,-10.3407680523546));
#46619=CARTESIAN_POINT('Ctrl Pts',(6.27154412491034,16.5521567025934,-10.4360939682438));
#46620=CARTESIAN_POINT('Ctrl Pts',(6.27185332794175,16.716940010019,-10.5268693882174));
#46621=CARTESIAN_POINT('Ctrl Pts',(6.27227096943169,16.939513332523,-10.6494800284631));
#46622=CARTESIAN_POINT('Ctrl Pts',(6.2726456594972,17.1637763762107,-10.7637884182362));
#46623=CARTESIAN_POINT('Ctrl Pts',(6.27297739020537,17.3890721242152,-10.8699988364842));
#46624=CARTESIAN_POINT('Ctrl Pts',(6.27330912091355,17.6143678722197,-10.9762092547322));
#46625=CARTESIAN_POINT('Ctrl Pts',(6.27359789228358,17.8406965014528,-11.0743217864376));
#46626=CARTESIAN_POINT('Ctrl Pts',(6.27384369852514,18.0674570588809,-11.1645574428798));
#46627=CARTESIAN_POINT('Ctrl Pts',(6.27395596459215,18.1710244694238,-11.2057704006462));
#46628=CARTESIAN_POINT('Ctrl Pts',(6.27405926826201,18.2746827342572,-11.2453404763723));
#46629=CARTESIAN_POINT('Ctrl Pts',(6.27415361615965,18.378378353274,-11.2832898174722));
#46630=CARTESIAN_POINT('Ctrl Pts',(6.27415651998732,18.3815698839283,-11.2844578174955));
#46631=CARTESIAN_POINT('Ctrl Pts',(6.27415941527061,18.3847614500127,-11.2856242822539));
#46632=CARTESIAN_POINT('Ctrl Pts',(6.27416230201534,18.3879530500141,-11.2867892124062));
#46633=CARTESIAN_POINT('Ctrl Pts',(6.2742063116997,18.4366103860962,-11.3045490814075));
#46634=CARTESIAN_POINT('Ctrl Pts',(6.27424833682322,18.4852755954915,-11.3219522716654));
#46635=CARTESIAN_POINT('Ctrl Pts',(6.27428839799666,18.5339430794972,-11.3390020011574));
#46636=CARTESIAN_POINT('Ctrl Pts',(6.27431785037792,18.5697226927903,-11.3515367097095));
#46637=CARTESIAN_POINT('Ctrl Pts',(6.27434670195756,18.6061342225264,-11.3640966709816));
#46638=CARTESIAN_POINT('Ctrl Pts',(6.27437398859951,18.6418706456722,-11.3762337368752));
#46639=CARTESIAN_POINT('Ctrl Pts',(6.27438625180983,18.6579313714314,-11.3816883982454));
#46640=CARTESIAN_POINT('Ctrl Pts',(6.27439819893397,18.6738555054533,-11.3870583204017));
#46641=CARTESIAN_POINT('Ctrl Pts',(6.2744097424524,18.6895233175027,-11.3923060605731));
#46642=CARTESIAN_POINT('Ctrl Pts',(6.2745606466654,18.8943429191852,-11.4609078569345));
#46643=CARTESIAN_POINT('Ctrl Pts',(6.27467736471317,19.1037515567848,-11.5248695127819));
#46644=CARTESIAN_POINT('Ctrl Pts',(6.27475989485597,19.317573690524,-11.5836612029585));
#46645=CARTESIAN_POINT('Ctrl Pts',(6.2748410715206,19.5278891831466,-11.6414887209304));
#46646=CARTESIAN_POINT('Ctrl Pts',(6.27488917244077,19.7424746815811,-11.6943144438987));
#46647=CARTESIAN_POINT('Ctrl Pts',(6.27490419693318,19.9611183014331,-11.7416108905639));
#46648=CARTESIAN_POINT('Ctrl Pts',(6.27490863072152,20.0256409159614,-11.7555682628339));
#46649=CARTESIAN_POINT('Ctrl Pts',(6.27491018400937,20.0905166317593,-11.7690439544347));
#46650=CARTESIAN_POINT('Ctrl Pts',(6.27490885679481,20.1557392228451,-11.7820240144788));
#46651=CARTESIAN_POINT('Ctrl Pts',(6.27490450834956,20.369432529316,-11.8245514869826));
#46652=CARTESIAN_POINT('Ctrl Pts',(6.27486923880992,20.5868530263642,-11.861759892537));
#46653=CARTESIAN_POINT('Ctrl Pts',(6.27480304864361,20.807724782831,-11.8931692264645));
#46654=CARTESIAN_POINT('Ctrl Pts',(6.27475277000862,20.9755009200281,-11.917028033958));
#46655=CARTESIAN_POINT('Ctrl Pts',(6.27468465001575,21.1452675351015,-11.9375403860185));
#46656=CARTESIAN_POINT('Ctrl Pts',(6.27459868919133,21.3168848037213,-11.9544888514541));
#46657=CARTESIAN_POINT('Ctrl Pts',(6.27448994471055,21.5339887099896,-11.975929456359));
#46658=CARTESIAN_POINT('Ctrl Pts',(6.27435264765825,21.7540558527808,-11.9916671410961));
#46659=CARTESIAN_POINT('Ctrl Pts',(6.27418680051457,21.9767636838208,-12.0012474184625));
#46660=CARTESIAN_POINT('Ctrl Pts',(6.27401315051287,22.2099495824815,-12.0112784334326));
#46661=CARTESIAN_POINT('Ctrl Pts',(6.27380820073295,22.4460306168683,-12.0145579480249));
#46662=CARTESIAN_POINT('Ctrl Pts',(6.27357195495289,22.6846268922175,-12.0106606315315));
#46663=CARTESIAN_POINT('Ctrl Pts',(6.27333930220717,22.9195943848128,-12.0068225888672));
#46664=CARTESIAN_POINT('Ctrl Pts',(6.2730762981723,23.1570012478186,-11.996024327057));
#46665=CARTESIAN_POINT('Ctrl Pts',(6.27278294744759,23.3964344665696,-11.9778551667814));
#46666=CARTESIAN_POINT('Ctrl Pts',(6.27261681610617,23.5320310697448,-11.9675655485371));
#46667=CARTESIAN_POINT('Ctrl Pts',(6.27244095193068,23.6682766505981,-11.9549118418849));
#46668=CARTESIAN_POINT('Ctrl Pts',(6.27225535591025,23.8050887673702,-11.9398188606727));
#46669=CARTESIAN_POINT('Ctrl Pts',(6.27204648314437,23.9590593383348,-11.9228329752875));
#46670=CARTESIAN_POINT('Ctrl Pts',(6.27182528439318,24.1137477394466,-11.9027576366664));
#46671=CARTESIAN_POINT('Ctrl Pts',(6.27159176124975,24.2690119676725,-11.8794807215117));
#46672=CARTESIAN_POINT('Ctrl Pts',(-6.390310997178,13.7249660550952,-8.13937950338793));
#46673=CARTESIAN_POINT('Ctrl Pts',(-4.260207331452,13.8221738588746,-9.11426650158688));
#46674=CARTESIAN_POINT('Ctrl Pts',(0.0001535202327188,13.918298461743,-10.0902631574918));
#46675=CARTESIAN_POINT('Ctrl Pts',(4.260514371917,13.8221669310088,-9.11419615982883));
#46676=CARTESIAN_POINT('Ctrl Pts',(6.390771557876,13.7249450365303,-8.13916871045812));
#46677=CARTESIAN_POINT('Ctrl Pts',(-6.390310997178,14.2543287817271,-8.71309690459039));
#46678=CARTESIAN_POINT('Ctrl Pts',(-4.260207331452,14.3567676707027,-9.62713419180366));
#46679=CARTESIAN_POINT('Ctrl Pts',(0.0001535202327188,14.4578350530778,
-10.5425537312138));
#46680=CARTESIAN_POINT('Ctrl Pts',(4.260514371917,14.3567603866034,-9.62706821594453));
#46681=CARTESIAN_POINT('Ctrl Pts',(6.390771557876,14.2543066320775,-8.71289926876272));
#46682=CARTESIAN_POINT('Ctrl Pts',(-6.390310997178,15.6641218054918,-9.96973300997693));
#46683=CARTESIAN_POINT('Ctrl Pts',(-4.260207331452,15.7526919792829,-10.7489906364333));
#46684=CARTESIAN_POINT('Ctrl Pts',(0.0001535202327188,15.8421753984554,
-11.5273040839069));
#46685=CARTESIAN_POINT('Ctrl Pts',(4.260514371917,15.752685530061,-10.7489345420424));
#46686=CARTESIAN_POINT('Ctrl Pts',(6.390771557876,15.6641026545996,-9.96956451659077));
#46687=CARTESIAN_POINT('Ctrl Pts',(-6.390310997178,18.3168609125034,-11.3879809585253));
#46688=CARTESIAN_POINT('Ctrl Pts',(-4.260207331452,18.305065900394,-12.0191857141961));
#46689=CARTESIAN_POINT('Ctrl Pts',(0.0001535202327188,18.2929947853426,
-12.6510838649568));
#46690=CARTESIAN_POINT('Ctrl Pts',(4.260514371917,18.3050667703745,-12.0191401722118));
#46691=CARTESIAN_POINT('Ctrl Pts',(6.390771557876,18.3168634628528,-11.3878444775859));
#46692=CARTESIAN_POINT('Ctrl Pts',(-6.390310997178,21.4528914163287,-12.0713618431433));
#46693=CARTESIAN_POINT('Ctrl Pts',(-4.260207331452,21.2792389757137,-12.6592425324047));
#46694=CARTESIAN_POINT('Ctrl Pts',(0.0001535202327188,21.1056340488841,
-13.2456889758127));
#46695=CARTESIAN_POINT('Ctrl Pts',(4.260514371917,21.2792514877189,-12.6592002662047));
#46696=CARTESIAN_POINT('Ctrl Pts',(6.390771557876,21.4529289639727,-12.071234729827));
#46697=CARTESIAN_POINT('Ctrl Pts',(-6.390310997178,23.5458951845797,-11.9720502124699));
#46698=CARTESIAN_POINT('Ctrl Pts',(-4.260207331452,23.2652553028773,-12.6077625569466));
#46699=CARTESIAN_POINT('Ctrl Pts',(0.0001535202327188,22.9846380445226,
-13.2461450660854));
#46700=CARTESIAN_POINT('Ctrl Pts',(4.260514371917,23.265275527447,-12.607716547628));
#46701=CARTESIAN_POINT('Ctrl Pts',(6.390771557876,23.5459558653553,-11.9719127568894));
#46702=CARTESIAN_POINT('Ctrl Pts',(-6.390310997178,24.5118462831574,-11.8061936876057));
#46703=CARTESIAN_POINT('Ctrl Pts',(-4.260207331452,24.1870546128076,-12.4817978962268));
#46704=CARTESIAN_POINT('Ctrl Pts',(0.0001535202327188,23.8622603664262,
-13.1582606881552));
#46705=CARTESIAN_POINT('Ctrl Pts',(4.260514371917,24.1870780212844,-12.4817491423853));
#46706=CARTESIAN_POINT('Ctrl Pts',(6.390771557876,24.5119165105666,-11.8060476064867));
#46707=CARTESIAN_POINT('Ctrl Pts',(-6.26386059966982,13.9442583573344,-8.42071137120996));
#46708=CARTESIAN_POINT('Ctrl Pts',(-5.97465264562961,13.9555888069264,-8.54542713090756));
#46709=CARTESIAN_POINT('Ctrl Pts',(-5.68350292691887,13.9652820825191,-8.66149310003109));
#46710=CARTESIAN_POINT('Ctrl Pts',(-5.3909022605167,13.9735953815832,-8.76876193425704));
#46711=CARTESIAN_POINT('Ctrl Pts',(-5.11637639590315,13.981395143769,-8.86940445781674));
#46712=CARTESIAN_POINT('Ctrl Pts',(-4.84057330552681,13.9879803358116,-8.96230247036302));
#46713=CARTESIAN_POINT('Ctrl Pts',(-4.56389835177543,13.9935747005038,-9.04737600273165));
#46714=CARTESIAN_POINT('Ctrl Pts',(-4.30687417419982,13.9987717267058,-9.12640720665533));
#46715=CARTESIAN_POINT('Ctrl Pts',(-4.04909758291724,14.0031137981319,-9.19868567286897));
#46716=CARTESIAN_POINT('Ctrl Pts',(-3.79089355733771,14.0067883134942,-9.26419037750946));
#46717=CARTESIAN_POINT('Ctrl Pts',(-3.57421217307386,14.0098719179168,-9.31916105445936));
#46718=CARTESIAN_POINT('Ctrl Pts',(-3.35722977490934,14.0124855440924,-9.36936192851386));
#46719=CARTESIAN_POINT('Ctrl Pts',(-3.14013842049977,14.0147440106155,-9.41480879995396));
#46720=CARTESIAN_POINT('Ctrl Pts',(-2.90223992213209,14.0172189401027,-9.46461153162198));
#46721=CARTESIAN_POINT('Ctrl Pts',(-2.66419710898026,14.0192828053626,-9.50872061924435));
#46722=CARTESIAN_POINT('Ctrl Pts',(-2.42625893543512,14.0209898784393,-9.54710744779563));
#46723=CARTESIAN_POINT('Ctrl Pts',(-2.19167929327942,14.0226728559351,-9.58495244076538));
#46724=CARTESIAN_POINT('Ctrl Pts',(-1.95720135757247,14.0240090622126,-9.61723553947319));
#46725=CARTESIAN_POINT('Ctrl Pts',(-1.72306368872734,14.0250552895158,-9.6439797497153));
#46726=CARTESIAN_POINT('Ctrl Pts',(-1.49041851325521,14.0260948477199,-9.67055348095356));
#46727=CARTESIAN_POINT('Ctrl Pts',(-1.25810928045884,14.0268481255946,-9.69165864347421));
#46728=CARTESIAN_POINT('Ctrl Pts',(-1.02637001771251,14.027375357038,-9.70736883014928));
#46729=CARTESIAN_POINT('Ctrl Pts',(-0.796211217154453,14.0278989927621,
-9.722971873323));
#46730=CARTESIAN_POINT('Ctrl Pts',(-0.566614638763602,14.0281996676435,
-9.73325324451101));
#46731=CARTESIAN_POINT('Ctrl Pts',(-0.337809554294219,14.028340667515,-9.73833628894296));
#46732=CARTESIAN_POINT('Ctrl Pts',(-0.225004826403271,14.0284101828064,
-9.74084231473926));
#46733=CARTESIAN_POINT('Ctrl Pts',(-0.112392483352252,14.0284409511869,
-9.74208559867157));
#46734=CARTESIAN_POINT('Ctrl Pts',(1.4050982599656E-12,14.0284409294389,
-9.74208557976265));
#46735=CARTESIAN_POINT('Ctrl Pts',(7.81016580919136E-6,14.0284409294374,
-9.74208557976133));
#46736=CARTESIAN_POINT('Ctrl Pts',(1.56203291527005E-5,14.0284409294358,
-9.74208557975401));
#46737=CARTESIAN_POINT('Ctrl Pts',(2.34304914347674E-5,14.028440929434,
-9.7420855797407));
#46738=CARTESIAN_POINT('Ctrl Pts',(0.230478574994379,14.0284408760724,-9.74208518673622));
#46739=CARTESIAN_POINT('Ctrl Pts',(0.461829118783569,14.0283110143972,-9.73685417253584));
#46740=CARTESIAN_POINT('Ctrl Pts',(0.693851093705858,14.0279842381151,-9.72624199356124));
#46741=CARTESIAN_POINT('Ctrl Pts',(0.927871388852005,14.0276546474287,-9.71553841577896));
#46742=CARTESIAN_POINT('Ctrl Pts',(1.16257473051679,14.0271247222249,-9.69936059187738));
#46743=CARTESIAN_POINT('Ctrl Pts',(1.39773131369698,14.0263298736297,-9.67760707303488));
#46744=CARTESIAN_POINT('Ctrl Pts',(1.63446134054756,14.0255297066655,-9.65570800038278));
#46745=CARTESIAN_POINT('Ctrl Pts',(1.87165069452548,14.0244610452605,-9.62815843071653));
#46746=CARTESIAN_POINT('Ctrl Pts',(2.1090649267855,14.0230625066786,-9.59490779642856));
#46747=CARTESIAN_POINT('Ctrl Pts',(2.34947150989978,14.0216463410233,-9.56123807368507));
#46748=CARTESIAN_POINT('Ctrl Pts',(2.59010867571746,14.0198919107936,-9.52172271517559));
#46749=CARTESIAN_POINT('Ctrl Pts',(2.830732998265,14.0177403552189,-9.47636256609525));
#46750=CARTESIAN_POINT('Ctrl Pts',(2.93369717152342,14.0168196954177,-9.45695276496006));
#46751=CARTESIAN_POINT('Ctrl Pts',(3.03665899315264,14.0158263831013,-9.43647342566048));
#46752=CARTESIAN_POINT('Ctrl Pts',(3.1395993906909,14.0147560870973,-9.41492750001361));
#46753=CARTESIAN_POINT('Ctrl Pts',(3.402364148134,14.0120240588886,-9.35992955885661));
#46754=CARTESIAN_POINT('Ctrl Pts',(3.66498146129631,14.0087716270681,-9.29796291359547));
#46755=CARTESIAN_POINT('Ctrl Pts',(3.92711006179015,14.0047954811542,-9.22900273258147));
#46756=CARTESIAN_POINT('Ctrl Pts',(4.19749553574368,14.0006940893358,-9.1578703525502));
#46757=CARTESIAN_POINT('Ctrl Pts',(4.46736102388801,13.9958226091972,-9.07929746709712));
#46758=CARTESIAN_POINT('Ctrl Pts',(4.73633198217297,13.9899668452079,-8.99331689554591));
#46759=CARTESIAN_POINT('Ctrl Pts',(5.03090948501449,13.9835536013982,-8.89915081076881));
#46760=CARTESIAN_POINT('Ctrl Pts',(5.32441402864121,13.9759595147058,-8.79609975055995));
#46761=CARTESIAN_POINT('Ctrl Pts',(5.61635358998981,13.9669161746218,-8.68427180594349));
#46762=CARTESIAN_POINT('Ctrl Pts',(5.83311830245842,13.9602015073668,-8.60123971481899));
#46763=CARTESIAN_POINT('Ctrl Pts',(6.04902023369438,13.9526881277119,-8.51337040698944));
#46764=CARTESIAN_POINT('Ctrl Pts',(6.26385797771861,13.9442712878222,-8.42072561445923));
#46765=CARTESIAN_POINT('Ctrl Pts',(-6.38374306817848,13.9414234665096,-8.37048976079463));
#46766=CARTESIAN_POINT('Ctrl Pts',(-5.82059584927031,13.9721064314624,-8.62634823145341));
#46767=CARTESIAN_POINT('Ctrl Pts',(-4.49614362021116,14.0259437405025,-9.14100802794636));
#46768=CARTESIAN_POINT('Ctrl Pts',(-2.35438543985914,14.0657479998801,-9.65806327216457));
#46769=CARTESIAN_POINT('Ctrl Pts',(0.000944862534166641,14.0770613980891,
-9.84571566180163));
#46770=CARTESIAN_POINT('Ctrl Pts',(2.35625308012023,14.0657286201865,-9.65776341049157));
#46771=CARTESIAN_POINT('Ctrl Pts',(4.49734856102933,14.0259052114703,-9.14058936099707));
#46772=CARTESIAN_POINT('Ctrl Pts',(5.82117757776206,13.9720747788879,-8.62608431902301));
#46773=CARTESIAN_POINT('Ctrl Pts',(6.38374993440966,13.9414230799749,-8.37048666385961));
#46774=CARTESIAN_POINT('Ctrl Pts',(-6.1773119863258,13.4690909032843,-7.96436356123403));
#46775=CARTESIAN_POINT('Ctrl Pts',(-5.63207697424702,13.500338411862,-8.21046045032616));
#46776=CARTESIAN_POINT('Ctrl Pts',(-4.34991588258102,13.5555619320176,-8.70553669287808));
#46777=CARTESIAN_POINT('Ctrl Pts',(-2.2774119989541,13.5972251815216,-9.20285462796731));
#46778=CARTESIAN_POINT('Ctrl Pts',(0.00091390089760303,13.609319564241,
-9.38330152096535));
#46779=CARTESIAN_POINT('Ctrl Pts',(2.27921883855988,13.5972045992365,-9.20256625844348));
#46780=CARTESIAN_POINT('Ctrl Pts',(4.35108223317131,13.5555221053603,-8.70513395156023));
#46781=CARTESIAN_POINT('Ctrl Pts',(5.63264019878497,13.5003061784947,-8.21020660346642));
#46782=CARTESIAN_POINT('Ctrl Pts',(6.17731863567807,13.4690905112704,-7.96436057927722));
#46783=CARTESIAN_POINT('Ctrl Pts',(-6.17551155032075,12.8181924090209,-8.03300126784152));
#46784=CARTESIAN_POINT('Ctrl Pts',(-5.63170106673364,12.8491198316558,-8.27611256190061));
#46785=CARTESIAN_POINT('Ctrl Pts',(-4.35219500761121,12.903814214672,-8.76567194552832));
#46786=CARTESIAN_POINT('Ctrl Pts',(-2.28031100801065,12.9451038841067,-9.25865895634552));
#46787=CARTESIAN_POINT('Ctrl Pts',(0.000915364060213764,12.9570860883808,
-9.43787048445677));
#46788=CARTESIAN_POINT('Ctrl Pts',(2.28211904695125,12.9450834869878,-9.2583727115523));
#46789=CARTESIAN_POINT('Ctrl Pts',(4.35335943163024,12.9037747559201,-8.76527331312379));
#46790=CARTESIAN_POINT('Ctrl Pts',(5.63226282281907,12.8490879200421,-8.27586179676238));
#46791=CARTESIAN_POINT('Ctrl Pts',(6.17551817586046,12.8181920167498,-8.03299832752118));
#46792=CARTESIAN_POINT('Ctrl Pts',(-6.37708413694345,12.4375777136251,-8.52351639529135));
#46793=CARTESIAN_POINT('Ctrl Pts',(-5.81743381263044,12.467530855356,-8.77238436612168));
#46794=CARTESIAN_POINT('Ctrl Pts',(-4.49960759980687,12.5201672053427,-9.2741081038561));
#46795=CARTESIAN_POINT('Ctrl Pts',(-2.36011990204123,12.5591342919587,-9.78095493227011));
#46796=CARTESIAN_POINT('Ctrl Pts',(0.000947852883720792,12.5701990184725,
-9.9656762487021));
#46797=CARTESIAN_POINT('Ctrl Pts',(2.36198956188397,12.5591153237873,-9.78066010083845));
#46798=CARTESIAN_POINT('Ctrl Pts',(4.50080763630646,12.5201295072611,-9.27369908790463));
#46799=CARTESIAN_POINT('Ctrl Pts',(5.81801193592241,12.4674999362466,-8.77212766913687));
#46800=CARTESIAN_POINT('Ctrl Pts',(6.37709094572465,12.4375773264369,-8.5235133956001));
#46801=CARTESIAN_POINT('Ctrl Pts',(-6.24994498501116,12.4626511593801,-8.55169008625593));
#46802=CARTESIAN_POINT('Ctrl Pts',(-5.93338368633412,12.4790326845279,-8.68959465523929));
#46803=CARTESIAN_POINT('Ctrl Pts',(-5.61265410177717,12.4932118124037,-8.81761728472444));
#46804=CARTESIAN_POINT('Ctrl Pts',(-5.28814114363494,12.5055419053853,-8.93533874511386));
#46805=CARTESIAN_POINT('Ctrl Pts',(-5.1109010599461,12.5122762642363,-8.99963498034231));
#46806=CARTESIAN_POINT('Ctrl Pts',(-4.93253192895896,12.5184587937767,-9.06085758779078));
#46807=CARTESIAN_POINT('Ctrl Pts',(-4.75309372274156,12.524145498013,-9.11893249178345));
#46808=CARTESIAN_POINT('Ctrl Pts',(-4.7187542017193,12.5252337762776,-9.13004642581435));
#46809=CARTESIAN_POINT('Ctrl Pts',(-4.68437576021377,12.5263036996257,-9.14104524604668));
#46810=CARTESIAN_POINT('Ctrl Pts',(-4.64995872620909,12.5273556136019,-9.15192850758437));
#46811=CARTESIAN_POINT('Ctrl Pts',(-4.42981456654124,12.5340840469209,-9.22154189917806));
#46812=CARTESIAN_POINT('Ctrl Pts',(-4.20809199462032,12.5400758465265,-9.28642855434412));
#46813=CARTESIAN_POINT('Ctrl Pts',(-3.98492302615565,12.5454105664597,-9.34648339944226));
#46814=CARTESIAN_POINT('Ctrl Pts',(-3.85589357770526,12.548494937801,-9.3812052677786));
#46815=CARTESIAN_POINT('Ctrl Pts',(-3.72638058446272,12.5513591804004,-9.41431224523432));
#46816=CARTESIAN_POINT('Ctrl Pts',(-3.59641035002401,12.5540151891641,-9.44578546448643));
#46817=CARTESIAN_POINT('Ctrl Pts',(-3.52576868899392,12.5554587879357,-9.46289184654025));
#46818=CARTESIAN_POINT('Ctrl Pts',(-3.45554254859571,12.5568302224045,-9.47938649079335));
#46819=CARTESIAN_POINT('Ctrl Pts',(-3.38483967534512,12.5581489342279,-9.49548180717088));
#46820=CARTESIAN_POINT('Ctrl Pts',(-3.325459692702,12.5592564576084,-9.50899949836493));
#46821=CARTESIAN_POINT('Ctrl Pts',(-3.26574318462488,12.560326673833,-9.52223473200989));
#46822=CARTESIAN_POINT('Ctrl Pts',(-3.2051550313525,12.5613679886932,-9.5352858943859));
#46823=CARTESIAN_POINT('Ctrl Pts',(-2.91383358558888,12.566374864364,-9.59803881367665));
#46824=CARTESIAN_POINT('Ctrl Pts',(-2.62163059281673,12.5704045423175,-9.6523014102567));
#46825=CARTESIAN_POINT('Ctrl Pts',(-2.32883742188271,12.5736768622578,-9.69794699246654));
#46826=CARTESIAN_POINT('Ctrl Pts',(-2.02607568806039,12.5770605930176,-9.74514664390341));
#46827=CARTESIAN_POINT('Ctrl Pts',(-1.72268277929252,12.5796341126242,-9.78313345602961));
#46828=CARTESIAN_POINT('Ctrl Pts',(-1.41906580927046,12.58151618669,-9.81191700308478));
#46829=CARTESIAN_POINT('Ctrl Pts',(-1.11206495483235,12.5834192369255,-9.84102134971946));
#46830=CARTESIAN_POINT('Ctrl Pts',(-0.804834430918333,12.5846152787206,
-9.86071627118328));
#46831=CARTESIAN_POINT('Ctrl Pts',(-0.49777905948838,12.585220668062,-9.87096135196521));
#46832=CARTESIAN_POINT('Ctrl Pts',(-0.33177214009757,12.5855479667479,-9.87650026923474));
#46833=CARTESIAN_POINT('Ctrl Pts',(-0.165816194680363,12.5857025170598,
-9.87927618530277));
#46834=CARTESIAN_POINT('Ctrl Pts',(2.58171329915067E-5,12.5857020423694,
-9.87927649675614));
#46835=CARTESIAN_POINT('Ctrl Pts',(0.000327485249286301,12.5857020415059,
-9.87927649732267));
#46836=CARTESIAN_POINT('Ctrl Pts',(0.000629153722568615,12.5857020401084,
-9.87927648873088));
#46837=CARTESIAN_POINT('Ctrl Pts',(0.00093082255248277,12.5857020381768,
-9.87927647098056));
#46838=CARTESIAN_POINT('Ctrl Pts',(0.29883321452666,12.5857001307359,-9.879258942275));
#46839=CARTESIAN_POINT('Ctrl Pts',(0.597084493922628,12.5851778676453,-9.87031429001266));
#46840=CARTESIAN_POINT('Ctrl Pts',(0.895336025094607,12.5840597930142,-9.85247090002633));
#46841=CARTESIAN_POINT('Ctrl Pts',(1.13208149249359,12.5831722901064,-9.83830721179413));
#46842=CARTESIAN_POINT('Ctrl Pts',(1.36882702253841,12.5819093075633,-9.81853557990205));
#46843=CARTESIAN_POINT('Ctrl Pts',(1.60539033451399,12.5802306826658,-9.79314830718627));
#46844=CARTESIAN_POINT('Ctrl Pts',(1.84741516945489,12.5785133034562,-9.76717492003117));
#46845=CARTESIAN_POINT('Ctrl Pts',(2.08925199887728,12.5763522816075,-9.73533445771998));
#46846=CARTESIAN_POINT('Ctrl Pts',(2.33070782969548,12.5736597148678,-9.69765040163421));
#46847=CARTESIAN_POINT('Ctrl Pts',(2.35606681193083,12.5733769271136,-9.69369262059576));
#46848=CARTESIAN_POINT('Ctrl Pts',(2.38142158883918,12.5730882736115,-9.68967036268841));
#46849=CARTESIAN_POINT('Ctrl Pts',(2.40677199762222,12.5727935830512,-9.68558375444369));
#46850=CARTESIAN_POINT('Ctrl Pts',(2.54013430131214,12.5712432880506,-9.66408510744125));
#46851=CARTESIAN_POINT('Ctrl Pts',(2.67337439519718,12.5695272160787,-9.64080421635102));
#46852=CARTESIAN_POINT('Ctrl Pts',(2.80646029870055,12.5676287808786,-9.61574910601489));
#46853=CARTESIAN_POINT('Ctrl Pts',(2.87846051899447,12.5666017167868,-9.60219415078521));
#46854=CARTESIAN_POINT('Ctrl Pts',(2.9509727355371,12.5655128307827,-9.58801061068387));
#46855=CARTESIAN_POINT('Ctrl Pts',(3.02308661174239,12.5643722825228,-9.57337240027714));
#46856=CARTESIAN_POINT('Ctrl Pts',(3.0842687217262,12.5634046303489,-9.56095320100236));
#46857=CARTESIAN_POINT('Ctrl Pts',(3.14516423945337,12.5623998611268,-9.54820765663932));
#46858=CARTESIAN_POINT('Ctrl Pts',(3.20522363885174,12.5613672627394,-9.53527055144678));
#46859=CARTESIAN_POINT('Ctrl Pts',(3.52196512413216,12.5559215415006,-9.46704279767362));
#46860=CARTESIAN_POINT('Ctrl Pts',(3.8362022023586,12.5493532214616,-9.3890832650296));
#46861=CARTESIAN_POINT('Ctrl Pts',(4.14754504429288,12.541448947496,-9.30172845627976));
#46862=CARTESIAN_POINT('Ctrl Pts',(4.31648149642719,12.5371600420817,-9.25432922469509));
#46863=CARTESIAN_POINT('Ctrl Pts',(4.48456554909833,12.5324777247987,-9.20416294759299));
#46864=CARTESIAN_POINT('Ctrl Pts',(4.65173253716364,12.5273671479188,-9.15127749971604));
#46865=CARTESIAN_POINT('Ctrl Pts',(4.9647529062626,12.5177975870876,-9.05224944037253));
#46866=CARTESIAN_POINT('Ctrl Pts',(5.27455949898563,12.5067271099657,-8.94368979231894));
#46867=CARTESIAN_POINT('Ctrl Pts',(5.58085220748431,12.4938926574309,-8.82593410453551));
#46868=CARTESIAN_POINT('Ctrl Pts',(5.80582191344839,12.4844658479352,-8.73944343165569));
#46869=CARTESIAN_POINT('Ctrl Pts',(6.02889546083625,12.4740872407875,-8.64799069239423));
#46870=CARTESIAN_POINT('Ctrl Pts',(6.24994363575164,12.4626483740505,-8.5516948379668));
#46871=CARTESIAN_POINT('Ctrl Pts',(7.10529336472858,7.16048923499633,-14.3567206907318));
#46872=CARTESIAN_POINT('Ctrl Pts',(7.1064275368113,7.24034649935247,-14.3164705260865));
#46873=CARTESIAN_POINT('Ctrl Pts',(7.09037559920597,7.42259570938419,-14.2296084470487));
#46874=CARTESIAN_POINT('Ctrl Pts',(7.00203596961012,7.70267882729892,-14.1129068657706));
#46875=CARTESIAN_POINT('Ctrl Pts',(6.84111528275874,7.97637671077655,-14.0188435983679));
#46876=CARTESIAN_POINT('Ctrl Pts',(6.62715076555215,8.20731154449834,-13.9610638995495));
#46877=CARTESIAN_POINT('Ctrl Pts',(6.42119926597592,8.35211939072247,-13.9452161478941));
#46878=CARTESIAN_POINT('Ctrl Pts',(6.29197222530054,8.41580527600954,-13.9494152732194));
#46879=CARTESIAN_POINT('Ctrl Pts',(6.25107867181893,8.43351433517937,-13.9520220265804));
#46880=CARTESIAN_POINT('Ctrl Pts',(6.81695434203023,6.90423125129657,-13.8395073332205));
#46881=CARTESIAN_POINT('Ctrl Pts',(6.81797118283742,6.97460530088759,-13.8040212512093));
#46882=CARTESIAN_POINT('Ctrl Pts',(6.80354599269152,7.13572701890584,-13.7274488397656));
#46883=CARTESIAN_POINT('Ctrl Pts',(6.72389639326869,7.38404253596884,-13.6251523381992));
#46884=CARTESIAN_POINT('Ctrl Pts',(6.57905010989704,7.62656630202561,-13.5437450468964));
#46885=CARTESIAN_POINT('Ctrl Pts',(6.38723329244376,7.83061781411381,-13.4949402802546));
#46886=CARTESIAN_POINT('Ctrl Pts',(6.20363484828439,7.95800648462909,-13.4827503106996));
#46887=CARTESIAN_POINT('Ctrl Pts',(6.08903468842784,8.01384149509141,-13.4872621068598));
#46888=CARTESIAN_POINT('Ctrl Pts',(6.05283226078958,8.02935410316426,-13.489777394369));
#46889=CARTESIAN_POINT('Ctrl Pts',(7.05875964334239,6.63234584950194,-13.3065825231142));
#46890=CARTESIAN_POINT('Ctrl Pts',(7.06010346820671,6.72332482551982,-13.260728454359));
#46891=CARTESIAN_POINT('Ctrl Pts',(7.04118734267824,6.92988246936252,-13.1622551946321));
#46892=CARTESIAN_POINT('Ctrl Pts',(6.93788435052611,7.24649106248276,-13.0301399355402));
#46893=CARTESIAN_POINT('Ctrl Pts',(6.74896177210885,7.55747236941287,-12.9230480356511));
#46894=CARTESIAN_POINT('Ctrl Pts',(6.49540659457737,7.8226841502203,-12.8567005545142));
#46895=CARTESIAN_POINT('Ctrl Pts',(6.24819682300408,7.99157414700557,-12.8385724942454));
#46896=CARTESIAN_POINT('Ctrl Pts',(6.09125158425211,8.06689842540132,-12.8439943442258));
#46897=CARTESIAN_POINT('Ctrl Pts',(6.04139644311579,8.08794686373372,-12.8472574438417));
#46898=CARTESIAN_POINT('Ctrl Pts',(7.66735121800432,6.52877730330966,-13.1185037491408));
#46899=CARTESIAN_POINT('Ctrl Pts',(7.66924531506772,6.65652225417889,-13.0541574622128));
#46900=CARTESIAN_POINT('Ctrl Pts',(7.64275624394143,6.9443687062556,-12.9163957628901));
#46901=CARTESIAN_POINT('Ctrl Pts',(7.49944502218963,7.38317117659575,-12.7303924191653));
#46902=CARTESIAN_POINT('Ctrl Pts',(7.23608901619539,7.81597033812076,-12.5766354500427));
#46903=CARTESIAN_POINT('Ctrl Pts',(6.87864190335745,8.18904651334705,-12.4780845072667));
#46904=CARTESIAN_POINT('Ctrl Pts',(6.52485516459777,8.43030637575862,-12.4484356813334));
#46905=CARTESIAN_POINT('Ctrl Pts',(6.29721660236423,8.53928654730601,-12.4547495191759));
#46906=CARTESIAN_POINT('Ctrl Pts',(6.22459365164253,8.56986120938434,-12.4590941392797));
#46907=CARTESIAN_POINT('',(6.26385989003177,8.42071839535226,-13.9442649557177));
#46908=CARTESIAN_POINT('',(6.24994593946664,8.55169414006259,-12.4626532547806));
#46909=CARTESIAN_POINT('Ctrl Pts',(6.26385687510184,8.42071068624793,-13.9442728359392));
#46910=CARTESIAN_POINT('Ctrl Pts',(6.25434589570407,8.4015288148462,-13.9218689631775));
#46911=CARTESIAN_POINT('Ctrl Pts',(6.24501143579651,8.38292246516115,-13.8980040452737));
#46912=CARTESIAN_POINT('Ctrl Pts',(6.23595649835892,8.36511937125287,-13.8726943205492));
#46913=CARTESIAN_POINT('Ctrl Pts',(6.22712817822746,8.34776183417036,-13.8480180205917));
#46914=CARTESIAN_POINT('Ctrl Pts',(6.21856585461717,8.33116854811689,-13.8219680644561));
#46915=CARTESIAN_POINT('Ctrl Pts',(6.21037090452425,8.31555920420894,-13.7946076666852));
#46916=CARTESIAN_POINT('Ctrl Pts',(6.20230230129337,8.30019051968255,-13.7676691019167));
#46917=CARTESIAN_POINT('Ctrl Pts',(6.19459015268015,8.28577642744152,-13.7394600730491));
#46918=CARTESIAN_POINT('Ctrl Pts',(6.18733252944957,8.27252438528487,-13.7100911322866));
#46919=CARTESIAN_POINT('Ctrl Pts',(6.18020247023623,8.25950526838217,-13.6812383963404));
#46920=CARTESIAN_POINT('Ctrl Pts',(6.17351143247687,8.24760846707906,-13.651266308102));
#46921=CARTESIAN_POINT('Ctrl Pts',(6.16734883482834,8.23701734476728,-13.6203283182696));
#46922=CARTESIAN_POINT('Ctrl Pts',(6.16655150095895,8.23564703617086,-13.6163254758725));
#46923=CARTESIAN_POINT('Ctrl Pts',(6.16576300405729,8.2342985566984,-13.6123065298336));
#46924=CARTESIAN_POINT('Ctrl Pts',(6.16498352875401,8.23297227653974,-13.6082718703713));
#46925=CARTESIAN_POINT('Ctrl Pts',(6.15905115567951,8.222878321453,-13.5775651820919));
#46926=CARTESIAN_POINT('Ctrl Pts',(6.15364235588507,8.21407261921391,-13.5459450166987));
#46927=CARTESIAN_POINT('Ctrl Pts',(6.14883171670341,8.20670298643533,-13.513607214262));
#46928=CARTESIAN_POINT('Ctrl Pts',(6.14408270715969,8.19942776684858,-13.4816836950382));
#46929=CARTESIAN_POINT('Ctrl Pts',(6.1399169029108,8.19355261195391,-13.4490613933326));
#46930=CARTESIAN_POINT('Ctrl Pts',(6.13639279479276,8.18918575798983,-13.4159640037694));
#46931=CARTESIAN_POINT('Ctrl Pts',(6.13288938116379,8.18484454733992,-13.3830609707763));
#46932=CARTESIAN_POINT('Ctrl Pts',(6.13002036913961,8.18199439530407,-13.3496891324172));
#46933=CARTESIAN_POINT('Ctrl Pts',(6.12782632623896,8.18070050838779,-13.3160936799609));
#46934=CARTESIAN_POINT('Ctrl Pts',(6.12563972821355,8.17941101191741,-13.282612224342));
#46935=CARTESIAN_POINT('Ctrl Pts',(6.12412366519578,8.17966746091332,-13.2489094999238));
#46936=CARTESIAN_POINT('Ctrl Pts',(6.12329875486801,8.18148856024423,-13.2152419051193));
#46937=CARTESIAN_POINT('Ctrl Pts',(6.122474587247,8.18330801995111,-13.1816046228829));
#46938=CARTESIAN_POINT('Ctrl Pts',(6.12234037294115,8.18668931913289,-13.1480032828271));
#46939=CARTESIAN_POINT('Ctrl Pts',(6.12289574278324,8.19160351827314,-13.1146944380087));
#46940=CARTESIAN_POINT('Ctrl Pts',(6.12345381872746,8.19654166240232,-13.0812232920913));
#46941=CARTESIAN_POINT('Ctrl Pts',(6.12470817202044,8.20302748811596,-13.0480483652075));
#46942=CARTESIAN_POINT('Ctrl Pts',(6.12663723832506,8.21098489540582,-13.0154176313383));
#46943=CARTESIAN_POINT('Ctrl Pts',(6.12857376793279,8.218973088855,-12.9826606534633));
#46944=CARTESIAN_POINT('Ctrl Pts',(6.13119008983231,8.22844384478804,-12.9504528531314));
#46945=CARTESIAN_POINT('Ctrl Pts',(6.13444456932835,8.239277915888,-12.9190202913252));
#46946=CARTESIAN_POINT('Ctrl Pts',(6.1377364432029,8.25023647182683,-12.8872265654326));
#46947=CARTESIAN_POINT('Ctrl Pts',(6.14168100076899,8.26258927480383,-12.8562266434431));
#46948=CARTESIAN_POINT('Ctrl Pts',(6.14621773612586,8.27617735011607,-12.8262182957706));
#46949=CARTESIAN_POINT('Ctrl Pts',(6.14952201341343,8.28607406330389,-12.8043620723299));
#46950=CARTESIAN_POINT('Ctrl Pts',(6.15314003900114,8.29662526281776,-12.7830310876382));
#46951=CARTESIAN_POINT('Ctrl Pts',(6.15704389852412,8.30776080160357,-12.7622874067421));
#46952=CARTESIAN_POINT('Ctrl Pts',(6.16249948673207,8.32332255881625,-12.7332984074658));
#46953=CARTESIAN_POINT('Ctrl Pts',(6.1685132782615,8.34002577189179,-12.7054585112995));
#46954=CARTESIAN_POINT('Ctrl Pts',(6.17499976480806,8.35766462314905,-12.6788945748029));
#46955=CARTESIAN_POINT('Ctrl Pts',(6.18163464544893,8.37570700586176,-12.6517229239035));
#46956=CARTESIAN_POINT('Ctrl Pts',(6.18876374432969,8.3947275157599,-12.6258863743513));
#46957=CARTESIAN_POINT('Ctrl Pts',(6.19628989507741,8.41449938873199,-12.6014667977307));
#46958=CARTESIAN_POINT('Ctrl Pts',(6.20392753003438,8.43456414071986,-12.5766854960689));
#46959=CARTESIAN_POINT('Ctrl Pts',(6.21197371279697,8.45540190412297,-12.5533632206732));
#46960=CARTESIAN_POINT('Ctrl Pts',(6.22032660104379,8.47678133667707,-12.5315318672047));
#46961=CARTESIAN_POINT('Ctrl Pts',(6.22887982626834,8.49867353688436,-12.5091769071411));
#46962=CARTESIAN_POINT('Ctrl Pts',(6.23775431758807,8.52113300253076,-12.4883848497663));
#46963=CARTESIAN_POINT('Ctrl Pts',(6.24684570637579,8.54392866164999,-12.46913883099));
#46964=CARTESIAN_POINT('Ctrl Pts',(6.24787632883521,8.54651283430105,-12.4669570544024));
#46965=CARTESIAN_POINT('Ctrl Pts',(6.24890974675756,8.54910135151727,-12.464795097349));
#46966=CARTESIAN_POINT('Ctrl Pts',(6.24994581473478,8.55169389599726,-12.4626528990853));
#46967=CARTESIAN_POINT('',(7.0000000055496,8.04447578018918,-12.5220651288373));
#46968=CARTESIAN_POINT('Ctrl Pts',(7.00000001330434,8.0444754912143,-12.5220639333861));
#46969=CARTESIAN_POINT('Ctrl Pts',(6.96230391367629,8.08169105625708,-12.5128233328542));
#46970=CARTESIAN_POINT('Ctrl Pts',(6.92358275821775,8.11749582950849,-12.5046001520993));
#46971=CARTESIAN_POINT('Ctrl Pts',(6.88384360033652,8.15194944871618,-12.4973741501251));
#46972=CARTESIAN_POINT('Ctrl Pts',(6.87536872889752,8.1592971130594,-12.4958331150098));
#46973=CARTESIAN_POINT('Ctrl Pts',(6.86684740727857,8.16658324491893,-12.494337512666));
#46974=CARTESIAN_POINT('Ctrl Pts',(6.85827946666746,8.17380828443588,-12.4928872796855));
#46975=CARTESIAN_POINT('Ctrl Pts',(6.82975275306883,8.19786384718938,-12.4880587703898));
#46976=CARTESIAN_POINT('Ctrl Pts',(6.80070995695535,8.22124272875811,-12.4837327177821));
#46977=CARTESIAN_POINT('Ctrl Pts',(6.77114945909981,8.24395849804649,-12.4799068065204));
#46978=CARTESIAN_POINT('Ctrl Pts',(6.70392153480423,8.29561980718607,-12.4712057327456));
#46979=CARTESIAN_POINT('Ctrl Pts',(6.63401832348786,8.343863738285,-12.4650822521963));
#46980=CARTESIAN_POINT('Ctrl Pts',(6.56187334522743,8.38842090408476,-12.4616052237448));
#46981=CARTESIAN_POINT('Ctrl Pts',(6.54809121393698,8.39693282998439,-12.4609409936934));
#46982=CARTESIAN_POINT('Ctrl Pts',(6.53422713052313,8.40531018090756,-12.4603733932308));
#46983=CARTESIAN_POINT('Ctrl Pts',(6.52028392429325,8.41355102861473,-12.4599029761146));
#46984=CARTESIAN_POINT('Ctrl Pts',(6.4919859927506,8.43027594399118,-12.4589482580154));
#46985=CARTESIAN_POINT('Ctrl Pts',(6.46336436275962,8.44643567541406,-12.4583951007039));
#46986=CARTESIAN_POINT('Ctrl Pts',(6.43440475968353,8.4620318338438,-12.4582494770983));
#46987=CARTESIAN_POINT('Ctrl Pts',(6.38955372914157,8.48618630088645,-12.4580239433172));
#46988=CARTESIAN_POINT('Ctrl Pts',(6.34389273458103,8.50899103300897,-12.4587745664364));
#46989=CARTESIAN_POINT('Ctrl Pts',(6.29738181090352,8.53043175235834,-12.4605287526016));
#46990=CARTESIAN_POINT('Ctrl Pts',(6.28166761543794,8.53767572061652,-12.4611214224972));
#46991=CARTESIAN_POINT('Ctrl Pts',(6.26585625737833,8.54476364661387,-12.4618288799934));
#46992=CARTESIAN_POINT('Ctrl Pts',(6.24994581473509,8.55169389599713,-12.4626528990853));
#46993=CARTESIAN_POINT('',(7.,6.97709641029578,-13.9487350316508));
#46994=CARTESIAN_POINT('Ctrl Pts',(7.,6.97709641029578,-13.9487350316508));
#46995=CARTESIAN_POINT('Ctrl Pts',(7.,7.03293718041427,-13.8193396715212));
#46996=CARTESIAN_POINT('Ctrl Pts',(7.,7.08905635229391,-13.6999263902358));
#46997=CARTESIAN_POINT('Ctrl Pts',(7.,7.14545392593474,-13.5904951877945));
#46998=CARTESIAN_POINT('Ctrl Pts',(7.,7.16425311714834,-13.554018120314));
#46999=CARTESIAN_POINT('Ctrl Pts',(7.,7.18201591735578,-13.5205888384398));
#47000=CARTESIAN_POINT('Ctrl Pts',(7.,7.20194430016261,-13.4843913449679));
#47001=CARTESIAN_POINT('Ctrl Pts',(7.,7.28165783138991,-13.3396013710801));
#47002=CARTESIAN_POINT('Ctrl Pts',(7.,7.36741849085433,-13.2055562149066));
#47003=CARTESIAN_POINT('Ctrl Pts',(7.,7.45610471591587,-13.0864482193812));
#47004=CARTESIAN_POINT('Ctrl Pts',(7.,7.63347716603895,-12.8482322283304));
#47005=CARTESIAN_POINT('Ctrl Pts',(7.,7.82960075808121,-12.6601046255877));
#47006=CARTESIAN_POINT('Ctrl Pts',(7.,8.04447549204264,-12.5220654111529));
#47007=CARTESIAN_POINT('Ctrl Pts',(6.99999409973866,6.97709640977505,-13.9487350319038));
#47008=CARTESIAN_POINT('Ctrl Pts',(6.99998773340224,7.02238008649688,-13.9417617463364));
#47009=CARTESIAN_POINT('Ctrl Pts',(6.99825780681655,7.0667383458091,-13.9353109212988));
#47010=CARTESIAN_POINT('Ctrl Pts',(6.99506629168637,7.1100004802052,-13.929375924186));
#47011=CARTESIAN_POINT('Ctrl Pts',(6.99192032954138,7.15264512751851,-13.9235256381978));
#47012=CARTESIAN_POINT('Ctrl Pts',(6.98735349753255,7.19422506924278,-13.9181766158872));
#47013=CARTESIAN_POINT('Ctrl Pts',(6.98158514077008,7.23461460637864,-13.9133177410806));
#47014=CARTESIAN_POINT('Ctrl Pts',(6.97530695511168,7.27857392152467,-13.9080294207871));
#47015=CARTESIAN_POINT('Ctrl Pts',(6.9676065761953,7.32112357876287,-13.9033213294894));
#47016=CARTESIAN_POINT('Ctrl Pts',(6.95878220379846,7.36217508309488,-13.8991509038545));
#47017=CARTESIAN_POINT('Ctrl Pts',(6.95175715564054,7.39485602423362,-13.8958308444094));
#47018=CARTESIAN_POINT('Ctrl Pts',(6.94401872090156,7.42658826306636,-13.8928515284589));
#47019=CARTESIAN_POINT('Ctrl Pts',(6.93569970011813,7.45734250331633,-13.8901905229079));
#47020=CARTESIAN_POINT('Ctrl Pts',(6.92545249237511,7.49522497735077,-13.8869127481077));
#47021=CARTESIAN_POINT('Ctrl Pts',(6.91432486971307,7.53162294634188,-13.8841180209678));
#47022=CARTESIAN_POINT('Ctrl Pts',(6.90253856527727,7.56650707684142,-13.8817619962387));
#47023=CARTESIAN_POINT('Ctrl Pts',(6.88931061744749,7.60565806440064,-13.8791177940316));
#47024=CARTESIAN_POINT('Ctrl Pts',(6.87525432449622,7.64290263392926,-13.8770257005009));
#47025=CARTESIAN_POINT('Ctrl Pts',(6.86067610400931,7.67825570504179,-13.8754032193005));
#47026=CARTESIAN_POINT('Ctrl Pts',(6.85201223617144,7.69926611135696,-13.8744389752282));
#47027=CARTESIAN_POINT('Ctrl Pts',(6.84316308205284,7.71960899951211,-13.8736406359784));
#47028=CARTESIAN_POINT('Ctrl Pts',(6.83418557292495,7.73929185965251,-13.8729911263498));
#47029=CARTESIAN_POINT('Ctrl Pts',(6.82792838530364,7.75301051446733,-13.8725384279956));
#47030=CARTESIAN_POINT('Ctrl Pts',(6.82160873308596,7.76640860216193,-13.8721580324725));
#47031=CARTESIAN_POINT('Ctrl Pts',(6.81524449342781,7.77948949420881,-13.8718441865394));
#47032=CARTESIAN_POINT('Ctrl Pts',(6.81206237359873,7.78602994023225,-13.8716872635729));
#47033=CARTESIAN_POINT('Ctrl Pts',(6.80886909868809,7.7924910834006,-13.871546982403));
#47034=CARTESIAN_POINT('Ctrl Pts',(6.8056667930717,7.79887342071668,-13.8714226207036));
#47035=CARTESIAN_POINT('Ctrl Pts',(6.80406564026351,7.80206458937472,-13.8713604398539));
#47036=CARTESIAN_POINT('Ctrl Pts',(6.80246222927231,7.80523605633618,-13.871302239133));
#47037=CARTESIAN_POINT('Ctrl Pts',(6.80085682107126,7.80838788492505,-13.8712479289958));
#47038=CARTESIAN_POINT('Ctrl Pts',(6.7994724279675,7.8111058041183,-13.8712010956861));
#47039=CARTESIAN_POINT('Ctrl Pts',(6.79847729449419,7.81305026698218,-13.8711691335029));
#47040=CARTESIAN_POINT('Ctrl Pts',(6.79686095399513,7.81618460023036,-13.8711208812908));
#47041=CARTESIAN_POINT('Ctrl Pts',(6.79660290904266,7.81668498914875,-13.8711131779388));
#47042=CARTESIAN_POINT('Ctrl Pts',(6.79632895166726,7.81721565513594,-13.8711051012948));
#47043=CARTESIAN_POINT('Ctrl Pts',(6.7960348629784,7.8177845195718,-13.8710965813229));
#47044=CARTESIAN_POINT('Ctrl Pts',(6.78633377486737,7.83654962079648,-13.8708155334567));
#47045=CARTESIAN_POINT('Ctrl Pts',(6.77635283842971,7.85503260700263,-13.8706755538496));
#47046=CARTESIAN_POINT('Ctrl Pts',(6.76610585975263,7.87322195488204,-13.8706790001011));
#47047=CARTESIAN_POINT('Ctrl Pts',(6.73511960207716,7.92822546743936,-13.870689421362));
#47048=CARTESIAN_POINT('Ctrl Pts',(6.70170471002237,7.98054310553255,-13.8720098209944));
#47049=CARTESIAN_POINT('Ctrl Pts',(6.66632523798378,8.02995177089685,-13.8746434658222));
#47050=CARTESIAN_POINT('Ctrl Pts',(6.63916138333988,8.0678870403277,-13.8766655408042));
#47051=CARTESIAN_POINT('Ctrl Pts',(6.61083810974908,8.1041076340751,-13.8794623048069));
#47052=CARTESIAN_POINT('Ctrl Pts',(6.58154671953346,8.13851818864679,-13.8830415512864));
#47053=CARTESIAN_POINT('Ctrl Pts',(6.54179775503399,8.18521395494564,-13.8878986557189));
#47054=CARTESIAN_POINT('Ctrl Pts',(6.5002682591157,8.22857660783537,-13.8941957405529));
#47055=CARTESIAN_POINT('Ctrl Pts',(6.45749341303235,8.26847853134568,-13.9018834005547));
#47056=CARTESIAN_POINT('Ctrl Pts',(6.42567623290322,8.29815874773624,-13.9076017066492));
#47057=CARTESIAN_POINT('Ctrl Pts',(6.39316882688615,8.32592430382819,-13.9140899065749));
#47058=CARTESIAN_POINT('Ctrl Pts',(6.36017433818513,8.35172762350273,-13.9213326680527));
#47059=CARTESIAN_POINT('Ctrl Pts',(6.3284535697521,8.37653483102203,-13.9282958297412));
#47060=CARTESIAN_POINT('Ctrl Pts',(6.29628264519726,8.39952869941061,-13.9359562792266));
#47061=CARTESIAN_POINT('Ctrl Pts',(6.2638568752866,8.42071068616162,-13.9442728359254));
#47062=CARTESIAN_POINT('Ctrl Pts',(6.99927529182611,10.8726415770594,-24.2327789237978));
#47063=CARTESIAN_POINT('Ctrl Pts',(6.99927529182611,10.8786673784413,-24.195315187381));
#47064=CARTESIAN_POINT('Ctrl Pts',(6.99927529182611,10.9735995203797,-23.5849660827267));
#47065=CARTESIAN_POINT('Ctrl Pts',(6.99927529182611,11.0582112387948,-22.3847865482758));
#47066=CARTESIAN_POINT('Ctrl Pts',(6.99927529182611,10.903047790836,-20.6453395628878));
#47067=CARTESIAN_POINT('Ctrl Pts',(6.99927529182611,10.4741299264985,-18.9496408568389));
#47068=CARTESIAN_POINT('Ctrl Pts',(6.99927529182611,9.78081713300028,-17.3432623946008));
#47069=CARTESIAN_POINT('Ctrl Pts',(6.99927529182611,8.84300079934772,-15.8679928669231));
#47070=CARTESIAN_POINT('Ctrl Pts',(6.99927529182611,7.83768636590236,-14.7356908281778));
#47071=CARTESIAN_POINT('Ctrl Pts',(6.99927529182611,7.13749347049657,-14.123730174869));
#47072=CARTESIAN_POINT('Ctrl Pts',(6.99927529182611,6.86420636501945,-13.9070393690543));
#47073=CARTESIAN_POINT('Ctrl Pts',(7.017832597561,11.3536240592414,-24.3101961947595));
#47074=CARTESIAN_POINT('Ctrl Pts',(7.017832597561,11.3599171239206,-24.2710685142874));
#47075=CARTESIAN_POINT('Ctrl Pts',(7.017832597561,11.4590599350526,-23.6336238827185));
#47076=CARTESIAN_POINT('Ctrl Pts',(7.017832597561,11.5474272379709,-22.3805204832481));
#47077=CARTESIAN_POINT('Ctrl Pts',(7.017832597561,11.3853285909672,-20.5631123377262));
#47078=CARTESIAN_POINT('Ctrl Pts',(7.017832597561,10.9373786509483,-18.7923604165634));
#47079=CARTESIAN_POINT('Ctrl Pts',(7.017832597561,10.2132342895059,-17.1143873744336));
#47080=CARTESIAN_POINT('Ctrl Pts',(7.017832597561,9.23354352116467,-15.5733329492476));
#47081=CARTESIAN_POINT('Ctrl Pts',(7.017832597561,8.18359794548622,-14.390762581988));
#47082=CARTESIAN_POINT('Ctrl Pts',(7.017832597561,7.45236474088215,-13.751653467176));
#47083=CARTESIAN_POINT('Ctrl Pts',(7.017832597561,7.1668757223976,-13.5252911594398));
#47084=CARTESIAN_POINT('Ctrl Pts',(6.72802461549766,11.741859342275,-24.3726851984411));
#47085=CARTESIAN_POINT('Ctrl Pts',(6.72802461549766,11.7483681342363,-24.3322144299968));
#47086=CARTESIAN_POINT('Ctrl Pts',(6.72802461549766,11.8509096769365,-23.6728990651836));
#47087=CARTESIAN_POINT('Ctrl Pts',(6.72802461549766,11.9423083800943,-22.377077037741));
#47088=CARTESIAN_POINT('Ctrl Pts',(6.72802461549766,11.7746118390656,-20.4967408767737));
#47089=CARTESIAN_POINT('Ctrl Pts',(6.72802461549766,11.3112997526846,-18.6654081500895));
#47090=CARTESIAN_POINT('Ctrl Pts',(6.72802461549766,10.5622690326939,-16.9296460137264));
#47091=CARTESIAN_POINT('Ctrl Pts',(6.72802461549766,9.54877842006116,-15.3354919035144));
#47092=CARTESIAN_POINT('Ctrl Pts',(6.72802461549766,8.46280786472511,-14.1123463812967));
#47093=CARTESIAN_POINT('Ctrl Pts',(6.72802461549766,7.70651981161201,-13.4513238059636));
#47094=CARTESIAN_POINT('Ctrl Pts',(6.72802461549766,7.41118175844214,-13.2171549388937));
#47095=CARTESIAN_POINT('Ctrl Pts',(6.2547269417983,11.8649496891146,-24.3924973934525));
#47096=CARTESIAN_POINT('Ctrl Pts',(6.2547269417983,11.8715268776038,-24.3516007977501));
#47097=CARTESIAN_POINT('Ctrl Pts',(6.2547269417983,11.9751459912159,-23.6853512972297));
#47098=CARTESIAN_POINT('Ctrl Pts',(6.2547269417983,12.0675058025525,-22.375985290233));
#47099=CARTESIAN_POINT('Ctrl Pts',(6.2547269417983,11.8980344441738,-20.4756977451863));
#47100=CARTESIAN_POINT('Ctrl Pts',(6.2547269417983,11.429851775427,-18.6251578194452));
#47101=CARTESIAN_POINT('Ctrl Pts',(6.2547269417983,10.6729308129992,-16.8710735986019));
#47102=CARTESIAN_POINT('Ctrl Pts',(6.2547269417983,9.64872392923276,-15.2600841853353));
#47103=CARTESIAN_POINT('Ctrl Pts',(6.2547269417983,8.55133162158488,-14.024074273618));
#47104=CARTESIAN_POINT('Ctrl Pts',(6.2547269417983,7.78709990614218,-13.3561040158518));
#47105=CARTESIAN_POINT('Ctrl Pts',(6.2547269417983,7.48863920763838,-13.1194600721039));
#47106=CARTESIAN_POINT('',(7.00000000000001,10.9277801898197,-24.1259420764688));
#47107=CARTESIAN_POINT('Ctrl Pts',(7.00000000000005,10.9277802009506,-24.1259420781411));
#47108=CARTESIAN_POINT('Ctrl Pts',(7.00000000000005,10.9521693515102,-23.9636096893172));
#47109=CARTESIAN_POINT('Ctrl Pts',(7.00000000006095,10.9728901444114,-23.801252032564));
#47110=CARTESIAN_POINT('Ctrl Pts',(6.99999999867112,10.9899908760259,-23.6387724641683));
#47111=CARTESIAN_POINT('Ctrl Pts',(6.99999999727843,11.0071267182727,-23.4759592983278));
#47112=CARTESIAN_POINT('Ctrl Pts',(6.99999999421914,11.0206276373359,-23.3130232621382));
#47113=CARTESIAN_POINT('Ctrl Pts',(6.99999999313357,11.0304902733626,-23.149860765446));
#47114=CARTESIAN_POINT('Ctrl Pts',(6.99999999205182,11.0403181946778,-22.9872725715058));
#47115=CARTESIAN_POINT('Ctrl Pts',(6.99999999470457,11.0465333999261,-22.8244590565224));
#47116=CARTESIAN_POINT('Ctrl Pts',(6.99999999802627,11.0490809628184,-22.6613182277958));
#47117=CARTESIAN_POINT('Ctrl Pts',(6.99999999906757,11.04987958869,-22.6101758254147));
#47118=CARTESIAN_POINT('Ctrl Pts',(7.00000000000005,11.0503173996174,-22.5590012875906));
#47119=CARTESIAN_POINT('Ctrl Pts',(7.00000000000005,11.0503916515239,-22.507791591419));
#47120=CARTESIAN_POINT('Ctrl Pts',(7.00000000000005,11.0504508814845,-22.4669421583217));
#47121=CARTESIAN_POINT('Ctrl Pts',(6.99999999938506,11.0502838028415,-22.426069923528));
#47122=CARTESIAN_POINT('Ctrl Pts',(6.99999999847366,11.0498891594648,-22.3851800824517));
#47123=CARTESIAN_POINT('Ctrl Pts',(6.99999999415778,11.0480203461542,-22.1915483537147));
#47124=CARTESIAN_POINT('Ctrl Pts',(6.99999998570413,11.0410443720245,-21.9975213270894));
#47125=CARTESIAN_POINT('Ctrl Pts',(6.99999998494295,11.0289325037734,-21.8035929264893));
#47126=CARTESIAN_POINT('Ctrl Pts',(6.99999998418016,11.016795034324,-21.6092546139492));
#47127=CARTESIAN_POINT('Ctrl Pts',(6.99999998976666,10.9994999282979,-21.4150157630175));
#47128=CARTESIAN_POINT('Ctrl Pts',(6.99999999468265,10.9770705166507,-21.2213760732062));
#47129=CARTESIAN_POINT('Ctrl Pts',(6.99999999757253,10.9638852767666,-21.1075440297526));
#47130=CARTESIAN_POINT('Ctrl Pts',(7.00000000000005,10.9489267433494,-20.9939190591194));
#47131=CARTESIAN_POINT('Ctrl Pts',(7.00000000000005,10.932208049831,-20.8806022008953));
#47132=CARTESIAN_POINT('Ctrl Pts',(7.00000000000005,10.9207197174214,-20.8027359649097));
#47133=CARTESIAN_POINT('Ctrl Pts',(6.99999999889749,10.9083941647938,-20.7250167855243));
#47134=CARTESIAN_POINT('Ctrl Pts',(6.99999999756676,10.8952339987249,-20.647455114461));
#47135=CARTESIAN_POINT('Ctrl Pts',(6.99999999341047,10.8541305337291,-20.4052048711987));
#47136=CARTESIAN_POINT('Ctrl Pts',(6.99999998911108,10.8048891706622,-20.1644906605692));
#47137=CARTESIAN_POINT('Ctrl Pts',(6.99999999137289,10.7476171238347,-19.9256794472572));
#47138=CARTESIAN_POINT('Ctrl Pts',(6.99999999340022,10.6962822476428,-19.711624864826));
#47139=CARTESIAN_POINT('Ctrl Pts',(7.00000000000005,10.6384946505734,-19.499098911231));
#47140=CARTESIAN_POINT('Ctrl Pts',(7.00000000000005,10.5742967747319,-19.2883734681814));
#47141=CARTESIAN_POINT('Ctrl Pts',(7.00000000000005,10.5400974275295,-19.176116286822));
#47142=CARTESIAN_POINT('Ctrl Pts',(6.99999999798936,10.504093508003,-19.0643633763299));
#47143=CARTESIAN_POINT('Ctrl Pts',(6.99999999626517,10.4662999237067,-18.9531935123782));
#47144=CARTESIAN_POINT('Ctrl Pts',(6.99999999250277,10.3838292711404,-18.7106060098555));
#47145=CARTESIAN_POINT('Ctrl Pts',(6.99999999167269,10.2928334595614,-18.4707958679957));
#47146=CARTESIAN_POINT('Ctrl Pts',(6.99999999476598,10.1936291084844,-18.234499293281));
#47147=CARTESIAN_POINT('Ctrl Pts',(6.99999999683537,10.1272621312739,-18.0764186323145));
#47148=CARTESIAN_POINT('Ctrl Pts',(7.00000000000005,10.0572224760596,-17.9199102275781));
#47149=CARTESIAN_POINT('Ctrl Pts',(7.00000000000005,9.98361708049291,-17.765189800066));
#47150=CARTESIAN_POINT('Ctrl Pts',(7.00000000000005,9.91648607953027,-17.6240787159086));
#47151=CARTESIAN_POINT('Ctrl Pts',(6.99999999705136,9.84637810930485,-17.4844629690789));
#47152=CARTESIAN_POINT('Ctrl Pts',(6.99999999409833,9.77333028856548,-17.3464250463554));
#47153=CARTESIAN_POINT('Ctrl Pts',(6.99999998947413,9.65894344405889,-17.1302690783503));
#47154=CARTESIAN_POINT('Ctrl Pts',(6.99999998692745,9.53734971276868,-16.9179803553399));
#47155=CARTESIAN_POINT('Ctrl Pts',(6.99999999182225,9.40869665247457,-16.7098917675291));
#47156=CARTESIAN_POINT('Ctrl Pts',(6.99999999469974,9.33306577083223,-16.5875633649255));
#47157=CARTESIAN_POINT('Ctrl Pts',(7.00000000000005,9.25499448752809,-16.4666870596751));
#47158=CARTESIAN_POINT('Ctrl Pts',(7.00000000000005,9.17450657072659,-16.3473361667542));
#47159=CARTESIAN_POINT('Ctrl Pts',(7.00000000000005,9.06569816815992,-16.1859904577374));
#47160=CARTESIAN_POINT('Ctrl Pts',(6.99999998960196,8.95252125830182,-16.027385824795));
#47161=CARTESIAN_POINT('Ctrl Pts',(6.99999998461871,8.83522853413698,-15.8719380527288));
#47162=CARTESIAN_POINT('Ctrl Pts',(6.99999997943771,8.71328140858451,-15.7103218134268));
#47163=CARTESIAN_POINT('Ctrl Pts',(6.99999998080586,8.58688537844239,-15.5521184867226));
#47164=CARTESIAN_POINT('Ctrl Pts',(6.99999998755719,8.45642472370038,-15.3977016699108));
#47165=CARTESIAN_POINT('Ctrl Pts',(6.99999999250482,8.36081825447468,-15.284539225083));
#47166=CARTESIAN_POINT('Ctrl Pts',(7.00000000000005,8.26302974978129,-15.1734096595939));
#47167=CARTESIAN_POINT('Ctrl Pts',(7.00000000000005,8.16322280872337,-15.0644472405567));
#47168=CARTESIAN_POINT('Ctrl Pts',(7.00000000000005,8.05103332172495,-14.9419664014054));
#47169=CARTESIAN_POINT('Ctrl Pts',(6.99999999328023,7.93625106258992,-14.8222864757151));
#47170=CARTESIAN_POINT('Ctrl Pts',(6.99999999271608,7.81883217509785,-14.7052852661705));
#47171=CARTESIAN_POINT('Ctrl Pts',(6.9999999924934,7.77248661607701,-14.6591045657885));
#47172=CARTESIAN_POINT('Ctrl Pts',(6.99999999280614,7.72572983592215,-14.6133415237277));
#47173=CARTESIAN_POINT('Ctrl Pts',(6.99999999341965,7.6785573913367,-14.5679900171479));
#47174=CARTESIAN_POINT('Ctrl Pts',(6.99999999496859,7.55946070981941,-14.4534906736664));
#47175=CARTESIAN_POINT('Ctrl Pts',(6.99999999795298,7.43771702120765,-14.3416119007437));
#47176=CARTESIAN_POINT('Ctrl Pts',(6.99999999909583,7.3132546940743,-14.2323043265284));
#47177=CARTESIAN_POINT('Ctrl Pts',(7.00000000010504,7.20334631839466,-14.1357785889161));
#47178=CARTESIAN_POINT('Ctrl Pts',(6.99999999999947,7.09131727001927,-14.0412582116215));
#47179=CARTESIAN_POINT('Ctrl Pts',(6.99999999999947,6.97709641029447,-13.9487350316524));
#47180=CARTESIAN_POINT('',(6.27159471697239,11.8794981306056,-24.2690139179354));
#47181=CARTESIAN_POINT('Origin',(5.999999877385,10.9277801432447,-24.1259420367213));
#47182=CARTESIAN_POINT('Ctrl Pts',(6.27159470456933,11.8794980693479,-24.2690136413586));
#47183=CARTESIAN_POINT('Ctrl Pts',(6.27193966899897,11.91387827254,-24.0395181149413));
#47184=CARTESIAN_POINT('Ctrl Pts',(6.2722578256641,11.9412741933855,-23.8113319282651));
#47185=CARTESIAN_POINT('Ctrl Pts',(6.27254917027625,11.9620370246289,-23.5849163959185));
#47186=CARTESIAN_POINT('Ctrl Pts',(6.27284515817359,11.9831307621011,-23.3548923812278));
#47187=CARTESIAN_POINT('Ctrl Pts',(6.27311347258153,11.9973783276931,-23.1266958622964));
#47188=CARTESIAN_POINT('Ctrl Pts',(6.27335410993762,12.0051465928033,-22.9007563434725));
#47189=CARTESIAN_POINT('Ctrl Pts',(6.27354178808869,12.0112052266602,-22.7245413457914));
#47190=CARTESIAN_POINT('Ctrl Pts',(6.27371263094733,12.0133226280565,-22.5496981157126));
#47191=CARTESIAN_POINT('Ctrl Pts',(6.27386663718285,12.0116720903008,-22.3764084710348));
#47192=CARTESIAN_POINT('Ctrl Pts',(6.27406868749932,12.0095066476175,-22.1490590560667));
#47193=CARTESIAN_POINT('Ctrl Pts',(6.27424175785168,12.0008569236811,-21.9243852895248));
#47194=CARTESIAN_POINT('Ctrl Pts',(6.27438584598699,11.9862082353842,-21.7027333745298));
#47195=CARTESIAN_POINT('Ctrl Pts',(6.27447251908356,11.9773966342575,-21.5694034664637));
#47196=CARTESIAN_POINT('Ctrl Pts',(6.27454870537683,11.9664140727742,-21.4371659889583));
#47197=CARTESIAN_POINT('Ctrl Pts',(6.27461440451541,11.9533633512297,-21.3060877049261));
#47198=CARTESIAN_POINT('Ctrl Pts',(6.27472591355225,11.9312127809046,-21.0836127453143));
#47199=CARTESIAN_POINT('Ctrl Pts',(6.27480721201525,11.9031053535267,-20.8644797536233));
#47200=CARTESIAN_POINT('Ctrl Pts',(6.27485829884291,11.8695299317154,-20.6489747555412));
#47201=CARTESIAN_POINT('Ctrl Pts',(6.27487121254234,11.8610427555617,-20.5944995238963));
#47202=CARTESIAN_POINT('Ctrl Pts',(6.27488219579953,11.8522061030633,-20.5402558654031));
#47203=CARTESIAN_POINT('Ctrl Pts',(6.27489124860539,11.8430276976174,-20.4862479066156));
#47204=CARTESIAN_POINT('Ctrl Pts',(6.27492812667111,11.8056379817079,-20.2662377700162));
#47205=CARTESIAN_POINT('Ctrl Pts',(6.27493296937425,11.7625789016338,-20.0501427398753));
#47206=CARTESIAN_POINT('Ctrl Pts',(6.27490577664845,11.7143943118651,-19.8381869763113));
#47207=CARTESIAN_POINT('Ctrl Pts',(6.27488257757199,11.6732863335747,-19.6573600154728));
#47208=CARTESIAN_POINT('Ctrl Pts',(6.27483606184378,11.6284473802591,-19.4795448890848));
#47209=CARTESIAN_POINT('Ctrl Pts',(6.27476622992978,11.5802014285004,-19.3048541862108));
#47210=CARTESIAN_POINT('Ctrl Pts',(6.27472435194866,11.551268481639,-19.200092716301));
#47211=CARTESIAN_POINT('Ctrl Pts',(6.2746740886978,11.5211100139789,-19.0964544409574));
#47212=CARTESIAN_POINT('Ctrl Pts',(6.27461544169057,11.489793764837,-18.9939596243062));
#47213=CARTESIAN_POINT('Ctrl Pts',(6.27458611818695,11.474135640266,-18.9427122159807));
#47214=CARTESIAN_POINT('Ctrl Pts',(6.27455469611227,11.458188061523,-18.8917506750642));
#47215=CARTESIAN_POINT('Ctrl Pts',(6.2745211789115,11.4419593308387,-18.8410772071659));
#47216=CARTESIAN_POINT('Ctrl Pts',(6.27450442031112,11.4338449654966,-18.8157404732167));
#47217=CARTESIAN_POINT('Ctrl Pts',(6.27448713775144,11.4256603115726,-18.7904757576991));
#47218=CARTESIAN_POINT('Ctrl Pts',(6.27446933123306,11.4174064002052,-18.7652833275414));
#47219=CARTESIAN_POINT('Ctrl Pts',(6.27445391940419,11.4102625067896,-18.7434788729119));
#47220=CARTESIAN_POINT('Ctrl Pts',(6.27443872975055,11.403338950616,-18.7225457109356));
#47221=CARTESIAN_POINT('Ctrl Pts',(6.27442216602411,11.395929825651,-18.7003621758541));
#47222=CARTESIAN_POINT('Ctrl Pts',(6.27441959235278,11.3947785960287,-18.6969152988161));
#47223=CARTESIAN_POINT('Ctrl Pts',(6.27441698550732,11.3936155468417,-18.6934382660929));
#47224=CARTESIAN_POINT('Ctrl Pts',(6.27441433949973,11.3924379209365,-18.689923155043));
#47225=CARTESIAN_POINT('Ctrl Pts',(6.27440279752698,11.3873010777388,-18.6745901242335));
#47226=CARTESIAN_POINT('Ctrl Pts',(6.27439106572956,11.3821298476611,-18.6592579804075));
#47227=CARTESIAN_POINT('Ctrl Pts',(6.27437914410846,11.3769241436459,-18.643926888831));
#47228=CARTESIAN_POINT('Ctrl Pts',(6.27420011134086,11.2987475610068,-18.4136924490583));
#47229=CARTESIAN_POINT('Ctrl Pts',(6.27397826846476,11.2127950847352,-18.1836912011832));
#47230=CARTESIAN_POINT('Ctrl Pts',(6.27371361975783,11.1188688560928,-17.9544927346738));
#47231=CARTESIAN_POINT('Ctrl Pts',(6.27345239300995,11.0261571117798,-17.728257848731));
#47232=CARTESIAN_POINT('Ctrl Pts',(6.27314946023938,10.9256764527698,-17.5028050812689));
#47233=CARTESIAN_POINT('Ctrl Pts',(6.27280482739841,10.8172505232637,-17.2787308995921));
#47234=CARTESIAN_POINT('Ctrl Pts',(6.27260798345405,10.7553208836645,-17.1507464462612));
#47235=CARTESIAN_POINT('Ctrl Pts',(6.272397535514,10.6907994758282,-17.0232126335942));
#47236=CARTESIAN_POINT('Ctrl Pts',(6.27217348498568,10.6236555852736,-16.8962479574695));
#47237=CARTESIAN_POINT('Ctrl Pts',(6.27177013698152,10.5027794844665,-16.6676792096146));
#47238=CARTESIAN_POINT('Ctrl Pts',(6.27132270396134,10.3734026228786,-16.4409516713369));
#47239=CARTESIAN_POINT('Ctrl Pts',(6.27083119612744,10.2354142164086,-16.2167887268486));
#47240=CARTESIAN_POINT('Ctrl Pts',(6.27036732554269,10.1051848316808,-16.0052303569369));
#47241=CARTESIAN_POINT('Ctrl Pts',(6.26986419868896,9.9672852585331,-15.7959566509888));
#47242=CARTESIAN_POINT('Ctrl Pts',(6.26932182550144,9.82164211896925,-15.5896237836272));
#47243=CARTESIAN_POINT('Ctrl Pts',(6.26905884966486,9.75102537877976,-15.4895809355352));
#47244=CARTESIAN_POINT('Ctrl Pts',(6.26878664742083,9.67858849328747,-15.3902301631767));
#47245=CARTESIAN_POINT('Ctrl Pts',(6.26850522012318,9.60432480000494,-15.2916503518621));
#47246=CARTESIAN_POINT('Ctrl Pts',(6.26791729758894,9.44918242710482,-15.0857098017579));
#47247=CARTESIAN_POINT('Ctrl Pts',(6.26728911457511,9.28606521508869,-14.8831314821586));
#47248=CARTESIAN_POINT('Ctrl Pts',(6.26662068570985,9.11502603156112,-14.6845483878654));
#47249=CARTESIAN_POINT('Ctrl Pts',(6.2659595690909,8.94585792318419,-14.4881376840467));
#47250=CARTESIAN_POINT('Ctrl Pts',(6.26525908231365,8.76894017634307,-14.2956352473713));
#47251=CARTESIAN_POINT('Ctrl Pts',(6.26451924289097,8.5843553372276,-14.107693790117));
#47252=CARTESIAN_POINT('Ctrl Pts',(6.26430323665952,8.53046327057285,-14.0528217129189));
#47253=CARTESIAN_POINT('Ctrl Pts',(6.26408387592249,8.47591784790006,-13.998338691807));
#47254=CARTESIAN_POINT('Ctrl Pts',(6.26386116117568,8.42072164460613,-13.9442616338722));
#47255=CARTESIAN_POINT('Ctrl Pts',(6.99999999998951,9.33248386900998,-24.7867299441529));
#47256=CARTESIAN_POINT('Ctrl Pts',(6.99999999998951,9.33249195738903,-24.7867268023194));
#47257=CARTESIAN_POINT('Ctrl Pts',(6.99999999998951,9.60233986589691,-24.6819075265188));
#47258=CARTESIAN_POINT('Ctrl Pts',(6.99999999998951,10.1365881548997,-24.4674868372888));
#47259=CARTESIAN_POINT('Ctrl Pts',(6.99999999998951,10.6659288230102,-24.2412740855147));
#47260=CARTESIAN_POINT('Ctrl Pts',(6.99999999998951,10.9277807259391,-24.1259369153972));
#47261=CARTESIAN_POINT('Ctrl Pts',(7.00000270566769,9.54650236981204,-25.3377021349734));
#47262=CARTESIAN_POINT('Ctrl Pts',(7.00000270566769,9.54651058119136,-25.3376989453619));
#47263=CARTESIAN_POINT('Ctrl Pts',(7.00000270566769,9.82046207621099,-25.2312856794742));
#47264=CARTESIAN_POINT('Ctrl Pts',(7.00000270566769,10.3628264314847,-25.0136075515436));
#47265=CARTESIAN_POINT('Ctrl Pts',(7.00000270566769,10.9002087461683,-24.783958270892));
#47266=CARTESIAN_POINT('Ctrl Pts',(7.00000270566769,11.1660426386392,-24.6668671648011));
#47267=CARTESIAN_POINT('Ctrl Pts',(6.57967198012589,9.69699923069234,-25.7251433367391));
#47268=CARTESIAN_POINT('Ctrl Pts',(6.57967198012589,9.6970075285649,-25.7251401135304));
#47269=CARTESIAN_POINT('Ctrl Pts',(6.57967198012589,9.97384464742593,-25.6176059608812));
#47270=CARTESIAN_POINT('Ctrl Pts',(6.57967198012589,10.5219161845169,-25.3976372164973));
#47271=CARTESIAN_POINT('Ctrl Pts',(6.57967198012589,11.0649533494165,-25.1655713839739));
#47272=CARTESIAN_POINT('Ctrl Pts',(6.57967198012589,11.3335873592823,-25.0472469178922));
#47273=CARTESIAN_POINT('Ctrl Pts',(5.98852436209119,9.69454278461807,-25.7188194279642));
#47274=CARTESIAN_POINT('Ctrl Pts',(5.98852436209119,9.69455108107884,-25.7188162053039));
#47275=CARTESIAN_POINT('Ctrl Pts',(5.98852436209119,9.9713411000889,-25.611300348033));
#47276=CARTESIAN_POINT('Ctrl Pts',(5.98852436209119,10.519319483182,-25.3913689916453));
#47277=CARTESIAN_POINT('Ctrl Pts',(5.98852436209119,11.062264348252,-25.159342602665));
#47278=CARTESIAN_POINT('Ctrl Pts',(5.98852436209119,11.330852653926,-25.0410382677823));
#47279=CARTESIAN_POINT('',(6.99999999994009,9.33250873275974,-24.7867180661797));
#47280=CARTESIAN_POINT('',(5.98852583803805,9.69456766152529,-25.7188097331007));
#47281=CARTESIAN_POINT('Origin',(5.999999999061,9.33250979146072,-24.7867247845918));
#47282=CARTESIAN_POINT('',(5.98852581751677,11.3308503372889,-25.041038957009));
#47283=CARTESIAN_POINT('Origin',(5.98846864787388,-4.75314843312467,11.4751155009116));
#47284=CARTESIAN_POINT('Origin',(6.,10.9277801936247,-24.1259421517584));
#47285=CARTESIAN_POINT('Origin',(6.9999999787379,-4.74946026808531,11.4664779416658));
#47286=CARTESIAN_POINT('Origin',(5.999999877385,10.9277801432447,-24.1259420367213));
#47287=CARTESIAN_POINT('Origin',(5.99999763275393,10.9277792104516,-24.1259401189103));
#47288=CARTESIAN_POINT('Ctrl Pts',(-6.094431914356,11.2713279469382,-25.06822360013));
#47289=CARTESIAN_POINT('Ctrl Pts',(-6.05633875273873,11.2835945308545,-25.0623206876246));
#47290=CARTESIAN_POINT('Ctrl Pts',(-5.71232895575907,11.3934006872462,-25.0095886523243));
#47291=CARTESIAN_POINT('Ctrl Pts',(-5.02622191935904,11.5949850066956,-24.9146104214381));
#47292=CARTESIAN_POINT('Ctrl Pts',(-3.98582966114027,11.8491084122632,-24.7976169741646));
#47293=CARTESIAN_POINT('Ctrl Pts',(-2.81226414593484,12.0688095588167,-24.6984861183588));
#47294=CARTESIAN_POINT('Ctrl Pts',(-1.52049089173392,12.2251956038408,-24.6294270360226));
#47295=CARTESIAN_POINT('Ctrl Pts',(-0.189402768830715,12.2883719696366,
-24.602518522178));
#47296=CARTESIAN_POINT('Ctrl Pts',(1.08608586084807,12.2535038348118,-24.6172525448486));
#47297=CARTESIAN_POINT('Ctrl Pts',(2.24125031189288,12.1446943722227,-24.6648482773845));
#47298=CARTESIAN_POINT('Ctrl Pts',(3.27297079100125,11.9869972429091,-24.7352727477233));
#47299=CARTESIAN_POINT('Ctrl Pts',(4.19996253752107,11.7980284275134,-24.8210647839224));
#47300=CARTESIAN_POINT('Ctrl Pts',(5.05700893760704,11.5844416805762,-24.9196521454285));
#47301=CARTESIAN_POINT('Ctrl Pts',(5.68046392601282,11.4027971502045,-25.0051676719571));
#47302=CARTESIAN_POINT('Ctrl Pts',(6.02236021770785,11.294542540446,-25.0570504367922));
#47303=CARTESIAN_POINT('Ctrl Pts',(6.09429718612962,11.2713792138499,-25.0681981524802));
#47304=CARTESIAN_POINT('Ctrl Pts',(-6.21850174075154,11.6026144911347,-24.9351568017923));
#47305=CARTESIAN_POINT('Ctrl Pts',(-6.17967941190587,11.6150637612153,-24.9290290295733));
#47306=CARTESIAN_POINT('Ctrl Pts',(-5.82908090970353,11.726491587308,-24.8742543611295));
#47307=CARTESIAN_POINT('Ctrl Pts',(-5.12975016911477,11.9308145015291,-24.7750066996334));
#47308=CARTESIAN_POINT('Ctrl Pts',(-4.06876019721386,12.1879451786412,-24.6515284137366));
#47309=CARTESIAN_POINT('Ctrl Pts',(-2.87125002534106,12.4098505899583,-24.5458499626876));
#47310=CARTESIAN_POINT('Ctrl Pts',(-1.55244063361097,12.5674388783431,-24.4713861765985));
#47311=CARTESIAN_POINT('Ctrl Pts',(-0.193343170191578,12.6308275658389,
-24.4418368498252));
#47312=CARTESIAN_POINT('Ctrl Pts',(1.10885808493883,12.5958746635933,-24.4580801160618));
#47313=CARTESIAN_POINT('Ctrl Pts',(2.28833313380122,12.4863530460059,-24.5096523636422));
#47314=CARTESIAN_POINT('Ctrl Pts',(3.34139767194732,12.3272452030784,-24.5851371770129));
#47315=CARTESIAN_POINT('Ctrl Pts',(4.28714760515426,12.1362723269595,-24.6763093639965));
#47316=CARTESIAN_POINT('Ctrl Pts',(5.16111360517402,11.9201148911425,-24.7802386217786));
#47317=CARTESIAN_POINT('Ctrl Pts',(5.79660359327198,11.736017123652,-24.8696394150045));
#47318=CARTESIAN_POINT('Ctrl Pts',(6.1450501863258,11.626174088922,-24.9235557444498));
#47319=CARTESIAN_POINT('Ctrl Pts',(6.21836436549247,11.6026655148077,-24.9351277338151));
#47320=CARTESIAN_POINT('Ctrl Pts',(-6.32914231245861,11.8134514838489,-24.6414301321201));
#47321=CARTESIAN_POINT('Ctrl Pts',(-6.28961575230152,11.826020158596,-24.6351228661687));
#47322=CARTESIAN_POINT('Ctrl Pts',(-5.93266612704154,11.9384843908636,-24.578725067509));
#47323=CARTESIAN_POINT('Ctrl Pts',(-5.22080330516413,12.1441505239257,-24.4762093893228));
#47324=CARTESIAN_POINT('Ctrl Pts',(-4.14080139185458,12.4019094797043,-24.3479823384532));
#47325=CARTESIAN_POINT('Ctrl Pts',(-2.92180263005805,12.6234437730966,-24.2376755293907));
#47326=CARTESIAN_POINT('Ctrl Pts',(-1.57941068834376,12.7799962770451,-24.1595144784238));
#47327=CARTESIAN_POINT('Ctrl Pts',(-0.196615490582365,12.8424503644217,
-24.1282201087162));
#47328=CARTESIAN_POINT('Ctrl Pts',(1.1279890562748,12.8080728412826,-24.1454554856207));
#47329=CARTESIAN_POINT('Ctrl Pts',(2.32846050235933,12.6995118079923,-24.1997176236243));
#47330=CARTESIAN_POINT('Ctrl Pts',(3.40038217913011,12.5410385067355,-24.2787204343849));
#47331=CARTESIAN_POINT('Ctrl Pts',(4.36310491630567,12.3501384318674,-24.3737347034933));
#47332=CARTESIAN_POINT('Ctrl Pts',(5.25272701250916,12.1333494366402,-24.4815931017532));
#47333=CARTESIAN_POINT('Ctrl Pts',(5.89960976867062,11.9480757051294,-24.5739613947287));
#47334=CARTESIAN_POINT('Ctrl Pts',(6.25435740425776,11.8372353972519,-24.6294877375989));
#47335=CARTESIAN_POINT('Ctrl Pts',(6.32900167463278,11.813500894588,-24.6413984641695));
#47336=CARTESIAN_POINT('Ctrl Pts',(-6.39488491639353,11.843659109667,-24.2701454915518));
#47337=CARTESIAN_POINT('Ctrl Pts',(-6.3548792244511,11.8562498366404,-24.263755202918));
#47338=CARTESIAN_POINT('Ctrl Pts',(-5.99362126599835,11.9688694024556,-24.2066159318454));
#47339=CARTESIAN_POINT('Ctrl Pts',(-5.27348053464344,12.1740985697827,-24.1027645072777));
#47340=CARTESIAN_POINT('Ctrl Pts',(-4.18145826340194,12.4299229451767,-23.9728780259458));
#47341=CARTESIAN_POINT('Ctrl Pts',(-2.94953848407,12.6486104098926,-23.8611815544649));
#47342=CARTESIAN_POINT('Ctrl Pts',(-1.5937263245113,12.8021783961345,-23.7820850898753));
#47343=CARTESIAN_POINT('Ctrl Pts',(-0.19828839899972,12.8628139539125,-23.7504393128011));
#47344=CARTESIAN_POINT('Ctrl Pts',(1.13803452697083,12.8295099441217,-23.7678665979002));
#47345=CARTESIAN_POINT('Ctrl Pts',(2.35021459441548,12.723313039055,-23.8227647798885));
#47346=CARTESIAN_POINT('Ctrl Pts',(3.4331426425149,12.5673438207858,-23.9027401395622));
#47347=CARTESIAN_POINT('Ctrl Pts',(4.40622596342085,12.3785773849159,-23.9989632401039));
#47348=CARTESIAN_POINT('Ctrl Pts',(5.30578912917227,12.1632797707017,-24.1082183846146));
#47349=CARTESIAN_POINT('Ctrl Pts',(5.96018372008034,11.9784443662577,-24.2017911337946));
#47350=CARTESIAN_POINT('Ctrl Pts',(6.31919213586667,11.867482639712,-24.2580455020914));
#47351=CARTESIAN_POINT('Ctrl Pts',(6.39474132614597,11.8437059930189,-24.2701129850578));
#47352=CARTESIAN_POINT('',(-5.98852245733775,11.3308498383565,-25.0410395152735));
#47353=CARTESIAN_POINT('Ctrl Pts',(-5.98852261949162,11.3308502493357,-25.0410393033403));
#47354=CARTESIAN_POINT('Ctrl Pts',(-5.87206434378358,11.3676808033278,-25.0233565226301));
#47355=CARTESIAN_POINT('Ctrl Pts',(-5.74891036709195,11.4056203108354,-25.0052460172911));
#47356=CARTESIAN_POINT('Ctrl Pts',(-5.61905842407995,11.4443053364402,-24.9868889199126));
#47357=CARTESIAN_POINT('Ctrl Pts',(-5.51153067681731,11.4763396176347,-24.9716877817424));
#47358=CARTESIAN_POINT('Ctrl Pts',(-5.39940999143908,11.5088843415234,-24.9563177908387));
#47359=CARTESIAN_POINT('Ctrl Pts',(-5.28269811087122,11.5417066610665,-24.9408868513054));
#47360=CARTESIAN_POINT('Ctrl Pts',(-5.21045748179925,11.5620225449325,-24.9313356318954));
#47361=CARTESIAN_POINT('Ctrl Pts',(-5.13645747600364,11.5824416608345,-24.9217623183797));
#47362=CARTESIAN_POINT('Ctrl Pts',(-5.06069821746738,11.6028970082404,-24.9121963780487));
#47363=CARTESIAN_POINT('Ctrl Pts',(-5.00135512740382,11.6189199148375,-24.9047032680372));
#47364=CARTESIAN_POINT('Ctrl Pts',(-4.94093262964919,11.6349649716179,-24.8972146778942));
#47365=CARTESIAN_POINT('Ctrl Pts',(-4.8794305921878,11.6509987287575,-24.8897461628098));
#47366=CARTESIAN_POINT('Ctrl Pts',(-4.80942185405327,11.6692502071026,-24.8812446344316));
#47367=CARTESIAN_POINT('Ctrl Pts',(-4.73801437161174,11.687486798311,-24.8727692375187));
#47368=CARTESIAN_POINT('Ctrl Pts',(-4.66520814405306,11.7056554054938,-24.8643442713963));
#47369=CARTESIAN_POINT('Ctrl Pts',(-4.62880503027372,11.7147397090852,-24.8601317883351));
#47370=CARTESIAN_POINT('Ctrl Pts',(-4.59205223025826,11.7238070144719,-24.8559319079964));
#47371=CARTESIAN_POINT('Ctrl Pts',(-4.55494974407041,11.7328503323779,-24.8517477910442));
#47372=CARTESIAN_POINT('Ctrl Pts',(-4.53639850097649,11.7373719913309,-24.8496557325681));
#47373=CARTESIAN_POINT('Ctrl Pts',(-4.51775983634088,11.7418876532688,-24.8475676146158));
#47374=CARTESIAN_POINT('Ctrl Pts',(-4.49903375017708,11.7463964357147,-24.8454838338858));
#47375=CARTESIAN_POINT('Ctrl Pts',(-4.48967070709519,11.7486508269376,-24.8444419435208));
#47376=CARTESIAN_POINT('Ctrl Pts',(-4.48028580863127,11.7509034982779,-24.8434011374401));
#47377=CARTESIAN_POINT('Ctrl Pts',(-4.47087905478714,11.7531543382301,-24.8423614656213));
#47378=CARTESIAN_POINT('Ctrl Pts',(-4.46147230094301,11.7554051781823,-24.8413217938026));
#47379=CARTESIAN_POINT('Ctrl Pts',(-4.45080026163169,11.7579498409444,-24.8401467680703));
#47380=CARTESIAN_POINT('Ctrl Pts',(-4.44259322711588,11.7599012520483,-24.8392459029919));
#47381=CARTESIAN_POINT('Ctrl Pts',(-4.30856578831259,11.7917693563927,-24.8245340556212));
#47382=CARTESIAN_POINT('Ctrl Pts',(-4.17021571232689,11.8233378307119,-24.8100191830527));
#47383=CARTESIAN_POINT('Ctrl Pts',(-4.02753511600434,11.854287492411,-24.7958396904698));
#47384=CARTESIAN_POINT('Ctrl Pts',(-3.89063485295398,11.8839833090611,-24.7822346431504));
#47385=CARTESIAN_POINT('Ctrl Pts',(-3.74974763050038,11.9131091571202,-24.7689383171711));
#47386=CARTESIAN_POINT('Ctrl Pts',(-3.60488117571044,11.9413675073944,-24.7560825402895));
#47387=CARTESIAN_POINT('Ctrl Pts',(-3.4569563762176,11.9702224331561,-24.7429553589812));
#47388=CARTESIAN_POINT('Ctrl Pts',(-3.30487851548619,11.9981719243682,-24.7302880082315));
#47389=CARTESIAN_POINT('Ctrl Pts',(-3.14864759365074,12.0248803860776,-24.7182264051025));
#47390=CARTESIAN_POINT('Ctrl Pts',(-3.07053213273301,12.0382346169323,-24.7121956035379));
#47391=CARTESIAN_POINT('Ctrl Pts',(-2.99137840642891,12.0512783404329,-24.7063163011558));
#47392=CARTESIAN_POINT('Ctrl Pts',(-2.91118641388078,12.0639682856377,-24.7006069887942));
#47393=CARTESIAN_POINT('Ctrl Pts',(-2.89492183652573,12.0665420662466,-24.6994490233964));
#47394=CARTESIAN_POINT('Ctrl Pts',(-2.87861455189655,12.0691012967118,-24.6982980484005));
#47395=CARTESIAN_POINT('Ctrl Pts',(-2.86226455461567,12.0716456047884,-24.6971542220298));
#47396=CARTESIAN_POINT('Ctrl Pts',(-2.83830797547933,12.0753736126124,-24.6954782482362));
#47397=CARTESIAN_POINT('Ctrl Pts',(-2.81425969567364,12.079069583887,-24.6938176217293));
#47398=CARTESIAN_POINT('Ctrl Pts',(-2.7901197252096,12.0827323810601,-24.6921728353577));
#47399=CARTESIAN_POINT('Ctrl Pts',(-2.76981216045503,12.0858136810512,-24.6907891714547));
#47400=CARTESIAN_POINT('Ctrl Pts',(-2.74943970405002,12.0888715008226,-24.6894167189943));
#47401=CARTESIAN_POINT('Ctrl Pts',(-2.72900235600345,12.0919051557977,-24.6880557739761));
#47402=CARTESIAN_POINT('Ctrl Pts',(-2.71878368198016,12.0934219832853,-24.687375301467));
#47403=CARTESIAN_POINT('Ctrl Pts',(-2.70854878504645,12.0949327695685,-24.6866977058071));
#47404=CARTESIAN_POINT('Ctrl Pts',(-2.69829766520351,12.0964374288369,-24.6860230240256));
#47405=CARTESIAN_POINT('Ctrl Pts',(-2.68804654536057,12.0979420881053,-24.6853483422442));
#47406=CARTESIAN_POINT('Ctrl Pts',(-2.67637482462903,12.0996444193795,-24.6845852371531));
#47407=CARTESIAN_POINT('Ctrl Pts',(-2.66749563694813,12.1009329397115,-24.6840077573249));
#47408=CARTESIAN_POINT('Ctrl Pts',(-2.48177212083922,12.1278845635803,-24.67192877127));
#47409=CARTESIAN_POINT('Ctrl Pts',(-2.29115211409166,12.1528042226412,-24.6608136069641));
#47410=CARTESIAN_POINT('Ctrl Pts',(-2.09562977712304,12.175220720871,-24.6508597438541));
#47411=CARTESIAN_POINT('Ctrl Pts',(-1.99202712449424,12.187098692029,-24.6455854276911));
#47412=CARTESIAN_POINT('Ctrl Pts',(-1.88704840017349,12.1982731209495,-24.6406374110466));
#47413=CARTESIAN_POINT('Ctrl Pts',(-1.78069528395011,12.2086687666313,-24.6360467563646));
#47414=CARTESIAN_POINT('Ctrl Pts',(-1.69992409321344,12.2165638684395,-24.6325603268353));
#47415=CARTESIAN_POINT('Ctrl Pts',(-1.61836026605962,12.224010927817,-24.629279446292));
#47416=CARTESIAN_POINT('Ctrl Pts',(-1.53600234379191,12.2309786067084,-24.6262166791347));
#47417=CARTESIAN_POINT('Ctrl Pts',(-1.46181103399259,12.2372553704852,-24.623457616002));
#47418=CARTESIAN_POINT('Ctrl Pts',(-1.38697529504412,12.2431430893884,-24.620875568631));
#47419=CARTESIAN_POINT('Ctrl Pts',(-1.31149638890661,12.2486185489259,-24.6184788953444));
#47420=CARTESIAN_POINT('Ctrl Pts',(-1.23186331041638,12.2543953642169,-24.6159503150865));
#47421=CARTESIAN_POINT('Ctrl Pts',(-1.15151359877784,12.2597132633044,-24.6136280968113));
#47422=CARTESIAN_POINT('Ctrl Pts',(-1.07044725243966,12.2645452944849,-24.6115216096605));
#47423=CARTESIAN_POINT('Ctrl Pts',(-1.02991407927057,12.2669613100752,-24.610468366085));
#47424=CARTESIAN_POINT('Ctrl Pts',(-0.989201747425264,12.269255856687,-24.6094690513367));
#47425=CARTESIAN_POINT('Ctrl Pts',(-0.948310256806896,12.2714255828555,
-24.6085247974033));
#47426=CARTESIAN_POINT('Ctrl Pts',(-0.927864511497712,12.2725104459398,
-24.6080526704366));
#47427=CARTESIAN_POINT('Ctrl Pts',(-0.907373976495706,12.2735641037824,
-24.6075943084147));
#47428=CARTESIAN_POINT('Ctrl Pts',(-0.886838651798443,12.2745861390056,
-24.6071498500979));
#47429=CARTESIAN_POINT('Ctrl Pts',(-0.876570989449812,12.2750971566172,
-24.6069276209395));
#47430=CARTESIAN_POINT('Ctrl Pts',(-0.866292129677403,12.2756002685656,
-24.6067088676909));
#47431=CARTESIAN_POINT('Ctrl Pts',(-0.856002072481586,12.276095422804,-24.6064936075101));
#47432=CARTESIAN_POINT('Ctrl Pts',(-0.84571201528577,12.2765905770423,-24.6062783473294));
#47433=CARTESIAN_POINT('Ctrl Pts',(-0.833723425588129,12.2771561786407,
-24.6060325049814));
#47434=CARTESIAN_POINT('Ctrl Pts',(-0.82509830862458,12.2775569603653,-24.6058583232348));
#47435=CARTESIAN_POINT('Ctrl Pts',(-0.60331200137841,12.2878626639384,-24.6013794128003));
#47436=CARTESIAN_POINT('Ctrl Pts',(-0.37942147470136,12.2940995949959,-24.5986970076597));
#47437=CARTESIAN_POINT('Ctrl Pts',(-0.153422040659201,12.2960206310907,
-24.5978631981353));
#47438=CARTESIAN_POINT('Ctrl Pts',(-0.0981746725502134,12.2964902437192,
-24.5976593667323));
#47439=CARTESIAN_POINT('Ctrl Pts',(-0.0428013115823766,12.2967017237989,
-24.5975660637919));
#47440=CARTESIAN_POINT('Ctrl Pts',(0.0126974871764322,12.2966538031459,
-24.5975843468163));
#47441=CARTESIAN_POINT('Ctrl Pts',(0.15396086503864,12.2965318287344,-24.597630883351));
#47442=CARTESIAN_POINT('Ctrl Pts',(0.296039615275695,12.2947248108631,-24.5984025596996));
#47443=CARTESIAN_POINT('Ctrl Pts',(0.43893375204779,12.2912000474167,-24.5999229059135));
#47444=CARTESIAN_POINT('Ctrl Pts',(0.510380820433836,12.2894376656936,-24.6006830790204));
#47445=CARTESIAN_POINT('Ctrl Pts',(0.582031734977933,12.2872458491615,-24.6016304233117));
#47446=CARTESIAN_POINT('Ctrl Pts',(0.65388649564414,12.2846217901291,-24.6027672829694));
#47447=CARTESIAN_POINT('Ctrl Pts',(0.689813875977243,12.2833097606128,-24.6033357127982));
#47448=CARTESIAN_POINT('Ctrl Pts',(0.725792217826846,12.2818896707049,-24.6039515219213));
#47449=CARTESIAN_POINT('Ctrl Pts',(0.761821521118555,12.2803612097145,-24.6046149872946));
#47450=CARTESIAN_POINT('Ctrl Pts',(0.779836172764409,12.2795969792193,-24.6049467199812));
#47451=CARTESIAN_POINT('Ctrl Pts',(0.797863564770144,12.2788056559728,-24.6052903667671));
#47452=CARTESIAN_POINT('Ctrl Pts',(0.815903697124266,12.2779872059043,-24.6056459601989));
#47453=CARTESIAN_POINT('Ctrl Pts',(0.833943829478388,12.2771687558359,-24.6060015536307));
#47454=CARTESIAN_POINT('Ctrl Pts',(0.853616708411465,12.2762449172183,-24.6064031266869));
#47455=CARTESIAN_POINT('Ctrl Pts',(0.870062315218929,12.2754504426786,-24.6067486124422));
#47456=CARTESIAN_POINT('Ctrl Pts',(0.95490688162133,12.2713516673258,-24.6085310087654));
#47457=CARTESIAN_POINT('Ctrl Pts',(1.03913119396567,12.2666920819471,-24.6105613373092));
#47458=CARTESIAN_POINT('Ctrl Pts',(1.12272942610553,12.2614987222179,-24.6128297808952));
#47459=CARTESIAN_POINT('Ctrl Pts',(1.3402298823131,12.2479869758395,-24.6187316702318));
#47460=CARTESIAN_POINT('Ctrl Pts',(1.553491070849,12.2308655865203,-24.6262443285959));
#47461=CARTESIAN_POINT('Ctrl Pts',(1.76251278772209,12.2106188688103,-24.6351844059209));
#47462=CARTESIAN_POINT('Ctrl Pts',(1.93917904843176,12.193506235908,-24.6427406065641));
#47463=CARTESIAN_POINT('Ctrl Pts',(2.11281720147879,12.174160036699,-24.6513167790797));
#47464=CARTESIAN_POINT('Ctrl Pts',(2.28343846124246,12.1528471286757,-24.6608097041831));
#47465=CARTESIAN_POINT('Ctrl Pts',(2.3146215826453,12.1489519341422,-24.6625446523154));
#47466=CARTESIAN_POINT('Ctrl Pts',(2.34570395955438,12.1449909873965,-24.6643102395043));
#47467=CARTESIAN_POINT('Ctrl Pts',(2.37668568819775,12.1409658927933,-24.6661058189143));
#47468=CARTESIAN_POINT('Ctrl Pts',(2.477450908615,12.1278746431226,-24.6719457756552));
#47469=CARTESIAN_POINT('Ctrl Pts',(2.57802287628754,12.1139949965248,-24.6781518005778));
#47470=CARTESIAN_POINT('Ctrl Pts',(2.67763147125897,12.0994620485983,-24.6846663127365));
#47471=CARTESIAN_POINT('Ctrl Pts',(2.77938420239324,12.084616270045,-24.6913210537691));
#47472=CARTESIAN_POINT('Ctrl Pts',(2.88013149186452,12.0690888669585,-24.6982976933924));
#47473=CARTESIAN_POINT('Ctrl Pts',(2.97906267521312,12.0530722864747,-24.7055117542209));
#47474=CARTESIAN_POINT('Ctrl Pts',(3.01306542757817,12.0475673708203,-24.7079912345586));
#47475=CARTESIAN_POINT('Ctrl Pts',(3.04685374015803,12.0420050730082,-24.7104985660293));
#47476=CARTESIAN_POINT('Ctrl Pts',(3.08039501457754,12.0363944358889,-24.7130297203968));
#47477=CARTESIAN_POINT('Ctrl Pts',(3.1589490848206,12.0232542559167,-24.7189577145299));
#47478=CARTESIAN_POINT('Ctrl Pts',(3.2363619939274,12.0098153834099,-24.7250314766478));
#47479=CARTESIAN_POINT('Ctrl Pts',(3.31263226369929,11.9961218910734,-24.7312316528785));
#47480=CARTESIAN_POINT('Ctrl Pts',(3.45643416665273,11.9703038329761,-24.7429216225521));
#47481=CARTESIAN_POINT('Ctrl Pts',(3.59617381541188,11.9435821435806,-24.7550605159897));
#47482=CARTESIAN_POINT('Ctrl Pts',(3.73185546034114,11.9162415601785,-24.7675242517846));
#47483=CARTESIAN_POINT('Ctrl Pts',(3.83567798906037,11.89532076056,-24.7770614044938));
#47484=CARTESIAN_POINT('Ctrl Pts',(3.93712341204653,11.874037281912,-24.7867888199111));
#47485=CARTESIAN_POINT('Ctrl Pts',(4.03619172864908,11.8525110818394,-24.7966530844071));
#47486=CARTESIAN_POINT('Ctrl Pts',(4.06095880779972,11.8471295318213,-24.7991191505311));
#47487=CARTESIAN_POINT('Ctrl Pts',(4.08659007135158,11.8415152815526,-24.8016933679325));
#47488=CARTESIAN_POINT('Ctrl Pts',(4.11454680505952,11.8353264265799,-24.8045332735786));
#47489=CARTESIAN_POINT('Ctrl Pts',(4.14250353876745,11.8291375716072,-24.8073731792247));
#47490=CARTESIAN_POINT('Ctrl Pts',(4.17028170984898,11.8229263741544,-24.810225435238));
#47491=CARTESIAN_POINT('Ctrl Pts',(4.19788131832375,11.8166954630904,-24.8130888540882));
#47492=CARTESIAN_POINT('Ctrl Pts',(4.20564503586813,11.8149427196198,-24.8138943283827));
#47493=CARTESIAN_POINT('Ctrl Pts',(4.21339462460221,11.8131884156165,-24.8147006862325));
#47494=CARTESIAN_POINT('Ctrl Pts',(4.22113008395014,11.8114326080531,-24.8155079018423));
#47495=CARTESIAN_POINT('Ctrl Pts',(4.26839292874062,11.8007048081103,-24.8204399045018));
#47496=CARTESIAN_POINT('Ctrl Pts',(4.31512830212096,11.7899209103131,-24.8254039196623));
#47497=CARTESIAN_POINT('Ctrl Pts',(4.36133621816581,11.7790939163167,-24.830394262819));
#47498=CARTESIAN_POINT('Ctrl Pts',(4.5192928999517,11.7420830274521,-24.8474532023575));
#47499=CARTESIAN_POINT('Ctrl Pts',(4.6710868612562,11.7045739579164,-24.8648180143462));
#47500=CARTESIAN_POINT('Ctrl Pts',(4.81671584757079,11.6670461923498,-24.8822738066032));
#47501=CARTESIAN_POINT('Ctrl Pts',(4.86938363032469,11.6534740028144,-24.8885868209121));
#47502=CARTESIAN_POINT('Ctrl Pts',(4.92124518390333,11.6398989012584,-24.894911863262));
#47503=CARTESIAN_POINT('Ctrl Pts',(4.97230079099022,11.6263420121853,-24.9012392056704));
#47504=CARTESIAN_POINT('Ctrl Pts',(5.00457282564062,11.6177727595824,-24.9052386922126));
#47505=CARTESIAN_POINT('Ctrl Pts',(5.03652280196598,11.6092116132764,-24.9092387214196));
#47506=CARTESIAN_POINT('Ctrl Pts',(5.06815068438951,11.6006631633034,-24.9132371465457));
#47507=CARTESIAN_POINT('Ctrl Pts',(5.21038989559504,11.5622184528763,-24.931219154585));
#47508=CARTESIAN_POINT('Ctrl Pts',(5.34611433022111,11.5240346408721,-24.9491680609103));
#47509=CARTESIAN_POINT('Ctrl Pts',(5.47532353418555,11.4865031871949,-24.9669056709416));
#47510=CARTESIAN_POINT('Ctrl Pts',(5.60704917663317,11.4482407825369,-24.9849887331784));
#47511=CARTESIAN_POINT('Ctrl Pts',(5.73200353346943,11.4106562721611,-25.0028520396424));
#47512=CARTESIAN_POINT('Ctrl Pts',(5.85018815143144,11.3741116577444,-25.0203170142959));
#47513=CARTESIAN_POINT('Ctrl Pts',(5.86232620871315,11.370358372158,-25.0221107406406));
#47514=CARTESIAN_POINT('Ctrl Pts',(5.87439285795211,11.3666160114644,-25.0239002752262));
#47515=CARTESIAN_POINT('Ctrl Pts',(5.88638810071823,11.3628849378978,-25.0256854315412));
#47516=CARTESIAN_POINT('Ctrl Pts',(5.92102970000301,11.3521098032951,-25.030840864485));
#47517=CARTESIAN_POINT('Ctrl Pts',(5.95507574647161,11.3414288270981,-25.0359597835312));
#47518=CARTESIAN_POINT('Ctrl Pts',(5.98852582557461,11.3308501354092,-25.0410382780203));
#47519=CARTESIAN_POINT('',(-6.27159361731535,11.8794975616035,-24.2690120888704));
#47520=CARTESIAN_POINT('Origin',(-5.999994980806,10.9277770011849,-24.1259380084193));
#47521=CARTESIAN_POINT('Ctrl Pts',(-6.27159386307714,11.8794985003159,-24.2690123725043));
#47522=CARTESIAN_POINT('Ctrl Pts',(-6.19708063788404,11.9025009437873,-24.2574475519448));
#47523=CARTESIAN_POINT('Ctrl Pts',(-6.1154389212118,11.9272858632909,-24.2450493518731));
#47524=CARTESIAN_POINT('Ctrl Pts',(-6.02658468059905,11.9536191513622,-24.2319368683802));
#47525=CARTESIAN_POINT('Ctrl Pts',(-5.93855991338491,11.9797066125399,-24.2189467927338));
#47526=CARTESIAN_POINT('Ctrl Pts',(-5.84345650103252,12.0073138014567,-24.2052557265519));
#47527=CARTESIAN_POINT('Ctrl Pts',(-5.74118376321366,12.0361672962737,-24.1909996607511));
#47528=CARTESIAN_POINT('Ctrl Pts',(-5.64049526534308,12.064573840514,-24.1769644263216));
#47529=CARTESIAN_POINT('Ctrl Pts',(-5.53285766402706,12.0941884806745,-24.1623815976342));
#47530=CARTESIAN_POINT('Ctrl Pts',(-5.41817807500658,12.1247040286673,-24.1474001686258));
#47531=CARTESIAN_POINT('Ctrl Pts',(-5.37925205568429,12.1350620079812,-24.1423149795348));
#47532=CARTESIAN_POINT('Ctrl Pts',(-5.33951465291907,12.1455233798207,-24.1371840288087));
#47533=CARTESIAN_POINT('Ctrl Pts',(-5.29896211848521,12.1560748552828,-24.1320136472455));
#47534=CARTESIAN_POINT('Ctrl Pts',(-5.21821342548053,12.1770850797912,-24.1217183214566));
#47535=CARTESIAN_POINT('Ctrl Pts',(-5.13423279998965,12.1984532303221,-24.1112662958196));
#47536=CARTESIAN_POINT('Ctrl Pts',(-5.04699089619075,12.2200666393085,-24.1007138120776));
#47537=CARTESIAN_POINT('Ctrl Pts',(-4.92201131250236,12.2510292242542,-24.0855967070222));
#47538=CARTESIAN_POINT('Ctrl Pts',(-4.79033868087646,12.282497284018,-24.0702723742906));
#47539=CARTESIAN_POINT('Ctrl Pts',(-4.65188708480657,12.3140998001835,-24.0549259456217));
#47540=CARTESIAN_POINT('Ctrl Pts',(-4.51343548873669,12.3457023163489,-24.0395795169528));
#47541=CARTESIAN_POINT('Ctrl Pts',(-4.36820473066936,12.3774395505853,-24.024210870021));
#47542=CARTESIAN_POINT('Ctrl Pts',(-4.21611190204382,12.4088902288773,-24.0090300413631));
#47543=CARTESIAN_POINT('Ctrl Pts',(-4.07082877054265,12.4389327566637,-23.9945289084291));
#47544=CARTESIAN_POINT('Ctrl Pts',(-3.91928373183408,12.4687134990666,-23.9801991837209));
#47545=CARTESIAN_POINT('Ctrl Pts',(-3.76142159657237,12.4978246559702,-23.9662477012005));
#47546=CARTESIAN_POINT('Ctrl Pts',(-3.73054731973014,12.5035181423527,-23.9635191055625));
#47547=CARTESIAN_POINT('Ctrl Pts',(-3.69943144642957,12.5091858792516,-23.9608050504824));
#47548=CARTESIAN_POINT('Ctrl Pts',(-3.66807361915617,12.5148246128436,-23.9581071905609));
#47549=CARTESIAN_POINT('Ctrl Pts',(-3.58017497289932,12.530630460775,-23.9505448606574));
#47550=CARTESIAN_POINT('Ctrl Pts',(-3.49037512701031,12.5462087349511,-23.9431096148398));
#47551=CARTESIAN_POINT('Ctrl Pts',(-3.39866710774328,12.5614848736542,-23.935839448839));
#47552=CARTESIAN_POINT('Ctrl Pts',(-3.35281309810976,12.5691229430058,-23.9322043658387));
#47553=CARTESIAN_POINT('Ctrl Pts',(-3.3064820361792,12.5766854208569,-23.9286105461331));
#47554=CARTESIAN_POINT('Ctrl Pts',(-3.25967322046985,12.5841625651488,-23.9250630070349));
#47555=CARTESIAN_POINT('Ctrl Pts',(-3.23626881261517,12.5879011372948,-23.9232892374858));
#47556=CARTESIAN_POINT('Ctrl Pts',(-3.21274496571995,12.5916183723679,-23.9215270376585));
#47557=CARTESIAN_POINT('Ctrl Pts',(-3.18910159606633,12.5953130280354,-23.9197770413011));
#47558=CARTESIAN_POINT('Ctrl Pts',(-3.17727991123952,12.5971603558692,-23.9189020431224));
#47559=CARTESIAN_POINT('Ctrl Pts',(-3.16542834568841,12.5990020386154,-23.9180300957842));
#47560=CARTESIAN_POINT('Ctrl Pts',(-3.15354688958086,12.6008379193071,-23.9171612794639));
#47561=CARTESIAN_POINT('Ctrl Pts',(-3.14166543347331,12.6026737999988,-23.9162924631437));
#47562=CARTESIAN_POINT('Ctrl Pts',(-3.12814004437027,12.6047504362156,-23.9153102011917));
#47563=CARTESIAN_POINT('Ctrl Pts',(-3.11781283988084,12.6063279972199,-23.914564303968));
#47564=CARTESIAN_POINT('Ctrl Pts',(-3.07662101472915,12.6126203696738,-23.9115891650469));
#47565=CARTESIAN_POINT('Ctrl Pts',(-3.03568844271223,12.6187482436968,-23.9086933705156));
#47566=CARTESIAN_POINT('Ctrl Pts',(-2.99501685896893,12.6247159725055,-23.9058747757425));
#47567=CARTESIAN_POINT('Ctrl Pts',(-2.79740091771027,12.6537120979859,-23.892179728541));
#47568=CARTESIAN_POINT('Ctrl Pts',(-2.60595035920182,12.6789291266892,-23.880306669677));
#47569=CARTESIAN_POINT('Ctrl Pts',(-2.42085823416444,12.7008772951465,-23.8700052682326));
#47570=CARTESIAN_POINT('Ctrl Pts',(-2.23093018158733,12.7233989064354,-23.8594347206484));
#47571=CARTESIAN_POINT('Ctrl Pts',(-2.04769684133198,12.7424789282856,-23.8505188343068));
#47572=CARTESIAN_POINT('Ctrl Pts',(-1.87131798152509,12.758644782564,-23.8429959900435));
#47573=CARTESIAN_POINT('Ctrl Pts',(-1.78117118117997,12.7669071108251,-23.8391510828899));
#47574=CARTESIAN_POINT('Ctrl Pts',(-1.69281416813676,12.7744077891968,-23.8356702264102));
#47575=CARTESIAN_POINT('Ctrl Pts',(-1.60626396046494,12.7812145160159,-23.8325195992654));
#47576=CARTESIAN_POINT('Ctrl Pts',(-1.43907018368183,12.7943634430379,-23.8264333602402));
#47577=CARTESIAN_POINT('Ctrl Pts',(-1.27862092434264,12.8049252529317,-23.8215783807087));
#47578=CARTESIAN_POINT('Ctrl Pts',(-1.12501574086879,12.8133804823945,-23.8177149964479));
#47579=CARTESIAN_POINT('Ctrl Pts',(-0.969938834043967,12.8219167231771,
-23.8138145962954));
#47580=CARTESIAN_POINT('Ctrl Pts',(-0.82183738744044,12.8283059524179,-23.8109247713977));
#47581=CARTESIAN_POINT('Ctrl Pts',(-0.680781472353746,12.8330037303229,
-23.8088158751191));
#47582=CARTESIAN_POINT('Ctrl Pts',(-0.538387190839892,12.8377460816741,
-23.8066869692154));
#47583=CARTESIAN_POINT('Ctrl Pts',(-0.40317239011466,12.8407648691305,-23.8053537705296));
#47584=CARTESIAN_POINT('Ctrl Pts',(-0.2751822190389,12.8424872425574,-23.8045989425387));
#47585=CARTESIAN_POINT('Ctrl Pts',(-0.236222340744794,12.8430115285907,
-23.8043691748432));
#47586=CARTESIAN_POINT('Ctrl Pts',(-0.197931715385525,12.8434153954412,
-23.8041931354355));
#47587=CARTESIAN_POINT('Ctrl Pts',(-0.160311209395224,12.8437101078661,
-23.8040650611514));
#47588=CARTESIAN_POINT('Ctrl Pts',(-0.153998805357433,12.8437595581288,
-23.8040435713652));
#47589=CARTESIAN_POINT('Ctrl Pts',(-0.147705267480093,12.8438059344178,
-23.804023432385));
#47590=CARTESIAN_POINT('Ctrl Pts',(-0.141430599074373,12.843849289921,-23.8040046162681));
#47591=CARTESIAN_POINT('Ctrl Pts',(-0.103047863108373,12.8441144996061,
-23.8038895163139));
#47592=CARTESIAN_POINT('Ctrl Pts',(-0.0662557649282347,12.844264401576,
-23.8038251195063));
#47593=CARTESIAN_POINT('Ctrl Pts',(-0.0289811583181769,12.8443170156573,
-23.8038019482852));
#47594=CARTESIAN_POINT('Ctrl Pts',(-0.0185590826975259,12.8443317266893,
-23.8037954695523));
#47595=CARTESIAN_POINT('Ctrl Pts',(-0.00809928444716131,12.8443385554483,
-23.803792357389));
#47596=CARTESIAN_POINT('Ctrl Pts',(0.00244355322809239,12.8443372524163,
-23.8037927386336));
#47597=CARTESIAN_POINT('Ctrl Pts',(0.127127961177523,12.8443218421664,-23.8037972474059));
#47598=CARTESIAN_POINT('Ctrl Pts',(0.258986374602228,12.8431696770572,-23.8042924738699));
#47599=CARTESIAN_POINT('Ctrl Pts',(0.397985575007477,12.8404650174786,-23.8054910540718));
#47600=CARTESIAN_POINT('Ctrl Pts',(0.535666628784619,12.8377860065216,-23.8066782679893));
#47601=CARTESIAN_POINT('Ctrl Pts',(0.680354002368223,12.8335836937305,-23.8085556417309));
#47602=CARTESIAN_POINT('Ctrl Pts',(0.831993459648986,12.8274126547388,-23.8113495682372));
#47603=CARTESIAN_POINT('Ctrl Pts',(0.942266738698048,12.8229250318144,-23.8133813312283));
#47604=CARTESIAN_POINT('Ctrl Pts',(1.05621605905989,12.8173954294566,-23.8158982066978));
#47605=CARTESIAN_POINT('Ctrl Pts',(1.17381162283179,12.8106390770448,-23.8189935431595));
#47606=CARTESIAN_POINT('Ctrl Pts',(1.33437225665151,12.8014142033273,-23.8232198010917));
#47607=CARTESIAN_POINT('Ctrl Pts',(1.5017320685743,12.7899032047958,-23.8285241622485));
#47608=CARTESIAN_POINT('Ctrl Pts',(1.67578004683143,12.7756204063144,-23.8351494352146));
#47609=CARTESIAN_POINT('Ctrl Pts',(1.8437866770057,12.7618333754834,-23.8415447395218));
#47610=CARTESIAN_POINT('Ctrl Pts',(2.01802545755619,12.7454633391203,-23.8491710217748));
#47611=CARTESIAN_POINT('Ctrl Pts',(2.19835985514866,12.7260475950067,-23.8582571155746));
#47612=CARTESIAN_POINT('Ctrl Pts',(2.26108424966836,12.7192943587415,-23.8614174651238));
#47613=CARTESIAN_POINT('Ctrl Pts',(2.32454574572609,12.7121724347413,-23.8647545068279));
#47614=CARTESIAN_POINT('Ctrl Pts',(2.38873742216605,12.7046616766872,-23.8682781206306));
#47615=CARTESIAN_POINT('Ctrl Pts',(2.47500004842828,12.6945685033834,-23.8730132544892));
#47616=CARTESIAN_POINT('Ctrl Pts',(2.56258134583149,12.6837731521358,-23.8780853123256));
#47617=CARTESIAN_POINT('Ctrl Pts',(2.65146464768891,12.6722277501361,-23.8835179324179));
#47618=CARTESIAN_POINT('Ctrl Pts',(2.72897721473141,12.6621593376465,-23.8882555639001));
#47619=CARTESIAN_POINT('Ctrl Pts',(2.80747997654866,12.6515204820078,-23.8932674650598));
#47620=CARTESIAN_POINT('Ctrl Pts',(2.88696064472235,12.6402790323444,-23.8985693852204));
#47621=CARTESIAN_POINT('Ctrl Pts',(2.92670097880919,12.6346583075128,-23.9012203453007));
#47622=CARTESIAN_POINT('Ctrl Pts',(2.96668578829657,12.6288869265186,-23.9039438092491));
#47623=CARTESIAN_POINT('Ctrl Pts',(3.00691341611986,12.6229608373452,-23.9067417717684));
#47624=CARTESIAN_POINT('Ctrl Pts',(3.0270272300315,12.6199977927584,-23.9081407530281));
#47625=CARTESIAN_POINT('Ctrl Pts',(3.04720174847246,12.6169960706657,-23.90955835888));
#47626=CARTESIAN_POINT('Ctrl Pts',(3.06743675972051,12.6139551624287,-23.9109948380374));
#47627=CARTESIAN_POINT('Ctrl Pts',(3.07755426534454,12.6124347083102,-23.9117130776161));
#47628=CARTESIAN_POINT('Ctrl Pts',(3.08768689416621,12.6109044576268,-23.9124360355178));
#47629=CARTESIAN_POINT('Ctrl Pts',(3.09783461924249,12.6093643466848,-23.9131637428685));
#47630=CARTESIAN_POINT('Ctrl Pts',(3.10798234431877,12.6078242357429,-23.9138914502192));
#47631=CARTESIAN_POINT('Ctrl Pts',(3.11649243293453,12.6065275675155,-23.9145041910091));
#47632=CARTESIAN_POINT('Ctrl Pts',(3.12832305613605,12.6047143692937,-23.9153611443954));
#47633=CARTESIAN_POINT('Ctrl Pts',(3.24396819268312,12.5869902348685,-23.9237379213154));
#47634=CARTESIAN_POINT('Ctrl Pts',(3.35682173873388,12.5687084797174,-23.9324156970004));
#47635=CARTESIAN_POINT('Ctrl Pts',(3.46689179393769,12.5500057596089,-23.9413244112923));
#47636=CARTESIAN_POINT('Ctrl Pts',(3.6391299746952,12.5207396483061,-23.9552648126092));
#47637=CARTESIAN_POINT('Ctrl Pts',(3.80455199630043,12.4904455345154,-23.9697692758995));
#47638=CARTESIAN_POINT('Ctrl Pts',(3.96321409848656,12.4596117546677,-23.9845901751178));
#47639=CARTESIAN_POINT('Ctrl Pts',(4.12187620067269,12.4287779748199,-23.999411074336));
#47640=CARTESIAN_POINT('Ctrl Pts',(4.27377865463948,12.3974042624314,-24.0145485508317));
#47641=CARTESIAN_POINT('Ctrl Pts',(4.41898996525194,12.3659261737581,-24.0297825391726));
#47642=CARTESIAN_POINT('Ctrl Pts',(4.56351963026574,12.3345958483719,-24.0449450166851));
#47643=CARTESIAN_POINT('Ctrl Pts',(4.70142133579754,12.3031619818066,-24.0602033369487));
#47644=CARTESIAN_POINT('Ctrl Pts',(4.8327759042808,12.2720083557111,-24.0753672902913));
#47645=CARTESIAN_POINT('Ctrl Pts',(4.90532428615046,12.2548019106769,-24.0837424864527));
#47646=CARTESIAN_POINT('Ctrl Pts',(4.97587555827759,12.2376800953812,-24.0920893088182));
#47647=CARTESIAN_POINT('Ctrl Pts',(5.04444364113545,12.2207014823019,-24.1003786547038));
#47648=CARTESIAN_POINT('Ctrl Pts',(5.13538850289719,12.1981820015896,-24.1113731784565));
#47649=CARTESIAN_POINT('Ctrl Pts',(5.22284458178628,12.1759148649416,-24.1222663823038));
#47650=CARTESIAN_POINT('Ctrl Pts',(5.30684444827954,12.1540256279075,-24.1329957660341));
#47651=CARTESIAN_POINT('Ctrl Pts',(5.42689922171342,12.1227409663661,-24.1483304777022));
#47652=CARTESIAN_POINT('Ctrl Pts',(5.53989448945818,12.0922301987086,-24.1633298754751));
#47653=CARTESIAN_POINT('Ctrl Pts',(5.64592729865616,12.0628173208656,-24.1778362675318));
#47654=CARTESIAN_POINT('Ctrl Pts',(5.75378658155754,12.0328977899561,-24.192592540204));
#47655=CARTESIAN_POINT('Ctrl Pts',(5.85444162547483,12.0041142009824,-24.2068386546953));
#47656=CARTESIAN_POINT('Ctrl Pts',(5.94798723082197,11.9767580922063,-24.220429963577));
#47657=CARTESIAN_POINT('Ctrl Pts',(6.02496433639105,11.9542472103172,-24.2316140231032));
#47658=CARTESIAN_POINT('Ctrl Pts',(6.09712727222615,11.9327019687062,-24.242355090011));
#47659=CARTESIAN_POINT('Ctrl Pts',(6.16452420707849,11.9122610939159,-24.2525832257952));
#47660=CARTESIAN_POINT('Ctrl Pts',(6.20165893254129,11.9009984708423,-24.2582187790318));
#47661=CARTESIAN_POINT('Ctrl Pts',(6.23734668812422,11.8900707437737,-24.2636988187805));
#47662=CARTESIAN_POINT('Ctrl Pts',(6.2715947931636,11.8794983798023,-24.2690136880224));
#47663=CARTESIAN_POINT('Ctrl Pts',(-6.390311350217,11.8061921052281,-24.5118549102149));
#47664=CARTESIAN_POINT('Ctrl Pts',(-4.260207566811,12.4817967425171,-24.1870628120273));
#47665=CARTESIAN_POINT('Ctrl Pts',(0.0001663376444951,13.1582619823406,
-23.8622671604308));
#47666=CARTESIAN_POINT('Ctrl Pts',(4.2605402421,12.4817439180343,-24.1870881749925));
#47667=CARTESIAN_POINT('Ctrl Pts',(6.39081036315,11.8060338272127,-24.5119310012438));
#47668=CARTESIAN_POINT('Ctrl Pts',(-6.390311350217,11.9720498317925,-23.5459010687554));
#47669=CARTESIAN_POINT('Ctrl Pts',(-4.260207566811,12.6077623797797,-23.2652608575561));
#47670=CARTESIAN_POINT('Ctrl Pts',(0.0001663376444951,13.2461470249007,
-22.9846424253836));
#47671=CARTESIAN_POINT('Ctrl Pts',(4.2605402421,12.6077125289674,-23.2652827707593));
#47672=CARTESIAN_POINT('Ctrl Pts',(6.39081036315,11.9719008995601,-23.5459668160588));
#47673=CARTESIAN_POINT('Ctrl Pts',(-6.390311350217,12.0713623708286,-21.4528943057181));
#47674=CARTESIAN_POINT('Ctrl Pts',(-4.260207566811,12.6592430855888,-21.279241698184));
#47675=CARTESIAN_POINT('Ctrl Pts',(0.0001663376444951,13.245691316649,-21.1056360824358));
#47676=CARTESIAN_POINT('Ctrl Pts',(4.2605402421,12.6591972904408,-21.2792552548697));
#47677=CARTESIAN_POINT('Ctrl Pts',(6.39081036315,12.0712246444089,-21.4529349883696));
#47678=CARTESIAN_POINT('Ctrl Pts',(-6.390311350217,11.387980855255,-18.3168609136256));
#47679=CARTESIAN_POINT('Ctrl Pts',(-4.260207566811,12.0191856806278,-18.3050659001773));
#47680=CARTESIAN_POINT('Ctrl Pts',(0.0001663376444952,12.6510858022935,
-18.2929947474349));
#47681=CARTESIAN_POINT('Ctrl Pts',(4.2605402421,12.019136336187,-18.3050668428002));
#47682=CARTESIAN_POINT('Ctrl Pts',(6.39081036315,11.3878329790519,-18.3168636769111));
#47683=CARTESIAN_POINT('Ctrl Pts',(-6.390311350217,9.96966247179778,-15.6639900925141));
#47684=CARTESIAN_POINT('Ctrl Pts',(-4.260207566811,10.7489275346341,-15.7525652586985));
#47685=CARTESIAN_POINT('Ctrl Pts',(0.0001663376444948,11.5272506786203,
-15.8420539986973));
#47686=CARTESIAN_POINT('Ctrl Pts',(4.2605402421,10.7488667561688,-15.7525582706139));
#47687=CARTESIAN_POINT('Ctrl Pts',(6.39081036315,9.9694799086042,-15.6639693414749));
#47688=CARTESIAN_POINT('Ctrl Pts',(-6.390311350217,8.71289904002423,-14.2541069570423));
#47689=CARTESIAN_POINT('Ctrl Pts',(-4.260207566811,9.62695763387275,-14.3565480390593));
#47690=CARTESIAN_POINT('Ctrl Pts',(0.0001663376444956,10.5424016003325,
-14.4576175588418));
#47691=CARTESIAN_POINT('Ctrl Pts',(4.2605402421,9.62688614778384,-14.3565401466471));
#47692=CARTESIAN_POINT('Ctrl Pts',(6.39081036315,8.71268489794962,-14.2540829575325));
#47693=CARTESIAN_POINT('Ctrl Pts',(-6.390311350217,8.13905341860134,-13.7246653228991));
#47694=CARTESIAN_POINT('Ctrl Pts',(-4.260207566811,9.11397509263302,-13.8218701645398));
#47695=CARTESIAN_POINT('Ctrl Pts',(0.0001663376444956,10.0900092059685,
-13.9179922581859));
#47696=CARTESIAN_POINT('Ctrl Pts',(4.2605402421,9.11389887511922,-13.8218626584636));
#47697=CARTESIAN_POINT('Ctrl Pts',(6.39081036315,8.13882501775734,-13.7246425501129));
#47698=CARTESIAN_POINT('',(-6.26385954125917,8.42070865985895,-13.9442611207816));
#47699=CARTESIAN_POINT('Ctrl Pts',(-6.27159552384948,11.8794980574136,-24.2690121660567));
#47700=CARTESIAN_POINT('Ctrl Pts',(-6.27195777359891,11.9156534386679,-24.0278185403221));
#47701=CARTESIAN_POINT('Ctrl Pts',(-6.27229031327766,11.9441024445609,-23.7878332543352));
#47702=CARTESIAN_POINT('Ctrl Pts',(-6.27259314313179,11.9652318805478,-23.549555389302));
#47703=CARTESIAN_POINT('Ctrl Pts',(-6.27289863582238,11.986547111402,-23.3091823048629));
#47704=CARTESIAN_POINT('Ctrl Pts',(-6.27317389390371,12.0004135052366,-23.0705467116799));
#47705=CARTESIAN_POINT('Ctrl Pts',(-6.2734189176284,12.0072245125693,-22.8341074537603));
#47706=CARTESIAN_POINT('Ctrl Pts',(-6.2736675427985,12.014135630498,-22.5941929279593));
#47707=CARTESIAN_POINT('Ctrl Pts',(-6.27388503828953,12.0137824613635,-22.3565397318801));
#47708=CARTESIAN_POINT('Ctrl Pts',(-6.27407140436542,12.0065719181025,-22.1215733227915));
#47709=CARTESIAN_POINT('Ctrl Pts',(-6.27421804490314,12.0008983643939,-21.9366920325141));
#47710=CARTESIAN_POINT('Ctrl Pts',(-6.27434541261805,11.9909791988454,-21.7534730876361));
#47711=CARTESIAN_POINT('Ctrl Pts',(-6.27445350763872,11.9770107164655,-21.5721011929313));
#47712=CARTESIAN_POINT('Ctrl Pts',(-6.27450262997305,11.970662926741,-21.4896791646682));
#47713=CARTESIAN_POINT('Ctrl Pts',(-6.27454777225262,11.9634788985147,-21.4076383087566));
#47714=CARTESIAN_POINT('Ctrl Pts',(-6.2745889344895,11.9554821775698,-21.3259943087072));
#47715=CARTESIAN_POINT('Ctrl Pts',(-6.27470712629419,11.9325206732496,-21.0915645877277));
#47716=CARTESIAN_POINT('Ctrl Pts',(-6.27479250331386,11.9028603066983,-20.8604106389224));
#47717=CARTESIAN_POINT('Ctrl Pts',(-6.27484506554851,11.8670439026963,-20.6328684248961));
#47718=CARTESIAN_POINT('Ctrl Pts',(-6.27489762778317,11.8312274986943,-20.4053262108699));
#47719=CARTESIAN_POINT('Ctrl Pts',(-6.2749173752328,11.7892550183211,-20.1813955414873));
#47720=CARTESIAN_POINT('Ctrl Pts',(-6.27490430789742,11.7416481097758,-19.9613622676294));
#47721=CARTESIAN_POINT('Ctrl Pts',(-6.27489476776732,11.7068915134432,-19.800721555747));
#47722=CARTESIAN_POINT('Ctrl Pts',(-6.27486753874024,11.6690645752864,-19.6418696984425));
#47723=CARTESIAN_POINT('Ctrl Pts',(-6.27482283800117,11.6284224018795,-19.4852203578817));
#47724=CARTESIAN_POINT('Ctrl Pts',(-6.27477792037291,11.5875830315618,-19.3278109505361));
#47725=CARTESIAN_POINT('Ctrl Pts',(-6.27471536107492,11.5439012264961,-19.1726257824396));
#47726=CARTESIAN_POINT('Ctrl Pts',(-6.2746353804689,11.4976813102105,-19.0200578211033));
#47727=CARTESIAN_POINT('Ctrl Pts',(-6.27457691089758,11.4638923852968,-18.9085234912273));
#47728=CARTESIAN_POINT('Ctrl Pts',(-6.274509130865,11.4287479827558,-18.7983873253195));
#47729=CARTESIAN_POINT('Ctrl Pts',(-6.27443212646492,11.3923813207739,-18.6897925952231));
#47730=CARTESIAN_POINT('Ctrl Pts',(-6.2743563547694,11.3565968248678,-18.5829362750997));
#47731=CARTESIAN_POINT('Ctrl Pts',(-6.27427024762582,11.3190562081082,-18.4758583357969));
#47732=CARTESIAN_POINT('Ctrl Pts',(-6.27417380503419,11.2797074661642,-18.3686262100786));
#47733=CARTESIAN_POINT('Ctrl Pts',(-6.27399075538353,11.2050228963577,-18.1650978434006));
#47734=CARTESIAN_POINT('Ctrl Pts',(-6.27377047261781,11.1238235000032,-17.9610111481595));
#47735=CARTESIAN_POINT('Ctrl Pts',(-6.27351295673702,11.0358412016767,-17.7568354684592));
#47736=CARTESIAN_POINT('Ctrl Pts',(-6.2732582330049,10.9488128626037,-17.5548735895199));
#47737=CARTESIAN_POINT('Ctrl Pts',(-6.27296707919006,10.8551478403144,-17.3528245563033));
#47738=CARTESIAN_POINT('Ctrl Pts',(-6.27263949529251,10.754600520291,-17.1511912440502));
#47739=CARTESIAN_POINT('Ctrl Pts',(-6.27231699856497,10.6556146363325,-16.9526891691644));
#47740=CARTESIAN_POINT('Ctrl Pts',(-6.27195919444132,10.549958495229,-16.7545899618257));
#47741=CARTESIAN_POINT('Ctrl Pts',(-6.27156608292156,10.437412155432,-16.5574217276117));
#47742=CARTESIAN_POINT('Ctrl Pts',(-6.27136275152317,10.3791991458823,-16.4554392346946));
#47743=CARTESIAN_POINT('Ctrl Pts',(-6.27114997423131,10.3191430227536,-16.3537066057444));
#47744=CARTESIAN_POINT('Ctrl Pts',(-6.27092775104597,10.2572149753916,-16.2523021740491));
#47745=CARTESIAN_POINT('Ctrl Pts',(-6.27050608299771,10.1397066297922,-16.0598874683938));
#47746=CARTESIAN_POINT('Ctrl Pts',(-6.27005040567849,10.0154574689945,-15.8686514742631));
#47747=CARTESIAN_POINT('Ctrl Pts',(-6.26956071861759,9.88428240632285,-15.6791662493658));
#47748=CARTESIAN_POINT('Ctrl Pts',(-6.26938505208526,9.8372256833115,-15.6111917917125));
#47749=CARTESIAN_POINT('Ctrl Pts',(-6.26920500887961,9.78927782249918,-15.5434430983117));
#47750=CARTESIAN_POINT('Ctrl Pts',(-6.2690205889789,9.74043078877536,-15.475948142725));
#47751=CARTESIAN_POINT('Ctrl Pts',(-6.26850854175106,9.60480557636394,-15.2885464319087));
#47752=CARTESIAN_POINT('Ctrl Pts',(-6.26796275408184,9.46224623827901,-15.1030978701136));
#47753=CARTESIAN_POINT('Ctrl Pts',(-6.26738322550613,9.31269281092479,-14.9201597106969));
#47754=CARTESIAN_POINT('Ctrl Pts',(-6.26681231337191,9.16536294666898,-14.7399414791867));
#47755=CARTESIAN_POINT('Ctrl Pts',(-6.26620865619333,9.01124537325366,-14.562159540734));
#47756=CARTESIAN_POINT('Ctrl Pts',(-6.26557225352572,8.85031207893392,-14.3873873981266));
#47757=CARTESIAN_POINT('Ctrl Pts',(-6.26502584199882,8.71213571425886,-14.2373290810205));
#47758=CARTESIAN_POINT('Ctrl Pts',(-6.26445529103124,8.5689353367174,-14.0894901472568));
#47759=CARTESIAN_POINT('Ctrl Pts',(-6.26386060034155,8.42071136787207,-13.9442583527127));
#47760=CARTESIAN_POINT('Ctrl Pts',(6.26385989003177,8.42071839535226,-13.9442649557177));
#47761=CARTESIAN_POINT('Ctrl Pts',(5.97577254680956,8.54495172007927,-13.9555523998957));
#47762=CARTESIAN_POINT('Ctrl Pts',(5.6858636247251,8.66055598080169,-13.9652104797869));
#47763=CARTESIAN_POINT('Ctrl Pts',(5.39461985275565,8.76740388601456,-13.9734951213447));
#47764=CARTESIAN_POINT('Ctrl Pts',(5.12099027440223,8.86778971419429,-13.9812787143154));
#47765=CARTESIAN_POINT('Ctrl Pts',(4.8461824249731,8.96044566896363,-13.9878501532703));
#47766=CARTESIAN_POINT('Ctrl Pts',(4.5705999557957,9.04530802050967,-13.9934329340466));
#47767=CARTESIAN_POINT('Ctrl Pts',(4.31429754858432,9.12423330573478,-13.9986251371507));
#47768=CARTESIAN_POINT('Ctrl Pts',(4.05732511675319,9.19641709480444,-14.0029623014545));
#47769=CARTESIAN_POINT('Ctrl Pts',(3.80000738078161,9.26185125996808,-14.0066322166875));
#47770=CARTESIAN_POINT('Ctrl Pts',(3.5789007966154,9.31807717339948,-14.0097856814819));
#47771=CARTESIAN_POINT('Ctrl Pts',(3.35753925618122,9.36931990538708,-14.0124466098116));
#47772=CARTESIAN_POINT('Ctrl Pts',(3.13612877765637,9.41560490622071,-14.0147385401857));
#47773=CARTESIAN_POINT('Ctrl Pts',(2.89298897625723,9.46643233762966,-14.0172554016264));
#47774=CARTESIAN_POINT('Ctrl Pts',(2.64981042803868,9.51128973564011,-14.0193424104729));
#47775=CARTESIAN_POINT('Ctrl Pts',(2.40683512391639,9.55016652404637,-14.021058970814));
#47776=CARTESIAN_POINT('Ctrl Pts',(2.1674244150099,9.58847296636557,-14.0227503481728));
#47777=CARTESIAN_POINT('Ctrl Pts',(1.92821103051466,9.62097295201155,-14.0240820878113));
#47778=CARTESIAN_POINT('Ctrl Pts',(1.68942646637008,9.64770677387914,-14.0251157328352));
#47779=CARTESIAN_POINT('Ctrl Pts',(1.45224648068838,9.67426095048804,-14.0261424319974));
#47780=CARTESIAN_POINT('Ctrl Pts',(1.21548957156862,9.69512612507554,-14.0268750438104));
#47781=CARTESIAN_POINT('Ctrl Pts',(0.97938259943816,9.71039281056508,-14.0273783103472));
#47782=CARTESIAN_POINT('Ctrl Pts',(0.744965115348874,9.72555025369582,-14.0278779757079));
#47783=CARTESIAN_POINT('Ctrl Pts',(0.511188300143692,9.73518900756007,-14.0281515795311));
#47784=CARTESIAN_POINT('Ctrl Pts',(0.278274179044154,9.73944891642537,-14.028266658906));
#47785=CARTESIAN_POINT('Ctrl Pts',(0.185516959949696,9.74114540995729,-14.0283124888572));
#47786=CARTESIAN_POINT('Ctrl Pts',(0.0928965643348469,9.74198939312604,
-14.0283332223861));
#47787=CARTESIAN_POINT('Ctrl Pts',(0.000427015751061975,9.74199199953944,
-14.0283333049114));
#47788=CARTESIAN_POINT('Ctrl Pts',(0.000284677535436571,9.74199200355149,
-14.0283333050384));
#47789=CARTESIAN_POINT('Ctrl Pts',(0.000142338952074239,9.74199200557029,
-14.0283333051166));
#47790=CARTESIAN_POINT('Ctrl Pts',(1.02735216839658E-12,9.74199200559579,
-14.0283333051459));
#47791=CARTESIAN_POINT('Ctrl Pts',(-0.229753074916458,9.74199204676546,
-14.0283333524958));
#47792=CARTESIAN_POINT('Ctrl Pts',(-0.460464115169766,9.73679441031726,
-14.0282057699318));
#47793=CARTESIAN_POINT('Ctrl Pts',(-0.691907629373254,9.72624035113783,
-14.0278832023527));
#47794=CARTESIAN_POINT('Ctrl Pts',(-0.925171026103522,9.71560330346787,
-14.0275580983659));
#47795=CARTESIAN_POINT('Ctrl Pts',(-1.15917846122486,9.69952527300279,-14.0270349177334));
#47796=CARTESIAN_POINT('Ctrl Pts',(-1.39369908217627,9.6778966747267,-14.0262489641265));
#47797=CARTESIAN_POINT('Ctrl Pts',(-1.62968668811577,9.65613278417288,-14.0254580941837));
#47798=CARTESIAN_POINT('Ctrl Pts',(-1.86619392017613,9.62874872580037,-14.0244011396557));
#47799=CARTESIAN_POINT('Ctrl Pts',(-2.10298556652029,9.5956857160992,-14.0230166836363));
#47800=CARTESIAN_POINT('Ctrl Pts',(-2.34260943261476,9.56222724604067,-14.0216156684023));
#47801=CARTESIAN_POINT('Ctrl Pts',(-2.58252455733169,9.52295320564077,-14.0198792512116));
#47802=CARTESIAN_POINT('Ctrl Pts',(-2.82248718751079,9.47785596126532,-14.0177486392004));
#47803=CARTESIAN_POINT('Ctrl Pts',(-2.92697581546807,9.45821894867745,-14.016820891719));
#47804=CARTESIAN_POINT('Ctrl Pts',(-3.03147345072008,9.4374784976985,-14.0158184661558));
#47805=CARTESIAN_POINT('Ctrl Pts',(-3.13595996870217,9.41563703601003,-14.014736804792));
#47806=CARTESIAN_POINT('Ctrl Pts',(-3.39875183271366,9.36070403086545,-14.0120163408361));
#47807=CARTESIAN_POINT('Ctrl Pts',(-3.66146917368842,9.29878661121169,-14.0087759041241));
#47808=CARTESIAN_POINT('Ctrl Pts',(-3.92376785677122,9.2298478371932,-14.0048097516279));
#47809=CARTESIAN_POINT('Ctrl Pts',(-4.1932923765918,9.15900992925567,-14.0007343390696));
#47810=CARTESIAN_POINT('Ctrl Pts',(-4.46237485432196,9.0807590675398,-13.9958926176489));
#47811=CARTESIAN_POINT('Ctrl Pts',(-4.73064192361157,8.99511526164949,-13.9900702628746));
#47812=CARTESIAN_POINT('Ctrl Pts',(-5.02409522627783,8.90143079356337,-13.9837012767655));
#47813=CARTESIAN_POINT('Ctrl Pts',(-5.31657282406583,8.79890033659665,-13.9761586571199));
#47814=CARTESIAN_POINT('Ctrl Pts',(-5.60758600825935,8.68761493815447,-13.9671747121499));
#47815=CARTESIAN_POINT('Ctrl Pts',(-5.82724861853753,8.6036144789471,-13.9603934496164));
#47816=CARTESIAN_POINT('Ctrl Pts',(-6.04607687414356,8.51462738981054,-13.9527912470521));
#47817=CARTESIAN_POINT('Ctrl Pts',(-6.26386060034155,8.42071136787207,-13.9442583527127));
#47818=CARTESIAN_POINT('Ctrl Pts',(6.38290223050635,8.3687128810708,-13.9393718887612));
#47819=CARTESIAN_POINT('Ctrl Pts',(6.33185069333287,8.39190678947241,-13.9421546546274));
#47820=CARTESIAN_POINT('Ctrl Pts',(5.69974726342303,8.67523140046431,-13.9757998821803));
#47821=CARTESIAN_POINT('Ctrl Pts',(4.36985154284018,9.17370085496103,-14.0265657717891));
#47822=CARTESIAN_POINT('Ctrl Pts',(2.2815889278797,9.66167562240798,-14.0640584776628));
#47823=CARTESIAN_POINT('Ctrl Pts',(0.00160354234010209,9.84365792812771,
-14.0750234441869));
#47824=CARTESIAN_POINT('Ctrl Pts',(-2.27862803912884,9.66215989653315,-14.0640901144711));
#47825=CARTESIAN_POINT('Ctrl Pts',(-4.36746288708299,9.17445077621545,-14.026632517581));
#47826=CARTESIAN_POINT('Ctrl Pts',(-5.69840031280849,8.67579539900824,-13.9758632341147));
#47827=CARTESIAN_POINT('Ctrl Pts',(-6.33127835061241,8.39216684434521,-13.9421858490072));
#47828=CARTESIAN_POINT('Ctrl Pts',(-6.38290560157758,8.36871136134604,-13.9393716976888));
#47829=CARTESIAN_POINT('Ctrl Pts',(6.18027446328495,7.97034175760265,-13.4733537657383));
#47830=CARTESIAN_POINT('Ctrl Pts',(6.13081737426996,7.99266609326119,-13.4761866177629));
#47831=CARTESIAN_POINT('Ctrl Pts',(5.51846302072903,8.26537074194175,-13.510454637066));
#47832=CARTESIAN_POINT('Ctrl Pts',(4.23030987628035,8.7451984323429,-13.5625812544442));
#47833=CARTESIAN_POINT('Ctrl Pts',(2.2083741148917,9.21486873360186,-13.6017979517399));
#47834=CARTESIAN_POINT('Ctrl Pts',(0.00155196199890026,9.3899873070007,
-13.6135063985893));
#47835=CARTESIAN_POINT('Ctrl Pts',(-2.20550781210377,9.21533478109097,-13.601831483555));
#47836=CARTESIAN_POINT('Ctrl Pts',(-4.22799656394489,8.74592029438878,-13.562650353087));
#47837=CARTESIAN_POINT('Ctrl Pts',(-5.51715822420132,8.26591362788774,-13.5105193424603));
#47838=CARTESIAN_POINT('Ctrl Pts',(-6.13026290690437,7.99291639770159,-13.476218374096));
#47839=CARTESIAN_POINT('Ctrl Pts',(-6.18027772914287,7.97034029398681,-13.4733535718789));
#47840=CARTESIAN_POINT('Ctrl Pts',(6.17611521160237,8.03272083803512,-12.8315071320912));
#47841=CARTESIAN_POINT('Ctrl Pts',(6.1268036055389,8.05477000112189,-12.8343123479053));
#47842=CARTESIAN_POINT('Ctrl Pts',(5.51621999278854,8.32413445990068,-12.8682474805547));
#47843=CARTESIAN_POINT('Ctrl Pts',(4.2309697607976,8.79862201718509,-12.9199037439559));
#47844=CARTESIAN_POINT('Ctrl Pts',(2.21024860961346,9.26409347188965,-12.9587969182466));
#47845=CARTESIAN_POINT('Ctrl Pts',(0.00155380889916294,9.43795850846309,
-12.9704078321066));
#47846=CARTESIAN_POINT('Ctrl Pts',(-2.20738170362344,9.26455590951104,-12.9588301760772));
#47847=CARTESIAN_POINT('Ctrl Pts',(-4.22866008373731,8.79933658603706,-12.9199722536396));
#47848=CARTESIAN_POINT('Ctrl Pts',(-5.51491866660961,8.32467091068186,-12.8683115755957));
#47849=CARTESIAN_POINT('Ctrl Pts',(-6.12625076973956,8.05501722081392,-12.8343437929296));
#47850=CARTESIAN_POINT('Ctrl Pts',(-6.17611846754463,8.03271939355596,-12.8315069384015));
#47851=CARTESIAN_POINT('Ctrl Pts',(6.37205883491417,8.51110576180117,-12.4473561916133));
#47852=CARTESIAN_POINT('Ctrl Pts',(6.32135424616034,8.53365607055721,-12.4500751281646));
#47853=CARTESIAN_POINT('Ctrl Pts',(5.69347570203072,8.80916794902699,-12.4829516268409));
#47854=CARTESIAN_POINT('Ctrl Pts',(4.3705612963381,9.29513699757964,-12.5326341666895));
#47855=CARTESIAN_POINT('Ctrl Pts',(2.28550734776402,9.77326146435145,-12.5693863519979));
#47856=CARTESIAN_POINT('Ctrl Pts',(0.00160752407789911,9.95229479522915,
-12.5801293896245));
#47857=CARTESIAN_POINT('Ctrl Pts',(-2.28254561616144,9.77373725523836,-12.5694173642325));
#47858=CARTESIAN_POINT('Ctrl Pts',(-4.36818151897362,9.29586983131238,-12.5326995597546));
#47859=CARTESIAN_POINT('Ctrl Pts',(-5.69213705177152,8.80971689183168,-12.483013570555));
#47860=CARTESIAN_POINT('Ctrl Pts',(-6.32078579437215,8.53390891051175,-12.4501056035139));
#47861=CARTESIAN_POINT('Ctrl Pts',(-6.37206218235826,8.51110428680498,-12.447356000907));
#47862=CARTESIAN_POINT('',(-6.24994617759994,8.55169242034562,-12.4626545592495));
#47863=CARTESIAN_POINT('Ctrl Pts',(-6.26386065742728,8.42071151387271,-13.9442582034044));
#47864=CARTESIAN_POINT('Ctrl Pts',(-6.25434637310214,8.4015320522143,-13.9218549829862));
#47865=CARTESIAN_POINT('Ctrl Pts',(-6.24501004821117,8.38292731079581,-13.8979905814307));
#47866=CARTESIAN_POINT('Ctrl Pts',(-6.23595412983899,8.36512533432891,-13.8726812830547));
#47867=CARTESIAN_POINT('Ctrl Pts',(-6.2271258172178,8.34777078153087,-13.8480080926499));
#47868=CARTESIAN_POINT('Ctrl Pts',(-6.21856428749895,8.33117984533034,-13.8219614612362));
#47869=CARTESIAN_POINT('Ctrl Pts',(-6.21037053095467,8.31557235347761,-13.7946046387324));
#47870=CARTESIAN_POINT('Ctrl Pts',(-6.20230307295131,8.3002054354615,-13.7676694942157));
#47871=CARTESIAN_POINT('Ctrl Pts',(-6.19459246438177,8.28579263233555,-13.7394641191199));
#47872=CARTESIAN_POINT('Ctrl Pts',(-6.18733649965018,8.27254147840909,-13.710099095204));
#47873=CARTESIAN_POINT('Ctrl Pts',(-6.18020802747487,8.25952315685577,-13.6812500360294));
#47874=CARTESIAN_POINT('Ctrl Pts',(-6.17351870157481,8.24762677503362,-13.6512818652735));
#47875=CARTESIAN_POINT('Ctrl Pts',(-6.16735769517278,8.23703574837833,-13.6203480581767));
#47876=CARTESIAN_POINT('Ctrl Pts',(-6.16655851772455,8.23566192905334,-13.6163354668229));
#47877=CARTESIAN_POINT('Ctrl Pts',(-6.16576822066994,8.23431004579379,-13.6123066933628));
#47878=CARTESIAN_POINT('Ctrl Pts',(-6.16498698947291,8.23298047175863,-13.6082621310938));
#47879=CARTESIAN_POINT('Ctrl Pts',(-6.15905579130535,8.22288619094789,-13.577555343642));
#47880=CARTESIAN_POINT('Ctrl Pts',(-6.1536480685766,8.21408021951287,-13.5459350859393));
#47881=CARTESIAN_POINT('Ctrl Pts',(-6.14883841710609,8.20671036772986,-13.5135971977432));
#47882=CARTESIAN_POINT('Ctrl Pts',(-6.14409038200413,8.1994349310009,-13.4816735897188));
#47883=CARTESIAN_POINT('Ctrl Pts',(-6.13992546528859,8.19355960821916,-13.4490512054137));
#47884=CARTESIAN_POINT('Ctrl Pts',(-6.13640216930785,8.18919262766077,-13.4159537386902));
#47885=CARTESIAN_POINT('Ctrl Pts',(-6.1328995619996,8.18485128986162,-13.3830506191498));
#47886=CARTESIAN_POINT('Ctrl Pts',(-6.13003128219596,8.18200105235029,-13.3496786993339));
#47887=CARTESIAN_POINT('Ctrl Pts',(-6.12783791167436,8.18070711233178,-13.316083169479));
#47888=CARTESIAN_POINT('Ctrl Pts',(-6.12565198276521,8.17941756236048,-13.2826016216944));
#47889=CARTESIAN_POINT('Ctrl Pts',(-6.12413653007737,8.17967399136537,-13.248898808936));
#47890=CARTESIAN_POINT('Ctrl Pts',(-6.12331218772028,8.18149509393478,-13.2152311285308));
#47891=CARTESIAN_POINT('Ctrl Pts',(-6.12248858712431,8.18331455783663,-13.1815937430341));
#47892=CARTESIAN_POINT('Ctrl Pts',(-6.12235489834618,8.1866958860133,-13.1479923024839));
#47893=CARTESIAN_POINT('Ctrl Pts',(-6.12291077007659,8.19161012802485,-13.1146833589572));
#47894=CARTESIAN_POINT('Ctrl Pts',(-6.12346935064114,8.19654831776705,-13.0812120966831));
#47895=CARTESIAN_POINT('Ctrl Pts',(-6.12472418546194,8.20303420465641,-13.0480370555447));
#47896=CARTESIAN_POINT('Ctrl Pts',(-6.12665372884193,8.21099167735592,-13.0154062086923));
#47897=CARTESIAN_POINT('Ctrl Pts',(-6.12859073792394,8.21897993874907,-12.9826491080424));
#47898=CARTESIAN_POINT('Ctrl Pts',(-6.13120753526199,8.22845076770164,-12.9504411865254));
#47899=CARTESIAN_POINT('Ctrl Pts',(-6.1344625045572,8.23928490573034,-12.9190085043198));
#47900=CARTESIAN_POINT('Ctrl Pts',(-6.13775487193949,8.25024352297854,-12.8872146751788));
#47901=CARTESIAN_POINT('Ctrl Pts',(-6.14169993700211,8.26259637936795,-12.8562146498089));
#47902=CARTESIAN_POINT('Ctrl Pts',(-6.14623721161599,8.27618448987975,-12.8262061973638));
#47903=CARTESIAN_POINT('Ctrl Pts',(-6.14954105285304,8.28607874660054,-12.8043553791778));
#47904=CARTESIAN_POINT('Ctrl Pts',(-6.15315850171545,8.29662715152438,-12.7830295350418));
#47905=CARTESIAN_POINT('Ctrl Pts',(-6.15706167140227,8.30775960757765,-12.7622906844641));
#47906=CARTESIAN_POINT('Ctrl Pts',(-6.16251763550829,8.32332087841957,-12.7333013159685));
#47907=CARTESIAN_POINT('Ctrl Pts',(-6.16853202930593,8.34002353013777,-12.7054609962895));
#47908=CARTESIAN_POINT('Ctrl Pts',(-6.17501884145997,8.35766197049687,-12.6788966167709));
#47909=CARTESIAN_POINT('Ctrl Pts',(-6.1816540436465,8.37570390161165,-12.6517245598528));
#47910=CARTESIAN_POINT('Ctrl Pts',(-6.18878317295267,8.39472411391086,-12.6258875792879));
#47911=CARTESIAN_POINT('Ctrl Pts',(-6.19630866220191,8.41449602201175,-12.6014675769469));
#47912=CARTESIAN_POINT('Ctrl Pts',(-6.20394561629464,8.43456078451306,-12.5766858743034));
#47913=CARTESIAN_POINT('Ctrl Pts',(-6.21199040546579,8.45539889874646,-12.5533631997356));
#47914=CARTESIAN_POINT('Ctrl Pts',(-6.22034090105188,8.47677914867427,-12.5315314734822));
#47915=CARTESIAN_POINT('Ctrl Pts',(-6.22889165472525,8.49867213080004,-12.5091761879146));
#47916=CARTESIAN_POINT('Ctrl Pts',(-6.23776262655085,8.52113286412999,-12.4883838248286));
#47917=CARTESIAN_POINT('Ctrl Pts',(-6.24684926282979,8.54393035742536,-12.4691375394487));
#47918=CARTESIAN_POINT('Ctrl Pts',(-6.24787884759462,8.54651348621501,-12.4669567894331));
#47919=CARTESIAN_POINT('Ctrl Pts',(-6.24891120939786,8.54910096258273,-12.4647958402509));
#47920=CARTESIAN_POINT('Ctrl Pts',(-6.24994620285641,8.55169246976548,-12.4626546312706));
#47921=CARTESIAN_POINT('Ctrl Pts',(6.24994600986387,8.55169427781047,-12.4626534555308));
#47922=CARTESIAN_POINT('Ctrl Pts',(6.23834714732467,8.55674697036125,-12.4632538750115));
#47923=CARTESIAN_POINT('Ctrl Pts',(6.2267385857704,8.56178829857455,-12.4638514563262));
#47924=CARTESIAN_POINT('Ctrl Pts',(6.21512033143819,8.56681821124616,-12.4644462123286));
#47925=CARTESIAN_POINT('Ctrl Pts',(5.96034508265897,8.67711853826633,-12.4774885424538));
#47926=CARTESIAN_POINT('Ctrl Pts',(5.70090661232431,8.78193286041189,-12.4891713191083));
#47927=CARTESIAN_POINT('Ctrl Pts',(5.43691813523151,8.88068309765021,-12.4996529176594));
#47928=CARTESIAN_POINT('Ctrl Pts',(5.2551888702222,8.9486626103564,-12.506868434116));
#47929=CARTESIAN_POINT('Ctrl Pts',(5.07130391006201,9.01376755359675,-12.5135149435913));
#47930=CARTESIAN_POINT('Ctrl Pts',(4.88530796602069,9.07579763495134,-12.5196473374325));
#47931=CARTESIAN_POINT('Ctrl Pts',(4.73779955267249,9.1249920350101,-12.5245107751285));
#47932=CARTESIAN_POINT('Ctrl Pts',(4.58896565423665,9.17225657896646,-12.529047255444));
#47933=CARTESIAN_POINT('Ctrl Pts',(4.4388298703262,9.21750139379221,-12.5332750896649));
#47934=CARTESIAN_POINT('Ctrl Pts',(4.35054152314884,9.24410790834369,-12.535761295723));
#47935=CARTESIAN_POINT('Ctrl Pts',(4.26180298671814,9.27001589812941,-12.5381407888862));
#47936=CARTESIAN_POINT('Ctrl Pts',(4.17262217431499,9.29520771022481,-12.540416752993));
#47937=CARTESIAN_POINT('Ctrl Pts',(4.05220505027363,9.32922316130868,-12.5434898922118));
#47938=CARTESIAN_POINT('Ctrl Pts',(3.93097978551739,9.36193304379587,-12.5463746310616));
#47939=CARTESIAN_POINT('Ctrl Pts',(3.80896296004634,9.39329538834622,-12.5490775242258));
#47940=CARTESIAN_POINT('Ctrl Pts',(3.74795454731081,9.4089765606214,-12.5504289708079));
#47941=CARTESIAN_POINT('Ctrl Pts',(3.68674824151337,9.42432084095514,-12.5517349456858));
#47942=CARTESIAN_POINT('Ctrl Pts',(3.62534627981748,9.43932314297662,-12.5529960128517));
#47943=CARTESIAN_POINT('Ctrl Pts',(3.59464529896954,9.44682429398735,-12.5536265464346));
#47944=CARTESIAN_POINT('Ctrl Pts',(3.56389540398993,9.45423994993378,-12.5542458524347));
#47945=CARTESIAN_POINT('Ctrl Pts',(3.53309687884755,9.46156947861001,-12.5548539913524));
#47946=CARTESIAN_POINT('Ctrl Pts',(3.51769761627636,9.46523424294812,-12.5551580608113));
#47947=CARTESIAN_POINT('Ctrl Pts',(3.50228619615571,9.46887747543691,-12.5554593384574));
#47948=CARTESIAN_POINT('Ctrl Pts',(3.48686265457938,9.47249909762948,-12.5557578308906));
#47949=CARTESIAN_POINT('Ctrl Pts',(3.47297546939743,9.47575996594551,-12.5560265901554));
#47950=CARTESIAN_POINT('Ctrl Pts',(3.46073395674727,9.47861878456373,-12.5562615773165));
#47951=CARTESIAN_POINT('Ctrl Pts',(3.44566639845783,9.4821143160989,-12.5565479383032));
#47952=CARTESIAN_POINT('Ctrl Pts',(3.44399945593332,9.48250103105628,-12.5565796187717));
#47953=CARTESIAN_POINT('Ctrl Pts',(3.4422979120268,9.48289548860676,-12.5566119220753));
#47954=CARTESIAN_POINT('Ctrl Pts',(3.44055570174106,9.48329905498223,-12.5566449587627));
#47955=CARTESIAN_POINT('Ctrl Pts',(3.14723349105595,9.55124434400876,-12.5622070853754));
#47956=CARTESIAN_POINT('Ctrl Pts',(2.85165500750086,9.61079217192647,-12.5667997901614));
#47957=CARTESIAN_POINT('Ctrl Pts',(2.55408711751812,9.66164092414786,-12.5705995014848));
#47958=CARTESIAN_POINT('Ctrl Pts',(2.47950005199353,9.67438644993023,-12.5715519205024));
#47959=CARTESIAN_POINT('Ctrl Pts',(2.40478795778839,9.68658517669469,-12.5724545017186));
#47960=CARTESIAN_POINT('Ctrl Pts',(2.32995497501033,9.69823183993254,-12.573309998081));
#47961=CARTESIAN_POINT('Ctrl Pts',(2.03343027723976,9.74438158792375,-12.5766998910251));
#47962=CARTESIAN_POINT('Ctrl Pts',(1.73500731960175,9.78186721768321,-12.5793506939259));
#47963=CARTESIAN_POINT('Ctrl Pts',(1.4350481173723,9.81050424466312,-12.5813273931514));
#47964=CARTESIAN_POINT('Ctrl Pts',(1.1412105272793,9.83855684292536,-12.5832637516042));
#47965=CARTESIAN_POINT('Ctrl Pts',(0.845898280575693,9.85811831741548,-12.5845531625828));
#47966=CARTESIAN_POINT('Ctrl Pts',(0.549457528734541,9.86896603464892,-12.5852549836228));
#47967=CARTESIAN_POINT('Ctrl Pts',(0.367266766940093,9.8756329785634,-12.5856863187518));
#47968=CARTESIAN_POINT('Ctrl Pts',(0.184649881599701,9.87900754648283,-12.5858956765151));
#47969=CARTESIAN_POINT('Ctrl Pts',(0.00168954384257825,9.87902850122962,
-12.5858966915729));
#47970=CARTESIAN_POINT('Ctrl Pts',(0.00126856427520073,9.8790285494451,
-12.5858966939085));
#47971=CARTESIAN_POINT('Ctrl Pts',(0.000847582890492026,9.87902857990227,
-12.585896695141));
#47972=CARTESIAN_POINT('Ctrl Pts',(0.000426599689475151,9.87902859260107,
-12.5858966952703));
#47973=CARTESIAN_POINT('Ctrl Pts',(-0.295036707193534,9.87903750513702,
-12.5858967859643));
#47974=CARTESIAN_POINT('Ctrl Pts',(-0.589594666757916,9.87037163946821,
-12.5852999029506));
#47975=CARTESIAN_POINT('Ctrl Pts',(-0.88292067783907,9.85320318925631,-12.5841083605291));
#47976=CARTESIAN_POINT('Ctrl Pts',(-1.16919227118,9.83644763600947,-12.5829454744071));
#47977=CARTESIAN_POINT('Ctrl Pts',(-1.45429085808452,9.81159306700723,-12.581216271102));
#47978=CARTESIAN_POINT('Ctrl Pts',(-1.73790621418847,9.77875217866173,-12.5789214638339));
#47979=CARTESIAN_POINT('Ctrl Pts',(-1.93498547871474,9.75593162969559,-12.5773268430953));
#47980=CARTESIAN_POINT('Ctrl Pts',(-2.13135422339377,9.72927182221161,-12.5754444582432));
#47981=CARTESIAN_POINT('Ctrl Pts',(-2.32690904026969,9.69884145796004,-12.5732400127974));
#47982=CARTESIAN_POINT('Ctrl Pts',(-2.41624320815342,9.68494013191632,-12.5722329688253));
#47983=CARTESIAN_POINT('Ctrl Pts',(-2.50540756274993,9.6702518021163,-12.5711587074841));
#47984=CARTESIAN_POINT('Ctrl Pts',(-2.5943952822042,9.65478713090383,-12.5700110627634));
#47985=CARTESIAN_POINT('Ctrl Pts',(-2.73628735805807,9.6301285115551,-12.5681811283324));
#47986=CARTESIAN_POINT('Ctrl Pts',(-2.87772704193816,9.60349283140064,-12.5661676436363));
#47987=CARTESIAN_POINT('Ctrl Pts',(-3.01867923181154,9.57491812838071,-12.5639494070577));
#47988=CARTESIAN_POINT('Ctrl Pts',(-3.08915532674823,9.56063077687074,-12.5628402887685));
#47989=CARTESIAN_POINT('Ctrl Pts',(-3.15950954702942,9.54585865784176,-12.5616799674469));
#47990=CARTESIAN_POINT('Ctrl Pts',(-3.2297376354622,9.53060698018096,-12.5604652815848));
#47991=CARTESIAN_POINT('Ctrl Pts',(-3.26485167967859,9.52298114135057,-12.5598579386538));
#47992=CARTESIAN_POINT('Ctrl Pts',(-3.29993419083247,9.51523541215242,-12.5592370036778));
#47993=CARTESIAN_POINT('Ctrl Pts',(-3.33498464004132,9.50737045297991,-12.5586020651489));
#47994=CARTESIAN_POINT('Ctrl Pts',(-3.35250986464574,9.50343797339365,-12.5582845958845));
#47995=CARTESIAN_POINT('Ctrl Pts',(-3.37002707375541,9.49947568627104,-12.5579636256764));
#47996=CARTESIAN_POINT('Ctrl Pts',(-3.38753620170862,9.49548367571953,-12.5576391012899));
#47997=CARTESIAN_POINT('Ctrl Pts',(-3.40305444461023,9.49194557892969,-12.5573514771278));
#47998=CARTESIAN_POINT('Ctrl Pts',(-3.42017127190382,9.48801362514177,-12.557030768135));
#47999=CARTESIAN_POINT('Ctrl Pts',(-3.43461926460173,9.48467283034959,-12.5567574607883));
#48000=CARTESIAN_POINT('Ctrl Pts',(-3.43647284382912,9.4842442290927,-12.556722397314));
#48001=CARTESIAN_POINT('Ctrl Pts',(-3.43828251345007,9.48382542630385,-12.5566881220856));
#48002=CARTESIAN_POINT('Ctrl Pts',(-3.44003927655192,9.48341855825448,-12.556654811709));
#48003=CARTESIAN_POINT('Ctrl Pts',(-3.71842562677252,9.41894400777795,-12.5513762660949));
#48004=CARTESIAN_POINT('Ctrl Pts',(-3.99291251944306,9.34736366168737,-12.5452387374728));
#48005=CARTESIAN_POINT('Ctrl Pts',(-4.26326703213689,9.26922774175394,-12.5381261540744));
#48006=CARTESIAN_POINT('Ctrl Pts',(-4.32118012884348,9.25249011439838,-12.5366025555737));
#48007=CARTESIAN_POINT('Ctrl Pts',(-4.37890370453842,9.23545151592402,-12.5350342529378));
#48008=CARTESIAN_POINT('Ctrl Pts',(-4.43643562971827,9.21811709981191,-12.5334201657359));
#48009=CARTESIAN_POINT('Ctrl Pts',(-4.71170121329105,9.13517935434142,-12.52569745084));
#48010=CARTESIAN_POINT('Ctrl Pts',(-4.9825779915345,9.04547352247087,-12.5169256906687));
#48011=CARTESIAN_POINT('Ctrl Pts',(-5.24893249317413,8.94957453395467,-12.5069723932165));
#48012=CARTESIAN_POINT('Ctrl Pts',(-5.52135149042552,8.85149206818748,-12.4967924739937));
#48013=CARTESIAN_POINT('Ctrl Pts',(-5.78904005213231,8.74693116129152,-12.4853766661013));
#48014=CARTESIAN_POINT('Ctrl Pts',(-6.05187470201982,8.6364575226633,-12.4725949241842));
#48015=CARTESIAN_POINT('Ctrl Pts',(-6.10592217001445,8.61374050095188,-12.4699665767138));
#48016=CARTESIAN_POINT('Ctrl Pts',(-6.15976445112939,8.5907732983932,-12.4672805075813));
#48017=CARTESIAN_POINT('Ctrl Pts',(-6.21340056281147,8.56756058651678,-12.4645356415522));
#48018=CARTESIAN_POINT('Ctrl Pts',(-6.22559309888096,8.5622838836025,-12.4639116798776));
#48019=CARTESIAN_POINT('Ctrl Pts',(-6.23777498143661,8.55699449386147,-12.4632846799959));
#48020=CARTESIAN_POINT('Ctrl Pts',(-6.24994620285641,8.55169246976548,-12.4626546312706));
#48021=CARTESIAN_POINT('Ctrl Pts',(-6.25018914864656,8.43438870834341,-13.9525601584504));
#48022=CARTESIAN_POINT('Ctrl Pts',(-6.29333242017986,8.41575013829568,-13.9497867189065));
#48023=CARTESIAN_POINT('Ctrl Pts',(-6.42498143684504,8.35057692490983,-13.9456631289492));
#48024=CARTESIAN_POINT('Ctrl Pts',(-6.63295097649907,8.20289362203243,-13.9624206396854));
#48025=CARTESIAN_POINT('Ctrl Pts',(-6.84635576793911,7.97012311971574,-14.0212942505881));
#48026=CARTESIAN_POINT('Ctrl Pts',(-7.00591486456679,7.69498486605711,-14.116453013348));
#48027=CARTESIAN_POINT('Ctrl Pts',(-7.09166336529848,7.41671876496553,-14.2329315229147));
#48028=CARTESIAN_POINT('Ctrl Pts',(-7.10675912386536,7.23705082250496,-14.3187568141423));
#48029=CARTESIAN_POINT('Ctrl Pts',(-7.10558341805161,7.15962818133564,-14.3578004370417));
#48030=CARTESIAN_POINT('Ctrl Pts',(-6.05187975179145,8.02971242238399,-13.49040582652));
#48031=CARTESIAN_POINT('Ctrl Pts',(-6.09005575691405,8.01339292600982,-13.487733176703));
#48032=CARTESIAN_POINT('Ctrl Pts',(-6.20676090005671,7.95627696143004,-13.4832682945061));
#48033=CARTESIAN_POINT('Ctrl Pts',(-6.39210913002687,7.82639664193588,-13.4962238277183));
#48034=CARTESIAN_POINT('Ctrl Pts',(-6.58337525180673,7.6207808979233,-13.545973170834));
#48035=CARTESIAN_POINT('Ctrl Pts',(-6.72695588659178,7.37705576592004,-13.628332337738));
#48036=CARTESIAN_POINT('Ctrl Pts',(-6.80424094438363,7.13044673300983,-13.7304209520421));
#48037=CARTESIAN_POINT('Ctrl Pts',(-6.81779957153361,6.97168361388838,-13.8060530499948));
#48038=CARTESIAN_POINT('Ctrl Pts',(-6.8167458887583,6.90348311857466,-13.8404623489865));
#48039=CARTESIAN_POINT('Ctrl Pts',(-6.03996297048261,8.08823314275827,-12.8475667646262));
#48040=CARTESIAN_POINT('Ctrl Pts',(-6.09254474875977,8.06608626798415,-12.8440967086183));
#48041=CARTESIAN_POINT('Ctrl Pts',(-6.25234888527267,7.98904341043708,-12.8387609712559));
#48042=CARTESIAN_POINT('Ctrl Pts',(-6.50181215036969,7.81693078662947,-12.8579363116836));
#48043=CARTESIAN_POINT('Ctrl Pts',(-6.75454537743524,7.54979157659601,-12.9254977297776));
#48044=CARTESIAN_POINT('Ctrl Pts',(-6.94177187240725,7.23734865246623,-13.0337722950875));
#48045=CARTESIAN_POINT('Ctrl Pts',(-7.04201525985038,6.9229090033521,-13.1655797489763));
#48046=CARTESIAN_POINT('Ctrl Pts',(-7.05980554193481,6.71930667450342,-13.2628609438922));
#48047=CARTESIAN_POINT('Ctrl Pts',(-7.05841299846996,6.63112648395583,-13.3073277280787));
#48048=CARTESIAN_POINT('Ctrl Pts',(-6.22264956594464,8.57067337177415,-12.4592145762074));
#48049=CARTESIAN_POINT('Ctrl Pts',(-6.29926973334839,8.53849259776433,-12.4545882139428));
#48050=CARTESIAN_POINT('Ctrl Pts',(-6.53107452795,8.42701132075841,-12.4484413705606));
#48051=CARTESIAN_POINT('Ctrl Pts',(-6.8880383586651,8.18118390664653,-12.4796540523942));
#48052=CARTESIAN_POINT('Ctrl Pts',(-7.24428436794399,7.80543742918326,-12.579922561284));
#48053=CARTESIAN_POINT('Ctrl Pts',(-7.50527072104853,7.37060329974535,-12.7353078198852));
#48054=CARTESIAN_POINT('Ctrl Pts',(-7.6443714140547,6.93470257276648,-12.9208516737137));
#48055=CARTESIAN_POINT('Ctrl Pts',(-7.66930097473565,6.65083078671604,-13.0569883447064));
#48056=CARTESIAN_POINT('Ctrl Pts',(-7.66733780264737,6.52697650901137,-13.1194049655982));
#48057=CARTESIAN_POINT('',(-7.00000855064648,6.97711954492367,-13.9487143138293));
#48058=CARTESIAN_POINT('',(-7.00000022782178,8.04447854521813,-12.5220639276637));
#48059=CARTESIAN_POINT('Ctrl Pts',(-7.,6.97711954482011,-13.9487143139614));
#48060=CARTESIAN_POINT('Ctrl Pts',(-7.,7.0212653751252,-13.8464534547224));
#48061=CARTESIAN_POINT('Ctrl Pts',(-7.,7.0628914752741,-13.7557906231791));
#48062=CARTESIAN_POINT('Ctrl Pts',(-7.,7.10101355047009,-13.67816421703));
#48063=CARTESIAN_POINT('Ctrl Pts',(-7.,7.12007458806808,-13.6393510139554));
#48064=CARTESIAN_POINT('Ctrl Pts',(-7.,7.13821566025969,-13.6037726540019));
#48065=CARTESIAN_POINT('Ctrl Pts',(-7.,7.15514766559505,-13.5714749226967));
#48066=CARTESIAN_POINT('Ctrl Pts',(-7.,7.16361366826273,-13.5553260570441));
#48067=CARTESIAN_POINT('Ctrl Pts',(-7.,7.17177624969455,-13.5399962417611));
#48068=CARTESIAN_POINT('Ctrl Pts',(-7.,7.17959497271063,-13.5254856024994));
#48069=CARTESIAN_POINT('Ctrl Pts',(-7.,7.18350433421868,-13.5182302828686));
#48070=CARTESIAN_POINT('Ctrl Pts',(-7.,7.18732773112278,-13.5111797572431));
#48071=CARTESIAN_POINT('Ctrl Pts',(-7.,7.19106003063175,-13.5043337119964));
#48072=CARTESIAN_POINT('Ctrl Pts',(-7.,7.19292618038623,-13.5009106893731));
#48073=CARTESIAN_POINT('Ctrl Pts',(-7.,7.19476955579192,-13.4975387868444));
#48074=CARTESIAN_POINT('Ctrl Pts',(-7.,7.19658952368337,-13.4942179595918));
#48075=CARTESIAN_POINT('Ctrl Pts',(-7.,7.19840949157481,-13.4908971323391));
#48076=CARTESIAN_POINT('Ctrl Pts',(-7.,7.19937899854009,-13.4891292310517));
#48077=CARTESIAN_POINT('Ctrl Pts',(-7.,7.20197857287697,-13.4844086544396));
#48078=CARTESIAN_POINT('Ctrl Pts',(-7.,7.24357176226704,-13.4088794286459));
#48079=CARTESIAN_POINT('Ctrl Pts',(-7.,7.28584553318823,-13.3376348089185));
#48080=CARTESIAN_POINT('Ctrl Pts',(-7.,7.328409342137,-13.2711767253503));
#48081=CARTESIAN_POINT('Ctrl Pts',(-7.,7.37097315108578,-13.2047186417821));
#48082=CARTESIAN_POINT('Ctrl Pts',(-7.,7.41284927480191,-13.1443363888025));
#48083=CARTESIAN_POINT('Ctrl Pts',(-7.,7.45600956171151,-13.0863542604578));
#48084=CARTESIAN_POINT('Ctrl Pts',(-7.,7.54233013553071,-12.9703900037684));
#48085=CARTESIAN_POINT('Ctrl Pts',(-7.,7.63589384217129,-12.8624384607559));
#48086=CARTESIAN_POINT('Ctrl Pts',(-7.,7.73524795321228,-12.7671719736965));
#48087=CARTESIAN_POINT('Ctrl Pts',(-7.,7.83460206425328,-12.6719054866371));
#48088=CARTESIAN_POINT('Ctrl Pts',(-7.,7.93956557936649,-12.5894601405347));
#48089=CARTESIAN_POINT('Ctrl Pts',(-7.,8.04447792928004,-12.5220637837759));
#48090=CARTESIAN_POINT('Ctrl Pts',(-6.249946127087,8.5516923215059,-12.4626544152073));
#48091=CARTESIAN_POINT('Ctrl Pts',(-6.343321450661,8.51101931861056,-12.4578186829295));
#48092=CARTESIAN_POINT('Ctrl Pts',(-6.523278504857,8.41889547577619,-12.4561262975012));
#48093=CARTESIAN_POINT('Ctrl Pts',(-6.77486797283079,8.24886074280407,-12.4762415338865));
#48094=CARTESIAN_POINT('Ctrl Pts',(-6.92747242449811,8.11608195573808,-12.5042843754154));
#48095=CARTESIAN_POINT('Ctrl Pts',(-7.00000066044537,8.04447888856054,-12.5220635455847));
#48096=CARTESIAN_POINT('Ctrl Pts',(-6.26385630696103,8.42070038979626,-13.9442695742879));
#48097=CARTESIAN_POINT('Ctrl Pts',(-6.29796810587027,8.39841656325678,-13.9355204336375));
#48098=CARTESIAN_POINT('Ctrl Pts',(-6.33179731289198,8.3741284883213,-13.9274976168449));
#48099=CARTESIAN_POINT('Ctrl Pts',(-6.36511664972141,8.34783587785705,-13.9202482699668));
#48100=CARTESIAN_POINT('Ctrl Pts',(-6.40970979856333,8.31264699346006,-13.9105460599258));
#48101=CARTESIAN_POINT('Ctrl Pts',(-6.45339109876207,8.2738663583666,-13.9022291972004));
#48102=CARTESIAN_POINT('Ctrl Pts',(-6.49565120757311,8.23161769795669,-13.8953353174991));
#48103=CARTESIAN_POINT('Ctrl Pts',(-6.51581268517414,8.21146168216562,-13.892046381311));
#48104=CARTESIAN_POINT('Ctrl Pts',(-6.53565002992448,8.19051657626437,-13.8890814791457));
#48105=CARTESIAN_POINT('Ctrl Pts',(-6.55510400910515,8.16879693701786,-13.8864458658826));
#48106=CARTESIAN_POINT('Ctrl Pts',(-6.56563072135863,8.15704425698905,-13.8850197133112));
#48107=CARTESIAN_POINT('Ctrl Pts',(-6.5760451534477,8.14506479690131,-13.8836899976213));
#48108=CARTESIAN_POINT('Ctrl Pts',(-6.58633757720893,8.13286091933527,-13.8824576824069));
#48109=CARTESIAN_POINT('Ctrl Pts',(-6.620385417617,8.09248989639961,-13.8783811235005));
#48110=CARTESIAN_POINT('Ctrl Pts',(-6.65310005362638,8.04966218117982,-13.8753698816525));
#48111=CARTESIAN_POINT('Ctrl Pts',(-6.68417663523944,8.00453222416122,-13.8734110619505));
#48112=CARTESIAN_POINT('Ctrl Pts',(-6.70441204256171,7.97514601064269,-13.8721355833592));
#48113=CARTESIAN_POINT('Ctrl Pts',(-6.72395244136366,7.94478389648954,-13.8713064535031));
#48114=CARTESIAN_POINT('Ctrl Pts',(-6.74270685114769,7.91349062623327,-13.8709224019828));
#48115=CARTESIAN_POINT('Ctrl Pts',(-6.75208405603971,7.89784399110514,-13.8707303762227));
#48116=CARTESIAN_POINT('Ctrl Pts',(-6.7612647072571,7.8819645336667,-13.870649656644));
#48117=CARTESIAN_POINT('Ctrl Pts',(-6.77023679072211,7.86585803887211,-13.8706803006051));
#48118=CARTESIAN_POINT('Ctrl Pts',(-6.77026987473812,7.86579864714513,-13.8706804136029));
#48119=CARTESIAN_POINT('Ctrl Pts',(-6.77030295591783,7.86573925233098,-13.8706805281151));
#48120=CARTESIAN_POINT('Ctrl Pts',(-6.77033603426063,7.86567985442995,-13.8706806441417));
#48121=CARTESIAN_POINT('Ctrl Pts',(-6.77478822838955,7.8576851677607,-13.8706962607982));
#48122=CARTESIAN_POINT('Ctrl Pts',(-6.77918903097313,7.84963455861528,-13.8707393125092));
#48123=CARTESIAN_POINT('Ctrl Pts',(-6.78353730413754,7.84152899674416,-13.870809592925));
#48124=CARTESIAN_POINT('Ctrl Pts',(-6.7857275938418,7.83744610497488,-13.8708449942132));
#48125=CARTESIAN_POINT('Ctrl Pts',(-6.78790455515289,7.83334927001429,-13.8708873043198));
#48126=CARTESIAN_POINT('Ctrl Pts',(-6.79006804053141,7.82923861688294,-13.8709364975064));
#48127=CARTESIAN_POINT('Ctrl Pts',(-6.7918685580019,7.82581760796298,-13.8709774375529));
#48128=CARTESIAN_POINT('Ctrl Pts',(-6.79402626678841,7.82168086079407,-13.8710331174161));
#48129=CARTESIAN_POINT('Ctrl Pts',(-6.79562563784836,7.81859131291439,-13.8710788063686));
#48130=CARTESIAN_POINT('Ctrl Pts',(-6.79594805647374,7.81796848822701,-13.8710880168449));
#48131=CARTESIAN_POINT('Ctrl Pts',(-6.79624792436415,7.81738830838156,-13.8710967474167));
#48132=CARTESIAN_POINT('Ctrl Pts',(-6.79651792025364,7.81686532799675,-13.8711047010087));
#48133=CARTESIAN_POINT('Ctrl Pts',(-6.81286579182502,7.78519960085733,-13.8715862798252));
#48134=CARTESIAN_POINT('Ctrl Pts',(-6.82902715496191,7.75152418985998,-13.8724615233629));
#48135=CARTESIAN_POINT('Ctrl Pts',(-6.84471562482565,7.71578378911281,-13.8738230072937));
#48136=CARTESIAN_POINT('Ctrl Pts',(-6.85958196904654,7.68191629886587,-13.8751131451428));
#48137=CARTESIAN_POINT('Ctrl Pts',(-6.87402383564703,7.64619448323108,-13.8768398510351));
#48138=CARTESIAN_POINT('Ctrl Pts',(-6.88775763634137,7.60859545149307,-13.8790826824863));
#48139=CARTESIAN_POINT('Ctrl Pts',(-6.89385972568219,7.59188975902672,-13.8800791989056));
#48140=CARTESIAN_POINT('Ctrl Pts',(-6.89982147569496,7.57481381720393,-13.88117762011));
#48141=CARTESIAN_POINT('Ctrl Pts',(-6.90561511753872,7.55736734222936,-13.8823850238945));
#48142=CARTESIAN_POINT('Ctrl Pts',(-6.91636947920041,7.52498258206334,-13.8846262492447));
#48143=CARTESIAN_POINT('Ctrl Pts',(-6.92654558933561,7.49131984950804,-13.887243193891));
#48144=CARTESIAN_POINT('Ctrl Pts',(-6.93597071590286,7.45640380866853,-13.8902697151454));
#48145=CARTESIAN_POINT('Ctrl Pts',(-6.9464108772029,7.41772750063998,-13.8936221762342));
#48146=CARTESIAN_POINT('Ctrl Pts',(-6.95593049190132,7.37751271587397,-13.8974771800602));
#48147=CARTESIAN_POINT('Ctrl Pts',(-6.96426462120672,7.33582224075069,-13.9018779416159));
#48148=CARTESIAN_POINT('Ctrl Pts',(-6.97143755969684,7.29994048241401,-13.9056655468704));
#48149=CARTESIAN_POINT('Ctrl Pts',(-6.97773208677669,7.26296598840208,-13.9098573515925));
#48150=CARTESIAN_POINT('Ctrl Pts',(-6.98295592997464,7.22495918651961,-13.9144796278969));
#48151=CARTESIAN_POINT('Ctrl Pts',(-6.98861460540534,7.1837887019047,-13.9194866620605));
#48152=CARTESIAN_POINT('Ctrl Pts',(-6.99301684031462,7.14140573016511,-13.924999197015));
#48153=CARTESIAN_POINT('Ctrl Pts',(-6.99593359400257,7.09794539883662,-13.9310276109909));
#48154=CARTESIAN_POINT('Ctrl Pts',(-6.99857998209795,7.05851357985103,-13.9364972271074));
#48155=CARTESIAN_POINT('Ctrl Pts',(-7.00000359100067,7.01819516235357,-13.9423914043819));
#48156=CARTESIAN_POINT('Ctrl Pts',(-7.00000966473096,6.97711954509652,-13.948714313882));
#48157=CARTESIAN_POINT('Ctrl Pts',(-6.2341298497682,11.870031945894,-24.393391026367));
#48158=CARTESIAN_POINT('Ctrl Pts',(-6.23490515007836,11.9504778000158,-23.8924703860421));
#48159=CARTESIAN_POINT('Ctrl Pts',(-6.23649294537174,12.0627648225871,-22.7260279240694));
#48160=CARTESIAN_POINT('Ctrl Pts',(-6.23803980036877,11.9701373820371,-20.8893409247744));
#48161=CARTESIAN_POINT('Ctrl Pts',(-6.23759260730665,11.5416382094031,-18.9411611420578));
#48162=CARTESIAN_POINT('Ctrl Pts',(-6.23570343585033,10.7961451762139,-17.0892587092505));
#48163=CARTESIAN_POINT('Ctrl Pts',(-6.23204961282645,9.75631588910903,-15.3875854443724));
#48164=CARTESIAN_POINT('Ctrl Pts',(-6.22726106267534,8.6169945866861,-14.0755190620509));
#48165=CARTESIAN_POINT('Ctrl Pts',(-6.22400151927379,7.81350031894818,-13.3673833063685));
#48166=CARTESIAN_POINT('Ctrl Pts',(-6.2226659932316,7.49367920211764,-13.1134096388249));
#48167=CARTESIAN_POINT('Ctrl Pts',(-6.72598992820685,11.7530860140233,-24.3745661708325));
#48168=CARTESIAN_POINT('Ctrl Pts',(-6.72668308530094,11.8323454549326,-23.8785347072491));
#48169=CARTESIAN_POINT('Ctrl Pts',(-6.72805134751943,11.9427141750406,-22.7235345581661));
#48170=CARTESIAN_POINT('Ctrl Pts',(-6.729418896676,11.8502318240213,-20.9054832492773));
#48171=CARTESIAN_POINT('Ctrl Pts',(-6.72902389879382,11.4262602892439,-18.9767992205318));
#48172=CARTESIAN_POINT('Ctrl Pts',(-6.7273678414525,10.6891576732562,-17.1431693745882));
#48173=CARTESIAN_POINT('Ctrl Pts',(-6.72416416502884,9.66125588094435,-15.4573959672442));
#48174=CARTESIAN_POINT('Ctrl Pts',(-6.71993329975334,8.53485935179034,-14.1564667453737));
#48175=CARTESIAN_POINT('Ctrl Pts',(-6.71707878522504,7.74006810589514,-13.4537901142132));
#48176=CARTESIAN_POINT('Ctrl Pts',(-6.7158900664978,7.42368987088072,-13.2016824589374));
#48177=CARTESIAN_POINT('Ctrl Pts',(-7.02718522726892,11.3520762594696,-24.3100157521472));
#48178=CARTESIAN_POINT('Ctrl Pts',(-7.02756392150913,11.4283599553699,-23.8309254769524));
#48179=CARTESIAN_POINT('Ctrl Pts',(-7.0282488325563,11.5344320553921,-22.7152040882476));
#48180=CARTESIAN_POINT('Ctrl Pts',(-7.02897715467319,11.4446324857795,-20.9601377668576));
#48181=CARTESIAN_POINT('Ctrl Pts',(-7.02876723083941,11.0353400441858,-19.0974452680292));
#48182=CARTESIAN_POINT('Ctrl Pts',(-7.0279026933489,10.3242146467833,-17.3268263925021));
#48183=CARTESIAN_POINT('Ctrl Pts',(-7.02622933623767,9.33267263994042,-15.6982356130382));
#48184=CARTESIAN_POINT('Ctrl Pts',(-7.02397930980613,8.24599547250213,-14.4407047902092));
#48185=CARTESIAN_POINT('Ctrl Pts',(-7.02249263040784,7.47887540073063,-13.7610260286471));
#48186=CARTESIAN_POINT('Ctrl Pts',(-7.02184967286603,7.17356126230332,-13.5171517118445));
#48187=CARTESIAN_POINT('Ctrl Pts',(-6.9983806254281,10.8539091305164,-24.2298260443849));
#48188=CARTESIAN_POINT('Ctrl Pts',(-6.99835912984722,10.9268138861166,-23.7718327253704));
#48189=CARTESIAN_POINT('Ctrl Pts',(-6.99821532188652,11.0282119309624,-22.7049190930737));
#48190=CARTESIAN_POINT('Ctrl Pts',(-6.99814245125572,10.9423807638968,-21.027831107362));
#48191=CARTESIAN_POINT('Ctrl Pts',(-6.99816421464904,10.5510777398404,-19.2468686040926));
#48192=CARTESIAN_POINT('Ctrl Pts',(-6.99828068956064,9.871410767818,-17.5546300609639));
#48193=CARTESIAN_POINT('Ctrl Pts',(-6.9985045686866,8.92371735875945,-15.9978504404111));
#48194=CARTESIAN_POINT('Ctrl Pts',(-6.99873523493892,7.88504484531634,-14.7957477722731));
#48195=CARTESIAN_POINT('Ctrl Pts',(-6.99894167920566,7.1516684994886,-14.1458833200365));
#48196=CARTESIAN_POINT('Ctrl Pts',(-6.99898903107869,6.85988337428983,-13.9127708060056));
#48197=CARTESIAN_POINT('',(-7.0000030891987,10.927769589406,-24.1259430621516));
#48198=CARTESIAN_POINT('Origin',(-5.99998370357436,10.9277595201359,-24.1259473086588));
#48199=CARTESIAN_POINT('Ctrl Pts',(-7.00001101651665,10.9277661762093,-24.1259401091756));
#48200=CARTESIAN_POINT('Ctrl Pts',(-7.0000178689439,10.9560764183263,-23.9375950050149));
#48201=CARTESIAN_POINT('Ctrl Pts',(-7.00001802523654,10.9791078956897,-23.7511663574579));
#48202=CARTESIAN_POINT('Ctrl Pts',(-7.00001556833325,10.997240350625,-23.566999236078));
#48203=CARTESIAN_POINT('Ctrl Pts',(-7.00001306404682,11.0157225030191,-23.37928031906));
#48204=CARTESIAN_POINT('Ctrl Pts',(-7.00000784335913,11.0291149028731,-23.1939109094671));
#48205=CARTESIAN_POINT('Ctrl Pts',(-7.00000354817103,11.0378133555915,-23.0112026941266));
#48206=CARTESIAN_POINT('Ctrl Pts',(-7.00000225617205,11.0404298631314,-22.9562437906837));
#48207=CARTESIAN_POINT('Ctrl Pts',(-7.00000104339744,11.0426216093023,-22.9015253189936));
#48208=CARTESIAN_POINT('Ctrl Pts',(-6.99999999753975,11.044399246237,-22.8470548569864));
#48209=CARTESIAN_POINT('Ctrl Pts',(-6.99999887667119,11.0463043786159,-22.7886776716144));
#48210=CARTESIAN_POINT('Ctrl Pts',(-6.99999794691843,11.0477338782397,-22.7305853426262));
#48211=CARTESIAN_POINT('Ctrl Pts',(-6.99999718088468,11.0487021581796,-22.6727848889157));
#48212=CARTESIAN_POINT('Ctrl Pts',(-6.99999462213086,11.0519364673514,-22.4797162009707));
#48213=CARTESIAN_POINT('Ctrl Pts',(-6.99999387749935,11.0500263119686,-22.2899077654462));
#48214=CARTESIAN_POINT('Ctrl Pts',(-6.99999403436533,11.0434957469855,-22.1035888577242));
#48215=CARTESIAN_POINT('Ctrl Pts',(-6.99999406718763,11.0421293056716,-22.064603891838));
#48216=CARTESIAN_POINT('Ctrl Pts',(-6.99999414005194,11.0405605105098,-22.0257715309591));
#48217=CARTESIAN_POINT('Ctrl Pts',(-6.99999424550212,11.0387940509543,-21.9870936125725));
#48218=CARTESIAN_POINT('Ctrl Pts',(-6.99999432423836,11.0374750927492,-21.9582140621436));
#48219=CARTESIAN_POINT('Ctrl Pts',(-6.99999441864869,11.0360814529893,-21.9301065592141));
#48220=CARTESIAN_POINT('Ctrl Pts',(-6.99999453140857,11.0345337169244,-21.9011843449435));
#48221=CARTESIAN_POINT('Ctrl Pts',(-6.99999463684067,11.0330865616108,-21.8741416617535));
#48222=CARTESIAN_POINT('Ctrl Pts',(-6.99999475849192,11.0315045688866,-21.846386673071));
#48223=CARTESIAN_POINT('Ctrl Pts',(-6.9999949035284,11.029681939679,-21.8166247929757));
#48224=CARTESIAN_POINT('Ctrl Pts',(-6.99999520368176,11.0259100041799,-21.755032511024));
#48225=CARTESIAN_POINT('Ctrl Pts',(-6.9999955626785,11.0216269151297,-21.6935868226501));
#48226=CARTESIAN_POINT('Ctrl Pts',(-6.9999959537239,11.0168388651946,-21.6322954802246));
#48227=CARTESIAN_POINT('Ctrl Pts',(-6.99999673581471,11.0072627653243,-21.5097127953737));
#48228=CARTESIAN_POINT('Ctrl Pts',(-6.99999764539611,10.9956668219142,-21.387747494317));
#48229=CARTESIAN_POINT('Ctrl Pts',(-6.99999847634374,10.9821001708853,-21.2664589704134));
#48230=CARTESIAN_POINT('Ctrl Pts',(-6.99999902467265,10.9731477573094,-21.1864226353089));
#48231=CARTESIAN_POINT('Ctrl Pts',(-6.99999953898542,10.9633371968182,-21.1066809430449));
#48232=CARTESIAN_POINT('Ctrl Pts',(-6.99999996276672,10.9526825043711,-21.0272502934151));
#48233=CARTESIAN_POINT('Ctrl Pts',(-7.00000126736559,10.9198823315757,-20.7827252593973));
#48234=CARTESIAN_POINT('Ctrl Pts',(-7.00000171384871,10.8790835251978,-20.5411517571741));
#48235=CARTESIAN_POINT('Ctrl Pts',(-7.00000170643162,10.8307721803972,-20.3030233611526));
#48236=CARTESIAN_POINT('Ctrl Pts',(-7.00000169893522,10.7819442740525,-20.0623488142742));
#48237=CARTESIAN_POINT('Ctrl Pts',(-7.00000122941415,10.7254423237568,-19.8251933968343));
#48238=CARTESIAN_POINT('Ctrl Pts',(-7.0000007234276,10.6617526620477,-19.5920156367625));
#48239=CARTESIAN_POINT('Ctrl Pts',(-7.00000046988901,10.6298391901355,-19.4751754511354));
#48240=CARTESIAN_POINT('Ctrl Pts',(-7.00000020716685,10.5961207929503,-19.3593331797781));
#48241=CARTESIAN_POINT('Ctrl Pts',(-6.99999998766517,10.5606572076705,-19.2445418256472));
#48242=CARTESIAN_POINT('Ctrl Pts',(-6.99999993928869,10.5528413054783,-19.219242691639));
#48243=CARTESIAN_POINT('Ctrl Pts',(-6.9999998930055,10.5449406310664,-19.1939945917012));
#48244=CARTESIAN_POINT('Ctrl Pts',(-6.99999984878303,10.5369559371202,-19.1687979951081));
#48245=CARTESIAN_POINT('Ctrl Pts',(-6.99999965374478,10.5017403435686,-19.0576712430394));
#48246=CARTESIAN_POINT('Ctrl Pts',(-6.99999949863674,10.4648905474801,-18.9475464970961));
#48247=CARTESIAN_POINT('Ctrl Pts',(-6.99999938184587,10.4264702932223,-18.8384625308438));
#48248=CARTESIAN_POINT('Ctrl Pts',(-6.99999932345044,10.4072601660933,-18.7839205477176));
#48249=CARTESIAN_POINT('Ctrl Pts',(-6.99999927466561,10.3876574244221,-18.7296387595141));
#48250=CARTESIAN_POINT('Ctrl Pts',(-6.99999923547375,10.3676698878029,-18.6756217474293));
#48251=CARTESIAN_POINT('Ctrl Pts',(-6.99999921587781,10.3576761194934,-18.6486132413869));
#48252=CARTESIAN_POINT('Ctrl Pts',(-6.99999919868214,10.3475861524468,-18.6216709293742));
#48253=CARTESIAN_POINT('Ctrl Pts',(-6.9999991838965,10.3374009596986,-18.5947953762306));
#48254=CARTESIAN_POINT('Ctrl Pts',(-6.99999917283138,10.3297786753504,-18.5746825405544));
#48255=CARTESIAN_POINT('Ctrl Pts',(-6.99999916268833,10.3217399609405,-18.5536617176207));
#48256=CARTESIAN_POINT('Ctrl Pts',(-6.99999915445986,10.31409937907,-18.5338560146091));
#48257=CARTESIAN_POINT('Ctrl Pts',(-6.99999915169312,10.3115303183315,-18.5271965670869));
#48258=CARTESIAN_POINT('Ctrl Pts',(-6.99999914913282,10.3090066899196,-18.5206743351133));
#48259=CARTESIAN_POINT('Ctrl Pts',(-6.99999914678744,10.3065606748726,-18.5143695537774));
#48260=CARTESIAN_POINT('Ctrl Pts',(-6.99999907529418,10.2319997646018,-18.3221833952997));
#48261=CARTESIAN_POINT('Ctrl Pts',(-6.99999912491849,10.1510712733243,-18.1296184689333));
#48262=CARTESIAN_POINT('Ctrl Pts',(-6.99999933315943,10.0634928197255,-17.9371558145606));
#48263=CARTESIAN_POINT('Ctrl Pts',(-6.99999947285716,10.0047411118898,-17.8080428972351));
#48264=CARTESIAN_POINT('Ctrl Pts',(-6.99999968443218,9.94299688374547,-17.678977014169));
#48265=CARTESIAN_POINT('Ctrl Pts',(-6.99999998816759,9.87817756885076,-17.5501163140756));
#48266=CARTESIAN_POINT('Ctrl Pts',(-7.00000042903653,9.78409297605115,-17.3630762857159));
#48267=CARTESIAN_POINT('Ctrl Pts',(-7.0000010678068,9.68352878376437,-17.1764663552485));
#48268=CARTESIAN_POINT('Ctrl Pts',(-7.00000153331188,9.57627842588298,-16.9908082299143));
#48269=CARTESIAN_POINT('Ctrl Pts',(-7.00000199134791,9.47074890515542,-16.8081289981363));
#48270=CARTESIAN_POINT('Ctrl Pts',(-7.00000228132013,9.35874600671699,-16.6263712423838));
#48271=CARTESIAN_POINT('Ctrl Pts',(-7.00000202662856,9.24008894373901,-16.4460793865259));
#48272=CARTESIAN_POINT('Ctrl Pts',(-7.000001812094,9.14014044338894,-16.2942140009678));
#48273=CARTESIAN_POINT('Ctrl Pts',(-7.0000012106318,9.03547091581878,-16.1433894613444));
#48274=CARTESIAN_POINT('Ctrl Pts',(-6.99999998662418,8.92598177928851,-15.9939582849167));
#48275=CARTESIAN_POINT('Ctrl Pts',(-6.99999852881463,8.7955787440933,-15.8159837426334));
#48276=CARTESIAN_POINT('Ctrl Pts',(-6.99999617286889,8.65833776962605,-15.639985120766));
#48277=CARTESIAN_POINT('Ctrl Pts',(-6.99999449845809,8.51417826060077,-15.4665284038773));
#48278=CARTESIAN_POINT('Ctrl Pts',(-6.99999284826976,8.37210420131663,-15.295580957919));
#48279=CARTESIAN_POINT('Ctrl Pts',(-6.99999186158911,8.22331027668761,-15.1271023856721));
#48280=CARTESIAN_POINT('Ctrl Pts',(-6.99999320067939,8.06774699367314,-14.9616765568042));
#48281=CARTESIAN_POINT('Ctrl Pts',(-6.99999413395892,7.95932709874448,-14.8463829564328));
#48282=CARTESIAN_POINT('Ctrl Pts',(-6.99999620011753,7.84761962633808,-14.7325730635345));
#48283=CARTESIAN_POINT('Ctrl Pts',(-6.99999999965478,7.73261617693726,-14.6204570168772));
#48284=CARTESIAN_POINT('Ctrl Pts',(-7.00000506883503,7.57918348853654,-14.4708765778458));
#48285=CARTESIAN_POINT('Ctrl Pts',(-7.0000132984882,7.41988233836246,-14.3243094370825));
#48286=CARTESIAN_POINT('Ctrl Pts',(-7.00001657716769,7.25479675802074,-14.1813267045858));
#48287=CARTESIAN_POINT('Ctrl Pts',(-7.00001838080306,7.16398147886925,-14.1026704298303));
#48288=CARTESIAN_POINT('Ctrl Pts',(-7.00001867122436,7.07141628639037,-14.0250995594017));
#48289=CARTESIAN_POINT('Ctrl Pts',(-7.00001598720849,6.97711954487508,-13.9487143136413));
#48290=CARTESIAN_POINT('Origin',(-5.999994980806,10.9277770011849,-24.1259380084193));
#48291=CARTESIAN_POINT('Origin',(-6.,10.9277790621896,-24.1259427055443));
#48292=CARTESIAN_POINT('Ctrl Pts',(-7.10365375325716,5.08556213759161,-15.2124200606729));
#48293=CARTESIAN_POINT('Ctrl Pts',(-7.10425940579783,5.03547652135492,-15.2289541394246));
#48294=CARTESIAN_POINT('Ctrl Pts',(-7.09698248863266,4.87479892200809,-15.2843333495191));
#48295=CARTESIAN_POINT('Ctrl Pts',(-7.03475514727946,4.61092148639726,-15.3877970248073));
#48296=CARTESIAN_POINT('Ctrl Pts',(-6.88260033893558,4.32655598757909,-15.5206346518419));
#48297=CARTESIAN_POINT('Ctrl Pts',(-6.66949670496425,4.10048277670444,-15.649982801355));
#48298=CARTESIAN_POINT('Ctrl Pts',(-6.45007050561619,3.96694228146696,-15.7511248346751));
#48299=CARTESIAN_POINT('Ctrl Pts',(-6.30610234990484,3.91682262999853,-15.8056261738581));
#48300=CARTESIAN_POINT('Ctrl Pts',(-6.25371803308994,3.90293324094133,-15.8240946813389));
#48301=CARTESIAN_POINT('Ctrl Pts',(-6.81817564339306,4.90140851365106,-14.6657612012878));
#48302=CARTESIAN_POINT('Ctrl Pts',(-6.8187209234073,4.8571674745428,-14.6803578801389));
#48303=CARTESIAN_POINT('Ctrl Pts',(-6.81217849063633,4.71506404703517,-14.7294286095061));
#48304=CARTESIAN_POINT('Ctrl Pts',(-6.75596877441542,4.48132758213125,-14.8218932719452));
#48305=CARTESIAN_POINT('Ctrl Pts',(-6.61862718319516,4.23005438056527,-14.9412123965516));
#48306=CARTESIAN_POINT('Ctrl Pts',(-6.42697177765079,4.03134800350222,-15.057457108221));
#48307=CARTESIAN_POINT('Ctrl Pts',(-6.23069936786126,3.91487721740648,-15.1480748819103));
#48308=CARTESIAN_POINT('Ctrl Pts',(-6.1026337152333,3.87149278153041,-15.1966642579316));
#48309=CARTESIAN_POINT('Ctrl Pts',(-6.05613610180907,3.85950522648497,-15.2130939828674));
#48310=CARTESIAN_POINT('Ctrl Pts',(-7.06073274467296,4.7170686558441,-14.098996840888));
#48311=CARTESIAN_POINT('Ctrl Pts',(-7.06144827708986,4.65990256849783,-14.1178698225721));
#48312=CARTESIAN_POINT('Ctrl Pts',(-7.05282245267813,4.47706838045324,-14.1808763385047));
#48313=CARTESIAN_POINT('Ctrl Pts',(-6.97988948335629,4.17817855160872,-14.2979140353396));
#48314=CARTESIAN_POINT('Ctrl Pts',(-6.80124511423192,3.85488795162216,-14.4486451526198));
#48315=CARTESIAN_POINT('Ctrl Pts',(-6.54883128807966,3.59536050662941,-14.5970203599067));
#48316=CARTESIAN_POINT('Ctrl Pts',(-6.28555951712999,3.43993495535892,-14.71508158883));
#48317=CARTESIAN_POINT('Ctrl Pts',(-6.11058332363383,3.38094754188304,-14.7799070207993));
#48318=CARTESIAN_POINT('Ctrl Pts',(-6.04660001229308,3.36455643057283,-14.8020435974322));
#48319=CARTESIAN_POINT('Ctrl Pts',(-7.66739167259926,4.65664426237229,-13.8937090025063));
#48320=CARTESIAN_POINT('Ctrl Pts',(-7.66839318582775,4.57650762421567,-13.9201855750848));
#48321=CARTESIAN_POINT('Ctrl Pts',(-7.65627208602678,4.32113029813062,-14.0079657876853));
#48322=CARTESIAN_POINT('Ctrl Pts',(-7.55516094421515,3.90577067771103,-14.1685624456636));
#48323=CARTESIAN_POINT('Ctrl Pts',(-7.30697159306207,3.45396377815488,-14.3744344773038));
#48324=CARTESIAN_POINT('Ctrl Pts',(-6.95259600190474,3.08648007996775,-14.5784884618108));
#48325=CARTESIAN_POINT('Ctrl Pts',(-6.57738617026409,2.86236823778828,-14.7434394142203));
#48326=CARTESIAN_POINT('Ctrl Pts',(-6.32434354928332,2.77597093213413,-14.8356916710563));
#48327=CARTESIAN_POINT('Ctrl Pts',(-6.23130215550449,2.7518430695664,-14.8674293899488));
#48328=CARTESIAN_POINT('',(-6.26386059950783,3.90573753004527,-15.8144217560873));
#48329=CARTESIAN_POINT('',(-6.24994547032252,2.76546740288181,-14.8593848470608));
#48330=CARTESIAN_POINT('Ctrl Pts',(-6.26385524237826,3.90575711203162,-15.8144219713711));
#48331=CARTESIAN_POINT('Ctrl Pts',(-6.25431842670559,3.90347140179835,-15.7850251932568));
#48332=CARTESIAN_POINT('Ctrl Pts',(-6.24496510276104,3.89974753513886,-15.7549999297834));
#48333=CARTESIAN_POINT('Ctrl Pts',(-6.23589623365663,3.89443541490935,-15.7245193832421));
#48334=CARTESIAN_POINT('Ctrl Pts',(-6.22705377181037,3.88925591348405,-15.6947997934297));
#48335=CARTESIAN_POINT('Ctrl Pts',(-6.21848203426885,3.88256579299046,-15.6646476750876));
#48336=CARTESIAN_POINT('Ctrl Pts',(-6.21028075854689,3.87425393748282,-15.6342636592137));
#48337=CARTESIAN_POINT('Ctrl Pts',(-6.2022059505754,3.86607025492093,-15.6043481799758));
#48338=CARTESIAN_POINT('Ctrl Pts',(-6.19449059505007,3.85631385047443,-15.5742083486252));
#48339=CARTESIAN_POINT('Ctrl Pts',(-6.18723134420193,3.8449157925931,-15.5440695413971));
#48340=CARTESIAN_POINT('Ctrl Pts',(-6.18009971140207,3.83371811322622,-15.5144605761369));
#48341=CARTESIAN_POINT('Ctrl Pts',(-6.17340862814906,3.82093556240753,-15.4848532328916));
#48342=CARTESIAN_POINT('Ctrl Pts',(-6.16724621350028,3.80654661238053,-15.4554861432826));
#48343=CARTESIAN_POINT('Ctrl Pts',(-6.16645007886344,3.8046876752338,-15.4516921504156));
#48344=CARTESIAN_POINT('Ctrl Pts',(-6.16566275894613,3.80280199211259,-15.447902194074));
#48345=CARTESIAN_POINT('Ctrl Pts',(-6.16488443472348,3.80088957628181,-15.4441168105991));
#48346=CARTESIAN_POINT('Ctrl Pts',(-6.15895241115861,3.78631403636689,-15.4152663864167));
#48347=CARTESIAN_POINT('Ctrl Pts',(-6.15354382259298,3.77018160286767,-15.3866810289208));
#48348=CARTESIAN_POINT('Ctrl Pts',(-6.14873326440852,3.752526237599,-15.3586037373115));
#48349=CARTESIAN_POINT('Ctrl Pts',(-6.14398433495375,3.73509705766934,-15.3308861477885));
#48350=CARTESIAN_POINT('Ctrl Pts',(-6.13981848386434,3.71618373826285,-15.3036644956293));
#48351=CARTESIAN_POINT('Ctrl Pts',(-6.13629421425756,3.69586792599309,-15.277173486802));
#48352=CARTESIAN_POINT('Ctrl Pts',(-6.13279064028137,3.67567141462606,-15.250838041593));
#48353=CARTESIAN_POINT('Ctrl Pts',(-6.12992135457027,3.65408904541089,-15.2252254892552));
#48354=CARTESIAN_POINT('Ctrl Pts',(-6.12772694082186,3.63124809294815,-15.2005553078385));
#48355=CARTESIAN_POINT('Ctrl Pts',(-6.12553997337744,3.60848464668758,-15.1759688397464));
#48356=CARTESIAN_POINT('Ctrl Pts',(-6.12402344438827,3.58447157299373,-15.152319103387));
#48357=CARTESIAN_POINT('Ctrl Pts',(-6.12319799097326,3.5593769534127,-15.1298006183463));
#48358=CARTESIAN_POINT('Ctrl Pts',(-6.12237328082849,3.5343049299996,-15.1073024098221));
#48359=CARTESIAN_POINT('Ctrl Pts',(-6.12223844696652,3.50815392308848,-15.0859340393127));
#48360=CARTESIAN_POINT('Ctrl Pts',(-6.12279314210064,3.48112581360472,-15.0658564449281));
#48361=CARTESIAN_POINT('Ctrl Pts',(-6.12335053997515,3.45396601022447,-15.045681022886));
#48362=CARTESIAN_POINT('Ctrl Pts',(-6.12460415940122,3.42592128542679,-15.0268094621603));
#48363=CARTESIAN_POINT('Ctrl Pts',(-6.12653245965907,3.39722080139595,-15.009363286171));
#48364=CARTESIAN_POINT('Ctrl Pts',(-6.12846822014428,3.36840928064495,-14.9918496142414));
#48365=CARTESIAN_POINT('Ctrl Pts',(-6.13108374049619,3.3389377607077,-14.9757726162461));
#48366=CARTESIAN_POINT('Ctrl Pts',(-6.13433741011253,3.30905041842281,-14.9612078107311));
#48367=CARTESIAN_POINT('Ctrl Pts',(-6.13762846464348,3.27881966827212,-14.9464756544786));
#48368=CARTESIAN_POINT('Ctrl Pts',(-6.14157219435981,3.24816435165046,-14.9332906905176));
#48369=CARTESIAN_POINT('Ctrl Pts',(-6.14610811724841,3.21733673198634,-14.9216803414444));
#48370=CARTESIAN_POINT('Ctrl Pts',(-6.14941180669293,3.19488377496189,-14.9132240716572));
#48371=CARTESIAN_POINT('Ctrl Pts',(-6.15302925331993,3.17233943514232,-14.9056019936076));
#48372=CARTESIAN_POINT('Ctrl Pts',(-6.15693255119853,3.14979720314684,-14.8988083887852));
#48373=CARTESIAN_POINT('Ctrl Pts',(-6.16238723402997,3.11829545009785,-14.8893146322898));
#48374=CARTESIAN_POINT('Ctrl Pts',(-6.16840043529369,3.08679919654159,-14.8814403581585));
#48375=CARTESIAN_POINT('Ctrl Pts',(-6.17488786719185,3.05554401213897,-14.8751293194312));
#48376=CARTESIAN_POINT('Ctrl Pts',(-6.1815237056771,3.0235738336803,-14.8686739092895));
#48377=CARTESIAN_POINT('Ctrl Pts',(-6.18865536712829,2.99185651849639,-14.8638535662064));
#48378=CARTESIAN_POINT('Ctrl Pts',(-6.19618723020727,2.9606107284726,-14.8605653101527));
#48379=CARTESIAN_POINT('Ctrl Pts',(-6.20383065418149,2.92890213020723,-14.8572283489135));
#48380=CARTESIAN_POINT('Ctrl Pts',(-6.21188586975053,2.89767951081031,-14.8554684804184));
#48381=CARTESIAN_POINT('Ctrl Pts',(-6.2202528897936,2.86712951671446,-14.8551440416511));
#48382=CARTESIAN_POINT('Ctrl Pts',(-6.22882057895255,2.83584683161588,-14.8548118217573));
#48383=CARTESIAN_POINT('Ctrl Pts',(-6.23771488179524,2.80526963802762,-14.8559839371986));
#48384=CARTESIAN_POINT('Ctrl Pts',(-6.24683365328605,2.77555001402948,-14.85848431103));
#48385=CARTESIAN_POINT('Ctrl Pts',(-6.24786821957997,2.77217818688287,-14.8587679898667));
#48386=CARTESIAN_POINT('Ctrl Pts',(-6.24890568355812,2.76881734680998,-14.8590687484887));
#48387=CARTESIAN_POINT('Ctrl Pts',(-6.24994590287157,2.76546767660005,-14.8593863177582));
#48388=CARTESIAN_POINT('',(-7.00000030631414,3.1661281488063,-14.5427419373966));
#48389=CARTESIAN_POINT('Ctrl Pts',(-7.00000091797045,3.16612715294925,-14.5427414491965));
#48390=CARTESIAN_POINT('Ctrl Pts',(-6.9770948764676,3.14616537143328,-14.5547620427858));
#48391=CARTESIAN_POINT('Ctrl Pts',(-6.9538163142397,3.12684702049389,-14.5666755023522));
#48392=CARTESIAN_POINT('Ctrl Pts',(-6.93017491231045,3.10816085848109,-14.5784854676487));
#48393=CARTESIAN_POINT('Ctrl Pts',(-6.88947876003189,3.07599462328698,-14.5988150634802));
#48394=CARTESIAN_POINT('Ctrl Pts',(-6.84770978866817,3.04569988961234,-14.6188379878143));
#48395=CARTESIAN_POINT('Ctrl Pts',(-6.80491841661944,3.01722957302793,-14.6385688721317));
#48396=CARTESIAN_POINT('Ctrl Pts',(-6.76163570292131,2.98843235287302,-14.6585263115882));
#48397=CARTESIAN_POINT('Ctrl Pts',(-6.71730648856817,2.96150123974364,-14.6781851761215));
#48398=CARTESIAN_POINT('Ctrl Pts',(-6.67194315514633,2.93642225616261,-14.6975594142133));
#48399=CARTESIAN_POINT('Ctrl Pts',(-6.66414019379478,2.93210841225261,-14.7008919830446));
#48400=CARTESIAN_POINT('Ctrl Pts',(-6.65630655130121,2.92784946010201,-14.7042161232254));
#48401=CARTESIAN_POINT('Ctrl Pts',(-6.64844218978448,2.92364544595408,-14.7075318951735));
#48402=CARTESIAN_POINT('Ctrl Pts',(-6.60349501531205,2.89961824972342,-14.7264825219913));
#48403=CARTESIAN_POINT('Ctrl Pts',(-6.55756813993438,2.87738307797186,-14.7451532943523));
#48404=CARTESIAN_POINT('Ctrl Pts',(-6.51063098898213,2.85696654565969,-14.7635563543032));
#48405=CARTESIAN_POINT('Ctrl Pts',(-6.50668245189925,2.85524902695004,-14.7651044918271));
#48406=CARTESIAN_POINT('Ctrl Pts',(-6.50272675016091,2.85354440476764,-14.7666507309458));
#48407=CARTESIAN_POINT('Ctrl Pts',(-6.4987638575357,2.85185270971999,-14.7681950766425));
#48408=CARTESIAN_POINT('Ctrl Pts',(-6.45236637950589,2.83204637348299,-14.7862762492376));
#48409=CARTESIAN_POINT('Ctrl Pts',(-6.40498461823921,2.81400816695435,-14.8040986136675));
#48410=CARTESIAN_POINT('Ctrl Pts',(-6.35660284408077,2.79778989501982,-14.8216604597072));
#48411=CARTESIAN_POINT('Ctrl Pts',(-6.32157843143683,2.78604920426411,-14.8343737872605));
#48412=CARTESIAN_POINT('Ctrl Pts',(-6.2860294977681,2.77526317253696,-14.8469504427215));
#48413=CARTESIAN_POINT('Ctrl Pts',(-6.24994590287805,2.76546767660181,-14.8593863177559));
#48414=CARTESIAN_POINT('',(-7.000003179836,4.92966193726001,-14.7967990013279));
#48415=CARTESIAN_POINT('Ctrl Pts',(-7.,4.92966193726001,-14.7967990013279));
#48416=CARTESIAN_POINT('Ctrl Pts',(-7.,4.77605682881269,-14.7360009948777));
#48417=CARTESIAN_POINT('Ctrl Pts',(-7.,4.63248720373973,-14.6852063747094));
#48418=CARTESIAN_POINT('Ctrl Pts',(-7.,4.49895306204113,-14.6444151408229));
#48419=CARTESIAN_POINT('Ctrl Pts',(-7.,4.47987675608419,-14.6385878216963));
#48420=CARTESIAN_POINT('Ctrl Pts',(-7.,4.46218562630564,-14.6333073196583));
#48421=CARTESIAN_POINT('Ctrl Pts',(-7.,4.44233856151975,-14.6275456356643));
#48422=CARTESIAN_POINT('Ctrl Pts',(-7.,4.28356204323264,-14.5814521637125));
#48423=CARTESIAN_POINT('Ctrl Pts',(-7.,4.12817410523823,-14.5472790797429));
#48424=CARTESIAN_POINT('Ctrl Pts',(-7.,3.98124764966623,-14.5257690562941));
#48425=CARTESIAN_POINT('Ctrl Pts',(-7.,3.68739473852224,-14.4827490093966));
#48426=CARTESIAN_POINT('Ctrl Pts',(-7.,3.41568850431818,-14.4884065002489));
#48427=CARTESIAN_POINT('Ctrl Pts',(-7.,3.16612894705406,-14.5427415288511));
#48428=CARTESIAN_POINT('Ctrl Pts',(-6.99999286694104,4.92966193658926,-14.7967990014538));
#48429=CARTESIAN_POINT('Ctrl Pts',(-6.99999564996434,4.89205532347658,-14.8244082330937));
#48430=CARTESIAN_POINT('Ctrl Pts',(-6.99822284827502,4.85539428974177,-14.8517940861305));
#48431=CARTESIAN_POINT('Ctrl Pts',(-6.99489375804626,4.81982245813974,-14.878828057977));
#48432=CARTESIAN_POINT('Ctrl Pts',(-6.99462619840172,4.81696354295125,-14.881000783677));
#48433=CARTESIAN_POINT('Ctrl Pts',(-6.9943485697214,4.81411164574981,-14.8831712499741));
#48434=CARTESIAN_POINT('Ctrl Pts',(-6.99406097763697,4.81126683193698,-14.8853393971188));
#48435=CARTESIAN_POINT('Ctrl Pts',(-6.99033942241299,4.7744538169769,-14.9133960779864));
#48436=CARTESIAN_POINT('Ctrl Pts',(-6.9849529474007,4.73882903512714,-14.9410624452149));
#48437=CARTESIAN_POINT('Ctrl Pts',(-6.9781797927941,4.70446949083707,-14.9682300007031));
#48438=CARTESIAN_POINT('Ctrl Pts',(-6.97105384631412,4.6683202682209,-14.9968126269157));
#48439=CARTESIAN_POINT('Ctrl Pts',(-6.96239262273182,4.63357165756106,-15.0248431548408));
#48440=CARTESIAN_POINT('Ctrl Pts',(-6.95247705584319,4.60028408585532,-15.0522212395062));
#48441=CARTESIAN_POINT('Ctrl Pts',(-6.94757952211403,4.58384256445549,-15.0657439250566));
#48442=CARTESIAN_POINT('Ctrl Pts',(-6.94237537208527,4.56775702816083,-15.0791078258971));
#48443=CARTESIAN_POINT('Ctrl Pts',(-6.93689528828872,4.55203217545746,-15.0923029711967));
#48444=CARTESIAN_POINT('Ctrl Pts',(-6.93467726086207,4.54566764603222,-15.0976436183947));
#48445=CARTESIAN_POINT('Ctrl Pts',(-6.93241400773592,4.53936217946447,-15.1029566354528));
#48446=CARTESIAN_POINT('Ctrl Pts',(-6.93010747891385,4.5331160093562,-15.1082414213626));
#48447=CARTESIAN_POINT('Ctrl Pts',(-6.91797461530297,4.50025974097198,-15.1360405912857));
#48448=CARTESIAN_POINT('Ctrl Pts',(-6.90464803705654,4.46904585533628,-15.1630568165268));
#48449=CARTESIAN_POINT('Ctrl Pts',(-6.89043334783286,4.43945534086122,-15.1892214494785));
#48450=CARTESIAN_POINT('Ctrl Pts',(-6.88415593696834,4.42638774479002,-15.2007761270781));
#48451=CARTESIAN_POINT('Ctrl Pts',(-6.87770473235698,4.41363646979168,-15.2121650142821));
#48452=CARTESIAN_POINT('Ctrl Pts',(-6.87110345805848,4.40119860659756,-15.2233834948398));
#48453=CARTESIAN_POINT('Ctrl Pts',(-6.8589079386848,4.37822028533836,-15.2441090685394));
#48454=CARTESIAN_POINT('Ctrl Pts',(-6.84620107686014,4.35631215709294,-15.2642525838018));
#48455=CARTESIAN_POINT('Ctrl Pts',(-6.83312021232246,4.33544918998589,-15.2837912532757));
#48456=CARTESIAN_POINT('Ctrl Pts',(-6.82657978005362,4.32501770643236,-15.2935605880126));
#48457=CARTESIAN_POINT('Ctrl Pts',(-6.81994561022378,4.31484737937306,-15.3031788347256));
#48458=CARTESIAN_POINT('Ctrl Pts',(-6.81323353961138,4.30493429434116,-15.3126438440873));
#48459=CARTESIAN_POINT('Ctrl Pts',(-6.80987750430517,4.2999777518252,-15.3173763487682));
#48460=CARTESIAN_POINT('Ctrl Pts',(-6.80650198885739,4.2950855234087,-15.3220705443057));
#48461=CARTESIAN_POINT('Ctrl Pts',(-6.80310888496519,4.29025705555333,-15.3267262121182));
#48462=CARTESIAN_POINT('Ctrl Pts',(-6.80264177898385,4.28959235258884,-15.3273671268533));
#48463=CARTESIAN_POINT('Ctrl Pts',(-6.80218983720927,4.28895089234423,-15.3279861090097));
#48464=CARTESIAN_POINT('Ctrl Pts',(-6.80174677252703,4.28832348630925,-15.3285919214149));
#48465=CARTESIAN_POINT('Ctrl Pts',(-6.79969749752605,4.28542159059405,-15.3313939416772));
#48466=CARTESIAN_POINT('Ctrl Pts',(-6.79784094933337,4.28281805980717,-15.3339144164748));
#48467=CARTESIAN_POINT('Ctrl Pts',(-6.79553303480481,4.27962145346957,-15.3370189588579));
#48468=CARTESIAN_POINT('Ctrl Pts',(-6.79471526443204,4.27848879022579,-15.3381190008008));
#48469=CARTESIAN_POINT('Ctrl Pts',(-6.79384050039992,4.27728192903732,-15.3392923513023));
#48470=CARTESIAN_POINT('Ctrl Pts',(-6.79287881305449,4.27596226696631,-15.3405774256209));
#48471=CARTESIAN_POINT('Ctrl Pts',(-6.76344871351334,4.23557722260151,-15.3799039960427));
#48472=CARTESIAN_POINT('Ctrl Pts',(-6.73147738565455,4.19791990254157,-15.4183236940747));
#48473=CARTESIAN_POINT('Ctrl Pts',(-6.69741369430494,4.16317486975606,-15.4556739695271));
#48474=CARTESIAN_POINT('Ctrl Pts',(-6.6723851532128,4.13764570816594,-15.4831173518185));
#48475=CARTESIAN_POINT('Ctrl Pts',(-6.64622571368188,4.11368903830416,-15.5099838815156));
#48476=CARTESIAN_POINT('Ctrl Pts',(-6.61909739248669,4.09137864535545,-15.53621638348));
#48477=CARTESIAN_POINT('Ctrl Pts',(-6.58048856707105,4.05962665966812,-15.5735502856139));
#48478=CARTESIAN_POINT('Ctrl Pts',(-6.53991979868992,4.03120839444587,-15.6095992241468));
#48479=CARTESIAN_POINT('Ctrl Pts',(-6.4979261990087,4.00620592936192,-15.6442274537135));
#48480=CARTESIAN_POINT('Ctrl Pts',(-6.46405457048637,3.98603918452713,-15.6721582464336));
#48481=CARTESIAN_POINT('Ctrl Pts',(-6.4292547471293,3.9680951187726,-15.6991651680106));
#48482=CARTESIAN_POINT('Ctrl Pts',(-6.39378500341098,3.95241730850598,-15.72518648339));
#48483=CARTESIAN_POINT('Ctrl Pts',(-6.35127484432409,3.93362759821485,-15.7563727886877));
#48484=CARTESIAN_POINT('Ctrl Pts',(-6.30780377631186,3.91809224092562,-15.7861432724349));
#48485=CARTESIAN_POINT('Ctrl Pts',(-6.26385524237827,3.90575711203162,-15.8144219713711));
#48486=CARTESIAN_POINT('Ctrl Pts',(-6.22266644339182,3.97375010659389,-14.571407576345));
#48487=CARTESIAN_POINT('Ctrl Pts',(-6.22400197463445,3.9271886321768,-14.9771430893856));
#48488=CARTESIAN_POINT('Ctrl Pts',(-6.22726156144324,3.85975967588295,-16.0460292272317));
#48489=CARTESIAN_POINT('Ctrl Pts',(-6.23205009249213,3.98190899774585,-17.7794229322491));
#48490=CARTESIAN_POINT('Ctrl Pts',(-6.2357039221351,4.44990335836682,-19.7179581688241));
#48491=CARTESIAN_POINT('Ctrl Pts',(-6.23759309150179,5.23225296824271,-21.5545940964061));
#48492=CARTESIAN_POINT('Ctrl Pts',(-6.23804028505047,6.30682939060215,-23.2351598502083));
#48493=CARTESIAN_POINT('Ctrl Pts',(-6.23649343327119,7.54006311272245,-24.5993882837727));
#48494=CARTESIAN_POINT('Ctrl Pts',(-6.23490564632112,8.44425758305475,-25.3447862637746));
#48495=CARTESIAN_POINT('Ctrl Pts',(-6.23413035365508,8.85534224317308,-25.6421049454179));
#48496=CARTESIAN_POINT('Ctrl Pts',(-6.7158893426021,4.08565830959416,-14.5843360049734));
#48497=CARTESIAN_POINT('Ctrl Pts',(-6.71707806185619,4.04021185391681,-14.986317551748));
#48498=CARTESIAN_POINT('Ctrl Pts',(-6.71993259305533,3.97507670179734,-16.0451895055534));
#48499=CARTESIAN_POINT('Ctrl Pts',(-6.72416345393324,4.09849003995885,-17.7615688573897));
#48500=CARTESIAN_POINT('Ctrl Pts',(-6.7273671322325,4.56367551651715,-19.6804271855846));
#48501=CARTESIAN_POINT('Ctrl Pts',(-6.72902318958527,5.33903737570472,-21.498209528469));
#48502=CARTESIAN_POINT('Ctrl Pts',(-6.72941818465536,6.40302974530858,-23.1617881848097));
#48503=CARTESIAN_POINT('Ctrl Pts',(-6.72805064861496,7.62318866866407,-24.5127366297367));
#48504=CARTESIAN_POINT('Ctrl Pts',(-6.72668237271919,8.51793580395378,-25.251400142793));
#48505=CARTESIAN_POINT('Ctrl Pts',(-6.72598922608832,8.92472441076612,-25.5461005895199));
#48506=CARTESIAN_POINT('Ctrl Pts',(-7.02184868340148,4.48559520701657,-14.6305388743154));
#48507=CARTESIAN_POINT('Ctrl Pts',(-7.0224916377447,4.44215040628042,-15.0188750689058));
#48508=CARTESIAN_POINT('Ctrl Pts',(-7.02397830295891,4.38031978877979,-16.0419185664938));
#48509=CARTESIAN_POINT('Ctrl Pts',(-7.02622834797599,4.50113166000826,-17.6995249602702));
#48510=CARTESIAN_POINT('Ctrl Pts',(-7.0279017053608,4.95159320929153,-19.5522389867469));
#48511=CARTESIAN_POINT('Ctrl Pts',(-7.02876624731174,5.70076832635135,-21.307097360822));
#48512=CARTESIAN_POINT('Ctrl Pts',(-7.02897616615894,6.72847743169267,-22.913633439955));
#48513=CARTESIAN_POINT('Ctrl Pts',(-7.02824786192413,7.90599646240988,-24.2181479833785));
#48514=CARTESIAN_POINT('Ctrl Pts',(-7.02756291581688,8.76993137994633,-24.9320755587743));
#48515=CARTESIAN_POINT('Ctrl Pts',(-7.0271842308215,9.16263674770637,-25.2169010333086));
#48516=CARTESIAN_POINT('Ctrl Pts',(-6.99898915857891,4.98714290566693,-14.6884801835189));
#48517=CARTESIAN_POINT('Ctrl Pts',(-6.99894180139976,4.94565482841703,-15.0596401545356));
#48518=CARTESIAN_POINT('Ctrl Pts',(-6.99873531968,4.88660272557302,-16.0377412505386));
#48519=CARTESIAN_POINT('Ctrl Pts',(-6.99850468875347,5.00216540786785,-17.622209754351));
#48520=CARTESIAN_POINT('Ctrl Pts',(-6.99828080922558,5.43285448097263,-19.3931401195663));
#48521=CARTESIAN_POINT('Ctrl Pts',(-6.99816434197815,6.14885086491948,-21.0703309166242));
#48522=CARTESIAN_POINT('Ctrl Pts',(-6.99814257319851,7.13148866687968,-22.6063548637163));
#48523=CARTESIAN_POINT('Ctrl Pts',(-6.99821546038094,8.25667497594392,-23.8529245372788));
#48524=CARTESIAN_POINT('Ctrl Pts',(-6.99835922376522,9.08279278767221,-24.5356450620554));
#48525=CARTESIAN_POINT('Ctrl Pts',(-6.99838072452425,9.45819126329241,-24.8079421081757));
#48526=CARTESIAN_POINT('',(-7.00000355772625,9.33251603084022,-24.7867164850604));
#48527=CARTESIAN_POINT('Ctrl Pts',(-7.00001601631093,4.92966193678578,-14.796799000993));
#48528=CARTESIAN_POINT('Ctrl Pts',(-7.00002088956044,4.90663940121656,-15.0161851012847));
#48529=CARTESIAN_POINT('Ctrl Pts',(-7.00001598261872,4.89043246190617,-15.2342927807288));
#48530=CARTESIAN_POINT('Ctrl Pts',(-7.00000988115456,4.88069442451672,-15.450630170061));
#48531=CARTESIAN_POINT('Ctrl Pts',(-7.00000652438509,4.87533696510621,-15.5696499207533));
#48532=CARTESIAN_POINT('Ctrl Pts',(-7.00000279083273,4.87193754627854,-15.6881347839494));
#48533=CARTESIAN_POINT('Ctrl Pts',(-6.99999999965565,4.87043898511339,-15.8060095302866));
#48534=CARTESIAN_POINT('Ctrl Pts',(-6.99999455428889,4.86751541025449,-16.035973880696));
#48535=CARTESIAN_POINT('Ctrl Pts',(-6.99999266088529,4.87182596457363,-16.2636132173433));
#48536=CARTESIAN_POINT('Ctrl Pts',(-6.99999257352099,4.88291847944131,-16.4885165155108));
#48537=CARTESIAN_POINT('Ctrl Pts',(-6.99999248489166,4.89417161290698,-16.7166763928098));
#48538=CARTESIAN_POINT('Ctrl Pts',(-6.99999425322773,4.91240450885411,-16.9420204741633));
#48539=CARTESIAN_POINT('Ctrl Pts',(-6.99999619758933,4.93715565208034,-17.1641725428281));
#48540=CARTESIAN_POINT('Ctrl Pts',(-6.9999975442523,4.95429827007814,-17.3180348519641));
#48541=CARTESIAN_POINT('Ctrl Pts',(-6.99999897835725,4.97456787013135,-17.4703670834906));
#48542=CARTESIAN_POINT('Ctrl Pts',(-6.99999998662342,4.99781411395893,-17.6210585462649));
#48543=CARTESIAN_POINT('Ctrl Pts',(-7.00000143707765,5.03125529598881,-17.8378376816109));
#48544=CARTESIAN_POINT('Ctrl Pts',(-7.00000201440503,5.07085505448822,-18.0512192862196));
#48545=CARTESIAN_POINT('Ctrl Pts',(-7.00000210874351,5.11608568717109,-18.2609089713827));
#48546=CARTESIAN_POINT('Ctrl Pts',(-7.00000220459618,5.16204229772174,-18.4739642975174));
#48547=CARTESIAN_POINT('Ctrl Pts',(-7.00000180216116,5.21381197632272,-18.6832082948446));
#48548=CARTESIAN_POINT('Ctrl Pts',(-7.00000129011628,5.27086486939416,-18.8883810460748));
#48549=CARTESIAN_POINT('Ctrl Pts',(-7.00000086166913,5.31860316431548,-19.0600567803058));
#48550=CARTESIAN_POINT('Ctrl Pts',(-7.00000035619187,5.37004082573362,-19.2288830308296));
#48551=CARTESIAN_POINT('Ctrl Pts',(-6.9999999881669,5.42487991567195,-19.3947325990114));
#48552=CARTESIAN_POINT('Ctrl Pts',(-6.99999970373616,5.46726269967022,-19.522910627355));
#48553=CARTESIAN_POINT('Ctrl Pts',(-6.99999950020192,5.51167736194704,-19.649311172218));
#48554=CARTESIAN_POINT('Ctrl Pts',(-6.99999936067801,5.55798420729282,-19.7738901766392));
#48555=CARTESIAN_POINT('Ctrl Pts',(-6.99999924479304,5.59644547829981,-19.8773622835177));
#48556=CARTESIAN_POINT('Ctrl Pts',(-6.99999917321881,5.63621216193175,-19.9795779269211));
#48557=CARTESIAN_POINT('Ctrl Pts',(-6.99999913936905,5.67720658810105,-20.0805154986122));
#48558=CARTESIAN_POINT('Ctrl Pts',(-6.99999912244417,5.69770380118571,-20.1309842844577));
#48559=CARTESIAN_POINT('Ctrl Pts',(-6.99999911499176,5.71850794990473,-20.1811335523751));
#48560=CARTESIAN_POINT('Ctrl Pts',(-6.99999911640478,5.73960956204947,-20.230960959118));
#48561=CARTESIAN_POINT('Ctrl Pts',(-6.99999911711129,5.75016036812184,-20.2558746624894));
#48562=CARTESIAN_POINT('Ctrl Pts',(-6.99999912003637,5.76078554005064,-20.2807079005672));
#48563=CARTESIAN_POINT('Ctrl Pts',(-6.99999912511632,5.77148390014131,-20.3054603897257));
#48564=CARTESIAN_POINT('Ctrl Pts',(-6.9999991276563,5.77683308018664,-20.3178366343049));
#48565=CARTESIAN_POINT('Ctrl Pts',(-6.99999913073513,5.78220055727244,-20.3301926916542));
#48566=CARTESIAN_POINT('Ctrl Pts',(-6.99999913434553,5.78758618501739,-20.3425285275642));
#48567=CARTESIAN_POINT('Ctrl Pts',(-6.99999913750175,5.79229430807622,-20.3533125320013));
#48568=CARTESIAN_POINT('Ctrl Pts',(-6.9999991405722,5.79641055093021,-20.3627040187471));
#48569=CARTESIAN_POINT('Ctrl Pts',(-6.99999914483738,5.8015232455565,-20.3743145538044));
#48570=CARTESIAN_POINT('Ctrl Pts',(-6.99999914545115,5.80225896858769,-20.375985324048));
#48571=CARTESIAN_POINT('Ctrl Pts',(-6.9999991460916,5.80301540493209,-20.3777020105704));
#48572=CARTESIAN_POINT('Ctrl Pts',(-6.99999914676467,5.80379737409617,-20.379475337135));
#48573=CARTESIAN_POINT('Ctrl Pts',(-6.99999923697453,5.90860230533353,-20.6171488634125));
#48574=CARTESIAN_POINT('Ctrl Pts',(-6.9999995214453,6.02101278168188,-20.8492787963373));
#48575=CARTESIAN_POINT('Ctrl Pts',(-6.99999999018456,6.14041872174611,-21.0754662956648));
#48576=CARTESIAN_POINT('Ctrl Pts',(-7.00000044364536,6.25593264860106,-21.2942812577912));
#48577=CARTESIAN_POINT('Ctrl Pts',(-7.00000106797376,6.37799274547658,-21.5075353975042));
#48578=CARTESIAN_POINT('Ctrl Pts',(-7.00000142593565,6.50595991927143,-21.7149354344823));
#48579=CARTESIAN_POINT('Ctrl Pts',(-7.00000178766098,6.63527247524171,-21.9245159706046));
#48580=CARTESIAN_POINT('Ctrl Pts',(-7.00000187627602,6.77061697952042,-22.1281187040794));
#48581=CARTESIAN_POINT('Ctrl Pts',(-7.00000131558935,6.91136695665694,-22.3254829114096));
#48582=CARTESIAN_POINT('Ctrl Pts',(-7.00000103872994,6.98086737080238,-22.4229386583022));
#48583=CARTESIAN_POINT('Ctrl Pts',(-7.00000060480719,7.05168627710489,-22.5188739333697));
#48584=CARTESIAN_POINT('Ctrl Pts',(-6.99999997635806,7.12375115357989,-22.6132610028137));
#48585=CARTESIAN_POINT('Ctrl Pts',(-6.99999887928565,7.24955351900321,-22.7780308210977));
#48586=CARTESIAN_POINT('Ctrl Pts',(-6.99999719588034,7.37915178875968,-22.938081812605));
#48587=CARTESIAN_POINT('Ctrl Pts',(-6.99999590265529,7.51215857783395,-23.0933374643164));
#48588=CARTESIAN_POINT('Ctrl Pts',(-6.99999568173125,7.53488037422716,-23.1198600751669));
#48589=CARTESIAN_POINT('Ctrl Pts',(-6.99999546003663,7.55895243512824,-23.1476964012996));
#48590=CARTESIAN_POINT('Ctrl Pts',(-6.99999525389908,7.58352724378226,-23.1758128231261));
#48591=CARTESIAN_POINT('Ctrl Pts',(-6.99999512031325,7.5994527562614,-23.1940334503127));
#48592=CARTESIAN_POINT('Ctrl Pts',(-6.99999499325438,7.61558863734904,-23.2123723370691));
#48593=CARTESIAN_POINT('Ctrl Pts',(-6.99999487632633,7.63169526645205,-23.2305558840532));
#48594=CARTESIAN_POINT('Ctrl Pts',(-6.99999457896547,7.67265618698126,-23.2767986340535));
#48595=CARTESIAN_POINT('Ctrl Pts',(-6.9999943432934,7.71387538342522,-23.3225491432378));
#48596=CARTESIAN_POINT('Ctrl Pts',(-6.99999419422085,7.75533955273339,-23.3678076333183));
#48597=CARTESIAN_POINT('Ctrl Pts',(-6.99999365475326,7.90539115674498,-23.5315902230827));
#48598=CARTESIAN_POINT('Ctrl Pts',(-6.99999426201921,8.05865167046422,-23.6889299522383));
#48599=CARTESIAN_POINT('Ctrl Pts',(-6.99999708882611,8.21454310880251,-23.8398765708448));
#48600=CARTESIAN_POINT('Ctrl Pts',(-6.99999738657627,8.23096329713509,-23.8557759167749));
#48601=CARTESIAN_POINT('Ctrl Pts',(-6.99999770879859,8.2474127126713,-23.8716043620776));
#48602=CARTESIAN_POINT('Ctrl Pts',(-6.9999980566388,8.26389070674912,-23.8873619847489));
#48603=CARTESIAN_POINT('Ctrl Pts',(-6.99999863108762,8.29110367429903,-23.913385278142));
#48604=CARTESIAN_POINT('Ctrl Pts',(-6.99999927541382,8.31839458405079,-23.9392154108886));
#48605=CARTESIAN_POINT('Ctrl Pts',(-6.99999999465517,8.34576054507866,-23.964852756693));
#48606=CARTESIAN_POINT('Ctrl Pts',(-7.00000393353144,8.49562836482666,-24.1052539330275));
#48607=CARTESIAN_POINT('Ctrl Pts',(-7.0000100648746,8.64774332432774,-24.2398711438475));
#48608=CARTESIAN_POINT('Ctrl Pts',(-7.00001375756538,8.801556306293,-24.3687673244932));
#48609=CARTESIAN_POINT('Ctrl Pts',(-7.00001750474233,8.95763882034422,-24.4995653863326));
#48610=CARTESIAN_POINT('Ctrl Pts',(-7.00001874207225,9.11546988079917,-24.6244724111923));
#48611=CARTESIAN_POINT('Ctrl Pts',(-7.00001328548767,9.27452274288354,-24.7435795241592));
#48612=CARTESIAN_POINT('Ctrl Pts',(-7.00001262288462,9.29383682270603,-24.7580429186377));
#48613=CARTESIAN_POINT('Ctrl Pts',(-7.00001186234282,9.31316897447241,-24.7724208189439));
#48614=CARTESIAN_POINT('Ctrl Pts',(-7.00001099700068,9.33251830079054,-24.78671341245));
#48615=CARTESIAN_POINT('',(-6.271594443024,8.76071211955143,-25.5608538793675));
#48616=CARTESIAN_POINT('Origin',(-5.99998362343976,9.33252812935656,-24.7867137526282));
#48617=CARTESIAN_POINT('Ctrl Pts',(-6.26386059972761,3.90573753010371,-15.8144217562401));
#48618=CARTESIAN_POINT('Ctrl Pts',(-6.26455151911071,3.90327937979186,-16.055503426337));
#48619=CARTESIAN_POINT('Ctrl Pts',(-6.26520985433926,3.90810428962811,-16.2942778967187));
#48620=CARTESIAN_POINT('Ctrl Pts',(-6.26583560602987,3.91978334776613,-16.530318334847));
#48621=CARTESIAN_POINT('Ctrl Pts',(-6.26647065912245,3.93163600769524,-16.7698673643654));
#48622=CARTESIAN_POINT('Ctrl Pts',(-6.26707215281053,3.95054807030025,-17.0066005232977));
#48623=CARTESIAN_POINT('Ctrl Pts',(-6.26764008773865,3.97607950396293,-17.2401251768554));
#48624=CARTESIAN_POINT('Ctrl Pts',(-6.26812467974631,3.99786426852748,-17.439380716712));
#48625=CARTESIAN_POINT('Ctrl Pts',(-6.26858483962897,4.02446833721895,-17.6363012859027));
#48626=CARTESIAN_POINT('Ctrl Pts',(-6.26902056778702,4.05562321087888,-17.8306725452879));
#48627=CARTESIAN_POINT('Ctrl Pts',(-6.26953467283132,4.09238208773099,-18.060006461558));
#48628=CARTESIAN_POINT('Ctrl Pts',(-6.27001476631168,4.13547469852272,-18.2857906056929));
#48629=CARTESIAN_POINT('Ctrl Pts',(-6.27046084888574,4.18435716611124,-18.5077346484473));
#48630=CARTESIAN_POINT('Ctrl Pts',(-6.27062083230447,4.2018884142141,-18.5873328412233));
#48631=CARTESIAN_POINT('Ctrl Pts',(-6.27077644113038,4.22016459485154,-18.6664375452147));
#48632=CARTESIAN_POINT('Ctrl Pts',(-6.27092767539381,4.23916135873699,-18.7450368123693));
#48633=CARTESIAN_POINT('Ctrl Pts',(-6.2713681556663,4.29449074999043,-18.9739626247259));
#48634=CARTESIAN_POINT('Ctrl Pts',(-6.27177152526386,4.35593088785102,-19.1985969560212));
#48635=CARTESIAN_POINT('Ctrl Pts',(-6.27213778418647,4.42289857276513,-19.418679907426));
#48636=CARTESIAN_POINT('Ctrl Pts',(-6.27250404310909,4.48986625767925,-19.6387628588308));
#48637=CARTESIAN_POINT('Ctrl Pts',(-6.27283319135677,4.56236154960823,-19.8542946369576));
#48638=CARTESIAN_POINT('Ctrl Pts',(-6.27312522892951,4.63982794512282,-20.0650654344146));
#48639=CARTESIAN_POINT('Ctrl Pts',(-6.27334042228337,4.69691050921155,-20.2203758431918));
#48640=CARTESIAN_POINT('Ctrl Pts',(-6.27353526484726,4.75658564368513,-20.372823737172));
#48641=CARTESIAN_POINT('Ctrl Pts',(-6.27370997834722,4.81874467904067,-20.5226549488179));
#48642=CARTESIAN_POINT('Ctrl Pts',(-6.27388469184718,4.8809037143962,-20.6724861604638));
#48643=CARTESIAN_POINT('Ctrl Pts',(-6.27403927628321,4.9455469204707,-20.8197010220538));
#48644=CARTESIAN_POINT('Ctrl Pts',(-6.27417395338137,5.01262254914156,-20.964537762537));
#48645=CARTESIAN_POINT('Ctrl Pts',(-6.27427013810291,5.06052713539966,-21.06797837525));
#48646=CARTESIAN_POINT('Ctrl Pts',(-6.2743561688078,5.10967355132922,-21.1702058670971));
#48647=CARTESIAN_POINT('Ctrl Pts',(-6.27443212626672,5.16004860092251,-21.2713083696084));
#48648=CARTESIAN_POINT('Ctrl Pts',(-6.27457884535597,5.25735282228214,-21.4665975130196));
#48649=CARTESIAN_POINT('Ctrl Pts',(-6.27469165518935,5.361220077299,-21.6616515214675));
#48650=CARTESIAN_POINT('Ctrl Pts',(-6.27477055576686,5.47186344552789,-21.8559685725165));
#48651=CARTESIAN_POINT('Ctrl Pts',(-6.2748486289147,5.5813464977181,-22.048247822344));
#48652=CARTESIAN_POINT('Ctrl Pts',(-6.27489350028957,5.69746436261258,-22.2398055710169));
#48653=CARTESIAN_POINT('Ctrl Pts',(-6.27490516989148,5.82040565000112,-22.4301086125228));
#48654=CARTESIAN_POINT('Ctrl Pts',(-6.27491664590315,5.94130743047287,-22.6172546643983));
#48655=CARTESIAN_POINT('Ctrl Pts',(-6.27489601259132,6.06880817075117,-22.8031873173268));
#48656=CARTESIAN_POINT('Ctrl Pts',(-6.274843269956,6.20306900142315,-22.9873530700936));
#48657=CARTESIAN_POINT('Ctrl Pts',(-6.27479056739024,6.33722783162172,-23.1713789086809));
#48658=CARTESIAN_POINT('Ctrl Pts',(-6.27470580427057,6.47813658315848,-23.3536406777549));
#48659=CARTESIAN_POINT('Ctrl Pts',(-6.27458898059699,6.62593646339166,-23.5335379663002));
#48660=CARTESIAN_POINT('Ctrl Pts',(-6.27454781430459,6.67801814255145,-23.5969301209417));
#48661=CARTESIAN_POINT('Ctrl Pts',(-6.2745026670527,6.73095531727352,-23.6600282253355));
#48662=CARTESIAN_POINT('Ctrl Pts',(-6.27445353882921,6.78475355174986,-23.7228045290797));
#48663=CARTESIAN_POINT('Ctrl Pts',(-6.2743162411642,6.9351024031862,-23.8982442113896));
#48664=CARTESIAN_POINT('Ctrl Pts',(-6.27414785116967,7.09217882866916,-24.0711732887822));
#48665=CARTESIAN_POINT('Ctrl Pts',(-6.27394836858148,7.25599619752528,-24.2410355074747));
#48666=CARTESIAN_POINT('Ctrl Pts',(-6.27375072704948,7.41830167010394,-24.4093300410193));
#48667=CARTESIAN_POINT('Ctrl Pts',(-6.27352256419231,7.58722431676834,-24.5746141115647));
#48668=CARTESIAN_POINT('Ctrl Pts',(-6.27326387975308,7.7627444823766,-24.7363080568393));
#48669=CARTESIAN_POINT('Ctrl Pts',(-6.27300884328111,7.93578946308133,-24.8957217945323));
#48670=CARTESIAN_POINT('Ctrl Pts',(-6.27272413998789,8.11524724760931,-25.0516459606413));
#48671=CARTESIAN_POINT('Ctrl Pts',(-6.27240976962724,8.30106617556184,-25.2034869209588));
#48672=CARTESIAN_POINT('Ctrl Pts',(-6.27215746663657,8.45019814572994,-25.3253493265483));
#48673=CARTESIAN_POINT('Ctrl Pts',(-6.27188605472208,8.60342680986372,-25.4445809859663));
#48674=CARTESIAN_POINT('Ctrl Pts',(-6.27159553375651,8.76070944735753,-25.5608567073952));
#48675=CARTESIAN_POINT('Origin',(-5.999994993362,9.33250915082854,-24.7867196013936));
#48676=CARTESIAN_POINT('',(-5.98852246669543,9.69456809148957,-25.7188096068238));
#48677=CARTESIAN_POINT('Origin',(-5.999994993362,9.33250915082854,-24.7867196013936));
#48678=CARTESIAN_POINT('Origin',(-6.,9.33251101023601,-24.7867243682982));
#48679=CARTESIAN_POINT('Ctrl Pts',(-5.9884183312965,9.69410641344453,-25.7189877462122));
#48680=CARTESIAN_POINT('Ctrl Pts',(-5.98810627248762,9.81679904525013,-25.6713270163599));
#48681=CARTESIAN_POINT('Ctrl Pts',(-5.9872640505538,10.2439466077869,-25.5029619472033));
#48682=CARTESIAN_POINT('Ctrl Pts',(-5.98726405055286,10.7897532290078,-25.2768814422167));
#48683=CARTESIAN_POINT('Ctrl Pts',(-5.98810627251012,11.2108442522874,-25.0938945847795));
#48684=CARTESIAN_POINT('Ctrl Pts',(-5.98841833133919,11.3313022744201,-25.0408390158645));
#48685=CARTESIAN_POINT('Ctrl Pts',(-6.58019637133009,9.69658812787628,-25.7253769286093));
#48686=CARTESIAN_POINT('Ctrl Pts',(-6.57988216396863,9.81936872043664,-25.6778801575558));
#48687=CARTESIAN_POINT('Ctrl Pts',(-6.57903377270813,10.2467760977028,-25.5099484803168));
#48688=CARTESIAN_POINT('Ctrl Pts',(-6.57903377270728,10.7926927024447,-25.2838224186652));
#48689=CARTESIAN_POINT('Ctrl Pts',(-6.57988216399013,11.2136609881125,-25.1003453900946));
#48690=CARTESIAN_POINT('Ctrl Pts',(-6.5801963713722,11.3340652715104,-25.0471116871477));
#48691=CARTESIAN_POINT('Ctrl Pts',(-7.00079676886773,9.54584602334702,-25.3372908808639));
#48692=CARTESIAN_POINT('Ctrl Pts',(-7.00061248422704,9.66739289539033,-25.2904141386208));
#48693=CARTESIAN_POINT('Ctrl Pts',(-7.00011448375567,10.0904742433784,-25.1245686185404));
#48694=CARTESIAN_POINT('Ctrl Pts',(-7.00011448375563,10.6307100898621,-24.9007956040115));
#48695=CARTESIAN_POINT('Ctrl Pts',(-7.0006124842397,11.04714427498,-24.7189024042084));
#48696=CARTESIAN_POINT('Ctrl Pts',(-7.00079676889193,11.1662377596005,-24.666102646838));
#48697=CARTESIAN_POINT('Ctrl Pts',(-6.99999917319659,9.33157252936654,-24.7856430600347));
#48698=CARTESIAN_POINT('Ctrl Pts',(-6.99999957777432,9.45129807495918,-24.7394735073194));
#48699=CARTESIAN_POINT('Ctrl Pts',(-7.00000004362305,9.86804157465028,-24.576125664719));
#48700=CARTESIAN_POINT('Ctrl Pts',(-7.00000004362386,10.4001860063983,-24.3557042239056));
#48701=CARTESIAN_POINT('Ctrl Pts',(-6.99999957777458,10.810372531279,-24.1765264349544));
#48702=CARTESIAN_POINT('Ctrl Pts',(-6.99999917319582,10.9276780850348,-24.1245144913973));
#48703=CARTESIAN_POINT('Origin',(-5.9885235341522,-4.75229019723222,11.4730434407793));
#48704=CARTESIAN_POINT('Origin',(-7.00021006962832,-4.74293597589513,11.4504603050761));
#48705=CARTESIAN_POINT('Ctrl Pts',(-6.05505067660194,9.37215177151571,-25.8432012822673));
#48706=CARTESIAN_POINT('Ctrl Pts',(-4.03670045106797,8.81554919752502,-26.0304401291589));
#48707=CARTESIAN_POINT('Ctrl Pts',(7.61017729489916E-7,8.27058403888204,
-26.2482623545472));
#48708=CARTESIAN_POINT('Ctrl Pts',(4.03670197310351,8.81554940300285,-26.030440047027));
#48709=CARTESIAN_POINT('Ctrl Pts',(6.05505295965479,9.37215240111522,-25.8432010704704));
#48710=CARTESIAN_POINT('Ctrl Pts',(-6.05505067660194,10.1400029312564,-25.5527891512987));
#48711=CARTESIAN_POINT('Ctrl Pts',(-4.03670045106797,9.95059815166984,-25.6069178790708));
#48712=CARTESIAN_POINT('Ctrl Pts',(7.61017729489916E-7,9.8134122476049,
-25.7964932163722));
#48713=CARTESIAN_POINT('Ctrl Pts',(4.03670197310351,9.95059820339512,-25.6069178075902));
#48714=CARTESIAN_POINT('Ctrl Pts',(6.05505295965479,10.1400031454992,-25.552789090066));
#48715=CARTESIAN_POINT('Ctrl Pts',(-6.05505067660194,10.8990942198713,-25.2383558203596));
#48716=CARTESIAN_POINT('Ctrl Pts',(-4.03670045106797,11.0715877475132,-25.1425762612566));
#48717=CARTESIAN_POINT('Ctrl Pts',(7.61017729489916E-7,11.302923524876,
-25.1794671417429));
#48718=CARTESIAN_POINT('Ctrl Pts',(4.03670197310351,11.0715876602892,-25.1425762473493));
#48719=CARTESIAN_POINT('Ctrl Pts',(6.05505295965479,10.8990940247534,-25.2383559286956));
#48720=CARTESIAN_POINT('Ctrl Pts',(-6.05505067660194,11.6473935737486,-24.9007429977581));
#48721=CARTESIAN_POINT('Ctrl Pts',(-4.03670045106797,12.1736538531869,-24.6394300651268));
#48722=CARTESIAN_POINT('Ctrl Pts',(7.61017729489916E-7,12.7132743263768,
-24.4078888772065));
#48723=CARTESIAN_POINT('Ctrl Pts',(4.03670197310351,12.1736536497231,-24.6394301524292));
#48724=CARTESIAN_POINT('Ctrl Pts',(6.05505295965479,11.6473929784695,-24.9007432933403));
#48725=CARTESIAN_POINT('Ctrl Pts',(-5.98852262888393,9.6945676509312,-25.7188097476035));
#48726=CARTESIAN_POINT('Ctrl Pts',(-5.93914474573397,9.67822396126561,-25.7245504584746));
#48727=CARTESIAN_POINT('Ctrl Pts',(-5.88279573294254,9.65973790752962,-25.731062674358));
#48728=CARTESIAN_POINT('Ctrl Pts',(-5.8194048475461,9.63929488404148,-25.7382945464948));
#48729=CARTESIAN_POINT('Ctrl Pts',(-5.75829929143766,9.61958885988725,-25.7452656996167));
#48730=CARTESIAN_POINT('Ctrl Pts',(-5.69065018696235,9.59806460605636,-25.7529056167575));
#48731=CARTESIAN_POINT('Ctrl Pts',(-5.61638362499844,9.57493013737895,-25.7611526723746));
#48732=CARTESIAN_POINT('Ctrl Pts',(-5.54072805329341,9.55136298403837,-25.7695539729209));
#48733=CARTESIAN_POINT('Ctrl Pts',(-5.4582049597275,9.52612458268054,-25.7785855835354));
#48734=CARTESIAN_POINT('Ctrl Pts',(-5.36872850624103,9.49948016899468,-25.7881637857989));
#48735=CARTESIAN_POINT('Ctrl Pts',(-5.3239902794978,9.48615796215175,-25.7929528869306));
#48736=CARTESIAN_POINT('Ctrl Pts',(-5.27751361368163,9.47248497632851,-25.7978783252447));
#48737=CARTESIAN_POINT('Ctrl Pts',(-5.22928736188671,9.45849880618232,-25.8029276205075));
#48738=CARTESIAN_POINT('Ctrl Pts',(-5.20517423598925,9.45150572110923,-25.8054522681389));
#48739=CARTESIAN_POINT('Ctrl Pts',(-5.18062371361782,9.44443433851998,-25.8080078762341));
#48740=CARTESIAN_POINT('Ctrl Pts',(-5.1556343858912,9.43728971218247,-25.8105927199721));
#48741=CARTESIAN_POINT('Ctrl Pts',(-5.13189984629429,9.43050383868607,-25.8130477710532));
#48742=CARTESIAN_POINT('Ctrl Pts',(-5.10666091353175,9.42333916306116,-25.8156425536409));
#48743=CARTESIAN_POINT('Ctrl Pts',(-5.08307503285008,9.41669114214869,-25.8180525556873));
#48744=CARTESIAN_POINT('Ctrl Pts',(-5.08182810396034,9.41633967724275,-25.8181799667098));
#48745=CARTESIAN_POINT('Ctrl Pts',(-5.08058579897438,9.4159896453358,-25.8183068646897));
#48746=CARTESIAN_POINT('Ctrl Pts',(-5.0793485856463,9.41564117510416,-25.8184332028057));
#48747=CARTESIAN_POINT('Ctrl Pts',(-5.06433554013984,9.41141264043952,-25.8199662608815));
#48748=CARTESIAN_POINT('Ctrl Pts',(-5.04943318284293,9.40723478799857,-25.8214818625031));
#48749=CARTESIAN_POINT('Ctrl Pts',(-5.03464184081241,9.40310682556614,-25.8229802157136));
#48750=CARTESIAN_POINT('Ctrl Pts',(-4.91702209302933,9.37028154851154,-25.834895018734));
#48751=CARTESIAN_POINT('Ctrl Pts',(-4.80642474277852,9.34060758757959,-25.8457196403818));
#48752=CARTESIAN_POINT('Ctrl Pts',(-4.70298901843753,9.31371271080518,-25.8555634948917));
#48753=CARTESIAN_POINT('Ctrl Pts',(-4.59988946245336,9.28690524296602,-25.86537535666));
#48754=CARTESIAN_POINT('Ctrl Pts',(-4.50390474764424,9.26285864773517,-25.8742130202874));
#48755=CARTESIAN_POINT('Ctrl Pts',(-4.41514468579301,9.24124704046678,-25.8821770968963));
#48756=CARTESIAN_POINT('Ctrl Pts',(-4.38360632789255,9.23356797185621,-25.8850069045057));
#48757=CARTESIAN_POINT('Ctrl Pts',(-4.35297986988857,9.22619673491393,-25.8877263331032));
#48758=CARTESIAN_POINT('Ctrl Pts',(-4.32326948852073,9.21912007669597,-25.8903395887858));
#48759=CARTESIAN_POINT('Ctrl Pts',(-4.2886422544966,9.21087228286294,-25.8933853193325));
#48760=CARTESIAN_POINT('Ctrl Pts',(-4.25525940683351,9.20302460535569,-25.8962868365517));
#48761=CARTESIAN_POINT('Ctrl Pts',(-4.22312693641565,9.19555734174392,-25.8990504778776));
#48762=CARTESIAN_POINT('Ctrl Pts',(-4.20706070120673,9.19182370993804,-25.9004322985405));
#48763=CARTESIAN_POINT('Ctrl Pts',(-4.19130706030953,9.18818518239483,-25.9017796523655));
#48764=CARTESIAN_POINT('Ctrl Pts',(-4.17586669145764,9.18463945126438,-25.9030932880816));
#48765=CARTESIAN_POINT('Ctrl Pts',(-4.1681465070317,9.18286658569916,-25.9037501059396));
#48766=CARTESIAN_POINT('Ctrl Pts',(-4.16050464061708,9.18111691928206,-25.9043984943918));
#48767=CARTESIAN_POINT('Ctrl Pts',(-4.15294117518514,9.17939016816571,-25.9050385461194));
#48768=CARTESIAN_POINT('Ctrl Pts',(-4.14915944246918,9.17852679260754,-25.9053585719832));
#48769=CARTESIAN_POINT('Ctrl Pts',(-4.14539730999889,9.17766914587717,-25.9056765136729));
#48770=CARTESIAN_POINT('Ctrl Pts',(-4.14165478791372,9.17681719302608,-25.9059923826253));
#48771=CARTESIAN_POINT('Ctrl Pts',(-4.13978352687113,9.17639121660053,-25.9061503171014));
#48772=CARTESIAN_POINT('Ctrl Pts',(-4.13791716842483,9.17596666364496,-25.9063077333937));
#48773=CARTESIAN_POINT('Ctrl Pts',(-4.13605571382735,9.1755435298259,-25.9064646329216));
#48774=CARTESIAN_POINT('Ctrl Pts',(-4.13419425922987,9.17512039600684,-25.9066215324495));
#48775=CARTESIAN_POINT('Ctrl Pts',(-4.1340901684656,9.17509646730814,-25.9066303970282));
#48776=CARTESIAN_POINT('Ctrl Pts',(-4.13048606282949,9.17427838145572,-25.9069337826298));
#48777=CARTESIAN_POINT('Ctrl Pts',(-4.08691193609688,9.16438761236891,-25.9106017557657));
#48778=CARTESIAN_POINT('Ctrl Pts',(-4.04447551159814,9.15491120120482,-25.9141211943608));
#48779=CARTESIAN_POINT('Ctrl Pts',(-4.00318382525737,9.1458261516899,-25.9174993986425));
#48780=CARTESIAN_POINT('Ctrl Pts',(-3.90005318180312,9.12313521592729,-25.9259368448254));
#48781=CARTESIAN_POINT('Ctrl Pts',(-3.80406510638285,9.10288246048144,-25.9334941271089));
#48782=CARTESIAN_POINT('Ctrl Pts',(-3.71531264401003,9.08473979632614,-25.9402797321664));
#48783=CARTESIAN_POINT('Ctrl Pts',(-3.62707651135985,9.06670267962835,-25.9470258610281));
#48784=CARTESIAN_POINT('Ctrl Pts',(-3.54599178209802,9.05075106996483,-25.9530093831139));
#48785=CARTESIAN_POINT('Ctrl Pts',(-3.4721292247771,9.03660782871565,-25.9583241854749));
#48786=CARTESIAN_POINT('Ctrl Pts',(-3.4138364983745,9.02544590686393,-25.9625186560044));
#48787=CARTESIAN_POINT('Ctrl Pts',(-3.36004163323143,9.01541118372412,-25.9662963853087));
#48788=CARTESIAN_POINT('Ctrl Pts',(-3.31077175302537,9.00638811719138,-25.9696972084536));
#48789=CARTESIAN_POINT('Ctrl Pts',(-3.27749897070262,9.00029468795283,-25.9719938417668));
#48790=CARTESIAN_POINT('Ctrl Pts',(-3.2462896846622,8.99466300700617,-25.9741184688898));
#48791=CARTESIAN_POINT('Ctrl Pts',(-3.21715071744293,8.98946236732531,-25.9760817903242));
#48792=CARTESIAN_POINT('Ctrl Pts',(-3.20258123383329,8.98686204748487,-25.9770634510415));
#48793=CARTESIAN_POINT('Ctrl Pts',(-3.18852932993462,8.98436948858393,-25.9780047870712));
#48794=CARTESIAN_POINT('Ctrl Pts',(-3.17499573175916,8.98198129761811,-25.9789069868615));
#48795=CARTESIAN_POINT('Ctrl Pts',(-3.16822893267142,8.98078720213521,-25.9793580867567));
#48796=CARTESIAN_POINT('Ctrl Pts',(-3.16159171001477,8.97961919866815,-25.9797994026812));
#48797=CARTESIAN_POINT('Ctrl Pts',(-3.15508415158759,8.97847687591692,-25.980231079151));
#48798=CARTESIAN_POINT('Ctrl Pts',(-3.15183037237399,8.97790571454131,-25.9804469173859));
#48799=CARTESIAN_POINT('Ctrl Pts',(-3.14860900921778,8.97734097334633,-25.9806603457618));
#48800=CARTESIAN_POINT('Ctrl Pts',(-3.14542007266562,8.97678260251498,-25.9808713818034));
#48801=CARTESIAN_POINT('Ctrl Pts',(-3.14223113611345,8.97622423168362,-25.9810824178449));
#48802=CARTESIAN_POINT('Ctrl Pts',(-3.13737712858202,8.97537573052988,-25.9814031398511));
#48803=CARTESIAN_POINT('Ctrl Pts',(-3.13595055324389,8.97512655178081,-25.9814973302948));
#48804=CARTESIAN_POINT('Ctrl Pts',(-3.12014621626011,8.97236602114898,-25.982540820585));
#48805=CARTESIAN_POINT('Ctrl Pts',(-3.09726105140332,8.96836944993973,-25.9840516043252));
#48806=CARTESIAN_POINT('Ctrl Pts',(-3.06727915898629,8.96321423979775,-25.9860020089781));
#48807=CARTESIAN_POINT('Ctrl Pts',(-3.03741246016798,8.95807883651785,-25.9879449199702));
#48808=CARTESIAN_POINT('Ctrl Pts',(-3.00050338114547,8.9517936639778,-25.9903241089074));
#48809=CARTESIAN_POINT('Ctrl Pts',(-2.95652740131304,8.94448308321903,-25.9930947938812));
#48810=CARTESIAN_POINT('Ctrl Pts',(-2.93861217939317,8.94150485107604,-25.9942235336243));
#48811=CARTESIAN_POINT('Ctrl Pts',(-2.91952401304476,8.93835699328653,-25.9954170434176));
#48812=CARTESIAN_POINT('Ctrl Pts',(-2.89926087786538,8.93505022264859,-25.9966714405561));
#48813=CARTESIAN_POINT('Ctrl Pts',(-2.84967927921722,8.92695892911775,-25.9997408083968));
#48814=CARTESIAN_POINT('Ctrl Pts',(-2.79306320428941,8.91791283508941,-26.0031759944465));
#48815=CARTESIAN_POINT('Ctrl Pts',(-2.72937889204199,8.90810252116344,-26.0069075036621));
#48816=CARTESIAN_POINT('Ctrl Pts',(-2.66611328203675,8.89835670664544,-26.0106144795002));
#48817=CARTESIAN_POINT('Ctrl Pts',(-2.59587189772266,8.88785667520502,-26.0146139373803));
#48818=CARTESIAN_POINT('Ctrl Pts',(-2.51861771041027,8.87683697547256,-26.0188193598197));
#48819=CARTESIAN_POINT('Ctrl Pts',(-2.46588274151833,8.86931474861592,-26.0216900498009));
#48820=CARTESIAN_POINT('Ctrl Pts',(-2.40987996642888,8.86155135889636,-26.0246563335322));
#48821=CARTESIAN_POINT('Ctrl Pts',(-2.35059722894411,8.85363439251256,-26.0276855409131));
#48822=CARTESIAN_POINT('Ctrl Pts',(-2.31881048549239,8.84938940332962,-26.0293097681665));
#48823=CARTESIAN_POINT('Ctrl Pts',(-2.28608075625419,8.84510044232466,-26.03095201316));
#48824=CARTESIAN_POINT('Ctrl Pts',(-2.25240618731547,8.84078228822473,-26.0326067213317));
#48825=CARTESIAN_POINT('Ctrl Pts',(-2.23556890284611,8.83862321117477,-26.0334340754176));
#48826=CARTESIAN_POINT('Ctrl Pts',(-2.21849540844796,8.83645683557932,-26.034264544514));
#48827=CARTESIAN_POINT('Ctrl Pts',(-2.20118547662363,8.8342851098282,-26.0350973937513));
#48828=CARTESIAN_POINT('Ctrl Pts',(-2.19253051071147,8.83319924695263,-26.03551381837));
#48829=CARTESIAN_POINT('Ctrl Pts',(-2.18381643544252,8.83211204652001,-26.0359308379717));
#48830=CARTESIAN_POINT('Ctrl Pts',(-2.175043222636,8.83102375488626,-26.0363483593618));
#48831=CARTESIAN_POINT('Ctrl Pts',(-2.16846331303111,8.83020753616095,-26.0366615004044));
#48832=CARTESIAN_POINT('Ctrl Pts',(-2.16185013856133,8.82939070363346,-26.0369749236986));
#48833=CARTESIAN_POINT('Ctrl Pts',(-2.15520368740763,8.82857336242411,-26.0372885894234));
#48834=CARTESIAN_POINT('Ctrl Pts',(-2.15298820368973,8.82830091535433,-26.0373931446651));
#48835=CARTESIAN_POINT('Ctrl Pts',(-2.14946255515765,8.82786822056567,-26.0375592085574));
#48836=CARTESIAN_POINT('Ctrl Pts',(-2.14854614359539,8.82775585565574,-26.0376023344423));
#48837=CARTESIAN_POINT('Ctrl Pts',(-2.0128572772243,8.81111849764294,-26.0439877868723));
#48838=CARTESIAN_POINT('Ctrl Pts',(-1.87311902758234,8.79563658753315,-26.0499557569825));
#48839=CARTESIAN_POINT('Ctrl Pts',(-1.72934488860467,8.78158234860393,-26.055398450122));
#48840=CARTESIAN_POINT('Ctrl Pts',(-1.55033452067602,8.76408369064244,-26.0621750408801));
#48841=CARTESIAN_POINT('Ctrl Pts',(-1.36506673402777,8.74879789740494,-26.0681381321527));
#48842=CARTESIAN_POINT('Ctrl Pts',(-1.17358540971037,8.73625506698945,-26.0730583965713));
#48843=CARTESIAN_POINT('Ctrl Pts',(-0.995034403883234,8.72455922670536,
-26.0776464062063));
#48844=CARTESIAN_POINT('Ctrl Pts',(-0.811080758346082,8.7152487315044,-26.0813275280306));
#48845=CARTESIAN_POINT('Ctrl Pts',(-0.621784930566627,8.7087784386549,-26.0838952427685));
#48846=CARTESIAN_POINT('Ctrl Pts',(-0.437450969383238,8.70247774663777,
-26.086395651966));
#48847=CARTESIAN_POINT('Ctrl Pts',(-0.248049563901548,8.69887060590274,
-26.0878396659788));
#48848=CARTESIAN_POINT('Ctrl Pts',(-0.0537262494172971,8.69839152673885,
-26.0880418643833));
#48849=CARTESIAN_POINT('Ctrl Pts',(0.0580379594840133,8.69811598644203,
-26.0881581579159));
#48850=CARTESIAN_POINT('Ctrl Pts',(0.171429490699651,8.69887554117705,-26.0878634374378));
#48851=CARTESIAN_POINT('Ctrl Pts',(0.286413558273367,8.70075569448962,-26.0871205175796));
#48852=CARTESIAN_POINT('Ctrl Pts',(0.308600630279844,8.7011184847249,-26.0869771654027));
#48853=CARTESIAN_POINT('Ctrl Pts',(0.330846980306243,8.70152300397326,-26.0868171213266));
#48854=CARTESIAN_POINT('Ctrl Pts',(0.353152334505659,8.70196987549253,-26.086640112036));
#48855=CARTESIAN_POINT('Ctrl Pts',(0.48453063270388,8.70460194397212,-26.0855975292031));
#48856=CARTESIAN_POINT('Ctrl Pts',(0.617956407365337,8.70870289305593,-26.0839663359402));
#48857=CARTESIAN_POINT('Ctrl Pts',(0.753387312203915,8.71441095614992,-26.081705841676));
#48858=CARTESIAN_POINT('Ctrl Pts',(0.832599466679027,8.71774954401577,-26.080383701644));
#48859=CARTESIAN_POINT('Ctrl Pts',(0.912497509964033,8.72163786730543,-26.0788463388806));
#48860=CARTESIAN_POINT('Ctrl Pts',(0.993071857462417,8.72610454453892,-26.0770856585089));
#48861=CARTESIAN_POINT('Ctrl Pts',(1.03335903121161,8.72833788315566,-26.076205318323));
#48862=CARTESIAN_POINT('Ctrl Pts',(1.07381528101382,8.73071581154904,-26.0752691526353));
#48863=CARTESIAN_POINT('Ctrl Pts',(1.11443933439587,8.73324193498107,-26.0742761670545));
#48864=CARTESIAN_POINT('Ctrl Pts',(1.1347513610869,8.73450499669708,-26.073779674264));
#48865=CARTESIAN_POINT('Ctrl Pts',(1.15510533867405,8.73580510725891,-26.0732689767542));
#48866=CARTESIAN_POINT('Ctrl Pts',(1.17550110474873,8.73714272111241,-26.0727439506748));
#48867=CARTESIAN_POINT('Ctrl Pts',(1.18569898778607,8.73781152803917,-26.0724814376351));
#48868=CARTESIAN_POINT('Ctrl Pts',(1.19590731794535,8.73848971079429,-26.0722153424692));
#48869=CARTESIAN_POINT('Ctrl Pts',(1.20612607461619,8.73917732641975,-26.0719456497258));
#48870=CARTESIAN_POINT('Ctrl Pts',(1.21003384007692,8.73944027823257,-26.0718425162408));
#48871=CARTESIAN_POINT('Ctrl Pts',(1.21394313029209,8.73970460947776,-26.0717388566579));
#48872=CARTESIAN_POINT('Ctrl Pts',(1.21785394410087,8.7399703233597,-26.071634670111));
#48873=CARTESIAN_POINT('Ctrl Pts',(1.21905649432309,8.74005202867819,-26.0716026334144));
#48874=CARTESIAN_POINT('Ctrl Pts',(1.22025918860458,8.7401338647282,-26.0715705468922));
#48875=CARTESIAN_POINT('Ctrl Pts',(1.22146202691165,8.74021583159409,-26.0715384105174));
#48876=CARTESIAN_POINT('Ctrl Pts',(1.22401932140998,8.74039009725719,-26.0714700869745));
#48877=CARTESIAN_POINT('Ctrl Pts',(1.2265772669166,8.74056495423914,-26.0714015380865));
#48878=CARTESIAN_POINT('Ctrl Pts',(1.22913586310785,8.7407404033154,-26.0713327636059));
#48879=CARTESIAN_POINT('Ctrl Pts',(1.2316944592991,8.74091585239167,-26.0712639891253));
#48880=CARTESIAN_POINT('Ctrl Pts',(1.23563112013739,8.741186935779,-26.0711577403777));
#48881=CARTESIAN_POINT('Ctrl Pts',(1.23681360340992,8.74126852767454,-26.0711257631143));
#48882=CARTESIAN_POINT('Ctrl Pts',(1.30415700015864,8.74591525335826,-26.0693046316134));
#48883=CARTESIAN_POINT('Ctrl Pts',(1.37864975928608,8.75145208437293,-26.0671401719801));
#48884=CARTESIAN_POINT('Ctrl Pts',(1.46026019920768,8.75813439531587,-26.0645364370334));
#48885=CARTESIAN_POINT('Ctrl Pts',(1.54192310568886,8.76482100225165,-26.0619310281708));
#48886=CARTESIAN_POINT('Ctrl Pts',(1.63071306962372,8.7726546079288,-26.058885709424));
#48887=CARTESIAN_POINT('Ctrl Pts',(1.72658512627508,8.78193883475825,-26.0552879837732));
#48888=CARTESIAN_POINT('Ctrl Pts',(1.81123511500212,8.79013631923811,-26.0521113810548));
#48889=CARTESIAN_POINT('Ctrl Pts',(1.90140620465113,8.79946541363449,-26.0485038513462));
#48890=CARTESIAN_POINT('Ctrl Pts',(1.99705663527059,8.81016555726613,-26.0443780748945));
#48891=CARTESIAN_POINT('Ctrl Pts',(2.10633112278669,8.82238978567916,-26.0396646396862));
#48892=CARTESIAN_POINT('Ctrl Pts',(2.22275768465182,8.83640277908269,-26.0342749055327));
#48893=CARTESIAN_POINT('Ctrl Pts',(2.34625422416244,8.85260251429612,-26.0280670817374));
#48894=CARTESIAN_POINT('Ctrl Pts',(2.46249286483808,8.86785019012556,-26.0222240921089));
#48895=CARTESIAN_POINT('Ctrl Pts',(2.58499495411797,8.88503560594046,-26.0156561357011));
#48896=CARTESIAN_POINT('Ctrl Pts',(2.71367114820033,8.90452607693472,-26.0082356891927));
#48897=CARTESIAN_POINT('Ctrl Pts',(2.74257980920367,8.90890484662702,-26.006568596269));
#48898=CARTESIAN_POINT('Ctrl Pts',(2.77180000596921,8.91340009384957,-26.0048584431687));
#48899=CARTESIAN_POINT('Ctrl Pts',(2.80133057639793,8.91801616406612,-26.0031037454239));
#48900=CARTESIAN_POINT('Ctrl Pts',(2.82674886760609,8.92198942348165,-26.0015933980919));
#48901=CARTESIAN_POINT('Ctrl Pts',(2.85519251276494,8.92649299991863,-25.9998825579851));
#48902=CARTESIAN_POINT('Ctrl Pts',(2.88386923276027,8.93110569654494,-25.9981317011542));
#48903=CARTESIAN_POINT('Ctrl Pts',(2.89904594651544,8.93354689541107,-25.9972050870591));
#48904=CARTESIAN_POINT('Ctrl Pts',(2.91428808430034,8.93601787623561,-25.9962675472531));
#48905=CARTESIAN_POINT('Ctrl Pts',(2.92918279413114,8.93845060795178,-25.9953448837206));
#48906=CARTESIAN_POINT('Ctrl Pts',(3.02452062843766,8.95402200047323,-25.989439112881));
#48907=CARTESIAN_POINT('Ctrl Pts',(3.11288301577595,8.96919620282964,-25.9836990070561));
#48908=CARTESIAN_POINT('Ctrl Pts',(3.1943190206272,8.98368049199339,-25.9782314355906));
#48909=CARTESIAN_POINT('Ctrl Pts',(3.25134055044255,8.99382239824129,-25.9744030394174));
#48910=CARTESIAN_POINT('Ctrl Pts',(3.30496622924687,9.0036270924581,-25.9707078341751));
#48911=CARTESIAN_POINT('Ctrl Pts',(3.35521234116732,9.01300818178171,-25.9671769151241));
#48912=CARTESIAN_POINT('Ctrl Pts',(3.42777531237928,9.02655589101746,-25.9620777349557));
#48913=CARTESIAN_POINT('Ctrl Pts',(3.49329027393557,9.03921804241095,-25.9573219778677));
#48914=CARTESIAN_POINT('Ctrl Pts',(3.5518024689862,9.05077578986301,-25.9529875386592));
#48915=CARTESIAN_POINT('Ctrl Pts',(3.6106020683201,9.06239030746564,-25.9486318092498));
#48916=CARTESIAN_POINT('Ctrl Pts',(3.66233009124901,9.07288959914803,-25.9447014803238));
#48917=CARTESIAN_POINT('Ctrl Pts',(3.70702540622173,9.08210053382569,-25.9412572827147));
#48918=CARTESIAN_POINT('Ctrl Pts',(3.75194675858638,9.09135805091702,-25.9377956667823));
#48919=CARTESIAN_POINT('Ctrl Pts',(3.78976421224823,9.09931417924152,-25.9348250627982));
#48920=CARTESIAN_POINT('Ctrl Pts',(3.82050805513342,9.10584182648722,-25.9323895408546));
#48921=CARTESIAN_POINT('Ctrl Pts',(3.82703720645496,9.10722812021764,-25.9318723026104));
#48922=CARTESIAN_POINT('Ctrl Pts',(3.83324728642847,9.10855015939838,-25.9313791362946));
#48923=CARTESIAN_POINT('Ctrl Pts',(3.83913852491444,9.10980700565233,-25.9309103654691));
#48924=CARTESIAN_POINT('Ctrl Pts',(3.85140011662712,9.11242291326637,-25.9299347002532));
#48925=CARTESIAN_POINT('Ctrl Pts',(3.86228053968236,9.11475629400514,-25.9290647547988));
#48926=CARTESIAN_POINT('Ctrl Pts',(3.87178155207577,9.11680004991352,-25.928302970545));
#48927=CARTESIAN_POINT('Ctrl Pts',(3.87653205827248,9.11782192786771,-25.9279220784181));
#48928=CARTESIAN_POINT('Ctrl Pts',(3.88093771180439,9.118771399769,-25.9275682270146));
#48929=CARTESIAN_POINT('Ctrl Pts',(3.88499868405716,9.11964778216551,-25.9272416501901));
#48930=CARTESIAN_POINT('Ctrl Pts',(3.88702917018354,9.12008597336377,-25.9270783617778));
#48931=CARTESIAN_POINT('Ctrl Pts',(3.88897348599018,9.12050589219657,-25.9269218920397));
#48932=CARTESIAN_POINT('Ctrl Pts',(3.89083165147538,9.12090745887444,-25.9267722683545));
#48933=CARTESIAN_POINT('Ctrl Pts',(3.89176073421798,9.12110824221338,-25.9266974565119));
#48934=CARTESIAN_POINT('Ctrl Pts',(3.89266827938022,9.1213044375143,-25.9266243561845));
#48935=CARTESIAN_POINT('Ctrl Pts',(3.89355428929539,9.12149603549233,-25.9265529705566));
#48936=CARTESIAN_POINT('Ctrl Pts',(3.89399729425297,9.12159183448135,-25.9265172777426));
#48937=CARTESIAN_POINT('Ctrl Pts',(3.89443491538337,9.12168648420069,-25.9264820135827));
#48938=CARTESIAN_POINT('Ctrl Pts',(3.89486446310959,9.12177940075376,-25.926447395576));
#48939=CARTESIAN_POINT('Ctrl Pts',(3.89529401083581,9.12187231730682,-25.9264127775693));
#48940=CARTESIAN_POINT('Ctrl Pts',(3.89572088354979,9.12196459230373,-25.9263783968016));
#48941=CARTESIAN_POINT('Ctrl Pts',(3.89744543978842,9.12233787339604,-25.9262393301259));
#48942=CARTESIAN_POINT('Ctrl Pts',(3.90615289557581,9.12422260671741,-25.925537168664));
#48943=CARTESIAN_POINT('Ctrl Pts',(3.91484190872599,9.12610953954907,-25.9248343676433));
#48944=CARTESIAN_POINT('Ctrl Pts',(3.92351248770352,9.12799859659242,-25.9241309558179));
#48945=CARTESIAN_POINT('Ctrl Pts',(4.08352426246704,9.16286032507885,-25.9111497956376));
#48946=CARTESIAN_POINT('Ctrl Pts',(4.23725682874554,9.19844174260805,-25.8979626235783));
#48947=CARTESIAN_POINT('Ctrl Pts',(4.38477077120115,9.23429180559824,-25.884741517799));
#48948=CARTESIAN_POINT('Ctrl Pts',(4.40473563112835,9.2391438316106,-25.8829521443976));
#48949=CARTESIAN_POINT('Ctrl Pts',(4.42458659941958,9.24400084552466,-25.881162113865));
#48950=CARTESIAN_POINT('Ctrl Pts',(4.44432384241613,9.2488617915148,-25.8793718199261));
#48951=CARTESIAN_POINT('Ctrl Pts',(4.59308111662287,9.28549816852476,-25.8658785855147));
#48952=CARTESIAN_POINT('Ctrl Pts',(4.7353774875914,9.32235418178061,-25.8523724581803));
#48953=CARTESIAN_POINT('Ctrl Pts',(4.87128883464031,9.35900449074716,-25.839012128568));
#48954=CARTESIAN_POINT('Ctrl Pts',(4.89544337741269,9.36551808563659,-25.836637693614));
#48955=CARTESIAN_POINT('Ctrl Pts',(4.91939626929584,9.37202529808466,-25.834267800704));
#48956=CARTESIAN_POINT('Ctrl Pts',(4.94314796326917,9.37852388795739,-25.8319032604887));
#48957=CARTESIAN_POINT('Ctrl Pts',(5.07995159413634,9.41595408940341,-25.8182841187488));
#48958=CARTESIAN_POINT('Ctrl Pts',(5.21008001283661,9.45309456680969,-25.8048447024304));
#48959=CARTESIAN_POINT('Ctrl Pts',(5.33362132246346,9.48954685475107,-25.791729222239));
#48960=CARTESIAN_POINT('Ctrl Pts',(5.36980640846317,9.50022368161998,-25.787887715458));
#48961=CARTESIAN_POINT('Ctrl Pts',(5.40542642866001,9.51084176427358,-25.7840738287903));
#48962=CARTESIAN_POINT('Ctrl Pts',(5.44048367932467,9.52139181573028,-25.7802907760697));
#48963=CARTESIAN_POINT('Ctrl Pts',(5.56340767817423,9.55838429199524,-25.7670259603906));
#48964=CARTESIAN_POINT('Ctrl Pts',(5.67941229471595,9.59453689009802,-25.7541423866658));
#48965=CARTESIAN_POINT('Ctrl Pts',(5.78859480714337,9.62948272158884,-25.7417662950012));
#48966=CARTESIAN_POINT('Ctrl Pts',(5.8424005745087,9.6467042274672,-25.7356672861563));
#48967=CARTESIAN_POINT('Ctrl Pts',(5.89454960227653,9.66363335678642,-25.7296910961071));
#48968=CARTESIAN_POINT('Ctrl Pts',(5.94505368243246,9.68023019451297,-25.7238505128447));
#48969=CARTESIAN_POINT('Ctrl Pts',(5.95968231208978,9.68503750892865,-25.7221587736968));
#48970=CARTESIAN_POINT('Ctrl Pts',(5.97417293278927,9.68981696133266,-25.7204784027516));
#48971=CARTESIAN_POINT('Ctrl Pts',(5.98852581858903,9.69456763489497,-25.7188097024601));
#48972=CARTESIAN_POINT('Ctrl Pts',(-6.39567215510559,8.78352119285945,-25.5334667703321));
#48973=CARTESIAN_POINT('Ctrl Pts',(-6.35564925586518,8.77012419979114,-25.5378748134888));
#48974=CARTESIAN_POINT('Ctrl Pts',(-5.98524940728022,8.64740171180838,-25.5783537688208));
#48975=CARTESIAN_POINT('Ctrl Pts',(-5.25616631877878,8.42856364545493,-25.6522248402877));
#48976=CARTESIAN_POINT('Ctrl Pts',(-4.17576145259447,8.16491258504182,-25.7436218164382));
#48977=CARTESIAN_POINT('Ctrl Pts',(-3.01936948320032,7.95089104185876,-25.8195372431799));
#48978=CARTESIAN_POINT('Ctrl Pts',(-1.83578686325012,7.80507999288669,-25.8725333135281));
#48979=CARTESIAN_POINT('Ctrl Pts',(-0.697923544185256,7.73463099532804,
-25.8989854355906));
#48980=CARTESIAN_POINT('Ctrl Pts',(0.331409741547889,7.72744130935177,-25.90178757463));
#48981=CARTESIAN_POINT('Ctrl Pts',(1.24580985109183,7.76509280122674,-25.8874719190707));
#48982=CARTESIAN_POINT('Ctrl Pts',(2.07030115244264,7.83520333598814,-25.8615912407003));
#48983=CARTESIAN_POINT('Ctrl Pts',(2.81706942622759,7.92875537879263,-25.8276638258317));
#48984=CARTESIAN_POINT('Ctrl Pts',(3.49018596874702,8.03787927094033,-25.7886683317855));
#48985=CARTESIAN_POINT('Ctrl Pts',(4.09497305491957,8.15592276052121,-25.7470116842076));
#48986=CARTESIAN_POINT('Ctrl Pts',(4.65005393611137,8.2809286723435,-25.7034074146544));
#48987=CARTESIAN_POINT('Ctrl Pts',(5.18050287184726,8.41545116246433,-25.657033997868));
#48988=CARTESIAN_POINT('Ctrl Pts',(5.70542267267832,8.56333394897149,-25.6067231591697));
#48989=CARTESIAN_POINT('Ctrl Pts',(6.10978283777007,8.68890996549213,-25.5646822403335));
#48990=CARTESIAN_POINT('Ctrl Pts',(6.34031611218397,8.76499221874828,-25.5395631156537));
#48991=CARTESIAN_POINT('Ctrl Pts',(6.39541677132646,8.78343680508604,-25.5334956871243));
#48992=CARTESIAN_POINT('Ctrl Pts',(-6.33018795411181,9.06735642773491,-25.77671820803));
#48993=CARTESIAN_POINT('Ctrl Pts',(-6.29063921470765,9.05404079125888,-25.7811588809681));
#48994=CARTESIAN_POINT('Ctrl Pts',(-5.92460030554049,8.932053466397,-25.8219404051921));
#48995=CARTESIAN_POINT('Ctrl Pts',(-5.20363640342463,8.71436008085963,-25.8964088150044));
#48996=CARTESIAN_POINT('Ctrl Pts',(-4.13466319807682,8.45189348050018,-25.9886127972182));
#48997=CARTESIAN_POINT('Ctrl Pts',(-2.99013101605859,8.23872192023846,-26.0652383022213));
#48998=CARTESIAN_POINT('Ctrl Pts',(-1.81835018684379,8.09342931773288,-26.1187427457967));
#48999=CARTESIAN_POINT('Ctrl Pts',(-0.691526419404934,8.02320305496896,
-26.1454435066478));
#49000=CARTESIAN_POINT('Ctrl Pts',(0.328410955095827,8.01603333520191,-26.1482705905495));
#49001=CARTESIAN_POINT('Ctrl Pts',(1.23410624358473,8.0535706645095,-26.1338226905678));
#49002=CARTESIAN_POINT('Ctrl Pts',(2.05052545172647,8.12344568133579,-26.1076952637506));
#49003=CARTESIAN_POINT('Ctrl Pts',(2.78983578864226,8.21666094545048,-26.0734438046011));
#49004=CARTESIAN_POINT('Ctrl Pts',(3.45611831449841,8.3253655430678,-26.0340802931943));
#49005=CARTESIAN_POINT('Ctrl Pts',(4.05467056746315,8.4429263129846,-25.9920389686468));
#49006=CARTESIAN_POINT('Ctrl Pts',(4.60393606387575,8.5673882161268,-25.948043276697));
#49007=CARTESIAN_POINT('Ctrl Pts',(5.1287201730569,8.70128514681539,-25.9012677464719));
#49008=CARTESIAN_POINT('Ctrl Pts',(5.64789136107948,8.84842606812645,-25.8505389176693));
#49009=CARTESIAN_POINT('Ctrl Pts',(6.04766215292126,8.97331108817879,-25.8081672346917));
#49010=CARTESIAN_POINT('Ctrl Pts',(6.27548786339907,9.04894002582314,-25.7828596868889));
#49011=CARTESIAN_POINT('Ctrl Pts',(6.3299352734096,9.06727244757323,-25.7767473024571));
#49012=CARTESIAN_POINT('Ctrl Pts',(-6.21932913978971,9.42526200359147,-25.836655617584));
#49013=CARTESIAN_POINT('Ctrl Pts',(-6.18048424923994,9.41215947646683,-25.8411253051844));
#49014=CARTESIAN_POINT('Ctrl Pts',(-5.82094614614534,9.2921196376942,-25.882174891286));
#49015=CARTESIAN_POINT('Ctrl Pts',(-5.11256398435598,9.07782589043016,-25.9571561089932));
#49016=CARTESIAN_POINT('Ctrl Pts',(-4.06219748980148,8.81943183420526,-26.0500334124317));
#49017=CARTESIAN_POINT('Ctrl Pts',(-2.93773430956758,8.60957997072274,-26.1272375575012));
#49018=CARTESIAN_POINT('Ctrl Pts',(-1.7866100482536,8.46655698550872,-26.1811436018126));
#49019=CARTESIAN_POINT('Ctrl Pts',(-0.679627595369357,8.39741828659515,
-26.208029917519));
#49020=CARTESIAN_POINT('Ctrl Pts',(0.322792418129926,8.39035713706467,-26.2108741294564));
#49021=CARTESIAN_POINT('Ctrl Pts',(1.21265278059722,8.42731721331204,-26.1963301004562));
#49022=CARTESIAN_POINT('Ctrl Pts',(2.01469390800156,8.4961038334689,-26.17001268345));
#49023=CARTESIAN_POINT('Ctrl Pts',(2.74097574438404,8.58786425206803,-26.1355046756559));
#49024=CARTESIAN_POINT('Ctrl Pts',(3.39554807850959,8.69487403657257,-26.0958440499998));
#49025=CARTESIAN_POINT('Ctrl Pts',(3.98362077402804,8.81060581083193,-26.0534876926084));
#49026=CARTESIAN_POINT('Ctrl Pts',(4.52330256827803,8.93313438616758,-26.0091675497922));
#49027=CARTESIAN_POINT('Ctrl Pts',(5.0389473427338,9.06495108380986,-25.9620546712903));
#49028=CARTESIAN_POINT('Ctrl Pts',(5.549066646743,9.20979810657306,-25.9109701561731));
#49029=CARTESIAN_POINT('Ctrl Pts',(5.94181973557236,9.33271765448443,-25.8683114791919));
#49030=CARTESIAN_POINT('Ctrl Pts',(6.16560267800382,9.40714039589557,-25.8428372330143));
#49031=CARTESIAN_POINT('Ctrl Pts',(6.2190806635456,9.42517926284858,-25.8366848568002));
#49032=CARTESIAN_POINT('Ctrl Pts',(-6.0947810190966,9.75500160844674,-25.6963174977319));
#49033=CARTESIAN_POINT('Ctrl Pts',(-6.056668542277,9.7421829968728,-25.7008043046412));
#49034=CARTESIAN_POINT('Ctrl Pts',(-5.70391349769015,9.62474600415793,-25.7420109467264));
#49035=CARTESIAN_POINT('Ctrl Pts',(-5.00898011869918,9.41513447437917,-25.817274113052));
#49036=CARTESIAN_POINT('Ctrl Pts',(-3.97907763476271,9.16253604844767,-25.9104989403831));
#49037=CARTESIAN_POINT('Ctrl Pts',(-2.87715661780143,8.95752386402045,-25.9879852028307));
#49038=CARTESIAN_POINT('Ctrl Pts',(-1.74963938183232,8.81787230129108,-26.0420715124369));
#49039=CARTESIAN_POINT('Ctrl Pts',(-0.665628470734567,8.75037480882317,
-26.0690273778441));
#49040=CARTESIAN_POINT('Ctrl Pts',(0.316160263875782,8.74347976631618,-26.0718760176018));
#49041=CARTESIAN_POINT('Ctrl Pts',(1.18758201208621,8.77956467271151,-26.0572993887014));
#49042=CARTESIAN_POINT('Ctrl Pts',(1.97304891123421,8.8467214319318,-26.0309029323584));
#49043=CARTESIAN_POINT('Ctrl Pts',(2.68445564142065,8.93632518388317,-25.9962790566787));
#49044=CARTESIAN_POINT('Ctrl Pts',(3.32578864567077,9.04084951748645,-25.9564769830062));
#49045=CARTESIAN_POINT('Ctrl Pts',(3.90213225627446,9.15392926544206,-25.9139651165193));
#49046=CARTESIAN_POINT('Ctrl Pts',(4.4312010877471,9.27368825933768,-25.8694800648335));
#49047=CARTESIAN_POINT('Ctrl Pts',(4.93684397707394,9.40256510806607,-25.8221908574905));
#49048=CARTESIAN_POINT('Ctrl Pts',(5.4371949782222,9.54422233392443,-25.7709144512917));
#49049=CARTESIAN_POINT('Ctrl Pts',(5.82250744905633,9.66446408245599,-25.7280944465767));
#49050=CARTESIAN_POINT('Ctrl Pts',(6.04206764945495,9.7372727096129,-25.7025227985368));
#49051=CARTESIAN_POINT('Ctrl Pts',(6.09453704716581,9.75492058441964,-25.6963468075841));
#49052=CARTESIAN_POINT('',(6.27159454904661,8.76071457496506,-25.5608537658249));
#49053=CARTESIAN_POINT('Origin',(5.999999949022,9.3325096643222,-24.7867247244474));
#49054=CARTESIAN_POINT('Ctrl Pts',(-6.27159387327987,8.76070928018864,-25.5608571664728));
#49055=CARTESIAN_POINT('Ctrl Pts',(-6.13239664126094,8.71504798036057,-25.5759656499857));
#49056=CARTESIAN_POINT('Ctrl Pts',(-5.98564490954805,8.66855402099739,-25.5914802279663));
#49057=CARTESIAN_POINT('Ctrl Pts',(-5.8313286216121,8.62173959728843,-25.6072278247019));
#49058=CARTESIAN_POINT('Ctrl Pts',(-5.67907406993691,8.57555063571428,-25.6227650263352));
#49059=CARTESIAN_POINT('Ctrl Pts',(-5.51945544863095,8.52904985474282,-25.6385292465986));
#49060=CARTESIAN_POINT('Ctrl Pts',(-5.35247240281457,8.48276840590744,-25.654323233739));
#49061=CARTESIAN_POINT('Ctrl Pts',(-5.32566690280835,8.47533892484259,-25.6568586152223));
#49062=CARTESIAN_POINT('Ctrl Pts',(-5.29867165164591,8.46791517640557,-25.6593946946507));
#49063=CARTESIAN_POINT('Ctrl Pts',(-5.27148667846808,8.46049945000971,-25.6619305752687));
#49064=CARTESIAN_POINT('Ctrl Pts',(-5.14595415524353,8.42625572131715,-25.6736405552818));
#49065=CARTESIAN_POINT('Ctrl Pts',(-5.01637573562252,8.39218193845674,-25.6853469322197));
#49066=CARTESIAN_POINT('Ctrl Pts',(-4.88275739116987,8.35851824273555,-25.6969639519717));
#49067=CARTESIAN_POINT('Ctrl Pts',(-4.71106407780363,8.31526197068548,-25.711891278162));
#49068=CARTESIAN_POINT('Ctrl Pts',(-4.53269550838595,8.27268031541968,-25.726672510368));
#49069=CARTESIAN_POINT('Ctrl Pts',(-4.34764549623653,8.23131618000222,-25.7411115978377));
#49070=CARTESIAN_POINT('Ctrl Pts',(-4.29584052381524,8.21973624077584,-25.7451538376596));
#49071=CARTESIAN_POINT('Ctrl Pts',(-4.24351201014023,8.20825197500909,-25.7491691109346));
#49072=CARTESIAN_POINT('Ctrl Pts',(-4.1906600681287,8.19687588895432,-25.7531527551433));
#49073=CARTESIAN_POINT('Ctrl Pts',(-4.14338502789855,8.18670019993642,-25.7567160478637));
#49074=CARTESIAN_POINT('Ctrl Pts',(-4.09569119417892,8.176611068498,-25.7602540308525));
#49075=CARTESIAN_POINT('Ctrl Pts',(-4.04757899551552,8.16661761811045,-25.7637634419695));
#49076=CARTESIAN_POINT('Ctrl Pts',(-3.90056247756111,8.13608061670243,-25.7744871548081));
#49077=CARTESIAN_POINT('Ctrl Pts',(-3.74963597646617,8.10643537187603,-25.7849451006779));
#49078=CARTESIAN_POINT('Ctrl Pts',(-3.59479966784943,8.07795017664252,-25.7950405856412));
#49079=CARTESIAN_POINT('Ctrl Pts',(-3.51738151354106,8.06370757902576,-25.8000883281229));
#49080=CARTESIAN_POINT('Ctrl Pts',(-3.43898589874054,8.04975523833549,-25.8050453460868));
#49081=CARTESIAN_POINT('Ctrl Pts',(-3.35961279608689,8.03612821158824,-25.8098988461251));
#49082=CARTESIAN_POINT('Ctrl Pts',(-3.31992624476006,8.02931469821461,-25.8123255961442));
#49083=CARTESIAN_POINT('Ctrl Pts',(-3.27999531907876,8.02258252322768,-25.814726454219));
#49084=CARTESIAN_POINT('Ctrl Pts',(-3.23982001507201,8.0159361753693,-25.8170997778563));
#49085=CARTESIAN_POINT('Ctrl Pts',(-3.21973236306863,8.01261300144011,-25.8182864396749));
#49086=CARTESIAN_POINT('Ctrl Pts',(-3.1995836163341,8.00931128494159,-25.8194662170694));
#49087=CARTESIAN_POINT('Ctrl Pts',(-3.17937377388052,8.00603159219767,-25.8206389007071));
#49088=CARTESIAN_POINT('Ctrl Pts',(-3.16169016173364,8.00316186104674,-25.82166499889));
#49089=CARTESIAN_POINT('Ctrl Pts',(-3.14395977316815,8.00030899187142,-25.8226856658672));
#49090=CARTESIAN_POINT('Ctrl Pts',(-3.12618260742901,7.99747336662541,-25.823700759923));
#49091=CARTESIAN_POINT('Ctrl Pts',(-3.12364301232342,7.99706827730455,-25.8238457733596));
#49092=CARTESIAN_POINT('Ctrl Pts',(-3.11986203701007,7.9964661730716,-25.8240613381855));
#49093=CARTESIAN_POINT('Ctrl Pts',(-3.11856095820616,7.99625915556182,-25.8241354586248));
#49094=CARTESIAN_POINT('Ctrl Pts',(-3.0916130474862,7.99197141422406,-25.8256706392563));
#49095=CARTESIAN_POINT('Ctrl Pts',(-3.06343997656186,7.98754605048026,-25.8272572377435));
#49096=CARTESIAN_POINT('Ctrl Pts',(-3.03404177226685,7.98299895427487,-25.8288895746158));
#49097=CARTESIAN_POINT('Ctrl Pts',(-2.96197570914269,7.97185231011659,-25.8328910466411));
#49098=CARTESIAN_POINT('Ctrl Pts',(-2.88254755643339,7.95997076361514,-25.8371686199672));
#49099=CARTESIAN_POINT('Ctrl Pts',(-2.79575694848145,7.94762209438742,-25.8416264233191));
#49100=CARTESIAN_POINT('Ctrl Pts',(-2.70929659493284,7.93532041414254,-25.8460672639003));
#49101=CARTESIAN_POINT('Ctrl Pts',(-2.61552946386812,7.92255516446984,-25.850687011103));
#49102=CARTESIAN_POINT('Ctrl Pts',(-2.51445628760933,7.90963948626493,-25.8553726467872));
#49103=CARTESIAN_POINT('Ctrl Pts',(-2.50259531789646,7.90812382727726,-25.8559225076404));
#49104=CARTESIAN_POINT('Ctrl Pts',(-2.49063373971749,7.90660615169088,-25.85647325465));
#49105=CARTESIAN_POINT('Ctrl Pts',(-2.47857155780431,7.90508700946898,-25.8570246881376));
#49106=CARTESIAN_POINT('Ctrl Pts',(-2.37688575047032,7.89228043729151,-25.8616733462153));
#49107=CARTESIAN_POINT('Ctrl Pts',(-2.2680499546683,7.87936601812897,-25.8663725574763));
#49108=CARTESIAN_POINT('Ctrl Pts',(-2.15206296372362,7.86670052544834,-25.8709938979129));
#49109=CARTESIAN_POINT('Ctrl Pts',(-2.11969750004126,7.86316629682463,-25.8722834548265));
#49110=CARTESIAN_POINT('Ctrl Pts',(-2.08677525064872,7.85965173629575,-25.8735668334012));
#49111=CARTESIAN_POINT('Ctrl Pts',(-2.05329630949648,7.85616526106339,-25.8748409727839));
#49112=CARTESIAN_POINT('Ctrl Pts',(-1.976568178131,7.84817484319402,-25.8777610870577));
#49113=CARTESIAN_POINT('Ctrl Pts',(-1.89691556848977,7.8403313974129,-25.8806329572634));
#49114=CARTESIAN_POINT('Ctrl Pts',(-1.81433843535376,7.83274216582671,-25.8834176170251));
#49115=CARTESIAN_POINT('Ctrl Pts',(-1.81240162542855,7.83256416377575,-25.8834829299812));
#49116=CARTESIAN_POINT('Ctrl Pts',(-1.81046320669852,7.83238630180687,-25.8835481946928));
#49117=CARTESIAN_POINT('Ctrl Pts',(-1.80852317914455,7.83220858138765,-25.8836134106612));
#49118=CARTESIAN_POINT('Ctrl Pts',(-1.76910604729783,7.82859768978881,-25.8849384570088));
#49119=CARTESIAN_POINT('Ctrl Pts',(-1.7290247580196,7.82504520050363,-25.8862433971052));
#49120=CARTESIAN_POINT('Ctrl Pts',(-1.68827933459894,7.82156332561972,-25.8875239403802));
#49121=CARTESIAN_POINT('Ctrl Pts',(-1.66690392126586,7.81973670293257,-25.8881957248285));
#49122=CARTESIAN_POINT('Ctrl Pts',(-1.64534572750955,7.81792951796679,-25.8888607900245));
#49123=CARTESIAN_POINT('Ctrl Pts',(-1.62360475418917,7.81614356986812,-25.8895184929336));
#49124=CARTESIAN_POINT('Ctrl Pts',(-1.61273426752898,7.81525059581879,-25.8898473443881));
#49125=CARTESIAN_POINT('Ctrl Pts',(-1.60181808594281,7.81436293126474,-25.890174354927));
#49126=CARTESIAN_POINT('Ctrl Pts',(-1.59085620953321,7.81348080406847,-25.8904994431246));
#49127=CARTESIAN_POINT('Ctrl Pts',(-1.58537527132841,7.81303974047034,-25.8906619872234));
#49128=CARTESIAN_POINT('Ctrl Pts',(-1.57988290941558,7.81260006122919,-25.8908240507153));
#49129=CARTESIAN_POINT('Ctrl Pts',(-1.57437912380769,7.81216179501792,-25.8909856233591));
#49130=CARTESIAN_POINT('Ctrl Pts',(-1.56887533819979,7.81172352880665,-25.891147196003));
#49131=CARTESIAN_POINT('Ctrl Pts',(-1.562059610469,7.81118421530923,-25.8913460653726));
#49132=CARTESIAN_POINT('Ctrl Pts',(-1.55783349590704,7.81085126424264,-25.8914688584386));
#49133=CARTESIAN_POINT('Ctrl Pts',(-1.33210040385418,7.79306706254572,-25.8980277100902));
#49134=CARTESIAN_POINT('Ctrl Pts',(-1.11005394165783,7.77943811713524,-25.9030588902186));
#49135=CARTESIAN_POINT('Ctrl Pts',(-0.891697167770649,7.76958904750523,
-25.9066954197387));
#49136=CARTESIAN_POINT('Ctrl Pts',(-0.848420846838444,7.76763705173884,
-25.9074161467204));
#49137=CARTESIAN_POINT('Ctrl Pts',(-0.805289349939968,7.76583365319063,
-25.9080820794156));
#49138=CARTESIAN_POINT('Ctrl Pts',(-0.76230254880461,7.76417611307551,-25.908694233414));
#49139=CARTESIAN_POINT('Ctrl Pts',(-0.72471610697533,7.76272680692871,-25.9092294835382));
#49140=CARTESIAN_POINT('Ctrl Pts',(-0.687240273846953,7.76138898873381,
-25.9097235975349));
#49141=CARTESIAN_POINT('Ctrl Pts',(-0.649875247235843,7.76016076114611,
-25.9101771549314));
#49142=CARTESIAN_POINT('Ctrl Pts',(-0.558064354964064,7.75714284088841,
-25.911291606413));
#49143=CARTESIAN_POINT('Ctrl Pts',(-0.466922504495176,7.7547865017556,-25.9121612187759));
#49144=CARTESIAN_POINT('Ctrl Pts',(-0.37644893037311,7.75306363496773,-25.91279674608));
#49145=CARTESIAN_POINT('Ctrl Pts',(-0.312801759636325,7.75185161700925,
-25.9132438325937));
#49146=CARTESIAN_POINT('Ctrl Pts',(-0.249485476869291,7.75095306674767,
-25.9135750126042));
#49147=CARTESIAN_POINT('Ctrl Pts',(-0.186500082391666,7.7503583420325,-25.9137938241309));
#49148=CARTESIAN_POINT('Ctrl Pts',(-0.155007385152853,7.75006097967492,
-25.9139032298942));
#49149=CARTESIAN_POINT('Ctrl Pts',(-0.123597409863337,7.74983957563556,
-25.9139845411683));
#49150=CARTESIAN_POINT('Ctrl Pts',(-0.0922701561442512,7.74969293819765,
-25.9140381881211));
#49151=CARTESIAN_POINT('Ctrl Pts',(-0.0647193029049692,7.74956397743501,
-25.9140853681049));
#49152=CARTESIAN_POINT('Ctrl Pts',(-0.0383382266194984,7.74949397646208,
-25.9141107435945));
#49153=CARTESIAN_POINT('Ctrl Pts',(-0.0102094372121516,7.74947894116212,
-25.9141157541827));
#49154=CARTESIAN_POINT('Ctrl Pts',(-0.00635381891635554,7.74947688027082,
-25.9141164409849));
#49155=CARTESIAN_POINT('Ctrl Pts',(-0.00246536406951166,7.7494759265866,
-25.9141167169437));
#49156=CARTESIAN_POINT('Ctrl Pts',(0.00146344075487862,7.74947614256322,
-25.9141165581924));
#49157=CARTESIAN_POINT('Ctrl Pts',(0.123997928647954,7.7494828786027,-25.9141116069383));
#49158=CARTESIAN_POINT('Ctrl Pts',(0.246529019799171,7.75063927878568,-25.9136952103562));
#49159=CARTESIAN_POINT('Ctrl Pts',(0.369061817166272,7.75293711554216,-25.9128591305864));
#49160=CARTESIAN_POINT('Ctrl Pts',(0.644876546180536,7.75810942235248,-25.9109771600438));
#49161=CARTESIAN_POINT('Ctrl Pts',(0.920699733188535,7.76906181808629,-25.9069698715593));
#49162=CARTESIAN_POINT('Ctrl Pts',(1.19652079068848,7.78581224103914,-25.9008590747492));
#49163=CARTESIAN_POINT('Ctrl Pts',(1.22211852106872,7.78736677358422,-25.9002919587698));
#49164=CARTESIAN_POINT('Ctrl Pts',(1.24771623489009,7.78897127892905,-25.8997067137304));
#49165=CARTESIAN_POINT('Ctrl Pts',(1.27331392445554,7.79062579306484,-25.8991033499562));
#49166=CARTESIAN_POINT('Ctrl Pts',(1.37082860575515,7.79692868295047,-25.8968048289902));
#49167=CARTESIAN_POINT('Ctrl Pts',(1.4683429363519,7.80395726080187,-25.8942433811165));
#49168=CARTESIAN_POINT('Ctrl Pts',(1.56585686940457,7.81170938476352,-25.8914183109224));
#49169=CARTESIAN_POINT('Ctrl Pts',(1.74018067032872,7.82556770912729,-25.886367986741));
#49170=CARTESIAN_POINT('Ctrl Pts',(1.91450485622957,7.84173917716822,-25.8804762009628));
#49171=CARTESIAN_POINT('Ctrl Pts',(2.08882858930538,7.86022412687243,-25.873742229202));
#49172=CARTESIAN_POINT('Ctrl Pts',(2.17523695511336,7.86938670197223,-25.8704043503889));
#49173=CARTESIAN_POINT('Ctrl Pts',(2.26164519245099,7.87911781127896,-25.8668595119862));
#49174=CARTESIAN_POINT('Ctrl Pts',(2.34805359236325,7.88941699556036,-25.863107937955));
#49175=CARTESIAN_POINT('Ctrl Pts',(2.47841969325897,7.90495558322703,-25.8574478623238));
#49176=CARTESIAN_POINT('Ctrl Pts',(2.60878583328091,7.92178731770248,-25.8513174295213));
#49177=CARTESIAN_POINT('Ctrl Pts',(2.7391519851156,7.93991205128417,-25.844716566341));
#49178=CARTESIAN_POINT('Ctrl Pts',(2.77254675013872,7.94455490689162,-25.8430256805416));
#49179=CARTESIAN_POINT('Ctrl Pts',(2.80594152186298,7.94928260741816,-25.8413039117632));
#49180=CARTESIAN_POINT('Ctrl Pts',(2.83933628185507,7.95409517550948,-25.8395512547973));
#49181=CARTESIAN_POINT('Ctrl Pts',(2.87112458796028,7.95867623516301,-25.8378829093401));
#49182=CARTESIAN_POINT('Ctrl Pts',(2.90291288340858,7.96333419376135,-25.8361865759424));
#49183=CARTESIAN_POINT('Ctrl Pts',(2.93470118421066,7.96806902181925,-25.8344622611208));
#49184=CARTESIAN_POINT('Ctrl Pts',(2.98358847562793,7.97535072336469,-25.831810433906));
#49185=CARTESIAN_POINT('Ctrl Pts',(3.03247576357619,7.98281424499757,-25.8290924418474));
#49186=CARTESIAN_POINT('Ctrl Pts',(3.08136305395075,7.99045953986186,-25.8263083278156));
#49187=CARTESIAN_POINT('Ctrl Pts',(3.09765881740894,7.99300797148329,-25.825380289805));
#49188=CARTESIAN_POINT('Ctrl Pts',(3.11203760759698,7.99527206051231,-25.8245558041096));
#49189=CARTESIAN_POINT('Ctrl Pts',(3.13025034515279,7.99816542513299,-25.8235021733253));
#49190=CARTESIAN_POINT('Ctrl Pts',(3.2587731856329,8.01858319255843,-25.816066958229));
#49191=CARTESIAN_POINT('Ctrl Pts',(3.3858763678512,8.04008539286075,-25.8082999187491));
#49192=CARTESIAN_POINT('Ctrl Pts',(3.51154612819138,8.06258692776756,-25.8002309208586));
#49193=CARTESIAN_POINT('Ctrl Pts',(3.71380564174188,8.09880208002115,-25.7872442518004));
#49194=CARTESIAN_POINT('Ctrl Pts',(3.91235133347899,8.13760487958652,-25.7734759965143));
#49195=CARTESIAN_POINT('Ctrl Pts',(4.10714944139394,8.17864887428146,-25.7590478093978));
#49196=CARTESIAN_POINT('Ctrl Pts',(4.29250029058855,8.21770232994627,-25.7453193560622));
#49197=CARTESIAN_POINT('Ctrl Pts',(4.47445852097808,8.25878502137493,-25.7309933926776));
#49198=CARTESIAN_POINT('Ctrl Pts',(4.65301431239839,8.30161272215025,-25.7161706651186));
#49199=CARTESIAN_POINT('Ctrl Pts',(4.83065430932707,8.3442207640047,-25.7014239618215));
#49200=CARTESIAN_POINT('Ctrl Pts',(5.00492682819878,8.38855605849592,-25.6861856286938));
#49201=CARTESIAN_POINT('Ctrl Pts',(5.1758378275253,8.43435590184726,-25.670551811168));
#49202=CARTESIAN_POINT('Ctrl Pts',(5.35320999678042,8.48188717601207,-25.6543269681841));
#49203=CARTESIAN_POINT('Ctrl Pts',(5.52696176321428,8.53099591182413,-25.637676341178));
#49204=CARTESIAN_POINT('Ctrl Pts',(5.69711466993971,8.58141145046569,-25.62070496883));
#49205=CARTESIAN_POINT('Ctrl Pts',(5.87744654478025,8.63484297143877,-25.6027183269734));
#49206=CARTESIAN_POINT('Ctrl Pts',(6.05373611659351,8.68974251290063,-25.5843717510258));
#49207=CARTESIAN_POINT('Ctrl Pts',(6.226022223609,8.74581972929454,-25.5657891374643));
#49208=CARTESIAN_POINT('Ctrl Pts',(6.24124473246824,8.75077448704109,-25.5641472523206));
#49209=CARTESIAN_POINT('Ctrl Pts',(6.2564359933192,8.75573844668456,-25.5625035131198));
#49210=CARTESIAN_POINT('Ctrl Pts',(6.27159604047972,8.76071143370063,-25.5608580130011));
#49211=CARTESIAN_POINT('Origin',(5.999999999061,9.33250979146072,-24.7867247845918));
#49212=CARTESIAN_POINT('Origin',(5.99996968669111,9.33251391750253,-24.7866936478717));
#49213=CARTESIAN_POINT('Ctrl Pts',(6.25392027494701,3.90298732745545,-15.8231684029013));
#49214=CARTESIAN_POINT('Ctrl Pts',(6.30498637037455,3.91655122781545,-15.8051570120035));
#49215=CARTESIAN_POINT('Ctrl Pts',(6.44770248625324,3.96600398299862,-15.7512014975234));
#49216=CARTESIAN_POINT('Ctrl Pts',(6.66633061405961,4.09807443964668,-15.6507405657398));
#49217=CARTESIAN_POINT('Ctrl Pts',(6.88010573794568,4.32343154619026,-15.5214493319802));
#49218=CARTESIAN_POINT('Ctrl Pts',(7.03309503798963,4.607315341482,-15.3885588610201));
#49219=CARTESIAN_POINT('Ctrl Pts',(7.09634443075797,4.87218675594795,-15.2845094186338));
#49220=CARTESIAN_POINT('Ctrl Pts',(7.10389711961593,5.03409215205006,-15.228651260299));
#49221=CARTESIAN_POINT('Ctrl Pts',(7.10327724980352,5.08536189847456,-15.2117263055378));
#49222=CARTESIAN_POINT('Ctrl Pts',(6.05652411355051,3.85906155699697,-15.2125089076995));
#49223=CARTESIAN_POINT('Ctrl Pts',(6.10187709936855,3.87077510290403,-15.1964773801162));
#49224=CARTESIAN_POINT('Ctrl Pts',(6.22889159885922,3.91360449797959,-15.1483525761357));
#49225=CARTESIAN_POINT('Ctrl Pts',(6.42453376431358,4.02884063488479,-15.0583089083087));
#49226=CARTESIAN_POINT('Ctrl Pts',(6.61687258416338,4.22699772610696,-14.9420678245189));
#49227=CARTESIAN_POINT('Ctrl Pts',(6.75502557493823,4.47794845855267,-14.8226484218656));
#49228=CARTESIAN_POINT('Ctrl Pts',(6.8121853548424,4.71267003637461,-14.7296123730615));
#49229=CARTESIAN_POINT('Ctrl Pts',(6.81897933253834,4.85592976215469,-14.6800904100871));
#49230=CARTESIAN_POINT('Ctrl Pts',(6.81842108595897,4.90123798330861,-14.6651416079335));
#49231=CARTESIAN_POINT('Ctrl Pts',(6.04728643245338,3.3642601016969,-14.8018988955162));
#49232=CARTESIAN_POINT('Ctrl Pts',(6.1096864082144,3.38027488763903,-14.780301688516));
#49233=CARTESIAN_POINT('Ctrl Pts',(6.28323634553052,3.43850801268331,-14.7160886442661));
#49234=CARTESIAN_POINT('Ctrl Pts',(6.54570992416607,3.59232396077953,-14.5987447339918));
#49235=CARTESIAN_POINT('Ctrl Pts',(6.79905716620728,3.8511821076201,-14.4503513769499));
#49236=CARTESIAN_POINT('Ctrl Pts',(6.97876410714886,4.17408834693898,-14.2994899754014));
#49237=CARTESIAN_POINT('Ctrl Pts',(7.05291929263889,4.47422356328171,-14.1817471419756));
#49238=CARTESIAN_POINT('Ctrl Pts',(7.06187440122695,4.65851681165845,-14.1181749926599));
#49239=CARTESIAN_POINT('Ctrl Pts',(7.06114148281948,4.71705880021148,-14.098847828217));
#49240=CARTESIAN_POINT('Ctrl Pts',(6.23212119064543,2.7520459899376,-14.8671517492495));
#49241=CARTESIAN_POINT('Ctrl Pts',(6.32282827124314,2.77561132425719,-14.8361981369132));
#49242=CARTESIAN_POINT('Ctrl Pts',(6.5737574938549,2.86088152010372,-14.744831804744));
#49243=CARTESIAN_POINT('Ctrl Pts',(6.94779412332067,3.08265908688098,-14.5808890356009));
#49244=CARTESIAN_POINT('Ctrl Pts',(7.30343635770547,3.44915925509986,-14.3768346722789));
#49245=CARTESIAN_POINT('Ctrl Pts',(7.55305356317214,3.90035404771087,-14.1708337848037));
#49246=CARTESIAN_POINT('Ctrl Pts',(7.65582336285289,4.31732496808673,-14.0093356417527));
#49247=CARTESIAN_POINT('Ctrl Pts',(7.66840148009804,4.57464175472762,-13.920807830227));
#49248=CARTESIAN_POINT('Ctrl Pts',(7.66737543417775,4.65668281802034,-13.8937022602362));
#49249=CARTESIAN_POINT('',(6.99999200753597,4.92968844883675,-14.7967977305573));
#49250=CARTESIAN_POINT('',(7.00000029677448,3.16613090165484,-14.5427412926877));
#49251=CARTESIAN_POINT('Ctrl Pts',(7.,4.92968844926947,-14.7967977304731));
#49252=CARTESIAN_POINT('Ctrl Pts',(7.,4.82769576894919,-14.7564330540733));
#49253=CARTESIAN_POINT('Ctrl Pts',(7.,4.7350293213622,-14.7220626972232));
#49254=CARTESIAN_POINT('Ctrl Pts',(7.,4.65323746896003,-14.6940819631314));
#49255=CARTESIAN_POINT('Ctrl Pts',(7.,4.61234154275894,-14.6800915960855));
#49256=CARTESIAN_POINT('Ctrl Pts',(7.,4.57417008110355,-14.6676560278867));
#49257=CARTESIAN_POINT('Ctrl Pts',(7.,4.53894527480209,-14.6566252007483));
#49258=CARTESIAN_POINT('Ctrl Pts',(7.,4.52133287165136,-14.6511097871791));
#49259=CARTESIAN_POINT('Ctrl Pts',(7.,4.50445726238892,-14.6459439846359));
#49260=CARTESIAN_POINT('Ctrl Pts',(7.,4.4883456810344,-14.6411019035005));
#49261=CARTESIAN_POINT('Ctrl Pts',(7.,4.48028989035715,-14.6386808629328));
#49262=CARTESIAN_POINT('Ctrl Pts',(7.,4.47242510665687,-14.6363407527171));
#49263=CARTESIAN_POINT('Ctrl Pts',(7.,4.46475458846243,-14.6340780114449));
#49264=CARTESIAN_POINT('Ctrl Pts',(7.,4.46091932936521,-14.6329466408089));
#49265=CARTESIAN_POINT('Ctrl Pts',(7.,4.45713263664445,-14.6318346124087));
#49266=CARTESIAN_POINT('Ctrl Pts',(7.,4.45339490911939,-14.6307414807438));
#49267=CARTESIAN_POINT('Ctrl Pts',(7.,4.44965718159433,-14.6296483490789));
#49268=CARTESIAN_POINT('Ctrl Pts',(7.,4.44750552652622,-14.6290200289085));
#49269=CARTESIAN_POINT('Ctrl Pts',(7.,4.44232901759576,-14.6275183273043));
#49270=CARTESIAN_POINT('Ctrl Pts',(7.,4.35950487470844,-14.6034911016374));
#49271=CARTESIAN_POINT('Ctrl Pts',(7.,4.27923941186931,-14.5829868342322));
#49272=CARTESIAN_POINT('Ctrl Pts',(7.,4.20215931213699,-14.5660822358387));
#49273=CARTESIAN_POINT('Ctrl Pts',(7.,4.12507921240467,-14.5491776374452));
#49274=CARTESIAN_POINT('Ctrl Pts',(7.,4.05278013298332,-14.5360945759712));
#49275=CARTESIAN_POINT('Ctrl Pts',(7.,3.98127020879684,-14.5256226924827));
#49276=CARTESIAN_POINT('Ctrl Pts',(7.,3.83825036042388,-14.5046789255058));
#49277=CARTESIAN_POINT('Ctrl Pts',(7.,3.69577797679041,-14.4945086567194));
#49278=CARTESIAN_POINT('Ctrl Pts',(7.,3.55815928031856,-14.4973986345922));
#49279=CARTESIAN_POINT('Ctrl Pts',(7.,3.42054058384671,-14.5002886124651));
#49280=CARTESIAN_POINT('Ctrl Pts',(7.,3.28800110200234,-14.5162068700801));
#49281=CARTESIAN_POINT('Ctrl Pts',(7.,3.16613170174698,-14.5427408959923));
#49282=CARTESIAN_POINT('',(6.24994411785848,2.76546207136057,-14.8593862266086));
#49283=CARTESIAN_POINT('Ctrl Pts',(6.24994455730984,2.7654623494508,-14.8593877207787));
#49284=CARTESIAN_POINT('Ctrl Pts',(6.29979781833251,2.77899594289883,-14.8422062667216));
#49285=CARTESIAN_POINT('Ctrl Pts',(6.34863096323173,2.7944176673382,-14.8247566362977));
#49286=CARTESIAN_POINT('Ctrl Pts',(6.39646857396924,2.81164057419167,-14.8070481760307));
#49287=CARTESIAN_POINT('Ctrl Pts',(6.42911332404107,2.82339361706054,-14.7949637878126));
#49288=CARTESIAN_POINT('Ctrl Pts',(6.46129434933223,2.83598654928082,-14.7827585948818));
#49289=CARTESIAN_POINT('Ctrl Pts',(6.49301580980901,2.84940483943542,-14.7704328360015));
#49290=CARTESIAN_POINT('Ctrl Pts',(6.54021855514441,2.8693717679275,-14.7520916357937));
#49291=CARTESIAN_POINT('Ctrl Pts',(6.58640506262817,2.89116430239203,-14.7334837053198));
#49292=CARTESIAN_POINT('Ctrl Pts',(6.63160836973239,2.91475048338072,-14.7145978869442));
#49293=CARTESIAN_POINT('Ctrl Pts',(6.63723860889029,2.91768822949478,-14.7122455883856));
#49294=CARTESIAN_POINT('Ctrl Pts',(6.64285356156666,2.92065385816639,-14.7098889707024));
#49295=CARTESIAN_POINT('Ctrl Pts',(6.64845326188242,2.92364735500386,-14.7075280059086));
#49296=CARTESIAN_POINT('Ctrl Pts',(6.69418400793763,2.94809417107832,-14.6882468523933));
#49297=CARTESIAN_POINT('Ctrl Pts',(6.73887860241311,2.9743951866194,-14.6686831423798));
#49298=CARTESIAN_POINT('Ctrl Pts',(6.7825302865664,3.00255784800113,-14.648823534793));
#49299=CARTESIAN_POINT('Ctrl Pts',(6.82571493102099,3.03041919040419,-14.6291764098476));
#49300=CARTESIAN_POINT('Ctrl Pts',(6.86787933734953,3.06010299316823,-14.609239479601));
#49301=CARTESIAN_POINT('Ctrl Pts',(6.90897979149492,3.09165114058264,-14.5889981419846));
#49302=CARTESIAN_POINT('Ctrl Pts',(6.91447876829732,3.09587208009287,-14.5862899810089));
#49303=CARTESIAN_POINT('Ctrl Pts',(6.91995863828218,3.10012643844517,-14.5835763710984));
#49304=CARTESIAN_POINT('Ctrl Pts',(6.92541923818674,3.10441435723096,-14.5808572780706));
#49305=CARTESIAN_POINT('Ctrl Pts',(6.95069604285227,3.12426288806353,-14.5682707519501));
#49306=CARTESIAN_POINT('Ctrl Pts',(6.97556046737544,3.14483022611502,-14.5555667144424));
#49307=CARTESIAN_POINT('Ctrl Pts',(7.00000088934497,3.16612989450563,-14.5427407493156));
#49308=CARTESIAN_POINT('',(6.26385789024229,3.90573692077446,-15.8144409741972));
#49309=CARTESIAN_POINT('Origin',(6.52774091094718,2.94125499125657,-15.8038022189583));
#49310=CARTESIAN_POINT('Ctrl Pts',(6.26385527955666,3.90574646326258,-15.8144410794374));
#49311=CARTESIAN_POINT('Ctrl Pts',(6.30677501622484,3.91779325316633,-15.7868226401676));
#49312=CARTESIAN_POINT('Ctrl Pts',(6.34923257297403,3.93289027417838,-15.75778635456));
#49313=CARTESIAN_POINT('Ctrl Pts',(6.3907785074684,3.95108686753143,-15.7274032517978));
#49314=CARTESIAN_POINT('Ctrl Pts',(6.43558717779547,3.97071249787424,-15.6946340662746));
#49315=CARTESIAN_POINT('Ctrl Pts',(6.47933557617439,3.99394464936472,-15.6602976444418));
#49316=CARTESIAN_POINT('Ctrl Pts',(6.52150122927541,4.02069411945903,-15.6245203039367));
#49317=CARTESIAN_POINT('Ctrl Pts',(6.53207018575043,4.02739896011403,-15.6155525985466));
#49318=CARTESIAN_POINT('Ctrl Pts',(6.54253947197269,4.03432477240376,-15.60649446611));
#49319=CARTESIAN_POINT('Ctrl Pts',(6.5529003759936,4.04147015600223,-15.5973481025264));
#49320=CARTESIAN_POINT('Ctrl Pts',(6.57464090466716,4.05646348252013,-15.5781560726277));
#49321=CARTESIAN_POINT('Ctrl Pts',(6.59590457157523,4.07242355443942,-15.5585754483081));
#49322=CARTESIAN_POINT('Ctrl Pts',(6.61660777073193,4.08933791168146,-15.5386277503673));
#49323=CARTESIAN_POINT('Ctrl Pts',(6.63876804721789,4.10744269008932,-15.5172761467683));
#49324=CARTESIAN_POINT('Ctrl Pts',(6.66028617076777,4.12664091652856,-15.4955039354844));
#49325=CARTESIAN_POINT('Ctrl Pts',(6.68107533790851,4.14689256153848,-15.4733417200545));
#49326=CARTESIAN_POINT('Ctrl Pts',(6.70118104281552,4.16647841582952,-15.4519081070337));
#49327=CARTESIAN_POINT('Ctrl Pts',(6.72060496323911,4.18704952161287,-15.4301097156608));
#49328=CARTESIAN_POINT('Ctrl Pts',(6.73926365585971,4.20856966843344,-15.4079765811578));
#49329=CARTESIAN_POINT('Ctrl Pts',(6.74859300217001,4.21932974184372,-15.3969100139063));
#49330=CARTESIAN_POINT('Ctrl Pts',(6.75773099346059,4.23032711811503,-15.3857597628736));
#49331=CARTESIAN_POINT('Ctrl Pts',(6.76666663238851,4.24155727259564,-15.3745298510729));
#49332=CARTESIAN_POINT('Ctrl Pts',(6.77113445185248,4.24717234983594,-15.3689148951726));
#49333=CARTESIAN_POINT('Ctrl Pts',(6.77555167975256,4.25284562488489,-15.3632800242269));
#49334=CARTESIAN_POINT('Ctrl Pts',(6.77991691030056,4.25857654281244,-15.3576257506515));
#49335=CARTESIAN_POINT('Ctrl Pts',(6.7826528047095,4.26216837745751,-15.3540819526112));
#49336=CARTESIAN_POINT('Ctrl Pts',(6.78569591686906,4.26622078384239,-15.3501001756321));
#49337=CARTESIAN_POINT('Ctrl Pts',(6.78842750025002,4.26991217685713,-15.3464895428362));
#49338=CARTESIAN_POINT('Ctrl Pts',(6.79005426899699,4.27211055118867,-15.3443392644922));
#49339=CARTESIAN_POINT('Ctrl Pts',(6.79157148607674,4.27418008599266,-15.3423206972513));
#49340=CARTESIAN_POINT('Ctrl Pts',(6.79285518238893,4.27594167920464,-15.3406052397862));
#49341=CARTESIAN_POINT('Ctrl Pts',(6.79521152840393,4.27917525018686,-15.3374563553317));
#49342=CARTESIAN_POINT('Ctrl Pts',(6.79756024076484,4.28243827572785,-15.3342895371218));
#49343=CARTESIAN_POINT('Ctrl Pts',(6.79990066491025,4.28573099267086,-15.3311048460252));
#49344=CARTESIAN_POINT('Ctrl Pts',(6.81783379914537,4.31096092163608,-15.3067026482244));
#49345=CARTESIAN_POINT('Ctrl Pts',(6.83528346595841,4.33793603225933,-15.2812494305542));
#49346=CARTESIAN_POINT('Ctrl Pts',(6.85196339539571,4.3667222959665,-15.2547860263646));
#49347=CARTESIAN_POINT('Ctrl Pts',(6.86776035936218,4.39398473566812,-15.2297234837451));
#49348=CARTESIAN_POINT('Ctrl Pts',(6.88286710000684,4.42287156068814,-15.2037548229464));
#49349=CARTESIAN_POINT('Ctrl Pts',(6.89700434437673,4.45341835639927,-15.176933537494));
#49350=CARTESIAN_POINT('Ctrl Pts',(6.90834830381464,4.47792961208946,-15.1554116930466));
#49351=CARTESIAN_POINT('Ctrl Pts',(6.91906750511668,4.50350931159876,-15.13334116626));
#49352=CARTESIAN_POINT('Ctrl Pts',(6.92899766648264,4.53016601726516,-15.1107595934415));
#49353=CARTESIAN_POINT('Ctrl Pts',(6.93174472990178,4.53754028423948,-15.1045126644793));
#49354=CARTESIAN_POINT('Ctrl Pts',(6.93443128870946,4.5449969226956,-15.0982266823882));
#49355=CARTESIAN_POINT('Ctrl Pts',(6.93705415527578,4.55253553000811,-15.0919026372694));
#49356=CARTESIAN_POINT('Ctrl Pts',(6.94825805191974,4.58473761693595,-15.0648887019085));
#49357=CARTESIAN_POINT('Ctrl Pts',(6.95830252975268,4.61843781676003,-15.0371784024747));
#49358=CARTESIAN_POINT('Ctrl Pts',(6.96691898512431,4.6535869298058,-15.0088629431602));
#49359=CARTESIAN_POINT('Ctrl Pts',(6.97510443426528,4.68697783880229,-14.9819638597059));
#49360=CARTESIAN_POINT('Ctrl Pts',(6.9820014634844,4.72167619755401,-14.9545186209884));
#49361=CARTESIAN_POINT('Ctrl Pts',(6.98734637694117,4.75761495687658,-14.9266266850321));
#49362=CARTESIAN_POINT('Ctrl Pts',(6.98981427690794,4.77420891366478,-14.9137481775732));
#49363=CARTESIAN_POINT('Ctrl Pts',(6.99195076731028,4.79106696982164,-14.9007747454111));
#49364=CARTESIAN_POINT('Ctrl Pts',(6.99372697726635,4.80818070467899,-14.8877178592447));
#49365=CARTESIAN_POINT('Ctrl Pts',(6.99740919774112,4.84365879930168,-14.8606499254039));
#49366=CARTESIAN_POINT('Ctrl Pts',(6.99954480901166,4.8802379977655,-14.8332216625081));
#49367=CARTESIAN_POINT('Ctrl Pts',(6.99991734819238,4.91777656577306,-14.8055596995045));
#49368=CARTESIAN_POINT('Ctrl Pts',(6.99995664834309,4.92173660932317,-14.8026415653297));
#49369=CARTESIAN_POINT('Ctrl Pts',(6.99997629845513,4.92570729933136,-14.799720853908));
#49370=CARTESIAN_POINT('Ctrl Pts',(6.99997602260847,4.92968844797978,-14.7967977308986));
#49371=CARTESIAN_POINT('Ctrl Pts',(6.99990207659395,4.95612342846035,-14.684705142693));
#49372=CARTESIAN_POINT('Ctrl Pts',(6.99990207659395,4.91843322561129,-15.0109955237193));
#49373=CARTESIAN_POINT('Ctrl Pts',(6.99990207659395,4.8561621330926,-15.8988757775478));
#49374=CARTESIAN_POINT('Ctrl Pts',(6.99990207659395,4.93000355594309,-17.3517252626563));
#49375=CARTESIAN_POINT('Ctrl Pts',(6.99990207659395,5.27370128699297,-19.0057031767965));
#49376=CARTESIAN_POINT('Ctrl Pts',(6.99990207659395,5.86661420603441,-20.5902607600442));
#49377=CARTESIAN_POINT('Ctrl Pts',(6.99990207659395,6.69609459969272,-22.0651325913196));
#49378=CARTESIAN_POINT('Ctrl Pts',(6.99990207659395,7.73957894060174,-23.3944692108351));
#49379=CARTESIAN_POINT('Ctrl Pts',(6.99990207659395,8.69530687990185,-24.2870452318747));
#49380=CARTESIAN_POINT('Ctrl Pts',(6.99990207659395,9.28612124925631,-24.7366401017851));
#49381=CARTESIAN_POINT('Ctrl Pts',(6.99990207659395,9.4330871100264,-24.8428478912403));
#49382=CARTESIAN_POINT('Ctrl Pts',(7.00660364663921,4.48044941032924,-14.629744314853));
#49383=CARTESIAN_POINT('Ctrl Pts',(7.00660364663921,4.44110729653057,-14.970322314067));
#49384=CARTESIAN_POINT('Ctrl Pts',(7.00660364663921,4.37614027536931,-15.8968427125844));
#49385=CARTESIAN_POINT('Ctrl Pts',(7.00660364663921,4.45318215224793,-17.4128418304199));
#49386=CARTESIAN_POINT('Ctrl Pts',(7.00660364663921,4.81191599524873,-19.1393493860805));
#49387=CARTESIAN_POINT('Ctrl Pts',(7.00660364663921,5.4307158401717,-20.792933289964));
#49388=CARTESIAN_POINT('Ctrl Pts',(7.00660364663921,6.29626827380092,-22.332051081099));
#49389=CARTESIAN_POINT('Ctrl Pts',(7.00660364663921,7.38553208571995,-23.7196527338312));
#49390=CARTESIAN_POINT('Ctrl Pts',(7.00660364663921,8.38275194446837,-24.650964724442));
#49391=CARTESIAN_POINT('Ctrl Pts',(7.00660364663921,8.99924836318557,-25.1201131729878));
#49392=CARTESIAN_POINT('Ctrl Pts',(7.00660364663921,9.1526167444896,-25.2309488097062));
#49393=CARTESIAN_POINT('Ctrl Pts',(6.71667356571233,4.1017052012643,-14.5859830529861));
#49394=CARTESIAN_POINT('Ctrl Pts',(6.71667356571233,4.06104779236811,-14.9379372309449));
#49395=CARTESIAN_POINT('Ctrl Pts',(6.71667356571233,3.99393420165435,-15.8952239325906));
#49396=CARTESIAN_POINT('Ctrl Pts',(6.71667356571233,4.07352436451027,-17.4615044548973));
#49397=CARTESIAN_POINT('Ctrl Pts',(6.71667356571233,4.44423035673658,-19.2457620256132));
#49398=CARTESIAN_POINT('Ctrl Pts',(6.71667356571233,5.08364205535591,-20.9543065080017));
#49399=CARTESIAN_POINT('Ctrl Pts',(6.71667356571233,5.97791599936316,-22.5445786282065));
#49400=CARTESIAN_POINT('Ctrl Pts',(6.71667356571233,7.10363063448991,-23.9785724383432));
#49401=CARTESIAN_POINT('Ctrl Pts',(6.71667356571233,8.13388745471671,-24.940727030391));
#49402=CARTESIAN_POINT('Ctrl Pts',(6.71667356571233,8.77083259903691,-25.4254445543805));
#49403=CARTESIAN_POINT('Ctrl Pts',(6.71667356571233,8.92929883618842,-25.5399650052432));
#49404=CARTESIAN_POINT('Ctrl Pts',(6.25321309030958,3.98119853671877,-14.5720593451688));
#49405=CARTESIAN_POINT('Ctrl Pts',(6.25321309030958,3.94012263475573,-14.9276331305612));
#49406=CARTESIAN_POINT('Ctrl Pts',(6.25321309030958,3.87232606083332,-15.8947088784425));
#49407=CARTESIAN_POINT('Ctrl Pts',(6.25321309030958,3.95272702273434,-17.4769876502149));
#49408=CARTESIAN_POINT('Ctrl Pts',(6.25321309030958,4.32724224487352,-19.2796197901663));
#49409=CARTESIAN_POINT('Ctrl Pts',(6.25321309030958,4.97321210511988,-21.0056513148311));
#49410=CARTESIAN_POINT('Ctrl Pts',(6.25321309030958,5.87662449490167,-22.6121994266604));
#49411=CARTESIAN_POINT('Ctrl Pts',(6.25321309030958,7.01393684431548,-24.0609540278942));
#49412=CARTESIAN_POINT('Ctrl Pts',(6.25321309030958,8.05470517584552,-25.0329219423298));
#49413=CARTESIAN_POINT('Ctrl Pts',(6.25321309030958,8.69815657863172,-25.5225931456291));
#49414=CARTESIAN_POINT('Ctrl Pts',(6.25321309030958,8.85824482237706,-25.6382860095647));
#49415=CARTESIAN_POINT('Ctrl Pts',(6.99999999999946,4.92968844925125,-14.7967977306008));
#49416=CARTESIAN_POINT('Ctrl Pts',(6.99999999999946,4.91233123517191,-14.9621835172955));
#49417=CARTESIAN_POINT('Ctrl Pts',(6.99999999997464,4.89876479509306,-15.1274620360007));
#49418=CARTESIAN_POINT('Ctrl Pts',(6.9999999993832,4.88893183450758,-15.2927163168167));
#49419=CARTESIAN_POINT('Ctrl Pts',(6.99999999893632,4.88150212010356,-15.4175812646452));
#49420=CARTESIAN_POINT('Ctrl Pts',(6.99999999820117,4.87620500438501,-15.5424326368658));
#49421=CARTESIAN_POINT('Ctrl Pts',(6.99999999795816,4.87303542048088,-15.6673078032506));
#49422=CARTESIAN_POINT('Ctrl Pts',(6.99999999763562,4.8688284502018,-15.8330538852174));
#49423=CARTESIAN_POINT('Ctrl Pts',(6.99999999919455,4.86836771463358,-15.9988422474281));
#49424=CARTESIAN_POINT('Ctrl Pts',(6.99999999987624,4.87168823513293,-16.1647921805699));
#49425=CARTESIAN_POINT('Ctrl Pts',(6.99999999995189,4.87205668724803,-16.183206343012));
#49426=CARTESIAN_POINT('Ctrl Pts',(6.99999999999964,4.87247174903354,-16.2016224895237));
#49427=CARTESIAN_POINT('Ctrl Pts',(6.99999999999964,4.87293350770597,-16.2200407785058));
#49428=CARTESIAN_POINT('Ctrl Pts',(6.99999999999964,4.87803551097676,-16.4235457178609));
#49429=CARTESIAN_POINT('Ctrl Pts',(6.99999999555513,4.88875796900593,-16.6272930258414));
#49430=CARTESIAN_POINT('Ctrl Pts',(6.99999999493485,4.90514631566278,-16.8307386153249));
#49431=CARTESIAN_POINT('Ctrl Pts',(6.99999999440965,4.91902260107297,-17.0029993762319));
#49432=CARTESIAN_POINT('Ctrl Pts',(6.99999999611632,4.93696006359404,-17.1750435554702));
#49433=CARTESIAN_POINT('Ctrl Pts',(6.99999999794794,4.95895705184918,-17.3465408121815));
#49434=CARTESIAN_POINT('Ctrl Pts',(6.99999999900192,4.97161496384682,-17.4452269213029));
#49435=CARTESIAN_POINT('Ctrl Pts',(6.99999999999964,4.98561660497,-17.5437319472142));
#49436=CARTESIAN_POINT('Ctrl Pts',(6.99999999999964,5.00094770326887,-17.6419939642891));
#49437=CARTESIAN_POINT('Ctrl Pts',(6.99999999999964,5.04134916509787,-17.9009401307474));
#49438=CARTESIAN_POINT('Ctrl Pts',(6.99999999748067,5.09107364972735,-18.1581948885142));
#49439=CARTESIAN_POINT('Ctrl Pts',(6.9999999983993,5.14990920187463,-18.4132918257843));
#49440=CARTESIAN_POINT('Ctrl Pts',(6.99999999910474,5.19509078503942,-18.6091884064351));
#49441=CARTESIAN_POINT('Ctrl Pts',(6.99999999994352,5.24564636503982,-18.803812805501));
#49442=CARTESIAN_POINT('Ctrl Pts',(6.99999999999482,5.30150075775557,-18.9969552607985));
#49443=CARTESIAN_POINT('Ctrl Pts',(6.99999999999814,5.30512332812396,-19.0094819771662));
#49444=CARTESIAN_POINT('Ctrl Pts',(6.99999999999964,5.30876819415222,-19.0220024596165));
#49445=CARTESIAN_POINT('Ctrl Pts',(6.99999999999964,5.3124353329409,-19.0345166513395));
#49446=CARTESIAN_POINT('Ctrl Pts',(6.99999999999964,5.41320704222893,-19.3784023243266));
#49447=CARTESIAN_POINT('Ctrl Pts',(7.0000000000075,5.53077138717327,-19.7175348267532));
#49448=CARTESIAN_POINT('Ctrl Pts',(6.99999999997804,5.66466508951816,-20.0501490251692));
#49449=CARTESIAN_POINT('Ctrl Pts',(6.99999999996837,5.7085987338504,-20.1592874957406));
#49450=CARTESIAN_POINT('Ctrl Pts',(6.99999999999964,5.7542901016912,-20.2677239882539));
#49451=CARTESIAN_POINT('Ctrl Pts',(6.99999999999964,5.80172169984713,-20.3753956739967));
#49452=CARTESIAN_POINT('Ctrl Pts',(6.99999999999964,5.83157383362071,-20.4431612499289));
#49453=CARTESIAN_POINT('Ctrl Pts',(6.99999999997177,5.86211302945351,-20.5106252086442));
#49454=CARTESIAN_POINT('Ctrl Pts',(6.99999999993234,5.89333412587516,-20.577772371119));
#49455=CARTESIAN_POINT('Ctrl Pts',(6.99999999971818,6.06290292235333,-20.9424637123202));
#49456=CARTESIAN_POINT('Ctrl Pts',(6.99999999999964,6.25259012480563,-21.2978070675131));
#49457=CARTESIAN_POINT('Ctrl Pts',(6.99999999999964,6.46101007423756,-21.6416318480036));
#49458=CARTESIAN_POINT('Ctrl Pts',(6.99999999999964,6.5445514342191,-21.7794477808633));
#49459=CARTESIAN_POINT('Ctrl Pts',(6.99999999962317,6.63110403210437,-21.9154125925419));
#49460=CARTESIAN_POINT('Ctrl Pts',(6.99999999912704,6.72060693187971,-22.0494138888238));
#49461=CARTESIAN_POINT('Ctrl Pts',(6.99999999825471,6.87797393131849,-22.2850194610423));
#49462=CARTESIAN_POINT('Ctrl Pts',(6.99999999886799,7.04445985882369,-22.5145575357774));
#49463=CARTESIAN_POINT('Ctrl Pts',(6.99999999981994,7.2197221995766,-22.7374276556396));
#49464=CARTESIAN_POINT('Ctrl Pts',(6.99999999992602,7.23925208826038,-22.7622625894488));
#49465=CARTESIAN_POINT('Ctrl Pts',(6.99999999999964,7.2588909847756,-22.7870146819099));
#49466=CARTESIAN_POINT('Ctrl Pts',(6.99999999999964,7.27863843674251,-22.811683068204));
#49467=CARTESIAN_POINT('Ctrl Pts',(6.99999999999964,7.4168811114768,-22.9843749024913));
#49468=CARTESIAN_POINT('Ctrl Pts',(6.99999999634605,7.56041237864492,-23.1529986871859));
#49469=CARTESIAN_POINT('Ctrl Pts',(6.99999999542156,7.70885456978368,-23.3170717122661));
#49470=CARTESIAN_POINT('Ctrl Pts',(6.99999999531129,7.72655977575305,-23.3366412610634));
#49471=CARTESIAN_POINT('Ctrl Pts',(6.99999999523589,7.74433480164425,-23.3561461126841));
#49472=CARTESIAN_POINT('Ctrl Pts',(6.99999999520038,7.76217897185983,-23.3755854834775));
#49473=CARTESIAN_POINT('Ctrl Pts',(6.99999999489231,7.91695873329861,-23.5442019636824));
#49474=CARTESIAN_POINT('Ctrl Pts',(6.99999999999964,8.07694373314969,-23.7078879606588));
#49475=CARTESIAN_POINT('Ctrl Pts',(6.99999999999964,8.24158930395947,-23.866242493597));
#49476=CARTESIAN_POINT('Ctrl Pts',(6.99999999999964,8.36428137259446,-23.9842465499974));
#49477=CARTESIAN_POINT('Ctrl Pts',(6.99999999741396,8.48959541717548,-24.0992443287782));
#49478=CARTESIAN_POINT('Ctrl Pts',(6.999999997457,8.61757747788213,-24.2113318768014));
#49479=CARTESIAN_POINT('Ctrl Pts',(6.99999999749808,8.73974118137153,-24.3183236685101));
#49480=CARTESIAN_POINT('Ctrl Pts',(6.99999999865099,8.86433631653384,-24.4226638135537));
#49481=CARTESIAN_POINT('Ctrl Pts',(6.9999999992403,8.99143397729645,-24.5244042570306));
#49482=CARTESIAN_POINT('Ctrl Pts',(6.99999999975841,9.10317464243632,-24.6138515746092));
#49483=CARTESIAN_POINT('Ctrl Pts',(6.99999999990827,9.21685018958274,-24.7012891605354));
#49484=CARTESIAN_POINT('Ctrl Pts',(6.99999999989361,9.33251047980344,-24.7867157008307));
#49485=CARTESIAN_POINT('Ctrl Pts',(6.26386081901915,3.90572621523646,-15.8144408559843));
#49486=CARTESIAN_POINT('Ctrl Pts',(6.26460715483143,3.90306655874706,-16.0736393146914));
#49487=CARTESIAN_POINT('Ctrl Pts',(6.26531568073978,3.9088164615582,-16.3306786832361));
#49488=CARTESIAN_POINT('Ctrl Pts',(6.26598637993336,3.92256301947529,-16.5850659454606));
#49489=CARTESIAN_POINT('Ctrl Pts',(6.26666472878982,3.93646636382485,-16.8423546228283));
#49490=CARTESIAN_POINT('Ctrl Pts',(6.26730438316959,3.95854979957321,-17.0969304079669));
#49491=CARTESIAN_POINT('Ctrl Pts',(6.26790532902729,3.98839267344383,-17.3483359936474));
#49492=CARTESIAN_POINT('Ctrl Pts',(6.26800175869402,3.99318135506081,-17.3886773264485));
#49493=CARTESIAN_POINT('Ctrl Pts',(6.26809719168382,3.99816984378879,-17.4289371396668));
#49494=CARTESIAN_POINT('Ctrl Pts',(6.26819162794592,4.00335641748679,-17.469113666875));
#49495=CARTESIAN_POINT('Ctrl Pts',(6.26876871361724,4.03505078253044,-17.7146263296978));
#49496=CARTESIAN_POINT('Ctrl Pts',(6.2693085788154,4.07414047215226,-17.9570248844362));
#49497=CARTESIAN_POINT('Ctrl Pts',(6.26981121343943,4.12010867076005,-18.1959008431826));
#49498=CARTESIAN_POINT('Ctrl Pts',(6.27017912193638,4.15375555867615,-18.3707485172967));
#49499=CARTESIAN_POINT('Ctrl Pts',(6.27052708362784,4.19108813783622,-18.5437099551103));
#49500=CARTESIAN_POINT('Ctrl Pts',(6.27085509534091,4.2319104395092,-18.7146413025029));
#49501=CARTESIAN_POINT('Ctrl Pts',(6.27121137967983,4.27625137669193,-18.900305898243));
#49502=CARTESIAN_POINT('Ctrl Pts',(6.2715441253586,4.32470945321996,-19.0835751290548));
#49503=CARTESIAN_POINT('Ctrl Pts',(6.27185332829706,4.37704091279458,-19.2642823708179));
#49504=CARTESIAN_POINT('Ctrl Pts',(6.27227096980512,4.44772520125795,-19.5083642846041));
#49505=CARTESIAN_POINT('Ctrl Pts',(6.27264565985936,4.52547487734651,-19.7477704244421));
#49506=CARTESIAN_POINT('Ctrl Pts',(6.27297739052688,4.60968091118585,-19.9821806569633));
#49507=CARTESIAN_POINT('Ctrl Pts',(6.27330912119439,4.6938869450252,-20.2165908894845));
#49508=CARTESIAN_POINT('Ctrl Pts',(6.27359789249436,4.78454940161974,-20.4460053998776));
#49509=CARTESIAN_POINT('Ctrl Pts',(6.27384369863648,4.88108706281011,-20.6701555296204));
#49510=CARTESIAN_POINT('Ctrl Pts',(6.27395596464763,4.92517830501504,-20.7725306808193));
#49511=CARTESIAN_POINT('Ctrl Pts',(6.27405926825717,4.9704954823184,-20.8738083811902));
#49512=CARTESIAN_POINT('Ctrl Pts',(6.27415361609019,5.01698510371503,-20.9739664611315));
#49513=CARTESIAN_POINT('Ctrl Pts',(6.27415651999336,5.01841599359143,-20.9770491961231));
#49514=CARTESIAN_POINT('Ctrl Pts',(6.2741594153517,5.01984799417455,-20.9801308705135));
#49515=CARTESIAN_POINT('Ctrl Pts',(6.27416230217101,5.02128110392859,-20.9832114836985));
#49516=CARTESIAN_POINT('Ctrl Pts',(6.27420631174089,5.04312886679225,-21.0301754417279));
#49517=CARTESIAN_POINT('Ctrl Pts',(6.27424833675569,5.06523440558947,-21.0768927576288));
#49518=CARTESIAN_POINT('Ctrl Pts',(6.2742883978265,5.08759148600678,-21.1233617479934));
#49519=CARTESIAN_POINT('Ctrl Pts',(6.27431785040983,5.10402823521087,-21.1575253832326));
#49520=CARTESIAN_POINT('Ctrl Pts',(6.2743467021673,5.12089395791622,-21.1921536959186));
#49521=CARTESIAN_POINT('Ctrl Pts',(6.27437398897063,5.1375813421622,-21.2260056020033));
#49522=CARTESIAN_POINT('Ctrl Pts',(6.27438625195006,5.14508083000008,-21.2412190083843));
#49523=CARTESIAN_POINT('Ctrl Pts',(6.27439819885563,5.15254365473743,-21.2562759175005));
#49524=CARTESIAN_POINT('Ctrl Pts',(6.27440974217502,5.15991163508647,-21.2710652003407));
#49525=CARTESIAN_POINT('Ctrl Pts',(6.27456064646664,5.25623227027768,-21.4644035440535));
#49526=CARTESIAN_POINT('Ctrl Pts',(6.27467736455278,5.35907892797542,-21.6577057407531));
#49527=CARTESIAN_POINT('Ctrl Pts',(6.2747598946937,5.46870212487468,-21.8504730214076));
#49528=CARTESIAN_POINT('Ctrl Pts',(6.27484107136038,5.57652752800879,-22.0400789655467));
#49529=CARTESIAN_POINT('Ctrl Pts',(6.27488917224047,5.69090909310062,-22.2291674455941));
#49530=CARTESIAN_POINT('Ctrl Pts',(6.27490419665066,5.81206997999551,-22.4172156503231));
#49531=CARTESIAN_POINT('Ctrl Pts',(6.27490863038766,5.84782482830833,-22.4727090955091));
#49532=CARTESIAN_POINT('Ctrl Pts',(6.27491018365568,5.88416995006603,-22.528111621419));
#49533=CARTESIAN_POINT('Ctrl Pts',(6.27490885645281,5.92111080747901,-22.5834089610956));
#49534=CARTESIAN_POINT('Ctrl Pts',(6.27490450801904,6.04214345090047,-22.7645845932802));
#49535=CARTESIAN_POINT('Ctrl Pts',(6.27486923844804,6.16957277182416,-22.9446345885511));
#49536=CARTESIAN_POINT('Ctrl Pts',(6.27480304820754,6.30354307114202,-23.1230244188957));
#49537=CARTESIAN_POINT('Ctrl Pts',(6.27475276959969,6.40530792487314,-23.2585306847215));
#49538=CARTESIAN_POINT('Ctrl Pts',(6.2746846496685,6.51084655159941,-23.3930781264593));
#49539=CARTESIAN_POINT('Ctrl Pts',(6.2745986889403,6.62021382699481,-23.5264141272963));
#49540=CARTESIAN_POINT('Ctrl Pts',(6.27448994453198,6.75856863043007,-23.6950905080506));
#49541=CARTESIAN_POINT('Ctrl Pts',(6.27435264758153,6.90305132253116,-23.8618296346804));
#49542=CARTESIAN_POINT('Ctrl Pts',(6.27418680056911,7.05375519708462,-24.0260820616461));
#49543=CARTESIAN_POINT('Ctrl Pts',(6.274013150482,7.21154966418197,-24.1980625383213));
#49544=CARTESIAN_POINT('Ctrl Pts',(6.27380820056856,7.37616533894926,-24.3673161423291));
#49545=CARTESIAN_POINT('Ctrl Pts',(6.27357195460688,7.5476343484384,-24.5332734929099));
#49546=CARTESIAN_POINT('Ctrl Pts',(6.27333930167313,7.71649551254562,-24.6967068240682));
#49547=CARTESIAN_POINT('Ctrl Pts',(6.27307629740119,7.89200319539931,-24.8569434210827));
#49548=CARTESIAN_POINT('Ctrl Pts',(6.27278294639037,8.07415574466986,-25.0134008439504));
#49549=CARTESIAN_POINT('Ctrl Pts',(6.27261681548821,8.17731259849041,-25.1020060024537));
#49550=CARTESIAN_POINT('Ctrl Pts',(6.27244095180671,8.28259999770744,-25.1893983995385));
#49551=CARTESIAN_POINT('Ctrl Pts',(6.27225535633498,8.39001281171083,-25.2754665765872));
#49552=CARTESIAN_POINT('Ctrl Pts',(6.27204648357802,8.51089728364193,-25.3723293785642));
#49553=CARTESIAN_POINT('Ctrl Pts',(6.27182528483322,8.63447390919248,-25.4675151877984));
#49554=CARTESIAN_POINT('Ctrl Pts',(6.27159176169366,8.76072155998436,-25.5608443101141));
#49555=CARTESIAN_POINT('Ctrl Pts',(-6.390310997166,3.94960612761086,-15.460427010644));
#49556=CARTESIAN_POINT('Ctrl Pts',(-4.260207331444,3.32899321753374,-16.2185125151969));
#49557=CARTESIAN_POINT('Ctrl Pts',(0.000153520239401,2.70682972226379,-16.9766167275286));
#49558=CARTESIAN_POINT('Ctrl Pts',(4.260514371923,3.32903805792829,-16.2184578773201));
#49559=CARTESIAN_POINT('Ctrl Pts',(6.390771557884,3.94974031835815,-15.4602630951545));
#49560=CARTESIAN_POINT('Ctrl Pts',(-6.390310997166,3.91824263644539,-16.2404224492195));
#49561=CARTESIAN_POINT('Ctrl Pts',(-4.260207331444,3.34435590545916,-16.9591796463154));
#49562=CARTESIAN_POINT('Ctrl Pts',(0.000153520239401,2.76852197294671,-17.6779444417002));
#49563=CARTESIAN_POINT('Ctrl Pts',(4.260514371923,3.34439740680201,-16.9591278436997));
#49564=CARTESIAN_POINT('Ctrl Pts',(6.390771557884,3.91836672392008,-16.24026703742));
#49565=CARTESIAN_POINT('Ctrl Pts',(-6.390310997166,4.02654093202666,-18.1258725679872));
#49566=CARTESIAN_POINT('Ctrl Pts',(-4.260207331444,3.53815115056139,-18.7395194904352));
#49567=CARTESIAN_POINT('Ctrl Pts',(0.0001535202393995,3.05107476647531,
-19.3531445395367));
#49568=CARTESIAN_POINT('Ctrl Pts',(4.260514371923,3.53818625499516,-18.7394752654212));
#49569=CARTESIAN_POINT('Ctrl Pts',(6.390771557884,4.02664653311775,-18.1257398834285));
#49570=CARTESIAN_POINT('Ctrl Pts',(-6.390310997166,4.89945800148072,-21.0044951210845));
#49571=CARTESIAN_POINT('Ctrl Pts',(-4.260207331444,4.44478850538018,-21.4424839510795));
#49572=CARTESIAN_POINT('Ctrl Pts',(0.0001535202394003,3.98943347064956,
-21.8807678511962));
#49573=CARTESIAN_POINT('Ctrl Pts',(4.260514371923,4.44482132360267,-21.4424523632058));
#49574=CARTESIAN_POINT('Ctrl Pts',(6.390771557884,4.89955631145556,-21.0044004178407));
#49575=CARTESIAN_POINT('Ctrl Pts',(-6.390310997166,6.63374317910258,-23.7052268139868));
#49576=CARTESIAN_POINT('Ctrl Pts',(-4.260207331444,6.09525793886643,-23.998130417564));
#49577=CARTESIAN_POINT('Ctrl Pts',(0.0001535202394,5.55782046091975,-24.2900534534943));
#49578=CARTESIAN_POINT('Ctrl Pts',(4.260514371923,6.09529667291084,-23.9981093781683));
#49579=CARTESIAN_POINT('Ctrl Pts',(6.390771557884,6.63385961198203,-23.7051634814939));
#49580=CARTESIAN_POINT('Ctrl Pts',(-6.390310997166,8.18394426417614,-25.1149800440698));
#49581=CARTESIAN_POINT('Ctrl Pts',(-4.260207331444,7.53598539108648,-25.3660541903064));
#49582=CARTESIAN_POINT('Ctrl Pts',(0.0001535202394001,6.88615442358477,
-25.6190324252077));
#49583=CARTESIAN_POINT('Ctrl Pts',(4.260514371923,7.53603222552418,-25.3660359577308));
#49584=CARTESIAN_POINT('Ctrl Pts',(6.390771557884,8.18408436774532,-25.1149257560885));
#49585=CARTESIAN_POINT('Ctrl Pts',(-6.390310997166,8.98425310970363,-25.6807323427288));
#49586=CARTESIAN_POINT('Ctrl Pts',(-4.260207331444,8.27686639982284,-25.9287942674702));
#49587=CARTESIAN_POINT('Ctrl Pts',(0.0001535202394001,7.5688707583203,-26.1774614807514));
#49588=CARTESIAN_POINT('Ctrl Pts',(4.260514371923,8.27691742628879,-25.9287763455956));
#49589=CARTESIAN_POINT('Ctrl Pts',(6.390771557884,8.98440606294867,-25.6806787060575));
#49590=CARTESIAN_POINT('Ctrl Pts',(-6.26386059950783,3.90573753004527,-15.8144217560873));
#49591=CARTESIAN_POINT('Ctrl Pts',(-5.97372627968023,3.82530519121327,-15.9109296281103));
#49592=CARTESIAN_POINT('Ctrl Pts',(-5.68164548281105,3.74986547664179,-16.0001140046338));
#49593=CARTESIAN_POINT('Ctrl Pts',(-5.38811095600305,3.67970569357336,-16.0820552820059));
#49594=CARTESIAN_POINT('Ctrl Pts',(-5.1129382354064,3.61393469690952,-16.1588707914754));
#49595=CARTESIAN_POINT('Ctrl Pts',(-4.83648797010696,3.55280433012687,-16.229320691623));
#49596=CARTESIAN_POINT('Ctrl Pts',(-4.55916610084168,3.49652988606607,-16.2935087073498));
#49597=CARTESIAN_POINT('Ctrl Pts',(-4.30168885183784,3.44428233312557,-16.3531035519689));
#49598=CARTESIAN_POINT('Ctrl Pts',(-4.04346027638,3.39622087517566,-16.4073005338585));
#49599=CARTESIAN_POINT('Ctrl Pts',(-3.78480525737339,3.35249305011429,-16.4562187999834));
#49600=CARTESIAN_POINT('Ctrl Pts',(-3.57018253931316,3.31620925904162,-16.4968094340984));
#49601=CARTESIAN_POINT('Ctrl Pts',(-3.35526621107239,3.28290892324508,-16.5337661150051));
#49602=CARTESIAN_POINT('Ctrl Pts',(-3.1402418783052,3.25265989964445,-16.5671788848135));
#49603=CARTESIAN_POINT('Ctrl Pts',(-2.90174875105576,3.219109351472,-16.6042384857393));
#49604=CARTESIAN_POINT('Ctrl Pts',(-2.66311062362395,3.18931283044879,-16.6369596995847));
#49605=CARTESIAN_POINT('Ctrl Pts',(-2.42457575010895,3.16332914900677,-16.6653611706952));
#49606=CARTESIAN_POINT('Ctrl Pts',(-2.18945145913184,3.13771698343113,-16.6933565562721));
#49607=CARTESIAN_POINT('Ctrl Pts',(-1.95442749052171,3.11580944452607,-16.7171548319756));
#49608=CARTESIAN_POINT('Ctrl Pts',(-1.71974160126147,3.09763059235909,-16.7368128800229));
#49609=CARTESIAN_POINT('Ctrl Pts',(-1.48657671707649,3.07956955778435,-16.7563435237727));
#49610=CARTESIAN_POINT('Ctrl Pts',(-1.25374554424066,3.0651890947204,-16.7717873914836));
#49611=CARTESIAN_POINT('Ctrl Pts',(-1.02148124690547,3.05447991685876,-16.7832395301357));
#49612=CARTESIAN_POINT('Ctrl Pts',(-0.790833753306384,3.04384528613577,
-16.7946119498608));
#49613=CARTESIAN_POINT('Ctrl Pts',(-0.560745270577479,3.03683103914573,
-16.8020480059554));
#49614=CARTESIAN_POINT('Ctrl Pts',(-0.331444127483368,3.03339486825846,
-16.8056800208761));
#49615=CARTESIAN_POINT('Ctrl Pts',(-0.220772843970497,3.03173641406442,
-16.807432998413));
#49616=CARTESIAN_POINT('Ctrl Pts',(-0.110284969003811,3.0309109629497,-16.8083004233882));
#49617=CARTESIAN_POINT('Ctrl Pts',(-6.17382099488752E-6,3.0309109343344,
-16.8083004870552));
#49618=CARTESIAN_POINT('Ctrl Pts',(-4.11588034283447E-6,3.03091093433386,
-16.8083004870564));
#49619=CARTESIAN_POINT('Ctrl Pts',(-2.05793961891125E-6,3.03091093433362,
-16.8083004870572));
#49620=CARTESIAN_POINT('Ctrl Pts',(1.1750539249883E-12,3.03091093433366,
-16.8083004870578));
#49621=CARTESIAN_POINT('Ctrl Pts',(0.230475565322468,3.03091093890162,-16.8083005524742));
#49622=CARTESIAN_POINT('Ctrl Pts',(0.461841095866946,3.03451839678727,-16.8045094946044));
#49623=CARTESIAN_POINT('Ctrl Pts',(0.693872690690212,3.04179180534984,-16.7967739675693));
#49624=CARTESIAN_POINT('Ctrl Pts',(0.927916161739583,3.04912827945217,-16.7889713681041));
#49625=CARTESIAN_POINT('Ctrl Pts',(1.16263729762952,3.06019453604654,-16.7771555978514));
#49626=CARTESIAN_POINT('Ctrl Pts',(1.39780632263695,3.0750161307351,-16.7612097989639));
#49627=CARTESIAN_POINT('Ctrl Pts',(1.63455675554439,3.08993739410635,-16.7451567716167));
#49628=CARTESIAN_POINT('Ctrl Pts',(1.871761121536,3.10866461740418,-16.7249180178633));
#49629=CARTESIAN_POINT('Ctrl Pts',(2.10918497822673,3.13118963469091,-16.7004149289351));
#49630=CARTESIAN_POINT('Ctrl Pts',(2.34961346391676,3.1539997089264,-16.6756017503109));
#49631=CARTESIAN_POINT('Ctrl Pts',(2.59026703082308,3.18070426197141,-16.6464156411019));
#49632=CARTESIAN_POINT('Ctrl Pts',(2.83090222275172,3.21126053308359,-16.6128161441932));
#49633=CARTESIAN_POINT('Ctrl Pts',(2.93386713401478,3.22433519485014,-16.5984393226237));
#49634=CARTESIAN_POINT('Ctrl Pts',(3.03682868103732,3.23811464118123,-16.5832549690811));
#49635=CARTESIAN_POINT('Ctrl Pts',(3.13976779116438,3.2525936804676,-16.5672621526594));
#49636=CARTESIAN_POINT('Ctrl Pts',(3.40252257005505,3.28955180805919,-16.5264400692207));
#49637=CARTESIAN_POINT('Ctrl Pts',(3.66512621014034,3.33106867965023,-16.4803234953586));
#49638=CARTESIAN_POINT('Ctrl Pts',(3.92723945364459,3.37701812899252,-16.4287510375096));
#49639=CARTESIAN_POINT('Ctrl Pts',(4.19826717559078,3.4245303203394,-16.3754245989859));
#49640=CARTESIAN_POINT('Ctrl Pts',(4.4687705769213,3.47678129432531,-16.3162651879646));
#49641=CARTESIAN_POINT('Ctrl Pts',(4.73837459477634,3.53359543051034,-16.2511431923738));
#49642=CARTESIAN_POINT('Ctrl Pts',(5.03395192678833,3.595882969575,-16.1797474251104));
#49643=CARTESIAN_POINT('Ctrl Pts',(5.32844823704742,3.66365486004385,-16.1011849319197));
#49644=CARTESIAN_POINT('Ctrl Pts',(5.62136928502598,3.73664288696887,-16.0153401939371));
#49645=CARTESIAN_POINT('Ctrl Pts',(5.83644665881003,3.79023436923702,-15.9523086674358));
#49646=CARTESIAN_POINT('Ctrl Pts',(6.05067477162441,3.84663711861222,-15.8853523700907));
#49647=CARTESIAN_POINT('Ctrl Pts',(6.26385797755097,3.90573660178328,-15.8144409707664));
#49648=CARTESIAN_POINT('Ctrl Pts',(-6.38246269292625,3.93894967362139,-15.7729097725756));
#49649=CARTESIAN_POINT('Ctrl Pts',(-5.83395600374064,3.78387662728214,-15.9702601123439));
#49650=CARTESIAN_POINT('Ctrl Pts',(-4.51676965304293,3.45862254641806,-16.3719120782295));
#49651=CARTESIAN_POINT('Ctrl Pts',(-2.37673153344301,3.11825374849332,-16.7692680861992));
#49652=CARTESIAN_POINT('Ctrl Pts',(0.000175407413350786,2.99129135223685,
-16.9125154471428));
#49653=CARTESIAN_POINT('Ctrl Pts',(2.37708240512334,3.11829116289182,-16.7692254872644));
#49654=CARTESIAN_POINT('Ctrl Pts',(4.51699670078421,3.45867323308068,-16.3718511298187));
#49655=CARTESIAN_POINT('Ctrl Pts',(5.83406738808232,3.78390812439344,-15.9702199714471));
#49656=CARTESIAN_POINT('Ctrl Pts',(6.38246334095398,3.93894987729812,-15.7729094699168));
#49657=CARTESIAN_POINT('Ctrl Pts',(-6.17758168919576,3.88967198539074,-15.154162882923));
#49658=CARTESIAN_POINT('Ctrl Pts',(-5.64640092257065,3.74166898124023,-15.3452128053215));
#49659=CARTESIAN_POINT('Ctrl Pts',(-4.370973200626,3.43112903201519,-15.7340791545028));
#49660=CARTESIAN_POINT('Ctrl Pts',(-2.29961550285046,3.10606644179156,-16.118753707528));
#49661=CARTESIAN_POINT('Ctrl Pts',(0.000169703128138686,2.98481674989937,
-16.257404296828));
#49662=CARTESIAN_POINT('Ctrl Pts',(2.29995503766859,3.10610217341112,-16.1187124731847));
#49663=CARTESIAN_POINT('Ctrl Pts',(4.37119302862394,3.43117743709702,-15.7340201451118));
#49664=CARTESIAN_POINT('Ctrl Pts',(5.64650878850444,3.74169904124616,-15.3451739455801));
#49665=CARTESIAN_POINT('Ctrl Pts',(6.1775823172684,3.88967217936339,-15.15416258936));
#49666=CARTESIAN_POINT('Ctrl Pts',(-6.17627524027959,3.38234690796609,-14.7450182290604));
#49667=CARTESIAN_POINT('Ctrl Pts',(-5.64643658833439,3.23615773351961,-14.9338120192099));
#49668=CARTESIAN_POINT('Ctrl Pts',(-4.37356735177373,2.92910800412423,-15.3184353559978));
#49669=CARTESIAN_POINT('Ctrl Pts',(-2.30271816604516,2.60683192149392,-15.6997831889741));
#49670=CARTESIAN_POINT('Ctrl Pts',(0.000169988787698856,2.48637475214055,
-15.8374778743519));
#49671=CARTESIAN_POINT('Ctrl Pts',(2.30305795089379,2.60686739928376,-15.6997422594087));
#49672=CARTESIAN_POINT('Ctrl Pts',(4.37378683344432,2.92915591510232,-15.3183769362156));
#49673=CARTESIAN_POINT('Ctrl Pts',(5.64654418199573,3.23618742585186,-14.9337736202781));
#49674=CARTESIAN_POINT('Ctrl Pts',(6.17627586451967,3.38234709913452,-14.7450179412791));
#49675=CARTESIAN_POINT('Ctrl Pts',(-6.37670151809056,2.76894332529829,-14.8215582716457));
#49676=CARTESIAN_POINT('Ctrl Pts',(-5.83152084753289,2.61814590976835,-15.0136238374691));
#49677=CARTESIAN_POINT('Ctrl Pts',(-4.52079209118095,2.30113400780086,-15.4053243805069));
#49678=CARTESIAN_POINT('Ctrl Pts',(-2.3828478805525,1.96739333350805,-15.794842346463));
#49679=CARTESIAN_POINT('Ctrl Pts',(0.000175989273597215,1.84233431609406,
-15.9358247251825));
#49680=CARTESIAN_POINT('Ctrl Pts',(2.38319917637242,1.96743014026188,-15.7948004683328));
#49681=CARTESIAN_POINT('Ctrl Pts',(4.52101824376224,2.30118352497297,-15.4052648171334));
#49682=CARTESIAN_POINT('Ctrl Pts',(5.83163155708262,2.61817654012613,-15.0135847758853));
#49683=CARTESIAN_POINT('Ctrl Pts',(6.37670215701753,2.7689435223799,-14.8215579824318));
#49684=CARTESIAN_POINT('Ctrl Pts',(-6.24994460521886,2.76546685544382,-14.8593819056678));
#49685=CARTESIAN_POINT('Ctrl Pts',(-5.99094249999219,2.69516002979088,-14.9486425804541));
#49686=CARTESIAN_POINT('Ctrl Pts',(-5.72720728127898,2.62787545102769,-15.0328670687827));
#49687=CARTESIAN_POINT('Ctrl Pts',(-5.45886142643465,2.56415819329477,-15.1117505190932));
#49688=CARTESIAN_POINT('Ctrl Pts',(-5.22285449580001,2.50811963650497,-15.181127558647));
#49689=CARTESIAN_POINT('Ctrl Pts',(-4.98328152550268,2.45484087388617,-15.2463730336044));
#49690=CARTESIAN_POINT('Ctrl Pts',(-4.74024475778304,2.40471692783325,-15.3072665448488));
#49691=CARTESIAN_POINT('Ctrl Pts',(-4.72533948106778,2.40164286092153,-15.3110011017382));
#49692=CARTESIAN_POINT('Ctrl Pts',(-4.71042120035891,2.39858060782454,-15.3147192911877));
#49693=CARTESIAN_POINT('Ctrl Pts',(-4.69548992988297,2.39553024632854,-15.3184210658687));
#49694=CARTESIAN_POINT('Ctrl Pts',(-4.45028046023139,2.34543554568759,-15.3792136292185));
#49695=CARTESIAN_POINT('Ctrl Pts',(-4.20156648623987,2.29854558829399,-15.4355808996657));
#49696=CARTESIAN_POINT('Ctrl Pts',(-3.94948718691868,2.25519371924219,-15.4873109946335));
#49697=CARTESIAN_POINT('Ctrl Pts',(-3.8157727435299,2.23219789588131,-15.5147510139992));
#49698=CARTESIAN_POINT('Ctrl Pts',(-3.6811117686411,2.21019665045448,-15.5408860893749));
#49699=CARTESIAN_POINT('Ctrl Pts',(-3.545527931086,2.18923389337213,-15.5656831929245));
#49700=CARTESIAN_POINT('Ctrl Pts',(-3.47773601230845,2.17875251483096,-15.5780817446993));
#49701=CARTESIAN_POINT('Ctrl Pts',(-3.4097133744286,2.16853075563841,-15.5901457844336));
#49702=CARTESIAN_POINT('Ctrl Pts',(-3.34146322033014,2.15857364302317,-15.601871087987));
#49703=CARTESIAN_POINT('Ctrl Pts',(-3.30733814328091,2.15359508671555,-15.6077337397637));
#49704=CARTESIAN_POINT('Ctrl Pts',(-3.27315618700011,2.14868269188944,-15.6135117062827));
#49705=CARTESIAN_POINT('Ctrl Pts',(-3.23891775843242,2.14383707189763,-15.6192044529497));
#49706=CARTESIAN_POINT('Ctrl Pts',(-3.22179854414857,2.14141426190172,-15.6220508262832));
#49707=CARTESIAN_POINT('Ctrl Pts',(-3.2046652117838,2.1390081456044,-15.6248758945757));
#49708=CARTESIAN_POINT('Ctrl Pts',(-3.187517813095,2.13661879796061,-15.6276795906241));
#49709=CARTESIAN_POINT('Ctrl Pts',(-3.17037041440618,2.13422945031681,-15.6304832866724));
#49710=CARTESIAN_POINT('Ctrl Pts',(-3.15207046448132,2.13170072040929,-15.6334486169825));
#49711=CARTESIAN_POINT('Ctrl Pts',(-3.13603347006549,2.12950113539336,-15.6360264945505));
#49712=CARTESIAN_POINT('Ctrl Pts',(-2.87501520781348,2.0937006703159,-15.6779840525346));
#49713=CARTESIAN_POINT('Ctrl Pts',(-2.61248816369087,2.06209953498922,-15.7147041617999));
#49714=CARTESIAN_POINT('Ctrl Pts',(-2.34863686523688,2.03493974475676,-15.7461369357379));
#49715=CARTESIAN_POINT('Ctrl Pts',(-2.04845599284398,2.00404033446862,-15.7818976750548));
#49716=CARTESIAN_POINT('Ctrl Pts',(-1.74656066392248,1.97888880541283,-15.8108155701126));
#49717=CARTESIAN_POINT('Ctrl Pts',(-1.44332961648421,1.95966138466728,-15.8328336538368));
#49718=CARTESIAN_POINT('Ctrl Pts',(-1.14508568668948,1.94075018948653,-15.8544896150977));
#49719=CARTESIAN_POINT('Ctrl Pts',(-0.845549100638975,1.9275697949549,-15.869470795419));
#49720=CARTESIAN_POINT('Ctrl Pts',(-0.545085108667407,1.92032135217525,
-15.8776861228819));
#49721=CARTESIAN_POINT('Ctrl Pts',(-0.363702352701681,1.91594564472622,
-15.8826455149428));
#49722=CARTESIAN_POINT('Ctrl Pts',(-0.181981756268516,1.91373233336849,
-15.885138558788));
#49723=CARTESIAN_POINT('Ctrl Pts',(-5.73471096132168E-6,1.91373185585388,
-15.8851386642953));
#49724=CARTESIAN_POINT('Ctrl Pts',(5.39138121133536E-5,1.91373185569736,
-15.8851386643299));
#49725=CARTESIAN_POINT('Ctrl Pts',(0.00011356230696275,1.91373185577524,
-15.885138664097));
#49726=CARTESIAN_POINT('Ctrl Pts',(0.000173210773584176,1.91373185608752,
-15.8851386635966));
#49727=CARTESIAN_POINT('Ctrl Pts',(0.297559266330309,1.91373341299712,-15.8851361688966));
#49728=CARTESIAN_POINT('Ctrl Pts',(0.594244088085259,1.91955829910996,-15.8784882520397));
#49729=CARTESIAN_POINT('Ctrl Pts',(0.889890545446005,1.93109463048215,-15.8652927006163));
#49730=CARTESIAN_POINT('Ctrl Pts',(1.12073841233604,1.94010247557111,-15.8549892965919));
#49731=CARTESIAN_POINT('Ctrl Pts',(1.35095322925663,1.95259331338095,-15.8406930825171));
#49732=CARTESIAN_POINT('Ctrl Pts',(1.58037070720459,1.9685285947701,-15.8224346483479));
#49733=CARTESIAN_POINT('Ctrl Pts',(1.83765030286678,1.98639917197822,-15.8019587778847));
#49734=CARTESIAN_POINT('Ctrl Pts',(2.09393063440068,2.00857720947524,-15.7765029281989));
#49735=CARTESIAN_POINT('Ctrl Pts',(2.34899413482236,2.03488903452172,-15.7461056736265));
#49736=CARTESIAN_POINT('Ctrl Pts',(2.35332241868072,2.03533553136445,-15.7455898493471));
#49737=CARTESIAN_POINT('Ctrl Pts',(2.35765035237713,2.03578321905682,-15.7450726015952));
#49738=CARTESIAN_POINT('Ctrl Pts',(2.36197793520127,2.03623209616452,-15.7445539306617));
#49739=CARTESIAN_POINT('Ctrl Pts',(2.49165282103475,2.04968258112567,-15.7290120919899));
#49740=CARTESIAN_POINT('Ctrl Pts',(2.62101226358897,2.06419998622132,-15.7121926420529));
#49741=CARTESIAN_POINT('Ctrl Pts',(2.75002880797683,2.07975509189862,-15.6941026937445));
#49742=CARTESIAN_POINT('Ctrl Pts',(2.81453708017076,2.08753264473727,-15.6850577195903));
#49743=CARTESIAN_POINT('Ctrl Pts',(2.87895962758892,2.09556962127403,-15.6756951086055));
#49744=CARTESIAN_POINT('Ctrl Pts',(2.94329309702094,2.10386188537721,-15.6660157300993));
#49745=CARTESIAN_POINT('Ctrl Pts',(2.97545983173696,2.10800801742881,-15.6611760408462));
#49746=CARTESIAN_POINT('Ctrl Pts',(3.0076042969285,2.1122179712847,-15.6562571589625));
#49747=CARTESIAN_POINT('Ctrl Pts',(3.0397260755728,2.11649121694422,-15.6512591900128));
#49748=CARTESIAN_POINT('Ctrl Pts',(3.05578696489494,2.11862783977398,-15.648760205538));
#49749=CARTESIAN_POINT('Ctrl Pts',(3.07184218257719,2.12078028554911,-15.6462414492505));
#49750=CARTESIAN_POINT('Ctrl Pts',(3.08789167676611,2.12294848633111,-15.6437029342547));
#49751=CARTESIAN_POINT('Ctrl Pts',(3.10394117095503,2.1251166871131,-15.6411644192589));
#49752=CARTESIAN_POINT('Ctrl Pts',(3.11884751751632,2.12714464314771,-15.6387889801949));
#49753=CARTESIAN_POINT('Ctrl Pts',(3.13602293707478,2.1295002852458,-15.6360281261192));
#49754=CARTESIAN_POINT('Ctrl Pts',(3.41741466579409,2.16809370649934,-15.5907959558965));
#49755=CARTESIAN_POINT('Ctrl Pts',(3.69506739828332,2.21131136347053,-15.5397930462567));
#49756=CARTESIAN_POINT('Ctrl Pts',(3.96874459550752,2.25866743763374,-15.4833263036421));
#49757=CARTESIAN_POINT('Ctrl Pts',(4.21434190285783,2.30116467313283,-15.4326531745628));
#49758=CARTESIAN_POINT('Ctrl Pts',(4.45673811956246,2.34699530799611,-15.3775795312776));
#49759=CARTESIAN_POINT('Ctrl Pts',(4.69578022911293,2.39583435949049,-15.318310772496));
#49760=CARTESIAN_POINT('Ctrl Pts',(4.97402015772782,2.45268197611741,-15.2493231985346));
#49761=CARTESIAN_POINT('Ctrl Pts',(5.24771606928571,2.51360455783964,-15.1746524946147));
#49762=CARTESIAN_POINT('Ctrl Pts',(5.5167488360978,2.57809132060363,-15.0946099661954));
#49763=CARTESIAN_POINT('Ctrl Pts',(5.76514914613282,2.63763251349824,-15.0207059986194));
#49764=CARTESIAN_POINT('Ctrl Pts',(6.00957444404958,2.70021279219826,-14.9422222022724));
#49765=CARTESIAN_POINT('Ctrl Pts',(6.24994323895025,2.76546151517861,-14.8593832382704));
#49766=CARTESIAN_POINT('Ctrl Pts',(7.10527469285759,-5.08837285721628,-15.2149674210636));
#49767=CARTESIAN_POINT('Ctrl Pts',(7.10577175309562,-5.05127732240867,-15.2272006288549));
#49768=CARTESIAN_POINT('Ctrl Pts',(7.10233361655264,-4.93362690673713,-15.2672676676193));
#49769=CARTESIAN_POINT('Ctrl Pts',(7.06814935170305,-4.72835757096628,-15.3442190548759));
#49770=CARTESIAN_POINT('Ctrl Pts',(6.97357315551598,-4.48015474944715,-15.4505389279076));
#49771=CARTESIAN_POINT('Ctrl Pts',(6.81834137563527,-4.24729988507321,-15.5671389409917));
#49772=CARTESIAN_POINT('Ctrl Pts',(6.60934038952052,-4.05649431802118,-15.6839486604479));
#49773=CARTESIAN_POINT('Ctrl Pts',(6.40994316745287,-3.9505452960972,-15.77095398068));
#49774=CARTESIAN_POINT('Ctrl Pts',(6.28626990966703,-3.91128985961304,-15.8165793739769));
#49775=CARTESIAN_POINT('Ctrl Pts',(6.24914971117037,-3.90167129702033,-15.829595813689));
#49776=CARTESIAN_POINT('Ctrl Pts',(6.81642516792956,-4.90351678924822,-14.6670079284464));
#49777=CARTESIAN_POINT('Ctrl Pts',(6.81687157292555,-4.87082825456401,-14.6777811179155));
#49778=CARTESIAN_POINT('Ctrl Pts',(6.81378644819866,-4.76705724898886,-14.7131664511101));
#49779=CARTESIAN_POINT('Ctrl Pts',(6.78300083518967,-4.58570531998746,-14.7816063849249));
#49780=CARTESIAN_POINT('Ctrl Pts',(6.69776708002038,-4.36656036449269,-14.8767160883548));
#49781=CARTESIAN_POINT('Ctrl Pts',(6.55813791989439,-4.16163596433278,-14.9812858449522));
#49782=CARTESIAN_POINT('Ctrl Pts',(6.3708916441972,-3.99466535000316,-15.0859722384302));
#49783=CARTESIAN_POINT('Ctrl Pts',(6.19324335984852,-3.90268987971195,-15.1636514989911));
#49784=CARTESIAN_POINT('Ctrl Pts',(6.08361516941286,-3.8688401576237,-15.2041933227212));
#49785=CARTESIAN_POINT('Ctrl Pts',(6.05076212875822,-3.86056538918408,-15.215740706429));
#49786=CARTESIAN_POINT('Ctrl Pts',(7.05949177097581,-4.7187225394648,-14.0973262672783));
#49787=CARTESIAN_POINT('Ctrl Pts',(7.06007854662092,-4.67643436909571,-14.1112731878018));
#49788=CARTESIAN_POINT('Ctrl Pts',(7.05601182042207,-4.54261602000926,-14.1568412078288));
#49789=CARTESIAN_POINT('Ctrl Pts',(7.01591712851095,-4.31014738785563,-14.2439120150253));
#49790=CARTESIAN_POINT('Ctrl Pts',(6.90517332848893,-4.02902460202869,-14.3641431158811));
#49791=CARTESIAN_POINT('Ctrl Pts',(6.72258565932859,-3.76383137770917,-14.4967470520898));
#49792=CARTESIAN_POINT('Ctrl Pts',(6.47447165821453,-3.54432976015602,-14.6311667794549));
#49793=CARTESIAN_POINT('Ctrl Pts',(6.23472572267083,-3.42079528084269,-14.733085402626));
#49794=CARTESIAN_POINT('Ctrl Pts',(6.08433124395451,-3.3746170314338,-14.7874360195946));
#49795=CARTESIAN_POINT('Ctrl Pts',(6.03903337281355,-3.36327931177702,-14.8030279496368));
#49796=CARTESIAN_POINT('Ctrl Pts',(7.66941902033053,-4.65925181838288,-13.8920899655214));
#49797=CARTESIAN_POINT('Ctrl Pts',(7.6702419374224,-4.59987218133953,-13.9116905082337));
#49798=CARTESIAN_POINT('Ctrl Pts',(7.66452510755031,-4.41247144972349,-13.975395110386));
#49799=CARTESIAN_POINT('Ctrl Pts',(7.60873074023539,-4.08854266857875,-14.0955952751784));
#49800=CARTESIAN_POINT('Ctrl Pts',(7.45493552358401,-3.69646802310441,-14.2602308509189));
#49801=CARTESIAN_POINT('Ctrl Pts',(7.1999797850509,-3.32370834451298,-14.4419084359676));
#49802=CARTESIAN_POINT('Ctrl Pts',(6.84968015880541,-3.01095984373919,-14.6277404369394));
#49803=CARTESIAN_POINT('Ctrl Pts',(6.50612889451362,-2.83175107132688,-14.7710147674676));
#49804=CARTESIAN_POINT('Ctrl Pts',(6.28782028218345,-2.76387668293926,-14.8486958800387));
#49805=CARTESIAN_POINT('Ctrl Pts',(6.22181049242793,-2.74714790790825,-14.8711013367127));
#49806=CARTESIAN_POINT('',(6.26385989016308,-3.90573722907187,-15.8144313885695));
#49807=CARTESIAN_POINT('',(6.24996242253145,-2.76547028474026,-14.8593821272229));
#49808=CARTESIAN_POINT('Origin',(6.527838794926,-2.94126717711685,-15.8037762219005));
#49809=CARTESIAN_POINT('',(6.99999979527712,-3.16612999317638,-14.5427403187255));
#49810=CARTESIAN_POINT('Ctrl Pts',(6.99999979527712,-3.16612999317638,-14.5427403187255));
#49811=CARTESIAN_POINT('Ctrl Pts',(6.96025925123918,-3.13150165427226,-14.5635935033793));
#49812=CARTESIAN_POINT('Ctrl Pts',(6.91940655197007,-3.09881147495865,-14.5841219942725));
#49813=CARTESIAN_POINT('Ctrl Pts',(6.87749829651554,-3.06800285157106,-14.6043423325847));
#49814=CARTESIAN_POINT('Ctrl Pts',(6.86185360058381,-3.05650173944537,-14.6118907509357));
#49815=CARTESIAN_POINT('Ctrl Pts',(6.84606134376919,-3.04526309517268,-14.6193962484639));
#49816=CARTESIAN_POINT('Ctrl Pts',(6.83012290677287,-3.03428495759989,-14.6268597356979));
#49817=CARTESIAN_POINT('Ctrl Pts',(6.78727089454268,-3.0047691847771,-14.6469260349407));
#49818=CARTESIAN_POINT('Ctrl Pts',(6.74336503020372,-2.9771339417348,-14.6666887601211));
#49819=CARTESIAN_POINT('Ctrl Pts',(6.69843860682942,-2.95134978681162,-14.6861604765471));
#49820=CARTESIAN_POINT('Ctrl Pts',(6.68185279676599,-2.94183086533775,-14.6933489898093));
#49821=CARTESIAN_POINT('Ctrl Pts',(6.66512751469401,-2.93256458045001,-14.7004978259819));
#49822=CARTESIAN_POINT('Ctrl Pts',(6.64826319259013,-2.92355073295329,-14.7076075327013));
#49823=CARTESIAN_POINT('Ctrl Pts',(6.60317001610057,-2.89944878485744,-14.7266180365279));
#49824=CARTESIAN_POINT('Ctrl Pts',(6.55709254862238,-2.8771564114029,-14.7453451674277));
#49825=CARTESIAN_POINT('Ctrl Pts',(6.51001371638684,-2.85669396795406,-14.7637988395615));
#49826=CARTESIAN_POINT('Ctrl Pts',(6.47779611569965,-2.84269084169084,-14.7764272972311));
#49827=CARTESIAN_POINT('Ctrl Pts',(6.44510892339048,-2.82954552561692,-14.788927602381));
#49828=CARTESIAN_POINT('Ctrl Pts',(6.41194011923371,-2.81727689091429,-14.801301031713));
#49829=CARTESIAN_POINT('Ctrl Pts',(6.36428119018118,-2.79964858004421,-14.8190799177978));
#49830=CARTESIAN_POINT('Ctrl Pts',(6.31562823555339,-2.78382801429811,-14.8365973961792));
#49831=CARTESIAN_POINT('Ctrl Pts',(6.26596696981809,-2.76988784963211,-14.8538446148066));
#49832=CARTESIAN_POINT('Ctrl Pts',(6.26065696768343,-2.76839730558258,-14.8556887636895));
#49833=CARTESIAN_POINT('Ctrl Pts',(6.25533542719756,-2.76692830682691,-14.8575298123915));
#49834=CARTESIAN_POINT('Ctrl Pts',(6.25000232416703,-2.76548097644809,-14.8593677423417));
#49835=CARTESIAN_POINT('',(6.99999610169145,-4.92964753519558,-14.7967972847303));
#49836=CARTESIAN_POINT('Ctrl Pts',(6.99999610169145,-4.92964753519558,-14.7967972847303));
#49837=CARTESIAN_POINT('Ctrl Pts',(6.99999610613836,-4.91661229043681,-14.791628391893));
#49838=CARTESIAN_POINT('Ctrl Pts',(7.00000000000004,-4.90361602938088,-14.7863598515099));
#49839=CARTESIAN_POINT('Ctrl Pts',(7.00000000000004,-4.68651912055677,-14.7023782689544));
#49840=CARTESIAN_POINT('Ctrl Pts',(7.,-4.37639477651136,-14.5833717164819));
#49841=CARTESIAN_POINT('Ctrl Pts',(7.,-3.62764529519874,-14.4736742989645));
#49842=CARTESIAN_POINT('Ctrl Pts',(7.,-3.36166428568053,-14.5001704079875));
#49843=CARTESIAN_POINT('Ctrl Pts',(7.,-3.16613006334553,-14.5427402348609));
#49844=CARTESIAN_POINT('Ctrl Pts',(6.9999961018476,-4.92964640469684,-14.7967897782623));
#49845=CARTESIAN_POINT('Ctrl Pts',(6.99999545357539,-4.90144163830488,-14.8174799284486));
#49846=CARTESIAN_POINT('Ctrl Pts',(6.99899242211926,-4.87385494684075,-14.8379871689643));
#49847=CARTESIAN_POINT('Ctrl Pts',(6.99710015379376,-4.84694425873787,-14.8582529829778));
#49848=CARTESIAN_POINT('Ctrl Pts',(6.99462095173791,-4.81168655645035,-14.8848047394535));
#49849=CARTESIAN_POINT('Ctrl Pts',(6.99061682905021,-4.77758978796254,-14.9109414498812));
#49850=CARTESIAN_POINT('Ctrl Pts',(6.98535378928391,-4.74472637574954,-14.9365584985346));
#49851=CARTESIAN_POINT('Ctrl Pts',(6.97984402030381,-4.71032233982514,-14.9633764642539));
#49852=CARTESIAN_POINT('Ctrl Pts',(6.9729541530082,-4.6772700776306,-14.9896249687013));
#49853=CARTESIAN_POINT('Ctrl Pts',(6.9649510374448,-4.64562082080034,-15.0152097168229));
#49854=CARTESIAN_POINT('Ctrl Pts',(6.96448148193806,-4.64376390861269,-15.0167108146483));
#49855=CARTESIAN_POINT('Ctrl Pts',(6.96400808470404,-4.64191181719858,-15.0182096344437));
#49856=CARTESIAN_POINT('Ctrl Pts',(6.96353089618533,-4.64006455362156,-15.0197061596802));
#49857=CARTESIAN_POINT('Ctrl Pts',(6.95827901842607,-4.61973379939072,-15.0361767311584));
#49858=CARTESIAN_POINT('Ctrl Pts',(6.9525684519033,-4.59998814679231,-15.0523690733808));
#49859=CARTESIAN_POINT('Ctrl Pts',(6.94647157041035,-4.58082833485301,-15.0682640391052));
#49860=CARTESIAN_POINT('Ctrl Pts',(6.93624916912817,-4.54870383212791,-15.0949145026561));
#49861=CARTESIAN_POINT('Ctrl Pts',(6.92494289805191,-4.51822761460672,-15.1207277618141));
#49862=CARTESIAN_POINT('Ctrl Pts',(6.91285653739889,-4.48938067867097,-15.1456340112259));
#49863=CARTESIAN_POINT('Ctrl Pts',(6.90347902408293,-4.46699904257488,-15.1649581644772));
#49864=CARTESIAN_POINT('Ctrl Pts',(6.89363089342732,-4.44559760714516,-15.1837368697021));
#49865=CARTESIAN_POINT('Ctrl Pts',(6.88343785827852,-4.42515687040387,-15.2019466950999));
#49866=CARTESIAN_POINT('Ctrl Pts',(6.87592821023104,-4.41009729918515,-15.2153626578379));
#49867=CARTESIAN_POINT('Ctrl Pts',(6.86823115088852,-4.39555891832723,-15.2284700122123));
#49868=CARTESIAN_POINT('Ctrl Pts',(6.86039673372419,-4.38152778746263,-15.2412620985545));
#49869=CARTESIAN_POINT('Ctrl Pts',(6.85503441981097,-4.37192409561483,-15.2500177189322));
#49870=CARTESIAN_POINT('Ctrl Pts',(6.84960766117097,-4.36255800803777,-15.2586256824296));
#49871=CARTESIAN_POINT('Ctrl Pts',(6.84413136976615,-4.35342466366611,-15.2670843255968));
#49872=CARTESIAN_POINT('Ctrl Pts',(6.84139322406374,-4.34885799148029,-15.2713136471804));
#49873=CARTESIAN_POINT('Ctrl Pts',(6.83864268736027,-4.34434951010423,-15.2755056389739));
#49874=CARTESIAN_POINT('Ctrl Pts',(6.83588153604075,-4.33989857293696,-15.2796601323838));
#49875=CARTESIAN_POINT('Ctrl Pts',(6.83450096038099,-4.33767310435332,-15.2817373790888));
#49876=CARTESIAN_POINT('Ctrl Pts',(6.83311773059012,-4.33546202211664,-15.2838052512154));
#49877=CARTESIAN_POINT('Ctrl Pts',(6.83173206482601,-4.33326524533274,-15.2858637287704));
#49878=CARTESIAN_POINT('Ctrl Pts',(6.83065726241951,-4.33156129836729,-15.2874604028653));
#49879=CARTESIAN_POINT('Ctrl Pts',(6.83004028587927,-4.33058748223666,-15.2883741809166));
#49880=CARTESIAN_POINT('Ctrl Pts',(6.82881311612304,-4.32866432005909,-15.2901810082252));
#49881=CARTESIAN_POINT('Ctrl Pts',(6.82845818380387,-4.32810808698022,-15.2907035939586));
#49882=CARTESIAN_POINT('Ctrl Pts',(6.82805199550011,-4.32747259371732,-15.2913008776399));
#49883=CARTESIAN_POINT('Ctrl Pts',(6.82756797534166,-4.32671775049805,-15.2920109583931));
#49884=CARTESIAN_POINT('Ctrl Pts',(6.80355964120888,-4.28927606979582,-15.3272323343803));
#49885=CARTESIAN_POINT('Ctrl Pts',(6.77748021137456,-4.25387016495786,-15.3617950155865));
#49886=CARTESIAN_POINT('Ctrl Pts',(6.74960463512441,-4.22067176874938,-15.395577183151));
#49887=CARTESIAN_POINT('Ctrl Pts',(6.71795255192088,-4.18297574447406,-15.4339360665316));
#49888=CARTESIAN_POINT('Ctrl Pts',(6.6839859149371,-4.14812527207758,-15.4712883958782));
#49889=CARTESIAN_POINT('Ctrl Pts',(6.64816824301974,-4.11626345192712,-15.5074860027474));
#49890=CARTESIAN_POINT('Ctrl Pts',(6.62199446893495,-4.092980417662,-15.5339374144078));
#49891=CARTESIAN_POINT('Ctrl Pts',(6.59483098593749,-4.07129351351006,-15.5597726972291));
#49892=CARTESIAN_POINT('Ctrl Pts',(6.56684287796802,-4.05125841777049,-15.5849411778566));
#49893=CARTESIAN_POINT('Ctrl Pts',(6.5270962587532,-4.02280607214707,-15.6206835730485));
#49894=CARTESIAN_POINT('Ctrl Pts',(6.48568899948451,-3.99768436133919,-15.6550804830691));
#49895=CARTESIAN_POINT('Ctrl Pts',(6.4431438002412,-3.97592981096522,-15.688016124873));
#49896=CARTESIAN_POINT('Ctrl Pts',(6.41212103682534,-3.96006700431551,-15.7120318691121));
#49897=CARTESIAN_POINT('Ctrl Pts',(6.38049206287102,-3.94599472702329,-15.7352710976102));
#49898=CARTESIAN_POINT('Ctrl Pts',(6.34844350829305,-3.93372675932074,-15.7576954210374));
#49899=CARTESIAN_POINT('Ctrl Pts',(6.32053397916,-3.92304318227627,-15.7772236748456));
#49900=CARTESIAN_POINT('Ctrl Pts',(6.29230613452632,-3.91372773195061,-15.79613405827));
#49901=CARTESIAN_POINT('Ctrl Pts',(6.26389264427641,-3.90575590947883,-15.8144088685689));
#49902=CARTESIAN_POINT('Ctrl Pts',(6.9993386693906,-9.44604681400665,-24.824660272019));
#49903=CARTESIAN_POINT('Ctrl Pts',(6.9993386693906,-9.4152902963795,-24.8024268448143));
#49904=CARTESIAN_POINT('Ctrl Pts',(6.9993386693906,-8.9165030314828,-24.437914914655));
#49905=CARTESIAN_POINT('Ctrl Pts',(6.9993386693906,-8.00787683705666,-23.6489663151524));
#49906=CARTESIAN_POINT('Ctrl Pts',(6.9993386693906,-6.88744313917509,-22.3090627902165));
#49907=CARTESIAN_POINT('Ctrl Pts',(6.9993386693906,-5.99155649181728,-20.8064994919115));
#49908=CARTESIAN_POINT('Ctrl Pts',(6.9993386693906,-5.34582279737036,-19.1801225035148));
#49909=CARTESIAN_POINT('Ctrl Pts',(6.9993386693906,-4.96572780212844,-17.4735522140584));
#49910=CARTESIAN_POINT('Ctrl Pts',(6.9993386693906,-4.8759191278038,-15.9617953190228));
#49911=CARTESIAN_POINT('Ctrl Pts',(6.9993386693906,-4.9383180577078,-15.0338172904337));
#49912=CARTESIAN_POINT('Ctrl Pts',(6.9993386693906,-4.9783443035646,-14.6872933671644));
#49913=CARTESIAN_POINT('Ctrl Pts',(7.01706646970942,-9.16066152666895,-25.2195383971088));
#49914=CARTESIAN_POINT('Ctrl Pts',(7.01706646970942,-9.12853933592334,-25.196317292769));
#49915=CARTESIAN_POINT('Ctrl Pts',(7.01706646970942,-8.60761353833628,-24.815622075188));
#49916=CARTESIAN_POINT('Ctrl Pts',(7.01706646970942,-7.65890581809753,-23.9919035502457));
#49917=CARTESIAN_POINT('Ctrl Pts',(7.01706646970942,-6.48824535535127,-22.5919646079468));
#49918=CARTESIAN_POINT('Ctrl Pts',(7.01706646970942,-5.552742828921,-21.0228679220168));
#49919=CARTESIAN_POINT('Ctrl Pts',(7.01706646970942,-4.87818323848258,-19.3240593792248));
#49920=CARTESIAN_POINT('Ctrl Pts',(7.01706646970942,-4.48117975208743,-17.5413569127717));
#49921=CARTESIAN_POINT('Ctrl Pts',(7.01706646970942,-4.38738464109396,-15.9624909042645));
#49922=CARTESIAN_POINT('Ctrl Pts',(7.01706646970942,-4.4525357174292,-14.9933640194634));
#49923=CARTESIAN_POINT('Ctrl Pts',(7.01706646970942,-4.49435138601102,-14.631371943798));
#49924=CARTESIAN_POINT('Ctrl Pts',(6.72658891709759,-8.93068742279116,-25.5377459115975));
#49925=CARTESIAN_POINT('Ctrl Pts',(6.72658891709759,-8.89746472174831,-25.5137289002038));
#49926=CARTESIAN_POINT('Ctrl Pts',(6.72658891709759,-8.35869886917577,-25.1199925862902));
#49927=CARTESIAN_POINT('Ctrl Pts',(6.72658891709759,-7.37769196117677,-24.2682551591898));
#49928=CARTESIAN_POINT('Ctrl Pts',(6.72658891709759,-6.16655689881398,-22.8199374394217));
#49929=CARTESIAN_POINT('Ctrl Pts',(6.72658891709759,-5.19913042013451,-21.197225669337));
#49930=CARTESIAN_POINT('Ctrl Pts',(6.72658891709759,-4.50134184805847,-19.4400490797251));
#49931=CARTESIAN_POINT('Ctrl Pts',(6.72658891709759,-4.09071286913051,-17.5959964667979));
#49932=CARTESIAN_POINT('Ctrl Pts',(6.72658891709759,-3.9937053388489,-15.963051432781));
#49933=CARTESIAN_POINT('Ctrl Pts',(6.72658891709759,-4.06107419738145,-14.960765265593));
#49934=CARTESIAN_POINT('Ctrl Pts',(6.72658891709759,-4.10433184950327,-14.5863083760655));
#49935=CARTESIAN_POINT('Ctrl Pts',(6.25330944738942,-8.85809586787838,-25.6381884304439));
#49936=CARTESIAN_POINT('Ctrl Pts',(6.25330944738942,-8.82452578966113,-25.6139201901951));
#49937=CARTESIAN_POINT('Ctrl Pts',(6.25330944738942,-8.28012870596488,-25.2160674412389));
#49938=CARTESIAN_POINT('Ctrl Pts',(6.25330944738942,-7.28892652718185,-24.355485819768));
#49939=CARTESIAN_POINT('Ctrl Pts',(6.25330944738942,-6.06501561714329,-22.8918972907141));
#49940=CARTESIAN_POINT('Ctrl Pts',(6.25330944738942,-5.08751231113854,-21.252261865925));
#49941=CARTESIAN_POINT('Ctrl Pts',(6.25330944738942,-4.38239148787448,-19.4766613441969));
#49942=CARTESIAN_POINT('Ctrl Pts',(6.25330944738942,-3.96746160866336,-17.6132434964464));
#49943=CARTESIAN_POINT('Ctrl Pts',(6.25330944738942,-3.86944007503447,-15.9632283641636));
#49944=CARTESIAN_POINT('Ctrl Pts',(6.25330944738942,-3.93750897872531,-14.950475436469));
#49945=CARTESIAN_POINT('Ctrl Pts',(6.25330944738942,-3.98122179438819,-14.5720840160315));
#49946=CARTESIAN_POINT('',(7.,-9.3325097692458,-24.7867247203242));
#49947=CARTESIAN_POINT('Ctrl Pts',(7.00000000000003,-9.3325097625576,-24.7867247293774));
#49948=CARTESIAN_POINT('Ctrl Pts',(7.00000000000003,-9.20047564887516,-24.6891826178643));
#49949=CARTESIAN_POINT('Ctrl Pts',(7.00000000006074,-9.07101759620012,-24.5890285581922));
#49950=CARTESIAN_POINT('Ctrl Pts',(6.99999999867344,-8.94403312611638,-24.4862283763798));
#49951=CARTESIAN_POINT('Ctrl Pts',(6.9999999972833,-8.816787959178,-24.3832171476257));
#49952=CARTESIAN_POINT('Ctrl Pts',(6.99999999422993,-8.69202620501044,-24.2775486102555));
#49953=CARTESIAN_POINT('Ctrl Pts',(6.99999999314803,-8.56967699865244,-24.1691471512216));
#49954=CARTESIAN_POINT('Ctrl Pts',(6.99999999206995,-8.44775837368218,-24.0611271875162));
#49955=CARTESIAN_POINT('Ctrl Pts',(6.99999999472217,-8.32823502604961,-23.9503931844797));
#49956=CARTESIAN_POINT('Ctrl Pts',(6.99999999803541,-8.21107368231993,-23.8368341942939));
#49957=CARTESIAN_POINT('Ctrl Pts',(6.99999999907234,-8.17440657537131,-23.8012944889135));
#49958=CARTESIAN_POINT('Ctrl Pts',(7.00000000000003,-8.13797110754852,-23.7654778407869));
#49959=CARTESIAN_POINT('Ctrl Pts',(7.00000000000003,-8.10176708255221,-23.7293801929953));
#49960=CARTESIAN_POINT('Ctrl Pts',(7.00000000000003,-8.07278510317455,-23.7004833705015));
#49961=CARTESIAN_POINT('Ctrl Pts',(6.99999999938399,-8.0439475664873,-23.671409737078));
#49962=CARTESIAN_POINT('Ctrl Pts',(6.99999999847202,-8.01525905976914,-23.6421620929155));
#49963=CARTESIAN_POINT('Ctrl Pts',(6.9999999941611,-7.87964747362771,-23.5039074442948));
#49964=CARTESIAN_POINT('Ctrl Pts',(6.99999998574664,-7.7473685255244,-23.3617612765062));
#49965=CARTESIAN_POINT('Ctrl Pts',(6.9999999850052,-7.61879186130439,-23.216052524166));
#49966=CARTESIAN_POINT('Ctrl Pts',(6.99999998426218,-7.48994339745887,-23.0700357564906));
#49967=CARTESIAN_POINT('Ctrl Pts',(6.99999998984224,-7.36481318793464,-22.9204416165475));
#49968=CARTESIAN_POINT('Ctrl Pts',(6.99999999473002,-7.24373815942285,-22.767639947986));
#49969=CARTESIAN_POINT('Ctrl Pts',(6.99999999759811,-7.17269293526201,-22.6779779513833));
#49970=CARTESIAN_POINT('Ctrl Pts',(7.00000000000003,-7.10304330304755,-22.5872122518149));
#49971=CARTESIAN_POINT('Ctrl Pts',(7.00000000000003,-7.03485110636723,-22.4954231417833));
#49972=CARTESIAN_POINT('Ctrl Pts',(7.00000000000003,-6.98781951651517,-22.4321169574095));
#49973=CARTESIAN_POINT('Ctrl Pts',(6.99999999890221,-6.9414866272677,-22.3683207500365));
#49974=CARTESIAN_POINT('Ctrl Pts',(6.99999999758213,-6.89585802963811,-22.3040438365628));
#49975=CARTESIAN_POINT('Ctrl Pts',(6.99999999346277,-6.75347250731112,-22.1034656383719));
#49976=CARTESIAN_POINT('Ctrl Pts',(6.99999998925871,-6.61794209682095,-21.898208866214));
#49977=CARTESIAN_POINT('Ctrl Pts',(6.99999999152161,-6.48945127241347,-21.6886107784926));
#49978=CARTESIAN_POINT('Ctrl Pts',(6.99999999354316,-6.37466462383332,-21.5013673535297));
#49979=CARTESIAN_POINT('Ctrl Pts',(7.00000000000003,-6.26549638305752,-21.3106585483591));
#49980=CARTESIAN_POINT('Ctrl Pts',(7.00000000000003,-6.16210765966451,-21.11670577957));
#49981=CARTESIAN_POINT('Ctrl Pts',(7.00000000000003,-6.10679638864214,-21.0129442298772));
#49982=CARTESIAN_POINT('Ctrl Pts',(6.9999999980303,-6.05312424078025,-20.9082598246668));
#49983=CARTESIAN_POINT('Ctrl Pts',(6.99999999636314,-6.00113654312204,-20.8027188607212));
#49984=CARTESIAN_POINT('Ctrl Pts',(6.99999999271528,-5.8873843169222,-20.5717888494901));
#49985=CARTESIAN_POINT('Ctrl Pts',(6.99999999204984,-5.78169965820049,-20.3367563671334));
#49986=CARTESIAN_POINT('Ctrl Pts',(6.99999999506637,-5.6843830048425,-20.0983727638304));
#49987=CARTESIAN_POINT('Ctrl Pts',(6.99999999705719,-5.62015694177595,-19.9410467583477));
#49988=CARTESIAN_POINT('Ctrl Pts',(7.00000000000003,-5.55957473197771,-19.782261714332));
#49989=CARTESIAN_POINT('Ctrl Pts',(7.00000000000003,-5.5027113982491,-19.6222387061761));
#49990=CARTESIAN_POINT('Ctrl Pts',(7.00000000000003,-5.45028577156463,-19.4747041538307));
#49991=CARTESIAN_POINT('Ctrl Pts',(6.99999999722477,-5.40103410796304,-19.3261153637749));
#49992=CARTESIAN_POINT('Ctrl Pts',(6.99999999446467,-5.3549894682949,-19.176560385357));
#49993=CARTESIAN_POINT('Ctrl Pts',(6.99999999008271,-5.28188871907092,-18.939125994485));
#49994=CARTESIAN_POINT('Ctrl Pts',(6.99999998784245,-5.21686862674689,-18.6992564658101));
#49995=CARTESIAN_POINT('Ctrl Pts',(6.99999999262694,-5.160067507945,-18.4573202583932));
#49996=CARTESIAN_POINT('Ctrl Pts',(6.99999999531402,-5.12816673181356,-18.3214434842435));
#49997=CARTESIAN_POINT('Ctrl Pts',(7.00000000000003,-5.09885930665234,-18.1849147103942));
#49998=CARTESIAN_POINT('Ctrl Pts',(7.00000000000003,-5.07217694828604,-18.0477988967269));
#49999=CARTESIAN_POINT('Ctrl Pts',(7.00000000000003,-5.03493020649233,-17.8563946273819));
#50000=CARTESIAN_POINT('Ctrl Pts',(6.99999999014834,-5.00273496135442,-17.6638469339319));
#50001=CARTESIAN_POINT('Ctrl Pts',(6.99999998525275,-4.97570204626941,-17.4706101632764));
#50002=CARTESIAN_POINT('Ctrl Pts',(6.99999998003397,-4.94688448272432,-17.2646163627521));
#50003=CARTESIAN_POINT('Ctrl Pts',(6.99999998145001,-4.92393390756773,-17.0578398871184));
#50004=CARTESIAN_POINT('Ctrl Pts',(6.99999998835933,-4.90684079792026,-16.8508352932017));
#50005=CARTESIAN_POINT('Ctrl Pts',(6.99999999308633,-4.89514657809842,-16.7092134774339));
#50006=CARTESIAN_POINT('Ctrl Pts',(7.00000000000003,-4.88619290480723,-16.5674849963347));
#50007=CARTESIAN_POINT('Ctrl Pts',(7.00000000000003,-4.87996268171837,-16.4258270845899));
#50008=CARTESIAN_POINT('Ctrl Pts',(7.00000000000003,-4.87263517759921,-16.2592200599269));
#50009=CARTESIAN_POINT('Ctrl Pts',(6.99999999283354,-4.86914729178053,-16.0927259175112));
#50010=CARTESIAN_POINT('Ctrl Pts',(6.9999999915726,-4.8694498897709,-15.9262297382788));
#50011=CARTESIAN_POINT('Ctrl Pts',(6.99999999107899,-4.86956834344757,-15.8610538772038));
#50012=CARTESIAN_POINT('Ctrl Pts',(6.99999999110873,-4.87026820069051,-15.7958776284049));
#50013=CARTESIAN_POINT('Ctrl Pts',(6.99999999149977,-4.87154867710779,-15.730693883814));
#50014=CARTESIAN_POINT('Ctrl Pts',(6.99999999249444,-4.87480578700939,-15.5648879251355));
#50015=CARTESIAN_POINT('Ctrl Pts',(6.99999999551013,-4.88181602636915,-15.3990333262998));
#50016=CARTESIAN_POINT('Ctrl Pts',(6.99999999717036,-4.89260120199109,-15.2330487286309));
#50017=CARTESIAN_POINT('Ctrl Pts',(6.9999999986237,-4.9020424443407,-15.0877473568381));
#50018=CARTESIAN_POINT('Ctrl Pts',(6.99999999923216,-4.91437718871111,-14.9423461487223));
#50019=CARTESIAN_POINT('Ctrl Pts',(6.99999999922774,-4.92965270723262,-14.7967937941787));
#50020=CARTESIAN_POINT('',(6.27159471697144,-8.76071062883554,-25.5608579993264));
#50021=CARTESIAN_POINT('Origin',(5.999999877385,-9.33250977407517,-24.7867246592848));
#50022=CARTESIAN_POINT('Ctrl Pts',(6.27159470456775,-8.76071047658199,-25.5608577604381));
#50023=CARTESIAN_POINT('Ctrl Pts',(6.27193966902754,-8.57412214084626,-25.4228903789273));
#50024=CARTESIAN_POINT('Ctrl Pts',(6.2722578257168,-8.39339828136479,-25.280910205322));
#50025=CARTESIAN_POINT('Ctrl Pts',(6.27254917034707,-8.218616766293,-25.1354917691069));
#50026=CARTESIAN_POINT('Ctrl Pts',(6.27284515826574,-8.04104968080664,-24.9877557348695));
#50027=CARTESIAN_POINT('Ctrl Pts',(6.27311347268825,-7.8696158047382,-24.8364709589357));
#50028=CARTESIAN_POINT('Ctrl Pts',(6.27335411005216,-7.70435942652848,-24.6822005640585));
#50029=CARTESIAN_POINT('Ctrl Pts',(6.27354178927092,-7.57547176147274,-24.5618811476563));
#50030=CARTESIAN_POINT('Ctrl Pts',(6.2737126330027,-7.45034099758903,-24.4397448236428));
#50031=CARTESIAN_POINT('Ctrl Pts',(6.27386663991676,-7.32897316278584,-24.3160426977429));
#50032=CARTESIAN_POINT('Ctrl Pts',(6.27406868997597,-7.16974408948665,-24.1537511408067));
#50033=CARTESIAN_POINT('Ctrl Pts',(6.27424176006529,-7.01699206497253,-23.9887664745278));
#50034=CARTESIAN_POINT('Ctrl Pts',(6.27438584793179,-6.87061872077468,-23.8216766723927));
#50035=CARTESIAN_POINT('Ctrl Pts',(6.27447252014277,-6.7825717416733,-23.721168260856));
#50036=CARTESIAN_POINT('Ctrl Pts',(6.27454870572353,-6.69683228994838,-23.6198972266081));
#50037=CARTESIAN_POINT('Ctrl Pts',(6.2746144043227,-6.61337488394086,-23.517983465972));
#50038=CARTESIAN_POINT('Ctrl Pts',(6.27472591337913,-6.47172412252793,-23.3450070641982));
#50039=CARTESIAN_POINT('Ctrl Pts',(6.27480721185364,-6.33664862454043,-23.1701816545098));
#50040=CARTESIAN_POINT('Ctrl Pts',(6.27485829868477,-6.208004962577,-22.9940551660041));
#50041=CARTESIAN_POINT('Ctrl Pts',(6.27487121294748,-6.17548507417922,-22.9495320728125));
#50042=CARTESIAN_POINT('Ctrl Pts',(6.27488219659928,-6.14337608568578,-22.9049256021009));
#50043=CARTESIAN_POINT('Ctrl Pts',(6.27489124963109,-6.11167545340995,-22.8602441341454));
#50044=CARTESIAN_POINT('Ctrl Pts',(6.27492812701298,-5.98254342920341,-22.6782348810993));
#50045=CARTESIAN_POINT('Ctrl Pts',(6.27493296902064,-5.86018864921786,-22.494985184616));
#50046=CARTESIAN_POINT('Ctrl Pts',(6.27490577558772,-5.74438505523325,-22.3110381127273));
#50047=CARTESIAN_POINT('Ctrl Pts',(6.27488257621681,-5.64559022719756,-22.1541084466469));
#50048=CARTESIAN_POINT('Ctrl Pts',(6.27483606080642,-5.55156315842536,-21.9966702876301));
#50049=CARTESIAN_POINT('Ctrl Pts',(6.27476622982249,-5.46215438129282,-21.8390323218734));
#50050=CARTESIAN_POINT('Ctrl Pts',(6.27472435185156,-5.40853551529692,-21.7444960891583));
#50051=CARTESIAN_POINT('Ctrl Pts',(6.27467408861181,-5.35657744174566,-21.6498875004173));
#50052=CARTESIAN_POINT('Ctrl Pts',(6.27461544161658,-5.30624659063555,-21.555268783472));
#50053=CARTESIAN_POINT('Ctrl Pts',(6.27458611811897,-5.28108116508049,-21.5079594249993));
#50054=CARTESIAN_POINT('Ctrl Pts',(6.27455469605052,-5.25632255329401,-21.4606475301866));
#50055=CARTESIAN_POINT('Ctrl Pts',(6.27452117885621,-5.23196644431683,-21.4133405291976));
#50056=CARTESIAN_POINT('Ctrl Pts',(6.27450442025905,-5.21978838982823,-21.3896870287031));
#50057=CARTESIAN_POINT('Ctrl Pts',(6.27448713770267,-5.20771096158906,-21.3660347513678));
#50058=CARTESIAN_POINT('Ctrl Pts',(6.27446933118762,-5.19573361922136,-21.3423846150635));
#50059=CARTESIAN_POINT('Ctrl Pts',(6.27445391935991,-5.18536703504556,-21.321915038321));
#50060=CARTESIAN_POINT('Ctrl Pts',(6.27443872970706,-5.17546074577125,-21.3022173602556));
#50061=CARTESIAN_POINT('Ctrl Pts',(6.27442216598168,-5.16501365823709,-21.2812921859785));
#50062=CARTESIAN_POINT('Ctrl Pts',(6.27441959231268,-5.16339039144624,-21.2780408357447));
#50063=CARTESIAN_POINT('Ctrl Pts',(6.27441698546962,-5.16175415908346,-21.274759804579));
#50064=CARTESIAN_POINT('Ctrl Pts',(6.2744143394645,-5.16010130860683,-21.2714415407458));
#50065=CARTESIAN_POINT('Ctrl Pts',(6.27440279605979,-5.15289061886207,-21.2569653547084));
#50066=CARTESIAN_POINT('Ctrl Pts',(6.27439106278321,-5.14570487770957,-21.2424654747839));
#50067=CARTESIAN_POINT('Ctrl Pts',(6.27437913963575,-5.13854426363549,-21.2279419562949));
#50068=CARTESIAN_POINT('Ctrl Pts',(6.274200106179,-5.03102320057894,-21.0098623152047));
#50069=CARTESIAN_POINT('Ctrl Pts',(6.27397826260158,-4.92916542322791,-20.7864491802973));
#50070=CARTESIAN_POINT('Ctrl Pts',(6.27371361318119,-4.83351359924625,-20.5579654055483));
#50071=CARTESIAN_POINT('Ctrl Pts',(6.27345238572287,-4.73909856963335,-20.3324359649062));
#50072=CARTESIAN_POINT('Ctrl Pts',(6.27314945222804,-4.65073004052687,-20.1019661153687));
#50073=CARTESIAN_POINT('Ctrl Pts',(6.27280481864902,-4.56895448022259,-19.8668529213087));
#50074=CARTESIAN_POINT('Ctrl Pts',(6.2726079764887,-4.52224725570509,-19.7325648198132));
#50075=CARTESIAN_POINT('Ctrl Pts',(6.27239753063306,-4.47769129316522,-19.5967627473317));
#50076=CARTESIAN_POINT('Ctrl Pts',(6.27217348248945,-4.4353920966628,-19.4595087727019));
#50077=CARTESIAN_POINT('Ctrl Pts',(6.27177013518626,-4.35924209353329,-19.2124144668563));
#50078=CARTESIAN_POINT('Ctrl Pts',(6.27132270305512,-4.29040493734449,-18.9606111698754));
#50079=CARTESIAN_POINT('Ctrl Pts',(6.27083119629828,-4.22947047044943,-18.7045320527505));
#50080=CARTESIAN_POINT('Ctrl Pts',(6.27036732545112,-4.17196216077399,-18.4628514749192));
#50081=CARTESIAN_POINT('Ctrl Pts',(6.26986419816364,-4.12149300234368,-18.217362749668));
#50082=CARTESIAN_POINT('Ctrl Pts',(6.26932182446785,-4.07857886873002,-17.9684779797761));
#50083=CARTESIAN_POINT('Ctrl Pts',(6.26905885247513,-4.05777178438981,-17.8478052325467));
#50084=CARTESIAN_POINT('Ctrl Pts',(6.26878665434446,-4.03874105556843,-17.7263348437419));
#50085=CARTESIAN_POINT('Ctrl Pts',(6.26850523144062,-4.02154717103653,-17.6041178806059));
#50086=CARTESIAN_POINT('Ctrl Pts',(6.26791730876932,-3.98562729960334,-17.3487935183506));
#50087=CARTESIAN_POINT('Ctrl Pts',(6.26728912556651,-3.95772395811605,-17.0902075422599));
#50088=CARTESIAN_POINT('Ctrl Pts',(6.26662069656093,-3.93824735949043,-16.8288449332124));
#50089=CARTESIAN_POINT('Ctrl Pts',(6.26595957943061,-3.91898381334836,-16.5703413425198));
#50090=CARTESIAN_POINT('Ctrl Pts',(6.2652590921452,-3.90796367252156,-16.3091214850602));
#50091=CARTESIAN_POINT('Ctrl Pts',(6.26451925231485,-3.90559010632334,-16.0457052708358));
#50092=CARTESIAN_POINT('Ctrl Pts',(6.26430324302721,-3.9048971018072,-15.9687962610009));
#50093=CARTESIAN_POINT('Ctrl Pts',(6.26408387915132,-3.9049412158933,-15.8917003575276));
#50094=CARTESIAN_POINT('Ctrl Pts',(6.26386116118544,-3.90573258304734,-15.8144313372742));
#50095=CARTESIAN_POINT('Ctrl Pts',(6.99999999998951,-10.9278021978185,-24.1259274559598));
#50096=CARTESIAN_POINT('Ctrl Pts',(6.99999999998951,-10.9277942568591,-24.1259309536957));
#50097=CARTESIAN_POINT('Ctrl Pts',(6.99999999998951,-10.6628645501556,-24.2426238189737));
#50098=CARTESIAN_POINT('Ctrl Pts',(6.99999999998951,-10.1334756387631,-24.4687760835904));
#50099=CARTESIAN_POINT('Ctrl Pts',(6.99999999998951,-9.59921869200086,-24.6831198888034));
#50100=CARTESIAN_POINT('Ctrl Pts',(6.99999999998951,-9.33250574064608,-24.7867214499183));
#50101=CARTESIAN_POINT('Ctrl Pts',(7.00000270572097,-11.1660644378211,-24.6668575634647));
#50102=CARTESIAN_POINT('Ctrl Pts',(7.00000270572097,-11.1660563761032,-24.6668611143908));
#50103=CARTESIAN_POINT('Ctrl Pts',(7.00000270572097,-10.8970978743297,-24.7853285323181));
#50104=CARTESIAN_POINT('Ctrl Pts',(7.00000270572097,-10.3596666804285,-25.0149163654536));
#50105=CARTESIAN_POINT('Ctrl Pts',(7.00000270572097,-9.81729343793422,-25.2325164806277));
#50106=CARTESIAN_POINT('Ctrl Pts',(7.00000270572097,-9.5465245747403,-25.3376935135454));
#50107=CARTESIAN_POINT('Ctrl Pts',(6.5796719778295,-11.3336093881581,-25.0472372157099));
#50108=CARTESIAN_POINT('Ctrl Pts',(6.5796719778295,-11.3336012415234,-25.0472408040392));
#50109=CARTESIAN_POINT('Ctrl Pts',(6.5796719778295,-11.0618097089271,-25.1669560795245));
#50110=CARTESIAN_POINT('Ctrl Pts',(6.5796719778295,-10.5187232176262,-25.3989597892034));
#50111=CARTESIAN_POINT('Ctrl Pts',(6.5796719778295,-9.97064263198303,-25.6188497270959));
#50112=CARTESIAN_POINT('Ctrl Pts',(6.5796719778295,-9.69702166956951,-25.7251346247928));
#50113=CARTESIAN_POINT('Ctrl Pts',(5.98852435812706,-11.3308746781034,-25.0410285650881));
#50114=CARTESIAN_POINT('Ctrl Pts',(5.98852435812706,-11.3308665328548,-25.0410321528068));
#50115=CARTESIAN_POINT('Ctrl Pts',(5.98852435812706,-11.0591212416852,-25.1607270604577));
#50116=CARTESIAN_POINT('Ctrl Pts',(5.98852435812706,-10.5161270575496,-25.3926913375982));
#50117=CARTESIAN_POINT('Ctrl Pts',(5.98852435812706,-9.96813962856907,-25.612543900438));
#50118=CARTESIAN_POINT('Ctrl Pts',(5.98852435812706,-9.69456521882714,-25.7188107152953));
#50119=CARTESIAN_POINT('',(6.99999999994032,-10.9277762174568,-24.1259366382796));
#50120=CARTESIAN_POINT('',(5.98852583803798,-11.3308502321837,-25.0410393004596));
#50121=CARTESIAN_POINT('Origin',(5.999999999061,-10.9277802195584,-24.1259421376201));
#50122=CARTESIAN_POINT('',(5.98852581355327,-9.69456736137568,-25.7188095579027));
#50123=CARTESIAN_POINT('Origin',(5.98846856056595,4.75314848987823,11.4751154608873));
#50124=CARTESIAN_POINT('Origin',(6.,-9.33250981979305,-24.7867247762541));
#50125=CARTESIAN_POINT('Origin',(6.99999997874466,4.74964867791879,11.46639970089));
#50126=CARTESIAN_POINT('Origin',(5.999999877385,-9.33250977407517,-24.7867246592848));
#50127=CARTESIAN_POINT('Origin',(5.99999764420532,-9.33250908124357,-24.7867226423044));
#50128=CARTESIAN_POINT('Ctrl Pts',(-6.09443191456128,-9.75587847514191,
-25.6959433244507));
#50129=CARTESIAN_POINT('Ctrl Pts',(-6.05633875294463,-9.74303070101173,
-25.700443119661));
#50130=CARTESIAN_POINT('Ctrl Pts',(-5.71232895595596,-9.62809884345565,
-25.7408006177088));
#50131=CARTESIAN_POINT('Ctrl Pts',(-5.02622191953824,-9.4183974530615,-25.8161825058434));
#50132=CARTESIAN_POINT('Ctrl Pts',(-3.98582966128773,-9.15597820979409,
-25.9131480292542));
#50133=CARTESIAN_POINT('Ctrl Pts',(-2.81226414604675,-8.93052993886067,
-25.9984040994506));
#50134=CARTESIAN_POINT('Ctrl Pts',(-1.52049089180403,-8.77111616050463,
-26.0601535869399));
#50135=CARTESIAN_POINT('Ctrl Pts',(-0.189402768854967,-8.70741653122222,
-26.0857988309911));
#50136=CARTESIAN_POINT('Ctrl Pts',(1.08608586087063,-8.74249055315278,-26.0715618637506));
#50137=CARTESIAN_POINT('Ctrl Pts',(2.24125031195963,-8.85308572724539,-26.0282772201452));
#50138=CARTESIAN_POINT('Ctrl Pts',(3.27297079110899,-9.01439205730505,-25.9665661311678));
#50139=CARTESIAN_POINT('Ctrl Pts',(4.19996253766372,-9.20867731868125,-25.8936091309432));
#50140=CARTESIAN_POINT('Ctrl Pts',(5.05700893778035,-9.42941774767843,-25.812292285677));
#50141=CARTESIAN_POINT('Ctrl Pts',(5.68046392620768,-9.6183284355846,-25.7443188151842));
#50142=CARTESIAN_POINT('Ctrl Pts',(6.02236021791466,-9.73156265908241,-25.7044579013743));
#50143=CARTESIAN_POINT('Ctrl Pts',(6.09429718633961,-9.75582422974853,-25.6959615814221));
#50144=CARTESIAN_POINT('Ctrl Pts',(-6.21850070569984,-9.42753381746598,
-25.836104681144));
#50145=CARTESIAN_POINT('Ctrl Pts',(-6.17967838293833,-9.41439786728843,
-25.8405746553953));
#50146=CARTESIAN_POINT('Ctrl Pts',(-5.82907993570433,-9.29687497796809,
-25.8806344898236));
#50147=CARTESIAN_POINT('Ctrl Pts',(-5.12974930543611,-9.08221820664856,
-25.9549339225927));
#50148=CARTESIAN_POINT('Ctrl Pts',(-4.06875950537382,-8.8130870839257,-26.0494404552579));
#50149=CARTESIAN_POINT('Ctrl Pts',(-2.87124953326329,-8.58145036507263,
-26.1316253526395));
#50150=CARTESIAN_POINT('Ctrl Pts',(-1.55244036708564,-8.41736480859588,
-26.1904032766854));
#50151=CARTESIAN_POINT('Ctrl Pts',(-0.193343137336627,-8.35164772530744,
-26.2143313324476));
#50152=CARTESIAN_POINT('Ctrl Pts',(1.10885789494489,-8.38784887380784,-26.2011016135553));
#50153=CARTESIAN_POINT('Ctrl Pts',(2.28833274099946,-8.5017594106142,-26.1601252018067));
#50154=CARTESIAN_POINT('Ctrl Pts',(3.34139710108736,-8.66764143052762,-26.1009947690095));
#50155=CARTESIAN_POINT('Ctrl Pts',(4.28714687780912,-8.86714807435702,-26.030425005036));
#50156=CARTESIAN_POINT('Ctrl Pts',(5.16111273668051,-9.09348349929248,-25.9510676829607));
#50157=CARTESIAN_POINT('Ctrl Pts',(5.79660262437972,-9.28687614882921,-25.8841068018567));
#50158=CARTESIAN_POINT('Ctrl Pts',(6.14504916278866,-9.40267148435833,-25.8445606466716));
#50159=CARTESIAN_POINT('Ctrl Pts',(6.21836333046621,-9.42747718413902,-25.8361202061885));
#50160=CARTESIAN_POINT('Ctrl Pts',(-6.32914064070096,-9.0707560819202,-25.7774948834612));
#50161=CARTESIAN_POINT('Ctrl Pts',(-6.28961409118642,-9.0574087794442,-25.7819223687199));
#50162=CARTESIAN_POINT('Ctrl Pts',(-5.93266456189295,-8.93800532070565,
-25.8215673303875));
#50163=CARTESIAN_POINT('Ctrl Pts',(-5.22080192937556,-8.72008792140814,
-25.8945057370815));
#50164=CARTESIAN_POINT('Ctrl Pts',(-4.14080030333458,-8.44715465611549,
-25.9860986694478));
#50165=CARTESIAN_POINT('Ctrl Pts',(-2.92180186623126,-8.21250760778291,
-26.0647484312864));
#50166=CARTESIAN_POINT('Ctrl Pts',(-1.57941028084733,-8.04654008989577,
-26.1201796098463));
#50167=CARTESIAN_POINT('Ctrl Pts',(-0.19661544115636,-7.98024992882376,
-26.1422128861359));
#50168=CARTESIAN_POINT('Ctrl Pts',(1.12798876719248,-8.01674575599185,-26.1300915415413));
#50169=CARTESIAN_POINT('Ctrl Pts',(2.32845989603055,-8.13187910606727,-26.0916963854716));
#50170=CARTESIAN_POINT('Ctrl Pts',(3.40038128787747,-8.29980004443677,-26.0355022183721));
#50171=CARTESIAN_POINT('Ctrl Pts',(4.36310376860213,-8.50197197562449,-25.9677006730754));
#50172=CARTESIAN_POINT('Ctrl Pts',(5.25272562824825,-8.73153230032595,-25.8906750740432));
#50173=CARTESIAN_POINT('Ctrl Pts',(5.89960821227025,-8.92785481431609,-25.8249809893108));
#50174=CARTESIAN_POINT('Ctrl Pts',(6.25435575265139,-9.04549377336416,-25.7858681030111));
#50175=CARTESIAN_POINT('Ctrl Pts',(6.32900000292914,-9.0706987506402,-25.777507429552));
#50176=CARTESIAN_POINT('Ctrl Pts',(-6.3948835674422,-8.78685861212201,-25.5363210765471));
#50177=CARTESIAN_POINT('Ctrl Pts',(-6.35487788533204,-8.77343700879775,
-25.5407054494319));
#50178=CARTESIAN_POINT('Ctrl Pts',(-5.99362001528234,-8.65339939708486,
-25.5799359505694));
#50179=CARTESIAN_POINT('Ctrl Pts',(-5.27347945378245,-8.43484642766188,
-25.6516208656583));
#50180=CARTESIAN_POINT('Ctrl Pts',(-4.18145742918569,-8.16210766130676,
-25.7406724567017));
#50181=CARTESIAN_POINT('Ctrl Pts',(-2.94953791498026,-7.92849091848468,
-25.8163265750121));
#50182=CARTESIAN_POINT('Ctrl Pts',(-1.59372603078983,-7.7639722778274,-25.8689859498486));
#50183=CARTESIAN_POINT('Ctrl Pts',(-0.198288364692249,-7.69871949889113,
-25.889484851852));
#50184=CARTESIAN_POINT('Ctrl Pts',(1.13803432083435,-7.73459195431683,-25.8782582937982));
#50185=CARTESIAN_POINT('Ctrl Pts',(2.35021414803826,-7.84850340786168,-25.841984575314));
#50186=CARTESIAN_POINT('Ctrl Pts',(3.43314197030597,-8.01534144112571,-25.7882487521332));
#50187=CARTESIAN_POINT('Ctrl Pts',(4.40622507863034,-8.21685948830795,-25.7228106836747));
#50188=CARTESIAN_POINT('Ctrl Pts',(5.30578804040778,-8.44635294622799,-25.6478272923519));
#50189=CARTESIAN_POINT('Ctrl Pts',(5.9601824771856,-8.64321722847831,-25.5832948261093));
#50190=CARTESIAN_POINT('Ctrl Pts',(6.31919080554775,-8.76145685074049,-25.5446108733089));
#50191=CARTESIAN_POINT('Ctrl Pts',(6.39473997725938,-8.78680247499924,-25.5363312425679));
#50192=CARTESIAN_POINT('',(-5.98852245733357,-9.69456809190394,-25.718809606518));
#50193=CARTESIAN_POINT('Ctrl Pts',(-5.98852261948844,-9.6945676514372,-25.7188097472701));
#50194=CARTESIAN_POINT('Ctrl Pts',(-5.87206434363686,-9.65602090275627,
-25.732349267617));
#50195=CARTESIAN_POINT('Ctrl Pts',(-5.74891036679771,-9.61638755853972,
-25.7463704895299));
#50196=CARTESIAN_POINT('Ctrl Pts',(-5.61905842363419,-9.57605268651985,
-25.7607445054415));
#50197=CARTESIAN_POINT('Ctrl Pts',(-5.51153067647356,-9.5426522012083,-25.7726473350102));
#50198=CARTESIAN_POINT('Ctrl Pts',(-5.39940999121403,-9.50877138149677,
-25.7847917051554));
#50199=CARTESIAN_POINT('Ctrl Pts',(-5.28269811078158,-9.47465117482898,
-25.7970892678802));
#50200=CARTESIAN_POINT('Ctrl Pts',(-5.21045748173724,-9.45353194357617,
-25.8047010351112));
#50201=CARTESIAN_POINT('Ctrl Pts',(-5.13645747597292,-9.43232409335956,
-25.8123701755227));
#50202=CARTESIAN_POINT('Ctrl Pts',(-5.06069821747161,-9.41109583723057,
-25.8200701491049));
#50203=CARTESIAN_POINT('Ctrl Pts',(-5.00135512738415,-9.39446750241339,
-25.8261016261151));
#50204=CARTESIAN_POINT('Ctrl Pts',(-4.940932629606,-9.3778267010815,-25.8321519616997));
#50205=CARTESIAN_POINT('Ctrl Pts',(-4.87943059212148,-9.36120808501283,
-25.8382085024417));
#50206=CARTESIAN_POINT('Ctrl Pts',(-4.80942185399454,-9.34229085254428,
-25.8451027581786));
#50207=CARTESIAN_POINT('Ctrl Pts',(-4.73801437156246,-9.32340262460789,
-25.8520049648563));
#50208=CARTESIAN_POINT('Ctrl Pts',(-4.66520814401506,-9.30459812859164,
-25.8588947595222));
#50209=CARTESIAN_POINT('Ctrl Pts',(-4.62880503024137,-9.29519588058352,
-25.8623396568552));
#50210=CARTESIAN_POINT('Ctrl Pts',(-4.59205223023201,-9.28581456359189,
-25.8657814461128));
#50211=CARTESIAN_POINT('Ctrl Pts',(-4.55494974405073,-9.27646135470819,
-25.8692174200576));
#50212=CARTESIAN_POINT('Ctrl Pts',(-4.53639850096009,-9.27178475026633,
-25.87093540703));
#50213=CARTESIAN_POINT('Ctrl Pts',(-4.51775983632789,-9.26711517272567,
-25.8726519398435));
#50214=CARTESIAN_POINT('Ctrl Pts',(-4.49903375016761,-9.2624535265998,-25.8743666750007));
#50215=CARTESIAN_POINT('Ctrl Pts',(-4.48967070708747,-9.26012270353686,
-25.8752240425794));
#50216=CARTESIAN_POINT('Ctrl Pts',(-4.48028580862534,-9.25779386331942,
-25.8760809607221));
#50217=CARTESIAN_POINT('Ctrl Pts',(-4.47087905478302,-9.25546712013321,
-25.8769373859222));
#50218=CARTESIAN_POINT('Ctrl Pts',(-4.4614723009407,-9.253140376947,-25.8777938111223));
#50219=CARTESIAN_POINT('Ctrl Pts',(-4.45080026163539,-9.25051015999041,
-25.8787622907533));
#50220=CARTESIAN_POINT('Ctrl Pts',(-4.4425932271173,-9.24849329615969,-25.8795051389721));
#50221=CARTESIAN_POINT('Ctrl Pts',(-4.30856578830439,-9.21555629643465,
-25.8916364446181));
#50222=CARTESIAN_POINT('Ctrl Pts',(-4.17021571232035,-9.18297044935259,
-25.9036951620593));
#50223=CARTESIAN_POINT('Ctrl Pts',(-4.02753511601077,-9.15105931833411,
-25.9155534623622));
#50224=CARTESIAN_POINT('Ctrl Pts',(-3.89063485291537,-9.12044098378059,
-25.9269313544744));
#50225=CARTESIAN_POINT('Ctrl Pts',(-3.74974763042379,-9.09044397683782,
-25.9381245168833));
#50226=CARTESIAN_POINT('Ctrl Pts',(-3.60488117560292,-9.06137189871749,
-25.9490157809797));
#50227=CARTESIAN_POINT('Ctrl Pts',(-3.4569563761102,-9.03168606612013,-25.9601369757358));
#50228=CARTESIAN_POINT('Ctrl Pts',(-3.30487851538804,-9.00296562174038,
-25.9709430808878));
#50229=CARTESIAN_POINT('Ctrl Pts',(-3.14864759357098,-8.97555104598866,
-25.9812999739124));
#50230=CARTESIAN_POINT('Ctrl Pts',(-3.07053213266245,-8.9618437581128,-25.9864784204247));
#50231=CARTESIAN_POINT('Ctrl Pts',(-2.99137840636983,-8.94846315819212,
-25.9915444311804));
#50232=CARTESIAN_POINT('Ctrl Pts',(-2.91118641383546,-8.93545291839981,
-25.9964804840002));
#50233=CARTESIAN_POINT('Ctrl Pts',(-2.89492183649935,-8.93281417549574,
-25.9974816165358));
#50234=CARTESIAN_POINT('Ctrl Pts',(-2.8786145518893,-8.93019066405754,-25.9984774035267));
#50235=CARTESIAN_POINT('Ctrl Pts',(-2.86226455462771,-8.92758275918284,
-25.9994676936367));
#50236=CARTESIAN_POINT('Ctrl Pts',(-2.83830797547962,-8.92376156713358,
-26.0009187008157));
#50237=CARTESIAN_POINT('Ctrl Pts',(-2.81425969566226,-8.91997388051614,
-26.0023579069037));
#50238=CARTESIAN_POINT('Ctrl Pts',(-2.79011972518663,-8.91622085219789,
-26.0037848560267));
#50239=CARTESIAN_POINT('Ctrl Pts',(-2.76981216043608,-8.91306364595109,
-26.0049852660165));
#50240=CARTESIAN_POINT('Ctrl Pts',(-2.74943970403522,-8.90993097041398,
-26.0061770006707));
#50241=CARTESIAN_POINT('Ctrl Pts',(-2.72900235599295,-8.90682351895854,
-26.007359785224));
#50242=CARTESIAN_POINT('Ctrl Pts',(-2.71878368197181,-8.90526979323082,
-26.0079511775006));
#50243=CARTESIAN_POINT('Ctrl Pts',(-2.70854878504028,-8.90372237351926,
-26.0085403322403));
#50244=CARTESIAN_POINT('Ctrl Pts',(-2.69829766519956,-8.90218134668462,
-26.0091272149495));
#50245=CARTESIAN_POINT('Ctrl Pts',(-2.68804654535884,-8.90064031984998,
-26.0097140976586));
#50246=CARTESIAN_POINT('Ctrl Pts',(-2.67637482465604,-8.8988969930817,-26.0103782308601));
#50247=CARTESIAN_POINT('Ctrl Pts',(-2.66749563695095,-8.89757753171104,
-26.0108810124235));
#50248=CARTESIAN_POINT('Ctrl Pts',(-2.4817721187646,-8.86997872244956,-26.021397555594));
#50249=CARTESIAN_POINT('Ctrl Pts',(-2.29115211002206,-8.84449825424844,
-26.031158807538));
#50250=CARTESIAN_POINT('Ctrl Pts',(-2.09562977114086,-8.82160895207015,
-26.0399712214066));
#50251=CARTESIAN_POINT('Ctrl Pts',(-1.9920271200296,-8.80948045360125,-26.044640710554));
#50252=CARTESIAN_POINT('Ctrl Pts',(-1.88704839731678,-8.79808016320673,
-26.0490434488219));
#50253=CARTESIAN_POINT('Ctrl Pts',(-1.78069528279165,-8.78748324876857,
-26.0531481972549));
#50254=CARTESIAN_POINT('Ctrl Pts',(-1.69992409241387,-8.77943529081903,
-26.0562655993038));
#50255=CARTESIAN_POINT('Ctrl Pts',(-1.61836026565276,-8.7718494917914,-26.059211532594));
#50256=CARTESIAN_POINT('Ctrl Pts',(-1.53600234381161,-8.76475689540864,
-26.0619727221466));
#50257=CARTESIAN_POINT('Ctrl Pts',(-1.4618110337009,-8.75836760090048,-26.0644601121366));
#50258=CARTESIAN_POINT('Ctrl Pts',(-1.38697529445642,-8.75237857171189,
-26.0667975749014));
#50259=CARTESIAN_POINT('Ctrl Pts',(-1.31149638803829,-8.74681213319418,
-26.0689746055433));
#50260=CARTESIAN_POINT('Ctrl Pts',(-1.23186330964479,-8.74093933169387,
-26.0712714545571));
#50261=CARTESIAN_POINT('Ctrl Pts',(-1.15151359812717,-8.73553695291215,
-26.0733897207682));
#50262=CARTESIAN_POINT('Ctrl Pts',(-1.07044725193411,-8.730630679564,-26.075316971428));
#50263=CARTESIAN_POINT('Ctrl Pts',(-1.02991407883757,-8.72817754288992,
-26.076280596758));
#50264=CARTESIAN_POINT('Ctrl Pts',(-0.98920174707087,-8.72584843119376,
-26.0771964639889));
#50265=CARTESIAN_POINT('Ctrl Pts',(-0.948310256537152,-8.72364651475522,
-26.0780630037134));
#50266=CARTESIAN_POINT('Ctrl Pts',(-0.927864511270293,-8.72254555653596,
-26.0784962735757));
#50267=CARTESIAN_POINT('Ctrl Pts',(-0.907373976312124,-8.72147639704049,
-26.0789172112858));
#50268=CARTESIAN_POINT('Ctrl Pts',(-0.88683865166021,-8.72043942951786,
-26.0793256198315));
#50269=CARTESIAN_POINT('Ctrl Pts',(-0.876570989334252,-8.71992094575655,
-26.0795298241043));
#50270=CARTESIAN_POINT('Ctrl Pts',(-0.866292129584895,-8.71941050998264,
-26.0797308960684));
#50271=CARTESIAN_POINT('Ctrl Pts',(-0.856002072412508,-8.71890817113153,
-26.0799288110538));
#50272=CARTESIAN_POINT('Ctrl Pts',(-0.845712015240121,-8.71840583228042,
-26.0801267260392));
#50273=CARTESIAN_POINT('Ctrl Pts',(-0.833723425538011,-8.71783205476417,
-26.0803528299732));
#50274=CARTESIAN_POINT('Ctrl Pts',(-0.825098308626926,-8.717425494198,-26.080513060353));
#50275=CARTESIAN_POINT('Ctrl Pts',(-0.603312001943076,-8.70697119342208,
-26.0846332252766));
#50276=CARTESIAN_POINT('Ctrl Pts',(-0.379421475271433,-8.70066427031859,
-26.0871466546555));
#50277=CARTESIAN_POINT('Ctrl Pts',(-0.1534220406775,-8.69871630031096,-26.0879154399325));
#50278=CARTESIAN_POINT('Ctrl Pts',(-0.0981746734312987,-8.69824010348069,
-26.0881033756351));
#50279=CARTESIAN_POINT('Ctrl Pts',(-0.0428013132975154,-8.69802458934256,
-26.088186939491));
#50280=CARTESIAN_POINT('Ctrl Pts',(0.0126974846559747,-8.69807140240537,
-26.0881659825254));
#50281=CARTESIAN_POINT('Ctrl Pts',(0.153960862518239,-8.69819055762358,
-26.088112639897));
#50282=CARTESIAN_POINT('Ctrl Pts',(0.29603961296522,-8.7000139697725,-26.0873805428933));
#50283=CARTESIAN_POINT('Ctrl Pts',(0.438933750157111,-8.70358140100969,
-26.0859632058811));
#50284=CARTESIAN_POINT('Ctrl Pts',(0.510380818753056,-8.70536511662828,
-26.085254537375));
#50285=CARTESIAN_POINT('Ctrl Pts',(0.582031733559519,-8.70758483852733,
-26.0843745626165));
#50286=CARTESIAN_POINT('Ctrl Pts',(0.653886494540562,-8.71024420963292,
-26.0833229538545));
#50287=CARTESIAN_POINT('Ctrl Pts',(0.689813875031083,-8.71157389518571,
-26.0827971494734));
#50288=CARTESIAN_POINT('Ctrl Pts',(0.725792217051223,-8.71301349319521,
-26.0822284370765));
#50289=CARTESIAN_POINT('Ctrl Pts',(0.761821520526584,-8.71456341919052,
-26.0816167928097));
#50290=CARTESIAN_POINT('Ctrl Pts',(0.779836172264264,-8.71533838218817,
-26.0813109706763));
#50291=CARTESIAN_POINT('Ctrl Pts',(0.797863564365103,-8.71614092719457,
-26.080994415615));
#50292=CARTESIAN_POINT('Ctrl Pts',(0.81590369681761,-8.71697110131534,-26.0806671265482));
#50293=CARTESIAN_POINT('Ctrl Pts',(0.833943829270117,-8.7178012754361,-26.0803398374813));
#50294=CARTESIAN_POINT('Ctrl Pts',(0.853616708032527,-8.71873848300525,
-26.0799705399663));
#50295=CARTESIAN_POINT('Ctrl Pts',(0.870062315217264,-8.71954455667472,
-26.0796530569462));
#50296=CARTESIAN_POINT('Ctrl Pts',(0.954906881865696,-8.72370317303982,
-26.0780151296288));
#50297=CARTESIAN_POINT('Ctrl Pts',(1.03913119420662,-8.72843365652,-26.0761559642982));
#50298=CARTESIAN_POINT('Ctrl Pts',(1.12272942609343,-8.7337099482048,-26.0740877362734));
#50299=CARTESIAN_POINT('Ctrl Pts',(1.34022986286555,-8.74743746037918,-26.0687067552576));
#50300=CARTESIAN_POINT('Ctrl Pts',(1.55349103100834,-8.76485636048876,-26.0619123572394));
#50301=CARTESIAN_POINT('Ctrl Pts',(1.76251272652862,-8.78549453835477,-26.0539173562375));
#50302=CARTESIAN_POINT('Ctrl Pts',(1.93917900970795,-8.80293803945215,-26.0471599375518));
#50303=CARTESIAN_POINT('Ctrl Pts',(2.11281718314964,-8.82268213996404,-26.0395443778246));
#50304=CARTESIAN_POINT('Ctrl Pts',(2.28343846123769,-8.84446515591452,-26.0311863868139));
#50305=CARTESIAN_POINT('Ctrl Pts',(2.3146215842016,-8.84844626819149,-26.0296588618514));
#50306=CARTESIAN_POINT('Ctrl Pts',(2.34570396261418,-8.85249553939135,-26.0281065081374));
#50307=CARTESIAN_POINT('Ctrl Pts',(2.37668569270351,-8.85661137768177,-26.0265300027406));
#50308=CARTESIAN_POINT('Ctrl Pts',(2.47745093085241,-8.86999776457236,-26.0214025633981));
#50309=CARTESIAN_POINT('Ctrl Pts',(2.57802291569005,-8.8842004818162,-26.015976492447));
#50310=CARTESIAN_POINT('Ctrl Pts',(2.67763152738052,-8.89908328647086,-26.0103066010436));
#50311=CARTESIAN_POINT('Ctrl Pts',(2.77938427561843,-8.9142864526369,-26.0045146617453));
#50312=CARTESIAN_POINT('Ctrl Pts',(2.88013158172736,-8.9301992170122,-25.9984683577212));
#50313=CARTESIAN_POINT('Ctrl Pts',(2.97906278137935,-8.94662576433618,-25.9922440351348));
#50314=CARTESIAN_POINT('Ctrl Pts',(3.01306549452358,-8.95227157858459,-25.990104731698));
#50315=CARTESIAN_POINT('Ctrl Pts',(3.04685376840857,-8.95797766172956,-25.9879445467223));
#50316=CARTESIAN_POINT('Ctrl Pts',(3.08039500479343,-8.96373477115169,-25.9857670260623));
#50317=CARTESIAN_POINT('Ctrl Pts',(3.15894907803007,-8.97721800683175,-25.9806672403705));
#50318=CARTESIAN_POINT('Ctrl Pts',(3.23636199036927,-8.99101552360982,-25.9754593206734));
#50319=CARTESIAN_POINT('Ctrl Pts',(3.31263226361224,-9.00508247212714,-25.9701607458246));
#50320=CARTESIAN_POINT('Ctrl Pts',(3.45643416232766,-9.03160465200025,-25.9601706790353));
#50321=CARTESIAN_POINT('Ctrl Pts',(3.59617380830651,-9.05908323278079,-25.9498590854424));
#50322=CARTESIAN_POINT('Ctrl Pts',(3.73185545191301,-9.0872291360773,-25.9393395658838));
#50323=CARTESIAN_POINT('Ctrl Pts',(3.83567798231805,-9.10876616071162,-25.9312901119548));
#50324=CARTESIAN_POINT('Ctrl Pts',(3.93712340771991,-9.13069417429627,-25.9231187412403));
#50325=CARTESIAN_POINT('Ctrl Pts',(4.03619172746806,-9.15289058487712,-25.9148725074305));
#50326=CARTESIAN_POINT('Ctrl Pts',(4.0609588074051,-9.15843968752233,-25.9128109489781));
#50327=CARTESIAN_POINT('Ctrl Pts',(4.08659006974544,-9.16422980812985,-25.910661321275));
#50328=CARTESIAN_POINT('Ctrl Pts',(4.11454679751779,-9.17061410451057,-25.9082932570447));
#50329=CARTESIAN_POINT('Ctrl Pts',(4.14250352529014,-9.17699840089129,-25.9059251928145));
#50330=CARTESIAN_POINT('Ctrl Pts',(4.17028169065756,-9.18340722888102,-25.90355006307));
#50331=CARTESIAN_POINT('Ctrl Pts',(4.19788129363969,-9.18983788987918,-25.9011688869911));
#50332=CARTESIAN_POINT('Ctrl Pts',(4.20564501959985,-9.19164682494845,-25.9004990658147));
#50333=CARTESIAN_POINT('Ctrl Pts',(4.21339461673097,-9.19345748825839,-25.8998287659398));
#50334=CARTESIAN_POINT('Ctrl Pts',(4.22113008445721,-9.19526982128289,-25.8991580094122));
#50335=CARTESIAN_POINT('Ctrl Pts',(4.26839290987553,-9.2063429693288,-25.8950597635421));
#50336=CARTESIAN_POINT('Ctrl Pts',(4.31512826475942,-9.21747842096176,-25.8909444866922));
#50337=CARTESIAN_POINT('Ctrl Pts',(4.36133616318358,-9.22866296308564,-25.8868173528634));
#50338=CARTESIAN_POINT('Ctrl Pts',(4.51929288752084,-9.26689611580086,-25.8727091903471));
#50339=CARTESIAN_POINT('Ctrl Pts',(4.67108689359218,-9.30569782268728,-25.8584650443958));
#50340=CARTESIAN_POINT('Ctrl Pts',(4.81671592687905,-9.34457708467627,-25.8442720103327));
#50341=CARTESIAN_POINT('Ctrl Pts',(4.86938363922463,-9.35863802939607,-25.8391390047879));
#50342=CARTESIAN_POINT('Ctrl Pts',(4.92124512535988,-9.37270953859383,-25.8340124451188));
#50343=CARTESIAN_POINT('Ctrl Pts',(4.97230066796867,-9.38676979635092,-25.8289003898528));
#50344=CARTESIAN_POINT('Ctrl Pts',(5.00457274340919,-9.39565724864042,-25.8256690730404));
#50345=CARTESIAN_POINT('Ctrl Pts',(5.03652276008337,-9.40453935274694,-25.8224438719359));
#50346=CARTESIAN_POINT('Ctrl Pts',(5.06815068241344,-9.41341134502733,-25.8192265142138));
#50347=CARTESIAN_POINT('Ctrl Pts',(5.21038996184149,-9.45331108222424,-25.8047571905804));
#50348=CARTESIAN_POINT('Ctrl Pts',(5.34611446592922,-9.49300293214208,-25.7904489428062));
#50349=CARTESIAN_POINT('Ctrl Pts',(5.47532374055758,-9.53208408751539,-25.7764525725624));
#50350=CARTESIAN_POINT('Ctrl Pts',(5.60704945441462,-9.57192637518952,-25.7621836134101));
#50351=CARTESIAN_POINT('Ctrl Pts',(5.73200388397534,-9.6111339299822,-25.7482386066609));
#50352=CARTESIAN_POINT('Ctrl Pts',(5.85018857600751,-9.64932450496305,-25.7347472541537));
#50353=CARTESIAN_POINT('Ctrl Pts',(5.86232648746063,-9.65324678803957,-25.7333616530298));
#50354=CARTESIAN_POINT('Ctrl Pts',(5.87439299269056,-9.65715838230777,-25.7319808128288));
#50355=CARTESIAN_POINT('Ctrl Pts',(5.88638809326722,-9.66105889975959,-25.7306048578009));
#50356=CARTESIAN_POINT('Ctrl Pts',(5.92102969266071,-9.67232351251794,-25.726631128481));
#50357=CARTESIAN_POINT('Ctrl Pts',(5.95507574029098,-9.68349572625319,-25.7226981598991));
#50358=CARTESIAN_POINT('Ctrl Pts',(5.98852582161058,-9.69456702968901,-25.7188089328263));
#50359=CARTESIAN_POINT('',(-6.27159361730922,-8.76070973783752,-25.5608563036425));
#50360=CARTESIAN_POINT('Origin',(-5.9999949808,-9.33250914740362,-24.7867195890602));
#50361=CARTESIAN_POINT('Ctrl Pts',(-6.27159386307039,-8.76070927462836,
-25.56085716797));
#50362=CARTESIAN_POINT('Ctrl Pts',(-6.19708064101881,-8.73626652885538,
-25.5689447883498));
#50363=CARTESIAN_POINT('Ctrl Pts',(-6.11543892747885,-8.70997409384621,
-25.5777035213267));
#50364=CARTESIAN_POINT('Ctrl Pts',(-6.02658468999164,-8.68208172222085,
-25.5870520415819));
#50365=CARTESIAN_POINT('Ctrl Pts',(-5.93855992585843,-8.6544497318637,-25.5963132913965));
#50366=CARTESIAN_POINT('Ctrl Pts',(-5.8434565165779,-8.62524745650439,-25.6061534758547));
#50367=CARTESIAN_POINT('Ctrl Pts',(-5.74118378182371,-8.59476439466987,
-25.6164754166227));
#50368=CARTESIAN_POINT('Ctrl Pts',(-5.6404952869802,-8.56475352596948,-25.6266374669707));
#50369=CARTESIAN_POINT('Ctrl Pts',(-5.53285768868566,-8.5335011967807,-25.6372665625407));
#50370=CARTESIAN_POINT('Ctrl Pts',(-5.41817810268241,-8.50132997649802,
-25.6482508431793));
#50371=CARTESIAN_POINT('Ctrl Pts',(-5.37925207454577,-8.49041000486612,
-25.6519792697642));
#50372=CARTESIAN_POINT('Ctrl Pts',(-5.33951466255555,-8.4793845652548,-25.6557484475657));
#50373=CARTESIAN_POINT('Ctrl Pts',(-5.29896211848324,-8.46826753089785,
-25.6595534564569));
#50374=CARTESIAN_POINT('Ctrl Pts',(-5.21821342920711,-8.44613116501754,
-25.6671300336527));
#50375=CARTESIAN_POINT('Ctrl Pts',(-5.13423280764027,-8.42363090369957,
-25.6748488992373));
#50376=CARTESIAN_POINT('Ctrl Pts',(-5.04699090796374,-8.40088618384965,
-25.6826701541321));
#50377=CARTESIAN_POINT('Ctrl Pts',(-4.92201132303848,-8.36830292217578,
-25.6938746005504));
#50378=CARTESIAN_POINT('Ctrl Pts',(-4.79033868981777,-8.33521570366159,
-25.7052899395705));
#50379=CARTESIAN_POINT('Ctrl Pts',(-4.6518870917885,-8.30201778587879,-25.7167847294538));
#50380=CARTESIAN_POINT('Ctrl Pts',(-4.51343549375923,-8.268819868096,-25.728279519337));
#50381=CARTESIAN_POINT('Ctrl Pts',(-4.36820473336794,-8.23551097951922,
-25.7398538586143));
#50382=CARTESIAN_POINT('Ctrl Pts',(-4.21611190204717,-8.20253752415175,
-25.7513583798219));
#50383=CARTESIAN_POINT('Ctrl Pts',(-4.07082877172975,-8.17104039985229,
-25.7623478054201));
#50384=CARTESIAN_POINT('Ctrl Pts',(-3.91928373419016,-8.13984958966014,
-25.7732733247265));
#50385=CARTESIAN_POINT('Ctrl Pts',(-3.76142160008198,-8.10939970549724,
-25.7839928332117));
#50386=CARTESIAN_POINT('Ctrl Pts',(-3.73054732381349,-8.10344439429294,
-25.786089327525));
#50387=CARTESIAN_POINT('Ctrl Pts',(-3.69943145109153,-8.09751757244847,
-25.7881778959314));
#50388=CARTESIAN_POINT('Ctrl Pts',(-3.66807362440159,-8.09162271074323,
-25.7902574076099));
#50389=CARTESIAN_POINT('Ctrl Pts',(-3.58017497740066,-8.07509891356584,
-25.7960864551638));
#50390=CARTESIAN_POINT('Ctrl Pts',(-3.49037513070284,-8.05882589735015,
-25.8018444457918));
#50391=CARTESIAN_POINT('Ctrl Pts',(-3.39866711056178,-8.04288325223482,
-25.8075055234358));
#50392=CARTESIAN_POINT('Ctrl Pts',(-3.35281310049126,-8.03491192967715,
-25.8103360622577));
#50393=CARTESIAN_POINT('Ctrl Pts',(-3.30648203810739,-8.02702323593776,
-25.8131423273727));
#50394=CARTESIAN_POINT('Ctrl Pts',(-3.25967322192836,-8.01922760746874,
-25.8159209778804));
#50395=CARTESIAN_POINT('Ctrl Pts',(-3.23626881383885,-8.01532979323423,
-25.8173103031342));
#50396=CARTESIAN_POINT('Ctrl Pts',(-3.2127449667047,-8.01145524761749,-25.8186927218278));
#50397=CARTESIAN_POINT('Ctrl Pts',(-3.18910159680807,-8.00760529720807,
-25.8200678036269));
#50398=CARTESIAN_POINT('Ctrl Pts',(-3.17727991185975,-8.00568032200336,
-25.8207553445264));
#50399=CARTESIAN_POINT('Ctrl Pts',(-3.16542834618611,-8.00376149574843,
-25.8214410510163));
#50400=CARTESIAN_POINT('Ctrl Pts',(-3.153546889955,-8.00184898612967,-25.822124868798));
#50401=CARTESIAN_POINT('Ctrl Pts',(-3.1416654337239,-7.99993647651091,-25.8228086865797));
#50402=CARTESIAN_POINT('Ctrl Pts',(-3.12814004446228,-7.99777350884686,
-25.8235825260523));
#50403=CARTESIAN_POINT('Ctrl Pts',(-3.11781283988124,-7.99613057576302,
-25.8241706011561));
#50404=CARTESIAN_POINT('Ctrl Pts',(-3.07662101472709,-7.98957745562305,
-25.8265162394809));
#50405=CARTESIAN_POINT('Ctrl Pts',(-3.03568844271409,-7.98319675839628,
-25.8288016648055));
#50406=CARTESIAN_POINT('Ctrl Pts',(-2.99501685898111,-7.97698388940999,
-25.8310284388352));
#50407=CARTESIAN_POINT('Ctrl Pts',(-2.79740091933288,-7.94679667194882,
-25.8418479349523));
#50408=CARTESIAN_POINT('Ctrl Pts',(-2.60595036248865,-7.92057001971489,
-25.8512835464356));
#50409=CARTESIAN_POINT('Ctrl Pts',(-2.42085823916677,-7.89776613030724,
-25.8595190543067));
#50410=CARTESIAN_POINT('Ctrl Pts',(-2.23093018845681,-7.87436644054158,
-25.8679697324258));
#50411=CARTESIAN_POINT('Ctrl Pts',(-2.04769685011509,-7.85457034414563,
-25.8751568615175));
#50412=CARTESIAN_POINT('Ctrl Pts',(-1.87131799226574,-7.83781990485744,
-25.8812683924748));
#50413=CARTESIAN_POINT('Ctrl Pts',(-1.78117118814471,-7.82925879618565,
-25.8843919810433));
#50414=CARTESIAN_POINT('Ctrl Pts',(-1.69281417152675,-7.82149367808869,
-25.8872344244849));
#50415=CARTESIAN_POINT('Ctrl Pts',(-1.60626396048369,-7.81445276530423,
-25.8898196774583));
#50416=CARTESIAN_POINT('Ctrl Pts',(-1.43907018611961,-7.80085144915243,
-25.8948137519626));
#50417=CARTESIAN_POINT('Ctrl Pts',(-1.27862092923838,-7.78995013294518,
-25.8988490903609));
#50418=CARTESIAN_POINT('Ctrl Pts',(-1.12501574825844,-7.78123955773252,
-25.9020960152113));
#50419=CARTESIAN_POINT('Ctrl Pts',(-0.969938844053647,-7.7724455246849,
-25.9053740495248));
#50420=CARTESIAN_POINT('Ctrl Pts',(-0.821837400097612,-7.76588424261616,
-25.9078485020547));
#50421=CARTESIAN_POINT('Ctrl Pts',(-0.680781487683452,-7.76107119712844,
-25.9096791178162));
#50422=CARTESIAN_POINT('Ctrl Pts',(-0.538387209027835,-7.75621248451844,
-25.9115271028202));
#50423=CARTESIAN_POINT('Ctrl Pts',(-0.403172411170193,-7.75313516554023,
-25.9127189940968));
#50424=CARTESIAN_POINT('Ctrl Pts',(-0.275182242969547,-7.75138351950705,
-25.9134031520801));
#50425=CARTESIAN_POINT('Ctrl Pts',(-0.236222356389467,-7.75085032284248,
-25.9136114080564));
#50426=CARTESIAN_POINT('Ctrl Pts',(-0.197931723059676,-7.75044026708882,
-25.9137725064282));
#50427=CARTESIAN_POINT('Ctrl Pts',(-0.160311209414855,-7.75014131167927,
-25.9138903374117));
#50428=CARTESIAN_POINT('Ctrl Pts',(-0.153998804667823,-7.75009114948414,
-25.9139101084564));
#50429=CARTESIAN_POINT('Ctrl Pts',(-0.147705266086702,-7.75004411608126,
-25.9139286610374));
#50430=CARTESIAN_POINT('Ctrl Pts',(-0.141430596982659,-7.75000015410289,
-25.9139460130055));
#50431=CARTESIAN_POINT('Ctrl Pts',(-0.103047862356985,-7.74973123459157,
-25.9140521566089));
#50432=CARTESIAN_POINT('Ctrl Pts',(-0.0662557655660949,-7.7495797024787,
-25.9141126178867));
#50433=CARTESIAN_POINT('Ctrl Pts',(-0.0289811603192746,-7.74952611417544,
-25.9141334371331));
#50434=CARTESIAN_POINT('Ctrl Pts',(-0.0185590840463095,-7.7495111307469,
-25.9141392582484));
#50435=CARTESIAN_POINT('Ctrl Pts',(-0.00809928513411629,-7.74950410145234,
-25.9141418862787));
#50436=CARTESIAN_POINT('Ctrl Pts',(0.00244355322760035,-7.74950529241563,
-25.9141412344764));
#50437=CARTESIAN_POINT('Ctrl Pts',(0.127127957617791,-7.74951937728952,
-25.9141335259665));
#50438=CARTESIAN_POINT('Ctrl Pts',(0.258986367500759,-7.75068425897285,
-25.9136690002192));
#50439=CARTESIAN_POINT('Ctrl Pts',(0.397985564384329,-7.75344426614272,
-25.9126040413307));
#50440=CARTESIAN_POINT('Ctrl Pts',(0.535666614760285,-7.7561780998246,-25.9115491815786));
#50441=CARTESIAN_POINT('Ctrl Pts',(0.680353984971248,-7.76047708718023,
-25.9099052014884));
#50442=CARTESIAN_POINT('Ctrl Pts',(0.831993438911318,-7.76681627477429,
-25.907517222457));
#50443=CARTESIAN_POINT('Ctrl Pts',(0.942266724269816,-7.7714261769095,-25.9057806671851));
#50444=CARTESIAN_POINT('Ctrl Pts',(1.05621605154075,-7.77711589621786,-25.9036503474668));
#50445=CARTESIAN_POINT('Ctrl Pts',(1.17381162281563,-7.78408209266922,-25.9010616180959));
#50446=CARTESIAN_POINT('Ctrl Pts',(1.33437225434298,-7.79359347893528,-25.8975270630261));
#50447=CARTESIAN_POINT('Ctrl Pts',(1.50173206401884,-7.80548373360795,-25.8931383077185));
#50448=CARTESIAN_POINT('Ctrl Pts',(1.67578004007753,-7.82026797246305,-25.8877236195892));
#50449=CARTESIAN_POINT('Ctrl Pts',(1.84378667050358,-7.83453903846281,-25.8824968796522));
#50450=CARTESIAN_POINT('Ctrl Pts',(2.01802545152726,-7.85150699806721,-25.8763141118331));
#50451=CARTESIAN_POINT('Ctrl Pts',(2.1983598498116,-7.87166084096275,-25.8690099460407));
#50452=CARTESIAN_POINT('Ctrl Pts',(2.26108424604589,-7.87867080489336,-25.8664693914173));
#50453=CARTESIAN_POINT('Ctrl Pts',(2.32454574387929,-7.88606641066583,-25.8637930754091));
#50454=CARTESIAN_POINT('Ctrl Pts',(2.38873742215535,-7.8938688900564,-25.860973738592));
#50455=CARTESIAN_POINT('Ctrl Pts',(2.47500004738477,-7.90435408648068,-25.8571850326134));
#50456=CARTESIAN_POINT('Ctrl Pts',(2.56258134375727,-7.91557403890685,-25.8531380530837));
#50457=CARTESIAN_POINT('Ctrl Pts',(2.65146464458645,-7.92757931330867,-25.8488156636023));
#50458=CARTESIAN_POINT('Ctrl Pts',(2.72897721207415,-7.93804876745358,-25.8450462321875));
#50459=CARTESIAN_POINT('Ctrl Pts',(2.80747997437277,-7.94911552377676,-25.8410673744993));
#50460=CARTESIAN_POINT('Ctrl Pts',(2.88696064306362,-7.96081345283505,-25.8368674928884));
#50461=CARTESIAN_POINT('Ctrl Pts',(2.92670097740905,-7.9666624173642,-25.8347675520829));
#50462=CARTESIAN_POINT('Ctrl Pts',(2.96668578716397,-7.97266917986723,-25.8326123492592));
#50463=CARTESIAN_POINT('Ctrl Pts',(3.00691341526369,-7.97883801602081,-25.8304004296764));
#50464=CARTESIAN_POINT('Ctrl Pts',(3.02702722931355,-7.9819224340976,-25.829294469885));
#50465=CARTESIAN_POINT('Ctrl Pts',(3.04720174789494,-7.98504737087738,-25.8281743305421));
#50466=CARTESIAN_POINT('Ctrl Pts',(3.06743675928565,-7.98821336188863,-25.8270398278529));
#50467=CARTESIAN_POINT('Ctrl Pts',(3.07755426498101,-7.98979635739425,-25.8264725765082));
#50468=CARTESIAN_POINT('Ctrl Pts',(3.08768689387456,-7.99138961647581,-25.8259017343043));
#50469=CARTESIAN_POINT('Ctrl Pts',(3.09783461902328,-7.99299320618079,-25.8253272782121));
#50470=CARTESIAN_POINT('Ctrl Pts',(3.10798234417199,-7.99459679588577,-25.82475282212));
#50471=CARTESIAN_POINT('Ctrl Pts',(3.1164924327771,-7.99594695194843,-25.8242692123921));
#50472=CARTESIAN_POINT('Ctrl Pts',(3.12832305613581,-7.99783503428302,-25.8235930451759));
#50473=CARTESIAN_POINT('Ctrl Pts',(3.24396819272957,-8.01629116570257,-25.8169834652994));
#50474=CARTESIAN_POINT('Ctrl Pts',(3.35682173877642,-8.03535443277902,-25.8101924262962));
#50475=CARTESIAN_POINT('Ctrl Pts',(3.46689179392627,-8.05487866527595,-25.803267018375));
#50476=CARTESIAN_POINT('Ctrl Pts',(3.63912997498682,-8.08543028340038,-25.7924301049036));
#50477=CARTESIAN_POINT('Ctrl Pts',(3.80455199674186,-8.11710766108124,-25.7812651359542));
#50478=CARTESIAN_POINT('Ctrl Pts',(3.96321409892716,-8.14939039424876,-25.7699423194765));
#50479=CARTESIAN_POINT('Ctrl Pts',(4.12187620111246,-8.18167312741628,-25.7586195029989));
#50480=CARTESIAN_POINT('Ctrl Pts',(4.27377865492778,-8.21456150445218,-25.7471387505097));
#50481=CARTESIAN_POINT('Ctrl Pts',(4.41898996524078,-8.24759193080513,-25.7356524370349));
#50482=CARTESIAN_POINT('Ctrl Pts',(4.56351962868667,-8.28046730665551,-25.7242200422913));
#50483=CARTESIAN_POINT('Ctrl Pts',(4.70142133262044,-8.31348366819116,-25.7127822039499));
#50484=CARTESIAN_POINT('Ctrl Pts',(4.83277589947591,-8.34623514225956,-25.7014757980672));
#50485=CARTESIAN_POINT('Ctrl Pts',(4.90532428829938,-8.36432409593767,-25.6952311615098));
#50486=CARTESIAN_POINT('Ctrl Pts',(4.97587556693888,-8.38233314402035,-25.6890263039231));
#50487=CARTESIAN_POINT('Ctrl Pts',(5.04444365587221,-8.40020029078686,-25.6828820636048));
#50488=CARTESIAN_POINT('Ctrl Pts',(5.1353885124747,-8.42389826933422,-25.6747326888246));
#50489=CARTESIAN_POINT('Ctrl Pts',(5.22284458645003,-8.44734616967657,-25.6666901042532));
#50490=CARTESIAN_POINT('Ctrl Pts',(5.30684444827134,-8.47041101632681,-25.6587988967422));
#50491=CARTESIAN_POINT('Ctrl Pts',(5.42689921939801,-8.50337589062097,-25.6475205792412));
#50492=CARTESIAN_POINT('Ctrl Pts',(5.53989448481551,-8.53555643652212,-25.6365523846394));
#50493=CARTESIAN_POINT('Ctrl Pts',(5.6459272916651,-8.56661204936056,-25.626011907698));
#50494=CARTESIAN_POINT('Ctrl Pts',(5.75378657216675,-8.59820261227985,-25.6152898652205));
#50495=CARTESIAN_POINT('Ctrl Pts',(5.85444161366389,-8.62862920659797,-25.6050103186927));
#50496=CARTESIAN_POINT('Ctrl Pts',(5.94798721656892,-8.65758340246176,-25.5952771356166));
#50497=CARTESIAN_POINT('Ctrl Pts',(6.02496432786757,-8.6814093257372,-25.5872678621321));
#50498=CARTESIAN_POINT('Ctrl Pts',(6.09712726844943,-8.70423919491187,-25.5796281564338));
#50499=CARTESIAN_POINT('Ctrl Pts',(6.16452420707897,-8.72592546147543,-25.5724066590223));
#50500=CARTESIAN_POINT('Ctrl Pts',(6.20165893268432,-8.73787427657916,-25.5684277197665));
#50501=CARTESIAN_POINT('Ctrl Pts',(6.23734668826649,-8.74947631976018,-25.5645756231204));
#50502=CARTESIAN_POINT('Ctrl Pts',(6.27159479316261,-8.76071029005264,-25.5608580129605));
#50503=CARTESIAN_POINT('Ctrl Pts',(-6.390311350308,-8.98426072265847,-25.6807376024135));
#50504=CARTESIAN_POINT('Ctrl Pts',(-4.260207566872,-8.27687337786428,-25.9287995262545));
#50505=CARTESIAN_POINT('Ctrl Pts',(0.0001663377215664,-7.56887498315389,
-26.1774674747135));
#50506=CARTESIAN_POINT('Ctrl Pts',(4.260540242315,-8.27692866476545,-25.9287801080206));
#50507=CARTESIAN_POINT('Ctrl Pts',(6.390810363473,-8.9844264466778,-25.6806794874087));
#50508=CARTESIAN_POINT('Ctrl Pts',(-6.390311350308,-8.18394893381911,-25.1149841535959));
#50509=CARTESIAN_POINT('Ctrl Pts',(-4.260207566872,-7.53598966689574,-25.3660582042809));
#50510=CARTESIAN_POINT('Ctrl Pts',(0.0001663377215664,-6.8861563415995,
-25.6190371135297));
#50511=CARTESIAN_POINT('Ctrl Pts',(4.260540242315,-7.53604041174194,-25.3660384494022));
#50512=CARTESIAN_POINT('Ctrl Pts',(6.390810363473,-8.18410073524863,-25.1149253329315));
#50513=CARTESIAN_POINT('Ctrl Pts',(-6.390311350308,-6.63374493681489,-23.7052293667987));
#50514=CARTESIAN_POINT('Ctrl Pts',(-4.260207566872,-6.09525955626641,-23.9981328630517));
#50515=CARTESIAN_POINT('Ctrl Pts',(0.0001663377215663,-5.5578203229384,
-24.2900566685128));
#50516=CARTESIAN_POINT('Ctrl Pts',(4.260540242315,-6.09530152436809,-23.998110067003));
#50517=CARTESIAN_POINT('Ctrl Pts',(6.390810363473,-6.63387109113548,-23.7051607464652));
#50518=CARTESIAN_POINT('Ctrl Pts',(-6.390311350308,-4.89945807532427,-21.0044950488243));
#50519=CARTESIAN_POINT('Ctrl Pts',(-4.260207566872,-4.44478852897079,-21.4424839271908));
#50520=CARTESIAN_POINT('Ctrl Pts',(0.0001663377215666,-3.98943207393405,
-21.8807691943046));
#50521=CARTESIAN_POINT('Ctrl Pts',(4.260540242315,-4.44482408731423,-21.4424497019158));
#50522=CARTESIAN_POINT('Ctrl Pts',(6.390810363473,-4.89956459357196,-21.0043924384536));
#50523=CARTESIAN_POINT('Ctrl Pts',(-6.390311350308,-4.02649527288926,-18.1257216335683));
#50524=CARTESIAN_POINT('Ctrl Pts',(-4.260207566872,-3.53810367046438,-18.7393778278849));
#50525=CARTESIAN_POINT('Ctrl Pts',(0.0001663377215658,-3.05102410498822,
-19.3530139783685));
#50526=CARTESIAN_POINT('Ctrl Pts',(4.260540242315,-3.5381417060386,-18.7393299096397));
#50527=CARTESIAN_POINT('Ctrl Pts',(6.390810363473,-4.02660969144102,-18.1255778685305));
#50528=CARTESIAN_POINT('Ctrl Pts',(-6.390311350308,-3.91822475000029,-16.2401092417364));
#50529=CARTESIAN_POINT('Ctrl Pts',(-4.260207566872,-3.34432375800902,-16.9588839722607));
#50530=CARTESIAN_POINT('Ctrl Pts',(0.0001663377215673,-2.76847329023801,
-17.67766846846));
#50531=CARTESIAN_POINT('Ctrl Pts',(4.260540242315,-3.34436872560761,-16.9588278430867));
#50532=CARTESIAN_POINT('Ctrl Pts',(6.390810363473,-3.91835920133192,-16.2399408499196));
#50533=CARTESIAN_POINT('Ctrl Pts',(-6.390311350308,-3.94962504311709,-15.4599592241865));
#50534=CARTESIAN_POINT('Ctrl Pts',(-4.260207566872,-3.32898404753985,-16.2180683920147));
#50535=CARTESIAN_POINT('Ctrl Pts',(0.0001663377215673,-2.70679083262895,
-16.9761985551425));
#50536=CARTESIAN_POINT('Ctrl Pts',(4.260540242315,-3.32903263399909,-16.2180091903709));
#50537=CARTESIAN_POINT('Ctrl Pts',(6.390810363473,-3.94977044452508,-15.4597816172428));
#50538=CARTESIAN_POINT('',(-6.26386060052019,-3.90573752923273,-15.8144217504595));
#50539=CARTESIAN_POINT('Ctrl Pts',(-6.2715955238423,-8.76070944182667,-25.5608567088109));
#50540=CARTESIAN_POINT('Ctrl Pts',(-6.27195777356125,-8.56459408488497,
-25.4158727806631));
#50541=CARTESIAN_POINT('Ctrl Pts',(-6.27229031321318,-8.37478238328197,
-25.2662940479724));
#50542=CARTESIAN_POINT('Ctrl Pts',(-6.27259314304416,-8.1913537279175,-25.112746927186));
#50543=CARTESIAN_POINT('Ctrl Pts',(-6.2728986357117,-8.00631215176943,-24.957849639263));
#50544=CARTESIAN_POINT('Ctrl Pts',(-6.27317389377364,-7.82776629043592,
-24.7989138205072));
#50545=CARTESIAN_POINT('Ctrl Pts',(-6.27341891748261,-7.65576238405222,
-24.6365421341386));
#50546=CARTESIAN_POINT('Ctrl Pts',(-6.27366754263728,-7.48123030302019,
-24.4717838509204));
#50547=CARTESIAN_POINT('Ctrl Pts',(-6.27388503811653,-7.31343384998446,
-24.3034879431072));
#50548=CARTESIAN_POINT('Ctrl Pts',(-6.27407140418428,-7.15238613772221,
-24.1322429852995));
#50549=CARTESIAN_POINT('Ctrl Pts',(-6.27421804474197,-7.02566711303238,
-23.9975003445527));
#50550=CARTESIAN_POINT('Ctrl Pts',(-6.27434541247218,-6.90312564630339,
-23.8609310582105));
#50551=CARTESIAN_POINT('Ctrl Pts',(-6.27445350750348,-6.78475354197435,
-23.7228045339384));
#50552=CARTESIAN_POINT('Ctrl Pts',(-6.27450262984591,-6.730960921048,-23.6600347808604));
#50553=CARTESIAN_POINT('Ctrl Pts',(-6.27454777213208,-6.67802913997596,
-23.5969432473287));
#50554=CARTESIAN_POINT('Ctrl Pts',(-6.27458893437407,-6.6259526392861,-23.5335576726619));
#50555=CARTESIAN_POINT('Ctrl Pts',(-6.27470712617076,-6.47642202861682,
-23.3515545894672));
#50556=CARTESIAN_POINT('Ctrl Pts',(-6.27479250318269,-6.33394454999158,
-23.1671310164002));
#50557=CARTESIAN_POINT('Ctrl Pts',(-6.27484506540985,-6.19837392969763,
-22.9809083500403));
#50558=CARTESIAN_POINT('Ctrl Pts',(-6.27489762763701,-6.06280330940369,
-22.7946856836805));
#50559=CARTESIAN_POINT('Ctrl Pts',(-6.27491737507941,-5.93413944051589,
-22.6066637620607));
#50560=CARTESIAN_POINT('Ctrl Pts',(-6.27490430773705,-5.81221558908333,
-22.4174135733054));
#50561=CARTESIAN_POINT('Ctrl Pts',(-6.2748947676246,-5.72320229014943,-22.2792471405111));
#50562=CARTESIAN_POINT('Ctrl Pts',(-6.27486753869774,-5.63762494416323,
-22.1401745615071));
#50563=CARTESIAN_POINT('Ctrl Pts',(-6.27482283814201,-5.55559566787712,
-22.000668726424));
#50564=CARTESIAN_POINT('Ctrl Pts',(-6.2747779206947,-5.47316837729791,-21.8604859950076));
#50565=CARTESIAN_POINT('Ctrl Pts',(-6.274715361659,-5.39432374986302,-21.7198661346417));
#50566=CARTESIAN_POINT('Ctrl Pts',(-6.27463538139726,-5.31912446741838,
-21.5793022040088));
#50567=CARTESIAN_POINT('Ctrl Pts',(-6.2745769115678,-5.2641497883714,-21.4765424871483));
#50568=CARTESIAN_POINT('Ctrl Pts',(-6.27450913115853,-5.21112225376327,
-21.3738129550114));
#50569=CARTESIAN_POINT('Ctrl Pts',(-6.27443212626573,-5.16004897315625,
-21.2713091205343));
#50570=CARTESIAN_POINT('Ctrl Pts',(-6.27435635457874,-5.10979361287016,
-21.1704468483025));
#50571=CARTESIAN_POINT('Ctrl Pts',(-6.27427024744633,-5.06062330858267,
-21.0681861027421));
#50572=CARTESIAN_POINT('Ctrl Pts',(-6.27417380486852,-5.01262251506725,
-20.9645377933814));
#50573=CARTESIAN_POINT('Ctrl Pts',(-6.27399075524317,-4.92151620632652,
-20.7678115690527));
#50574=CARTESIAN_POINT('Ctrl Pts',(-6.27377047251187,-4.83462177577421,
-20.5660838688701));
#50575=CARTESIAN_POINT('Ctrl Pts',(-6.27351295667464,-4.75246065776447,
-20.3594970111178));
#50576=CARTESIAN_POINT('Ctrl Pts',(-6.27325823298668,-4.67119038245961,
-20.1551500984832));
#50577=CARTESIAN_POINT('Ctrl Pts',(-6.27296707922523,-4.59455132156058,
-19.9460487147278));
#50578=CARTESIAN_POINT('Ctrl Pts',(-6.2726394953903,-4.52307273725537,-19.7323747704891));
#50579=CARTESIAN_POINT('Ctrl Pts',(-6.27231699872677,-4.45270417051253,
-19.5220190485268));
#50580=CARTESIAN_POINT('Ctrl Pts',(-6.2719591946766,-4.38733705627334,-19.3072316127526));
#50581=CARTESIAN_POINT('Ctrl Pts',(-6.27156608323978,-4.32750034373043,
-19.0882303678766));
#50582=CARTESIAN_POINT('Ctrl Pts',(-6.27136275171617,-4.29655062110826,
-18.974954963952));
#50583=CARTESIAN_POINT('Ctrl Pts',(-6.27114997428599,-4.2670808590318,-18.8605529604809));
#50584=CARTESIAN_POINT('Ctrl Pts',(-6.27092775094925,-4.23916681989789,
-18.7450593753188));
#50585=CARTESIAN_POINT('Ctrl Pts',(-6.27050608281783,-4.18620001229596,
-18.5259106353175));
#50586=CARTESIAN_POINT('Ctrl Pts',(-6.27005040532724,-4.13883315746638,
-18.3028288891132));
#50587=CARTESIAN_POINT('Ctrl Pts',(-6.2695607180599,-4.09760163845932,-18.0760877681166));
#50588=CARTESIAN_POINT('Ctrl Pts',(-6.26938505158857,-4.08281057498897,
-17.9947484822313));
#50589=CARTESIAN_POINT('Ctrl Pts',(-6.26920500844612,-4.06880927968371,
-17.9129387064842));
#50590=CARTESIAN_POINT('Ctrl Pts',(-6.26902058861328,-4.05562321450361,
-17.8306725395332));
#50591=CARTESIAN_POINT('Ctrl Pts',(-6.26850854126086,-4.01901169794123,
-17.602257990332));
#50592=CARTESIAN_POINT('Ctrl Pts',(-6.26796275346181,-3.98868443460602,
-17.3703213570019));
#50593=CARTESIAN_POINT('Ctrl Pts',(-6.26738322480352,-3.96507786318383,
-17.1352142780564));
#50594=CARTESIAN_POINT('Ctrl Pts',(-6.2668123124285,-3.94182226820349,-16.9036027107862));
#50595=CARTESIAN_POINT('Ctrl Pts',(-6.26620865503669,-3.9250890327587,-16.6689142257609));
#50596=CARTESIAN_POINT('Ctrl Pts',(-6.26557225223362,-3.91530349225849,
-16.4315345452492));
#50597=CARTESIAN_POINT('Ctrl Pts',(-6.26502584108532,-3.90690169327874,
-16.2277219548773));
#50598=CARTESIAN_POINT('Ctrl Pts',(-6.2644552905974,-3.903621743592,-16.0219261954994));
#50599=CARTESIAN_POINT('Ctrl Pts',(-6.26386060052019,-3.90573752923273,
-15.8144217504595));
#50600=CARTESIAN_POINT('Ctrl Pts',(6.26385989016308,-3.90573722907187,-15.8144313885695));
#50601=CARTESIAN_POINT('Ctrl Pts',(5.97553399679439,-3.82580629714082,-15.9103385752986));
#50602=CARTESIAN_POINT('Ctrl Pts',(5.68536880827791,-3.75082902346428,-15.998984836958));
#50603=CARTESIAN_POINT('Ctrl Pts',(5.39385181719438,-3.68107864601722,-16.0804594738038));
#50604=CARTESIAN_POINT('Ctrl Pts',(5.12003902107913,-3.61556429706663,-16.1569860530755));
#50605=CARTESIAN_POINT('Ctrl Pts',(4.84503362991563,-3.55466183515149,-16.2271853098323));
#50606=CARTESIAN_POINT('Ctrl Pts',(4.56923960300567,-3.49857607970672,-16.2911687766404));
#50607=CARTESIAN_POINT('Ctrl Pts',(4.31279432864831,-3.44642510637448,-16.3506633852936));
#50608=CARTESIAN_POINT('Ctrl Pts',(4.05566719282585,-3.39843896167755,-16.4047836798324));
#50609=CARTESIAN_POINT('Ctrl Pts',(3.79818295898821,-3.35475746998996,-16.4536554844221));
#50610=CARTESIAN_POINT('Ctrl Pts',(3.57800514413088,-3.3174049096171,-16.4954463427683));
#50611=CARTESIAN_POINT('Ctrl Pts',(3.35756621340383,-3.28319976136122,-16.5333998249633));
#50612=CARTESIAN_POINT('Ctrl Pts',(3.13706923218936,-3.25221122731596,-16.5676189494495));
#50613=CARTESIAN_POINT('Ctrl Pts',(2.89173684623179,-3.21773233806868,-16.6056923026961));
#50614=CARTESIAN_POINT('Ctrl Pts',(2.64636709253532,-3.18724212042279,-16.639157630225));
#50615=CARTESIAN_POINT('Ctrl Pts',(2.4011994254868,-3.16079038021371,-16.6680517792548));
#50616=CARTESIAN_POINT('Ctrl Pts',(2.15979139190104,-3.13474427606927,-16.6965028380074));
#50617=CARTESIAN_POINT('Ctrl Pts',(1.91857929450951,-3.11261378305586,-16.7205218280064));
#50618=CARTESIAN_POINT('Ctrl Pts',(1.67779173970442,-3.09441416005317,-16.7401828536933));
#50619=CARTESIAN_POINT('Ctrl Pts',(1.43871515257066,-3.07634385837945,-16.7597041737406));
#50620=CARTESIAN_POINT('Ctrl Pts',(1.20005709610199,-3.06214882614483,-16.7749291990503));
#50621=CARTESIAN_POINT('Ctrl Pts',(0.962041338001033,-3.05181105112491,
-16.7859696350219));
#50622=CARTESIAN_POINT('Ctrl Pts',(0.725844259084509,-3.04155226707765,
-16.7969257109862));
#50623=CARTESIAN_POINT('Ctrl Pts',(0.490279700428395,-3.03509205442575,
-16.8037608856791));
#50624=CARTESIAN_POINT('Ctrl Pts',(0.255566339400218,-3.03237950988673,
-16.806623472729));
#50625=CARTESIAN_POINT('Ctrl Pts',(0.170630036434285,-3.03139791470287,
-16.8076593641664));
#50626=CARTESIAN_POINT('Ctrl Pts',(0.0858051992296905,-3.03090676284046,
-16.8081754131188));
#50627=CARTESIAN_POINT('Ctrl Pts',(0.00110219042761073,-3.03090254471751,
-16.8081799291764));
#50628=CARTESIAN_POINT('Ctrl Pts',(0.000734796036953708,-3.03090252642165,
-16.8081799487646));
#50629=CARTESIAN_POINT('Ctrl Pts',(0.000367399226901863,-3.0309025172856,
-16.8081799587317));
#50630=CARTESIAN_POINT('Ctrl Pts',(-1.6247122406382E-12,-3.03090251730972,
-16.808179959077));
#50631=CARTESIAN_POINT('Ctrl Pts',(-0.229875830423132,-3.03090253239659,
-16.8081801751603));
#50632=CARTESIAN_POINT('Ctrl Pts',(-0.46069844667378,-3.03449140238313,
-16.8044103498536));
#50633=CARTESIAN_POINT('Ctrl Pts',(-0.692242623528576,-3.04173275150852,
-16.7967117441749));
#50634=CARTESIAN_POINT('Ctrl Pts',(-0.925635275154074,-3.04903191012559,
-16.7889516786116));
#50635=CARTESIAN_POINT('Ctrl Pts',(-1.15976105416605,-3.06004208265118,
-16.7771998500654));
#50636=CARTESIAN_POINT('Ctrl Pts',(-1.39438929807558,-3.07479400283838,
-16.7613341401061));
#50637=CARTESIAN_POINT('Ctrl Pts',(-1.63050140140359,-3.08963921859541,
-16.7453680906362));
#50638=CARTESIAN_POINT('Ctrl Pts',(-1.86712234520368,-3.10827360850861,
-16.7252359917334));
#50639=CARTESIAN_POINT('Ctrl Pts',(-2.10401706291493,-3.13069428508702,
-16.7008539691834));
#50640=CARTESIAN_POINT('Ctrl Pts',(-2.34376869870852,-3.15338535197618,
-16.6761779027569));
#50641=CARTESIAN_POINT('Ctrl Pts',(-2.58380075158332,-3.17995453594481,
-16.6471488047795));
#50642=CARTESIAN_POINT('Ctrl Pts',(-2.82386954738932,-3.21036459359605,
-16.6137208487122));
#50643=CARTESIAN_POINT('Ctrl Pts',(-2.927994146548,-3.22355429221014,-16.5992222025449));
#50644=CARTESIAN_POINT('Ctrl Pts',(-3.03212565779147,-3.23746610815007,
-16.5838965601351));
#50645=CARTESIAN_POINT('Ctrl Pts',(-3.13624419901553,-3.25209507527437,
-16.5677425234917));
#50646=CARTESIAN_POINT('Ctrl Pts',(-3.3990646725385,-3.28902213957589,-16.5269658135031));
#50647=CARTESIAN_POINT('Ctrl Pts',(-3.66179671230626,-3.33051927196033,
-16.4808834330153));
#50648=CARTESIAN_POINT('Ctrl Pts',(-3.92409681112318,-3.37646580551342,
-16.4293256145461));
#50649=CARTESIAN_POINT('Ctrl Pts',(-4.19384845018918,-3.423717609044,-16.376303118171));
#50650=CARTESIAN_POINT('Ctrl Pts',(-4.46314325816149,-3.47567475800782,
-16.3174900314543));
#50651=CARTESIAN_POINT('Ctrl Pts',(-4.7316076127716,-3.53216981419204,-16.2527504905616));
#50652=CARTESIAN_POINT('Ctrl Pts',(-5.02537496897885,-3.59398957912181,
-16.1819091909868));
#50653=CARTESIAN_POINT('Ctrl Pts',(-5.31814795279717,-3.66124259971326,
-16.103971693354));
#50654=CARTESIAN_POINT('Ctrl Pts',(-5.60943702954381,-3.73367270940399,
-16.0188149762675));
#50655=CARTESIAN_POINT('Ctrl Pts',(-5.82848677133169,-3.78814024043064,
-15.9547770209221));
#50656=CARTESIAN_POINT('Ctrl Pts',(-6.04669735500675,-3.84553455164856,
-15.8866578189599));
#50657=CARTESIAN_POINT('Ctrl Pts',(-6.26386060052019,-3.90573752923273,
-15.8144217504595));
#50658=CARTESIAN_POINT('Ctrl Pts',(6.38277618953878,-3.93902298367305,-15.7736509876441));
#50659=CARTESIAN_POINT('Ctrl Pts',(6.32406965201728,-3.92242603988433,-15.7947737499583));
#50660=CARTESIAN_POINT('Ctrl Pts',(5.68189763608108,-3.74339185396048,-16.0219765267289));
#50661=CARTESIAN_POINT('Ctrl Pts',(4.3416298703543,-3.42592551432459,-16.4111224147635));
#50662=CARTESIAN_POINT('Ctrl Pts',(2.26093495053969,-3.1113690382538,-16.7778275679097));
#50663=CARTESIAN_POINT('Ctrl Pts',(0.00239109326725635,-2.99312376423343,
-16.9112693274866));
#50664=CARTESIAN_POINT('Ctrl Pts',(-2.25660966670575,-3.11089910253385,
-16.7783633179704));
#50665=CARTESIAN_POINT('Ctrl Pts',(-4.33836522858824,-3.42525974347605,
-16.4119189559543));
#50666=CARTESIAN_POINT('Ctrl Pts',(-5.68016038563479,-3.74293403065789,
-16.0225505707191));
#50667=CARTESIAN_POINT('Ctrl Pts',(-6.32338632353712,-3.92223285081666,
-15.7950196002647));
#50668=CARTESIAN_POINT('Ctrl Pts',(-6.38277186385808,-3.93902174367425,
-15.7736525473708));
#50669=CARTESIAN_POINT('Ctrl Pts',(6.17957679916044,-3.89068228939978,-15.1604192383161));
#50670=CARTESIAN_POINT('Ctrl Pts',(6.12270909368446,-3.87483541835791,-15.1808735763493));
#50671=CARTESIAN_POINT('Ctrl Pts',(5.500659799661,-3.70388659307422,-15.400888496091));
#50672=CARTESIAN_POINT('Ctrl Pts',(4.2025877538095,-3.40064492207699,-15.7777527540127));
#50673=CARTESIAN_POINT('Ctrl Pts',(2.18817889704034,-3.10011512502998,-16.1328510982524));
#50674=CARTESIAN_POINT('Ctrl Pts',(0.00231396716250085,-2.98714523578678,
-16.2620475592341));
#50675=CARTESIAN_POINT('Ctrl Pts',(-2.18399216732578,-3.09966614175185,
-16.1333698383091));
#50676=CARTESIAN_POINT('Ctrl Pts',(-4.19942635557926,-3.40000887948827,
-15.7785241473102));
#50677=CARTESIAN_POINT('Ctrl Pts',(-5.49897707124986,-3.7034493797774,-15.4014444027214));
#50678=CARTESIAN_POINT('Ctrl Pts',(-6.12204716868564,-3.87465096080647,
-15.1811116463534));
#50679=CARTESIAN_POINT('Ctrl Pts',(-6.17957260911428,-3.89068110637816,
-15.1604207480391));
#50680=CARTESIAN_POINT('Ctrl Pts',(6.17623614235066,-3.3901470900782,-14.7509334303916));
#50681=CARTESIAN_POINT('Ctrl Pts',(6.1195290660352,-3.37449952843537,-14.7711429291056));
#50682=CARTESIAN_POINT('Ctrl Pts',(5.49920093562508,-3.2056835753871,-14.9885423978857));
#50683=CARTESIAN_POINT('Ctrl Pts',(4.20386779883051,-2.90584507060185,-15.3613285942364));
#50684=CARTESIAN_POINT('Ctrl Pts',(2.19034988765805,-2.60796875639558,-15.7133110788741));
#50685=CARTESIAN_POINT('Ctrl Pts',(0.00231704624412195,-2.49578212587921,
-15.841584047978));
#50686=CARTESIAN_POINT('Ctrl Pts',(-2.18616172967826,-2.60752317468483,
-15.7138258279247));
#50687=CARTESIAN_POINT('Ctrl Pts',(-4.20071107704675,-2.90521550125399,
-15.3620923337382));
#50688=CARTESIAN_POINT('Ctrl Pts',(-5.49752249868785,-3.20525164179727,
-14.9890918874241));
#50689=CARTESIAN_POINT('Ctrl Pts',(-6.118869010867,-3.37431738868919,-14.7713781487167));
#50690=CARTESIAN_POINT('Ctrl Pts',(-6.17623196352304,-3.39014591921539,
-14.7509349215014));
#50691=CARTESIAN_POINT('Ctrl Pts',(6.37340174051362,-2.779344847644,-14.8203009020849));
#50692=CARTESIAN_POINT('Ctrl Pts',(6.31508205120875,-2.76321556726599,-14.8408512070517));
#50693=CARTESIAN_POINT('Ctrl Pts',(5.67705854619564,-2.58918646586821,-15.0619384307092));
#50694=CARTESIAN_POINT('Ctrl Pts',(4.34347432998779,-2.27971680019969,-15.4415401757572));
#50695=CARTESIAN_POINT('Ctrl Pts',(2.26537698871116,-1.97141906261117,-15.8009351771397));
#50696=CARTESIAN_POINT('Ctrl Pts',(0.00239760332421311,-1.85503039601574,
-15.9322038348625));
#50697=CARTESIAN_POINT('Ctrl Pts',(-2.26104951319322,-1.97095717406781,
-15.8014615465953));
#50698=CARTESIAN_POINT('Ctrl Pts',(-4.34022135115418,-2.27906626152107,
-15.4423187874132));
#50699=CARTESIAN_POINT('Ctrl Pts',(-5.67533167450272,-2.58874103693919,
-15.0624974659534));
#50700=CARTESIAN_POINT('Ctrl Pts',(-6.31440322588509,-2.76302781680913,
-14.8410903928893));
#50701=CARTESIAN_POINT('Ctrl Pts',(-6.37339744190952,-2.77934363626544,
-14.8203024183022));
#50702=CARTESIAN_POINT('',(-6.249946133935,-2.76546782187014,-14.8593871026385));
#50703=CARTESIAN_POINT('Ctrl Pts',(-6.26386069626091,-3.90573717912781,
-15.8144217465729));
#50704=CARTESIAN_POINT('Ctrl Pts',(-6.25435278828631,-3.90345940501981,
-15.7850161412327));
#50705=CARTESIAN_POINT('Ctrl Pts',(-6.24502133065853,-3.89974161222485,
-15.7549842405191));
#50706=CARTESIAN_POINT('Ctrl Pts',(-6.23596915592907,-3.89443417155273,
-15.7244986756939));
#50707=CARTESIAN_POINT('Ctrl Pts',(-6.2271444796111,-3.88926011698486,-15.6947792712421));
#50708=CARTESIAN_POINT('Ctrl Pts',(-6.21858551912677,-3.88257463437956,
-15.6646290267509));
#50709=CARTESIAN_POINT('Ctrl Pts',(-6.21039361594383,-3.87426710369931,
-15.6342479860573));
#50710=CARTESIAN_POINT('Ctrl Pts',(-6.20232798335637,-3.86608762590524,
-15.6043352409495));
#50711=CARTESIAN_POINT('Ctrl Pts',(-6.19461850613904,-3.85633510187562,
-15.5741992093649));
#50712=CARTESIAN_POINT('Ctrl Pts',(-6.18736330797966,-3.84494106661073,
-15.5440647189826));
#50713=CARTESIAN_POINT('Ctrl Pts',(-6.18023558928131,-3.83374723338617,
-15.5144597149779));
#50714=CARTESIAN_POINT('Ctrl Pts',(-6.17354666467265,-3.82096863573755,
-15.4848568331048));
#50715=CARTESIAN_POINT('Ctrl Pts',(-6.1673860145996,-3.80658418723543,-15.4554941847338));
#50716=CARTESIAN_POINT('Ctrl Pts',(-6.16658691141318,-3.80471836812597,
-15.4516855305177));
#50717=CARTESIAN_POINT('Ctrl Pts',(-6.16579668723456,-3.8028255969964,-15.4478809449517));
#50718=CARTESIAN_POINT('Ctrl Pts',(-6.16501552817343,-3.80090588826776,
-15.4440809697158));
#50719=CARTESIAN_POINT('Ctrl Pts',(-6.15908467647008,-3.78633074173258,
-15.4152301367392));
#50720=CARTESIAN_POINT('Ctrl Pts',(-6.15367730115858,-3.7701987020078,-15.3866443546201));
#50721=CARTESIAN_POINT('Ctrl Pts',(-6.14886799870019,-3.75254373120564,
-15.3585666204129));
#50722=CARTESIAN_POINT('Ctrl Pts',(-6.14412030816652,-3.73511493805424,
-15.3308485897722));
#50723=CARTESIAN_POINT('Ctrl Pts',(-6.13995573756892,-3.71620200565619,
-15.303626479117));
#50724=CARTESIAN_POINT('Ctrl Pts',(-6.13643278986983,-3.69588658064368,
-15.2771349926435));
#50725=CARTESIAN_POINT('Ctrl Pts',(-6.13293052880874,-3.67569044716736,
-15.2507990633447));
#50726=CARTESIAN_POINT('Ctrl Pts',(-6.13006259738892,-3.65410845511605,
-15.2251860084886));
#50727=CARTESIAN_POINT('Ctrl Pts',(-6.12786957795671,-3.63126787890627,
-15.2005153049664));
#50728=CARTESIAN_POINT('Ctrl Pts',(-6.12568399895156,-3.60850479569017,
-15.1759283036527));
#50729=CARTESIAN_POINT('Ctrl Pts',(-6.12416889885337,-3.58449208282344,
-15.1522780155925));
#50730=CARTESIAN_POINT('Ctrl Pts',(-6.12334491227003,-3.55939782163374,
-15.1297589600051));
#50731=CARTESIAN_POINT('Ctrl Pts',(-6.12252166712978,-3.53432614086812,
-15.1072601676095));
#50732=CARTESIAN_POINT('Ctrl Pts',(-6.12238833698384,-3.50817547284213,
-15.0858911958049));
#50733=CARTESIAN_POINT('Ctrl Pts',(-6.12294457092848,-3.4811476984129,-15.0658129831534));
#50734=CARTESIAN_POINT('Ctrl Pts',(-6.1235035154685,-3.453988214365,-15.0456369269396));
#50735=CARTESIAN_POINT('Ctrl Pts',(-6.12475871787342,-3.42594380389806,
-15.0267647165739));
#50736=CARTESIAN_POINT('Ctrl Pts',(-6.12668863274399,-3.39724362941968,
-15.0093178766538));
#50737=CARTESIAN_POINT('Ctrl Pts',(-6.12862601474739,-3.3684324096208,-14.9918035322684));
#50738=CARTESIAN_POINT('Ctrl Pts',(-6.13124318893959,-3.338961185371,-14.9757258483972));
#50739=CARTESIAN_POINT('Ctrl Pts',(-6.13449853919524,-3.30907413388349,
-14.9611603452345));
#50740=CARTESIAN_POINT('Ctrl Pts',(-6.13779129187055,-3.27884369444872,
-14.9464274913971));
#50741=CARTESIAN_POINT('Ctrl Pts',(-6.14173674640982,-3.24818868400451,
-14.9332418161091));
#50742=CARTESIAN_POINT('Ctrl Pts',(-6.14627441472987,-3.21736136586032,
-14.9216307439335));
#50743=CARTESIAN_POINT('Ctrl Pts',(-6.14957853519337,-3.19491433678491,
-14.9131760975221));
#50744=CARTESIAN_POINT('Ctrl Pts',(-6.15319626410588,-3.1723759686912,-14.9055552119477));
#50745=CARTESIAN_POINT('Ctrl Pts',(-6.15709971483306,-3.14983968148244,
-14.8987623755919));
#50746=CARTESIAN_POINT('Ctrl Pts',(-6.16255610037322,-3.11833763873896,
-14.8892671016255));
#50747=CARTESIAN_POINT('Ctrl Pts',(-6.16857091169139,-3.08684101637309,
-14.8813914186133));
#50748=CARTESIAN_POINT('Ctrl Pts',(-6.17505758164135,-3.05558476286159,
-14.8750798677663));
#50749=CARTESIAN_POINT('Ctrl Pts',(-6.18169263943854,-3.02361349714708,
-14.8686239350639));
#50750=CARTESIAN_POINT('Ctrl Pts',(-6.18882103907761,-2.99189436209302,
-14.8638040067938));
#50751=CARTESIAN_POINT('Ctrl Pts',(-6.19634461080315,-2.96064532558646,
-14.8605179833599));
#50752=CARTESIAN_POINT('Ctrl Pts',(-6.20397961974074,-2.92893343637719,
-14.8571832881909));
#50753=CARTESIAN_POINT('Ctrl Pts',(-6.21202124066049,-2.89770605675946,
-14.8554275574933));
#50754=CARTESIAN_POINT('Ctrl Pts',(-6.22036670484762,-2.86714907664217,
-14.8551100875152));
#50755=CARTESIAN_POINT('Ctrl Pts',(-6.22891230656577,-2.8358592914443,-14.854785004101));
#50756=CARTESIAN_POINT('Ctrl Pts',(-6.23777617294652,-2.80527266144069,
-14.8559672194602));
#50757=CARTESIAN_POINT('Ctrl Pts',(-6.2468530507251,-2.775540419464,-14.8584817266279));
#50758=CARTESIAN_POINT('Ctrl Pts',(-6.2478814089936,-2.77217192672634,-14.8587666058893));
#50759=CARTESIAN_POINT('Ctrl Pts',(-6.24891250958138,-2.76881434916645,
-14.8590685685164));
#50760=CARTESIAN_POINT('Ctrl Pts',(-6.2499462061289,-2.76546786755201,-14.8593873480964));
#50761=CARTESIAN_POINT('Ctrl Pts',(6.24994601332121,-2.76546575790955,-14.8593877960249));
#50762=CARTESIAN_POINT('Ctrl Pts',(6.23073047753292,-2.76025017414552,-14.8660101204524));
#50763=CARTESIAN_POINT('Ctrl Pts',(6.21150010023597,-2.75505455214819,-14.8726007831637));
#50764=CARTESIAN_POINT('Ctrl Pts',(6.19225495680607,-2.74987900475405,-14.8791597838055));
#50765=CARTESIAN_POINT('Ctrl Pts',(5.87844425507332,-2.66548669219361,-14.9861106413847));
#50766=CARTESIAN_POINT('Ctrl Pts',(5.560709433538,-2.58643024421835,-15.0846465181307));
#50767=CARTESIAN_POINT('Ctrl Pts',(5.23942746496503,-2.51325265395543,-15.1747448746766));
#50768=CARTESIAN_POINT('Ctrl Pts',(5.1126024482369,-2.48436603716071,-15.2103109091692));
#50769=CARTESIAN_POINT('Ctrl Pts',(4.9852244466522,-2.45639572037815,-15.2445617066485));
#50770=CARTESIAN_POINT('Ctrl Pts',(4.85731578768611,-2.42937608683371,-15.2774940624876));
#50771=CARTESIAN_POINT('Ctrl Pts',(4.70825219270268,-2.39788765013344,-15.3158731323045));
#50772=CARTESIAN_POINT('Ctrl Pts',(4.55847124802094,-2.36768574506229,-15.3524616131821));
#50773=CARTESIAN_POINT('Ctrl Pts',(4.40800948962857,-2.33881486398786,-15.3872540434359));
#50774=CARTESIAN_POINT('Ctrl Pts',(4.32035481797119,-2.32199552312626,-15.4075231076994));
#50775=CARTESIAN_POINT('Ctrl Pts',(4.23246905680847,-2.30562793676945,-15.4271825781245));
#50776=CARTESIAN_POINT('Ctrl Pts',(4.14436205067732,-2.28971964526396,-15.4462315091494));
#50777=CARTESIAN_POINT('Ctrl Pts',(4.02468944586554,-2.26811198015124,-15.4721049929362));
#50778=CARTESIAN_POINT('Ctrl Pts',(3.90460700146106,-2.2473522258916,-15.4968523834063));
#50779=CARTESIAN_POINT('Ctrl Pts',(3.7841358923644,-2.2274589624909,-15.5204711633146));
#50780=CARTESIAN_POINT('Ctrl Pts',(3.72390033781608,-2.21751233079056,-15.5322805532687));
#50781=CARTESIAN_POINT('Ctrl Pts',(3.66356761388492,-2.20778231952401,-15.5438077759747));
#50782=CARTESIAN_POINT('Ctrl Pts',(3.6031404319624,-2.19827105127879,-15.5550524434222));
#50783=CARTESIAN_POINT('Ctrl Pts',(3.57292684100114,-2.19351541715618,-15.5606747771459));
#50784=CARTESIAN_POINT('Ctrl Pts',(3.54268963537251,-2.18881446865928,-15.5662264711738));
#50785=CARTESIAN_POINT('Ctrl Pts',(3.5124291552237,-2.18416846515596,-15.5717074721342));
#50786=CARTESIAN_POINT('Ctrl Pts',(3.49729891514929,-2.18184546340429,-15.5744479726143));
#50787=CARTESIAN_POINT('Ctrl Pts',(3.4821628564358,-2.1795361978934,-15.5771707997731));
#50788=CARTESIAN_POINT('Ctrl Pts',(3.46702102182034,-2.17724070036537,-15.5798759466597));
#50789=CARTESIAN_POINT('Ctrl Pts',(3.45945010451261,-2.17609295160136,-15.581228520103));
#50790=CARTESIAN_POINT('Ctrl Pts',(3.45187774322886,-2.1749486448326,-15.5825766734749));
#50791=CARTESIAN_POINT('Ctrl Pts',(3.4443039433257,-2.17380778398253,-15.5839204058893));
#50792=CARTESIAN_POINT('Ctrl Pts',(3.43673014342255,-2.17266692313246,-15.5852641383038));
#50793=CARTESIAN_POINT('Ctrl Pts',(3.43037813366342,-2.17171258314623,-15.5863879362203));
#50794=CARTESIAN_POINT('Ctrl Pts',(3.42157823311786,-2.17039554309748,-15.5879383393621));
#50795=CARTESIAN_POINT('Ctrl Pts',(3.12618810143945,-2.12618588056643,-15.6399814034683));
#50796=CARTESIAN_POINT('Ctrl Pts',(2.82944930104073,-2.0874553149349,-15.6851449519319));
#50797=CARTESIAN_POINT('Ctrl Pts',(2.5316589119422,-2.05443685070837,-15.7234683965577));
#50798=CARTESIAN_POINT('Ctrl Pts',(2.45451197504621,-2.04588293671605,-15.7333966429767));
#50799=CARTESIAN_POINT('Ctrl Pts',(2.3772943200674,-2.03771250803676,-15.742865620832));
#50800=CARTESIAN_POINT('Ctrl Pts',(2.3000108328019,-2.02992988165436,-15.7518755957562));
#50801=CARTESIAN_POINT('Ctrl Pts',(2.0056692737147,-2.00028900409772,-15.7861909477202));
#50802=CARTESIAN_POINT('Ctrl Pts',(1.71037431067632,-1.97627097834048,-15.813851236479));
#50803=CARTESIAN_POINT('Ctrl Pts',(1.41448173569927,-1.95793907528011,-15.8348961980598));
#50804=CARTESIAN_POINT('Ctrl Pts',(1.11826650418036,-1.93958718216609,-15.8559641081533));
#50805=CARTESIAN_POINT('Ctrl Pts',(0.82145181565684,-1.92693366275149,-15.8704022996846));
#50806=CARTESIAN_POINT('Ctrl Pts',(0.524379711120614,-1.92007368135013,
-15.8782121451863));
#50807=CARTESIAN_POINT('Ctrl Pts',(0.350504318392921,-1.91605855525094,
-15.8827832238335));
#50808=CARTESIAN_POINT('Ctrl Pts',(0.176540502814779,-1.91402874194139,
-15.8850828882085));
#50809=CARTESIAN_POINT('Ctrl Pts',(0.00255561583708888,-1.9140086853341,
-15.8851052067127));
#50810=CARTESIAN_POINT('Ctrl Pts',(0.0020716235670054,-1.9140086295405,
-15.8851052687984));
#50811=CARTESIAN_POINT('Ctrl Pts',(0.00158763113357761,-1.91400858930194,
-15.8851053132581));
#50812=CARTESIAN_POINT('Ctrl Pts',(0.00110363853824586,-1.91400856461776,
-15.8851053400918));
#50813=CARTESIAN_POINT('Ctrl Pts',(-0.295367109470143,-1.91399344426611,
-15.8851217771233));
#50814=CARTESIAN_POINT('Ctrl Pts',(-0.591802808432749,-1.91978340639987,
-15.8785311956525));
#50815=CARTESIAN_POINT('Ctrl Pts',(-0.887865890379048,-1.93130552535533,
-15.865347476795));
#50816=CARTESIAN_POINT('Ctrl Pts',(-1.1648013594823,-1.94208324001336,-15.8530155124639));
#50817=CARTESIAN_POINT('Ctrl Pts',(-1.44141105838077,-1.95787681441081,
-15.8349144089549));
#50818=CARTESIAN_POINT('Ctrl Pts',(-1.71740521728641,-1.97865173277633,
-15.8110257152412));
#50819=CARTESIAN_POINT('Ctrl Pts',(-1.91042473226883,-1.99318089775074,
-15.7943188976315));
#50820=CARTESIAN_POINT('Ctrl Pts',(-2.10314787222578,-2.01013167948437,
-15.7747822528312));
#50821=CARTESIAN_POINT('Ctrl Pts',(-2.29547328915249,-2.02947446977817,
-15.7524039455861));
#50822=CARTESIAN_POINT('Ctrl Pts',(-2.38764658058091,-2.03874463632858,
-15.7416789864604));
#50823=CARTESIAN_POINT('Ctrl Pts',(-2.47972848825322,-2.04856429938607,
-15.7303012338651));
#50824=CARTESIAN_POINT('Ctrl Pts',(-2.57171070235722,-2.05892465772404,
-15.7182703465243));
#50825=CARTESIAN_POINT('Ctrl Pts',(-2.71366517039613,-2.07491360918477,
-15.6997032982191));
#50826=CARTESIAN_POINT('Ctrl Pts',(-2.85537926672626,-2.09219563824349,
-15.6795803778416));
#50827=CARTESIAN_POINT('Ctrl Pts',(-2.99681541196094,-2.1107489567871,-15.6578985020398));
#50828=CARTESIAN_POINT('Ctrl Pts',(-3.06753348457829,-2.1200256160589,-15.6470575641389));
#50829=CARTESIAN_POINT('Ctrl Pts',(-3.13818206762113,-2.12962009476506,
-15.6358268636259));
#50830=CARTESIAN_POINT('Ctrl Pts',(-3.20875652118209,-2.13952927635221,
-15.624205909158));
#50831=CARTESIAN_POINT('Ctrl Pts',(-3.24404374796257,-2.14448386714579,
-15.618395431924));
#50832=CARTESIAN_POINT('Ctrl Pts',(-3.27931244221733,-2.14951713346246,
-15.6124873896378));
#50833=CARTESIAN_POINT('Ctrl Pts',(-3.3145620252032,-2.15462867384623,-15.6064817125059));
#50834=CARTESIAN_POINT('Ctrl Pts',(-3.33218681669613,-2.15718444403811,
-15.6034788739399));
#50835=CARTESIAN_POINT('Ctrl Pts',(-3.34980683035885,-2.15975978273357,
-15.6004516265627));
#50836=CARTESIAN_POINT('Ctrl Pts',(-3.36742199402595,-2.1623546383924,-15.5973999611852));
#50837=CARTESIAN_POINT('Ctrl Pts',(-3.3762295758595,-2.16365206622181,-15.5958741284965));
#50838=CARTESIAN_POINT('Ctrl Pts',(-3.38503594519326,-2.16495437329122,
-15.5943421913015));
#50839=CARTESIAN_POINT('Ctrl Pts',(-3.39384109301869,-2.16626155306888,
-15.5928041484225));
#50840=CARTESIAN_POINT('Ctrl Pts',(-3.40264624084412,-2.16756873284654,
-15.5912661055435));
#50841=CARTESIAN_POINT('Ctrl Pts',(-3.41267288227766,-2.16906370843053,
-15.5895066228579));
#50842=CARTESIAN_POINT('Ctrl Pts',(-3.42025286296309,-2.17019770396608,
-15.5881717015338));
#50843=CARTESIAN_POINT('Ctrl Pts',(-3.7512914807498,-2.21972240993068,-15.5298720134026));
#50844=CARTESIAN_POINT('Ctrl Pts',(-4.079618287111,-2.27588861931481,-15.4631235878544));
#50845=CARTESIAN_POINT('Ctrl Pts',(-4.40475725936993,-2.3382578308419,-15.3879956510477));
#50846=CARTESIAN_POINT('Ctrl Pts',(-4.72371670931558,-2.39944166636925,
-15.3142955798661));
#50847=CARTESIAN_POINT('Ctrl Pts',(-5.03960868942063,-2.4665955473129,-15.2325312282107));
#50848=CARTESIAN_POINT('Ctrl Pts',(-5.35209806335916,-2.53926302950475,
-15.1427479434758));
#50849=CARTESIAN_POINT('Ctrl Pts',(-5.63433594988217,-2.60489571433585,
-15.0616564035962));
#50850=CARTESIAN_POINT('Ctrl Pts',(-5.91379807239021,-2.67502673187186,
-14.9740228129603));
#50851=CARTESIAN_POINT('Ctrl Pts',(-6.19021699498113,-2.7493336727775,-14.8798537270554));
#50852=CARTESIAN_POINT('Ctrl Pts',(-6.21014258404868,-2.75469007007286,
-14.8730655719934));
#50853=CARTESIAN_POINT('Ctrl Pts',(-6.23005235057421,-2.76006817087034,
-14.8662434464133));
#50854=CARTESIAN_POINT('Ctrl Pts',(-6.2499462061289,-2.76546786755201,-14.8593873480964));
#50855=CARTESIAN_POINT('Ctrl Pts',(-6.25025869058268,-3.90195425102708,
-15.8298806636529));
#50856=CARTESIAN_POINT('Ctrl Pts',(-6.29004325280698,-3.91230167814786,
-15.8159179950948));
#50857=CARTESIAN_POINT('Ctrl Pts',(-6.41684493426804,-3.95321250785999,
-15.7689312449806));
#50858=CARTESIAN_POINT('Ctrl Pts',(-6.61884385638551,-4.06299859433413,
-15.6800117310403));
#50859=CARTESIAN_POINT('Ctrl Pts',(-6.82673050587102,-4.25689239114287,
-15.5624948978267));
#50860=CARTESIAN_POINT('Ctrl Pts',(-6.9795005695021,-4.49148568888774,-15.4459527338404));
#50861=CARTESIAN_POINT('Ctrl Pts',(-7.07130089065108,-4.73958816623202,
-15.3403618218109));
#50862=CARTESIAN_POINT('Ctrl Pts',(-7.10319232002285,-4.94126548594463,
-15.2651787834553));
#50863=CARTESIAN_POINT('Ctrl Pts',(-7.1060521427303,-5.05547800808013,-15.2264033130095));
#50864=CARTESIAN_POINT('Ctrl Pts',(-7.10556044294757,-5.0897512085814,-15.2151090406844));
#50865=CARTESIAN_POINT('Ctrl Pts',(-6.05195504581396,-3.8612747752879,-15.216963146136));
#50866=CARTESIAN_POINT('Ctrl Pts',(-6.08716037978976,-3.87017573546989,
-15.2045780432604));
#50867=CARTESIAN_POINT('Ctrl Pts',(-6.1995564342606,-3.90545408683933,-15.162827533509));
#50868=CARTESIAN_POINT('Ctrl Pts',(-6.37953440856656,-4.00078013167406,
-15.0834346606072));
#50869=CARTESIAN_POINT('Ctrl Pts',(-6.5657926704312,-4.17048213829989,-14.9781170113052));
#50870=CARTESIAN_POINT('Ctrl Pts',(-6.70320606919983,-4.3769561365539,-14.8736153645538));
#50871=CARTESIAN_POINT('Ctrl Pts',(-6.78592821391996,-4.59600742080904,
-14.7791864889897));
#50872=CARTESIAN_POINT('Ctrl Pts',(-6.81464125639214,-4.77415894173948,
-14.7123493325573));
#50873=CARTESIAN_POINT('Ctrl Pts',(-6.81720646837307,-4.87487688660176,
-14.6781178958172));
#50874=CARTESIAN_POINT('Ctrl Pts',(-6.81676488843804,-4.90507416047635,
-14.6681734327106));
#50875=CARTESIAN_POINT('Ctrl Pts',(-6.04007731699225,-3.3653514635855,-14.8038119958432));
#50876=CARTESIAN_POINT('Ctrl Pts',(-6.08856713435085,-3.37753324040758,
-14.7871067961518));
#50877=CARTESIAN_POINT('Ctrl Pts',(-6.24254103358638,-3.425594380489,-14.7312217087171));
#50878=CARTESIAN_POINT('Ctrl Pts',(-6.48501737959783,-3.55339098767982,
-14.6272481342667));
#50879=CARTESIAN_POINT('Ctrl Pts',(-6.73142927381077,-3.77609611461869,
-14.4922306969956));
#50880=CARTESIAN_POINT('Ctrl Pts',(-6.91088322984329,-4.04290408094191,
-14.3598675521506));
#50881=CARTESIAN_POINT('Ctrl Pts',(-7.01826470959118,-4.32360657295049,
-14.240582028433));
#50882=CARTESIAN_POINT('Ctrl Pts',(-7.05564360353183,-4.55181817515552,
-14.1555764233942));
#50883=CARTESIAN_POINT('Ctrl Pts',(-7.05902455314479,-4.6816266250268,-14.111509966447));
#50884=CARTESIAN_POINT('Ctrl Pts',(-7.05844486989701,-4.7206606857481,-14.0986455118703));
#50885=CARTESIAN_POINT('Ctrl Pts',(-6.2228042713461,-2.74964964265847,-14.8703245545406));
#50886=CARTESIAN_POINT('Ctrl Pts',(-6.2934601889109,-2.76762147752745,-14.846322496578));
#50887=CARTESIAN_POINT('Ctrl Pts',(-6.51688325161155,-2.8382386871185,-14.7664886202973));
#50888=CARTESIAN_POINT('Ctrl Pts',(-6.86412034506044,-3.02348438622559,
-14.6204460875284));
#50889=CARTESIAN_POINT('Ctrl Pts',(-7.21179661010534,-3.34055464141455,
-14.4339095029604));
#50890=CARTESIAN_POINT('Ctrl Pts',(-7.46226391480826,-3.71536132613924,
-14.2526191794921));
#50891=CARTESIAN_POINT('Ctrl Pts',(-7.61136964107686,-4.10673862760579,
-14.0892628607977));
#50892=CARTESIAN_POINT('Ctrl Pts',(-7.66339948514605,-4.42475343273525,
-13.9718572663327));
#50893=CARTESIAN_POINT('Ctrl Pts',(-7.66815498236441,-4.60657091398318,
-13.9102256869705));
#50894=CARTESIAN_POINT('Ctrl Pts',(-7.66734234719229,-4.66138037255722,
-13.8921454958944));
#50895=CARTESIAN_POINT('',(-7.00000966899638,-4.92966193733403,-14.7967990230951));
#50896=CARTESIAN_POINT('',(-6.99999994660866,-3.16612878336916,-14.5427417016117));
#50897=CARTESIAN_POINT('Ctrl Pts',(-7.,-4.92966193738822,-14.7967990231518));
#50898=CARTESIAN_POINT('Ctrl Pts',(-7.,-4.82655938421173,-14.7559075381302));
#50899=CARTESIAN_POINT('Ctrl Pts',(-7.,-4.73328972165707,-14.7213201925373));
#50900=CARTESIAN_POINT('Ctrl Pts',(-7.,-4.65148596355912,-14.6933836120477));
#50901=CARTESIAN_POINT('Ctrl Pts',(-7.,-4.61058408451014,-14.6794153218028));
#50902=CARTESIAN_POINT('Ctrl Pts',(-7.,-4.57256028200403,-14.6670630335082));
#50903=CARTESIAN_POINT('Ctrl Pts',(-7.,-4.53765362432334,-14.6561593075045));
#50904=CARTESIAN_POINT('Ctrl Pts',(-7.,-4.520200295483,-14.6507074445026));
#50905=CARTESIAN_POINT('Ctrl Pts',(-7.,-4.50352626970067,-14.6456161316604));
#50906=CARTESIAN_POINT('Ctrl Pts',(-7.,-4.48766007054382,-14.6408574818086));
#50907=CARTESIAN_POINT('Ctrl Pts',(-7.,-4.4797269709654,-14.6384781568827));
#50908=CARTESIAN_POINT('Ctrl Pts',(-7.,-4.47199582804335,-14.6361819977044));
#50909=CARTESIAN_POINT('Ctrl Pts',(-7.,-4.46446994884579,-14.6339652362007));
#50910=CARTESIAN_POINT('Ctrl Pts',(-7.,-4.46070700924702,-14.6328568554488));
#50911=CARTESIAN_POINT('Ctrl Pts',(-7.,-4.45699538557936,-14.6317683241155));
#50912=CARTESIAN_POINT('Ctrl Pts',(-7.,-4.45333548850481,-14.6306991714511));
#50913=CARTESIAN_POINT('Ctrl Pts',(-7.,-4.44967559143025,-14.6296300187866));
#50914=CARTESIAN_POINT('Ctrl Pts',(-7.,-4.44768768929838,-14.629049949197));
#50915=CARTESIAN_POINT('Ctrl Pts',(-7.,-4.44251138169973,-14.6275493766042));
#50916=CARTESIAN_POINT('Ctrl Pts',(-7.,-4.35969046012135,-14.6035402151185));
#50917=CARTESIAN_POINT('Ctrl Pts',(-7.,-4.27942521485861,-14.583045316773));
#50918=CARTESIAN_POINT('Ctrl Pts',(-7.,-4.20233627926549,-14.5661438464499));
#50919=CARTESIAN_POINT('Ctrl Pts',(-7.,-4.12524734367237,-14.5492423761268));
#50920=CARTESIAN_POINT('Ctrl Pts',(-7.,-4.05295709621141,-14.5361569482499));
#50921=CARTESIAN_POINT('Ctrl Pts',(-7.,-3.98143433660398,-14.5256713498039));
#50922=CARTESIAN_POINT('Ctrl Pts',(-7.,-3.83838881738911,-14.5047001529118));
#50923=CARTESIAN_POINT('Ctrl Pts',(-7.,-3.69587225506059,-14.4945152230835));
#50924=CARTESIAN_POINT('Ctrl Pts',(-7.,-3.55821948693664,-14.4973989631904));
#50925=CARTESIAN_POINT('Ctrl Pts',(-7.,-3.42056671881268,-14.5002827032973));
#50926=CARTESIAN_POINT('Ctrl Pts',(-7.,-3.28800980542072,-14.5162054735111));
#50927=CARTESIAN_POINT('Ctrl Pts',(-7.,-3.1661290724247,-14.5427417758091));
#50928=CARTESIAN_POINT('Ctrl Pts',(-6.24994600940207,-2.76546774305749,
-14.8593866792155));
#50929=CARTESIAN_POINT('Ctrl Pts',(-6.29984424415668,-2.77900840334636,
-14.8421907554761));
#50930=CARTESIAN_POINT('Ctrl Pts',(-6.3487263309393,-2.79444082765551,-14.824724359647));
#50931=CARTESIAN_POINT('Ctrl Pts',(-6.39660944973819,-2.81168414910411,
-14.8069977010491));
#50932=CARTESIAN_POINT('Ctrl Pts',(-6.40679347373321,-2.81535154596111,
-14.8032275056014));
#50933=CARTESIAN_POINT('Ctrl Pts',(-6.41693226861308,-2.81910103784002,
-14.7994454978845));
#50934=CARTESIAN_POINT('Ctrl Pts',(-6.42702592397545,-2.82293213144578,
-14.7956517160494));
#50935=CARTESIAN_POINT('Ctrl Pts',(-6.47528669444697,-2.84124973022688,
-14.777512515949));
#50936=CARTESIAN_POINT('Ctrl Pts',(-6.52251730631065,-2.86142901124132,
-14.7591047840457));
#50937=CARTESIAN_POINT('Ctrl Pts',(-6.56875184392231,-2.88342099387357,
-14.7404224436367));
#50938=CARTESIAN_POINT('Ctrl Pts',(-6.59562994595511,-2.89620586820405,
-14.7295616050155));
#50939=CARTESIAN_POINT('Ctrl Pts',(-6.62217102362711,-2.90960426555278,
-14.7186078033138));
#50940=CARTESIAN_POINT('Ctrl Pts',(-6.6483778235703,-2.92361352158998,-14.7075588234604));
#50941=CARTESIAN_POINT('Ctrl Pts',(-6.6940303125624,-2.94801777576873,-14.6883113978981));
#50942=CARTESIAN_POINT('Ctrl Pts',(-6.73865998128682,-2.97426707548207,
-14.668779879028));
#50943=CARTESIAN_POINT('Ctrl Pts',(-6.78225031116346,-3.00237511820988,
-14.648952239572));
#50944=CARTESIAN_POINT('Ctrl Pts',(-6.80367803687637,-3.01619220634853,
-14.6392055544471));
#50945=CARTESIAN_POINT('Ctrl Pts',(-6.82485408960695,-3.03045902932654,
-14.6293872670855));
#50946=CARTESIAN_POINT('Ctrl Pts',(-6.84577313284396,-3.0451803876863,-14.6194957968782));
#50947=CARTESIAN_POINT('Ctrl Pts',(-6.88817037401047,-3.07501659833921,
-14.5994484628238));
#50948=CARTESIAN_POINT('Ctrl Pts',(-6.92951466896079,-3.10671819929499,
-14.5791004207225));
#50949=CARTESIAN_POINT('Ctrl Pts',(-6.96976417942069,-3.14033372433756,
-14.5584342379362));
#50950=CARTESIAN_POINT('Ctrl Pts',(-6.97991293236787,-3.14880974441703,
-14.5532233426716));
#50951=CARTESIAN_POINT('Ctrl Pts',(-6.98999186172936,-3.15740758124442,
-14.5479922288204));
#50952=CARTESIAN_POINT('Ctrl Pts',(-6.99999983624227,-3.16612827049482,
-14.5427406396167));
#50953=CARTESIAN_POINT('Ctrl Pts',(-6.26385672821774,-3.90575168809173,
-15.8144219056792));
#50954=CARTESIAN_POINT('Ctrl Pts',(-6.29496070557119,-3.91447746283058,
-15.7944156170949));
#50955=CARTESIAN_POINT('Ctrl Pts',(-6.32584063897265,-3.92481222694173,
-15.7736495821958));
#50956=CARTESIAN_POINT('Ctrl Pts',(-6.35632273915694,-3.93678606640697,
-15.7521476173342));
#50957=CARTESIAN_POINT('Ctrl Pts',(-6.40025562382785,-3.95404358164096,
-15.7211575170211));
#50958=CARTESIAN_POINT('Ctrl Pts',(-6.44336383185676,-3.97470665376692,
-15.688637704132));
#50959=CARTESIAN_POINT('Ctrl Pts',(-6.48515831758161,-3.99873227768996,
-15.6546924201779));
#50960=CARTESIAN_POINT('Ctrl Pts',(-6.51589372349728,-4.01640057270173,
-15.6297292686244));
#50961=CARTESIAN_POINT('Ctrl Pts',(-6.54591786321893,-4.03588708150959,
-15.6039955938197));
#50962=CARTESIAN_POINT('Ctrl Pts',(-6.57501945966857,-4.05717477201828,
-15.5775396377571));
#50963=CARTESIAN_POINT('Ctrl Pts',(-6.57561881429194,-4.05761319730362,
-15.5769947707561));
#50964=CARTESIAN_POINT('Ctrl Pts',(-6.57621777705022,-4.05805238665068,
-15.5764495976003));
#50965=CARTESIAN_POINT('Ctrl Pts',(-6.57681634635688,-4.0584923394855,-15.5759041187764));
#50966=CARTESIAN_POINT('Ctrl Pts',(-6.61481470367452,-4.0864214110811,-15.5412760497653));
#50967=CARTESIAN_POINT('Ctrl Pts',(-6.65123111078806,-4.11742775113867,
-15.505414438286));
#50968=CARTESIAN_POINT('Ctrl Pts',(-6.68563918955076,-4.15136225110879,
-15.4684540374091));
#50969=CARTESIAN_POINT('Ctrl Pts',(-6.71047710027362,-4.17585830293707,
-15.441773700399));
#50970=CARTESIAN_POINT('Ctrl Pts',(-6.73426779502671,-4.20187999599657,
-15.4145211940823));
#50971=CARTESIAN_POINT('Ctrl Pts',(-6.75683528395995,-4.2293715007421,-15.3867541360492));
#50972=CARTESIAN_POINT('Ctrl Pts',(-6.76261505054204,-4.23641235853934,
-15.3796427062141));
#50973=CARTESIAN_POINT('Ctrl Pts',(-6.76831450584281,-4.24354963337093,
-15.3724975569579));
#50974=CARTESIAN_POINT('Ctrl Pts',(-6.77393124261298,-4.25078171331711,
-15.3653197709766));
#50975=CARTESIAN_POINT('Ctrl Pts',(-6.78358602365561,-4.26321315727118,
-15.3529816545836));
#50976=CARTESIAN_POINT('Ctrl Pts',(-6.79299642325081,-4.27592472578274,
-15.3405470914351));
#50977=CARTESIAN_POINT('Ctrl Pts',(-6.80214982425869,-4.28890819117643,
-15.3280217832807));
#50978=CARTESIAN_POINT('Ctrl Pts',(-6.80672652476263,-4.29539992387327,
-15.3217591292036));
#50979=CARTESIAN_POINT('Ctrl Pts',(-6.81123897066713,-4.30195963441504,
-15.3154737890702));
#50980=CARTESIAN_POINT('Ctrl Pts',(-6.81568553119839,-4.30858628652225,
-15.3091665045848));
#50981=CARTESIAN_POINT('Ctrl Pts',(-6.81790881146402,-4.31189961257586,
-15.3060128623421));
#50982=CARTESIAN_POINT('Ctrl Pts',(-6.82011562004755,-4.31522967427845,
-15.3028537340249));
#50983=CARTESIAN_POINT('Ctrl Pts',(-6.82230575025301,-4.31857634267313,
-15.2996892133226));
#50984=CARTESIAN_POINT('Ctrl Pts',(-6.82390724309922,-4.32102353301795,
-15.2973752151623));
#50985=CARTESIAN_POINT('Ctrl Pts',(-6.82591988230215,-4.32413073507111,
-15.2944445695705));
#50986=CARTESIAN_POINT('Ctrl Pts',(-6.82742098616778,-4.32647033414201,
-15.2922436785592));
#50987=CARTESIAN_POINT('Ctrl Pts',(-6.82797272501414,-4.3273302664371,-15.2914347291618));
#50988=CARTESIAN_POINT('Ctrl Pts',(-6.82845586142347,-4.32808612215464,
-15.2907243891491));
#50989=CARTESIAN_POINT('Ctrl Pts',(-6.82882589711254,-4.32866603950762,
-15.2901795682984));
#50990=CARTESIAN_POINT('Ctrl Pts',(-6.84354636430377,-4.35173585309678,
-15.2685059360108));
#50991=CARTESIAN_POINT('Ctrl Pts',(-6.85802914311084,-4.37643135241196,
-15.2457503303666));
#50992=CARTESIAN_POINT('Ctrl Pts',(-6.8719932617384,-4.40284622357026,-15.2219432148758));
#50993=CARTESIAN_POINT('Ctrl Pts',(-6.87753155881442,-4.41332260289653,
-15.2125010952815));
#50994=CARTESIAN_POINT('Ctrl Pts',(-6.88298778531057,-4.42406926830202,
-15.2028937746778));
#50995=CARTESIAN_POINT('Ctrl Pts',(-6.88834236978538,-4.43509135495778,
-15.1931240035397));
#50996=CARTESIAN_POINT('Ctrl Pts',(-6.90122774509452,-4.46161511677671,
-15.1696138379252));
#50997=CARTESIAN_POINT('Ctrl Pts',(-6.91352688599134,-4.48973564698527,
-15.1451614820643));
#50998=CARTESIAN_POINT('Ctrl Pts',(-6.92496496488142,-4.5194897156191,-15.1198210062146));
#50999=CARTESIAN_POINT('Ctrl Pts',(-6.93265775367141,-4.53950109758651,
-15.1027780280691));
#51000=CARTESIAN_POINT('Ctrl Pts',(-6.93996038631962,-4.56025090255248,
-15.0853337152217));
#51001=CARTESIAN_POINT('Ctrl Pts',(-6.94677915170763,-4.58174363379248,
-15.0675102808871));
#51002=CARTESIAN_POINT('Ctrl Pts',(-6.95371914500644,-4.60361847510039,
-15.0493699713434));
#51003=CARTESIAN_POINT('Ctrl Pts',(-6.96015804529918,-4.62626292645609,
-15.0308368775598));
#51004=CARTESIAN_POINT('Ctrl Pts',(-6.96598676876777,-4.64967549092573,
-15.0119400880676));
#51005=CARTESIAN_POINT('Ctrl Pts',(-6.97384657551408,-4.68124642290739,
-14.9864585028913));
#51006=CARTESIAN_POINT('Ctrl Pts',(-6.98059788182425,-4.71421565278788,
-14.9603145265921));
#51007=CARTESIAN_POINT('Ctrl Pts',(-6.98597534825046,-4.74853165282223,
-14.9336023621482));
#51008=CARTESIAN_POINT('Ctrl Pts',(-6.99135281467668,-4.78284765285657,
-14.9068901977044));
#51009=CARTESIAN_POINT('Ctrl Pts',(-6.99535715189965,-4.81851060906578,
-14.8796095675904));
#51010=CARTESIAN_POINT('Ctrl Pts',(-6.99768410298933,-4.85543612803544,
-14.8518810527172));
#51011=CARTESIAN_POINT('Ctrl Pts',(-6.99920998548749,-4.8796497882972,-14.8336982659226));
#51012=CARTESIAN_POINT('Ctrl Pts',(-7.00001358933039,-4.90440581697676,
-14.8153234008063));
#51013=CARTESIAN_POINT('Ctrl Pts',(-7.00001301944785,-4.92966193744617,
-14.7967990231449));
#51014=CARTESIAN_POINT('Ctrl Pts',(-6.22833844179566,-8.85454586402646,
-25.6432279269192));
#51015=CARTESIAN_POINT('Ctrl Pts',(-6.2291146949257,-8.44340768883296,-25.3458769589811));
#51016=CARTESIAN_POINT('Ctrl Pts',(-6.23070504669655,-7.53909867425292,
-24.6003976212981));
#51017=CARTESIAN_POINT('Ctrl Pts',(-6.23225398339099,-6.30570986941791,
-23.2360111793486));
#51018=CARTESIAN_POINT('Ctrl Pts',(-6.23180618158922,-5.23101094495107,
-21.5552478274574));
#51019=CARTESIAN_POINT('Ctrl Pts',(-6.22991430233278,-4.44858169421722,
-19.7183955817659));
#51020=CARTESIAN_POINT('Ctrl Pts',(-6.22625526139252,-3.98055545467836,
-17.7796362264324));
#51021=CARTESIAN_POINT('Ctrl Pts',(-6.22146023609855,-3.85842008520426,
-16.046045618656));
#51022=CARTESIAN_POINT('Ctrl Pts',(-6.21819598059103,-3.92587530766592,
-14.9770433487066));
#51023=CARTESIAN_POINT('Ctrl Pts',(-6.21685873948199,-3.97244993924363,
-14.5712621246747));
#51024=CARTESIAN_POINT('Ctrl Pts',(-6.72318434148056,-8.92252624598781,
-25.5491630136165));
#51025=CARTESIAN_POINT('Ctrl Pts',(-6.72388041677531,-8.51560341410963,
-25.2543690324476));
#51026=CARTESIAN_POINT('Ctrl Pts',(-6.72525502274418,-7.62056569287233,
-24.5154728102739));
#51027=CARTESIAN_POINT('Ctrl Pts',(-6.72662850357054,-6.40000803919394,
-23.1640897398429));
#51028=CARTESIAN_POINT('Ctrl Pts',(-6.72623178592576,-5.33567942894206,
-21.499981562341));
#51029=CARTESIAN_POINT('Ctrl Pts',(-6.7245683841393,-4.56007598310717,-19.6816180801987));
#51030=CARTESIAN_POINT('Ctrl Pts',(-6.72135051761313,-4.09475438480478,
-17.7621504532083));
#51031=CARTESIAN_POINT('Ctrl Pts',(-6.71710127101458,-3.97131583603131,
-16.0452264577192));
#51032=CARTESIAN_POINT('Ctrl Pts',(-6.7142340588082,-4.03648107493104,-14.9860221510941));
#51033=CARTESIAN_POINT('Ctrl Pts',(-6.71304026512286,-4.0819462151573,-14.5839118639174));
#51034=CARTESIAN_POINT('Ctrl Pts',(-7.02734369613163,-9.16102046075851,
-25.2191575822356));
#51035=CARTESIAN_POINT('Ctrl Pts',(-7.02772459263739,-8.76821649492092,
-24.9342613568181));
#51036=CARTESIAN_POINT('Ctrl Pts',(-7.02841406477176,-7.90406911102415,
-24.2201590873639));
#51037=CARTESIAN_POINT('Ctrl Pts',(-7.02914679556069,-6.72625932453338,
-22.9153222295337));
#51038=CARTESIAN_POINT('Ctrl Pts',(-7.02893559561167,-5.69830277108108,
-21.3083981705397));
#51039=CARTESIAN_POINT('Ctrl Pts',(-7.02806566033587,-4.94894652445456,
-19.5531153239726));
#51040=CARTESIAN_POINT('Ctrl Pts',(-7.02638186928547,-4.49837668820159,
-17.6999558310792));
#51041=CARTESIAN_POINT('Ctrl Pts',(-7.02411819232694,-4.3775348597053,-16.0419479461919));
#51042=CARTESIAN_POINT('Ctrl Pts',(-7.02262219464857,-4.43938017157472,
-15.0186573153932));
#51043=CARTESIAN_POINT('Ctrl Pts',(-7.0219754326037,-4.48283582413942,-14.6302246026994));
#51044=CARTESIAN_POINT('Ctrl Pts',(-6.99838063008314,-9.45820150649603,
-24.80794711765));
#51045=CARTESIAN_POINT('Ctrl Pts',(-6.99835913457881,-9.08279985143789,
-24.5356483641088));
#51046=CARTESIAN_POINT('Ctrl Pts',(-6.99821532661173,-8.25667795636497,
-23.852925090981));
#51047=CARTESIAN_POINT('Ctrl Pts',(-6.99814245618034,-7.13148909047522,
-22.6063522236937));
#51048=CARTESIAN_POINT('Ctrl Pts',(-6.99816421970605,-6.14885192790038,
-21.070328455353));
#51049=CARTESIAN_POINT('Ctrl Pts',(-6.99828069432312,-5.43285699584306,
-19.3931406078209));
#51050=CARTESIAN_POINT('Ctrl Pts',(-6.9985045724283,-5.00216845859944,-17.6222147600737));
#51051=CARTESIAN_POINT('Ctrl Pts',(-6.9987352379504,-4.88660477512488,-16.0377473888359));
#51052=CARTESIAN_POINT('Ctrl Pts',(-6.99894168315531,-4.94565629452344,
-15.0596464715112));
#51053=CARTESIAN_POINT('Ctrl Pts',(-6.99898903503866,-4.98714444952959,
-14.6884846237969));
#51054=CARTESIAN_POINT('',(-7.00000308919771,-9.33251796322024,-24.7867179209035));
#51055=CARTESIAN_POINT('Origin',(-5.99998370363197,-9.33252808557812,-24.7867138051333));
#51056=CARTESIAN_POINT('Ctrl Pts',(-7.00001101651463,-9.33251828870258,
-24.7867134185486));
#51057=CARTESIAN_POINT('Ctrl Pts',(-7.00001786889538,-9.17932096987487,
-24.6735525287245));
#51058=CARTESIAN_POINT('Ctrl Pts',(-7.00001802523764,-9.03121143047395,
-24.5580142123416));
#51059=CARTESIAN_POINT('Ctrl Pts',(-7.00001556839827,-8.88816514599322,
-24.4406109868492));
#51060=CARTESIAN_POINT('Ctrl Pts',(-7.00001306417584,-8.74236004418057,
-24.320943500845));
#51061=CARTESIAN_POINT('Ctrl Pts',(-7.00000784356451,-8.60181528010428,
-24.1993384527498));
#51062=CARTESIAN_POINT('Ctrl Pts',(-7.00000354838409,-8.4664713655905,-24.0762961134802));
#51063=CARTESIAN_POINT('Ctrl Pts',(-7.00000225630549,-8.42575713295274,
-24.0392824476401));
#51064=CARTESIAN_POINT('Ctrl Pts',(-7.00000104345516,-8.38551332065751,
-24.0021384319859));
#51065=CARTESIAN_POINT('Ctrl Pts',(-6.99999999753994,-8.34573775429907,
-23.9648769595113));
#51066=CARTESIAN_POINT('Ctrl Pts',(-6.99999887666334,-8.30311144841288,
-23.924944934178));
#51067=CARTESIAN_POINT('Ctrl Pts',(-6.99999794690503,-8.26102290376838,
-23.8848780147828));
#51068=CARTESIAN_POINT('Ctrl Pts',(-6.99999718086759,-8.21946689146059,
-23.8446913566483));
#51069=CARTESIAN_POINT('Ctrl Pts',(-6.9999946221417,-8.08066108527976,-23.7104594809152));
#51070=CARTESIAN_POINT('Ctrl Pts',(-6.99999387750149,-7.94779827828375,
-23.5748953731845));
#51071=CARTESIAN_POINT('Ctrl Pts',(-6.99999403434654,-7.82067002322657,
-23.4385317151514));
#51072=CARTESIAN_POINT('Ctrl Pts',(-6.99999406716621,-7.79406856362658,
-23.4099977567608));
#51073=CARTESIAN_POINT('Ctrl Pts',(-6.99999414003161,-7.76771812286174,
-23.3814286214255));
#51074=CARTESIAN_POINT('Ctrl Pts',(-6.99999424548565,-7.74161668390431,
-23.3528289250926));
#51075=CARTESIAN_POINT('Ctrl Pts',(-6.99999432422097,-7.7221285250655,-23.3314754883804));
#51076=CARTESIAN_POINT('Ctrl Pts',(-6.99999441863014,-7.70323909902872,
-23.3106151714184));
#51077=CARTESIAN_POINT('Ctrl Pts',(-6.9999945313887,-7.68388254652659,-23.2890698050573));
#51078=CARTESIAN_POINT('Ctrl Pts',(-6.99999463682047,-7.66578373583508,
-23.2689244043199));
#51079=CARTESIAN_POINT('Ctrl Pts',(-6.99999475847151,-7.64727658542074,
-23.2481799736132));
#51080=CARTESIAN_POINT('Ctrl Pts',(-6.99999490350817,-7.62752046923564,
-23.2258462598882));
#51081=CARTESIAN_POINT('Ctrl Pts',(-6.99999520366053,-7.58663532381801,
-23.1796267942398));
#51082=CARTESIAN_POINT('Ctrl Pts',(-6.99999556265644,-7.5462152748296,-23.1331495451411));
#51083=CARTESIAN_POINT('Ctrl Pts',(-6.99999595370125,-7.50626142519057,
-23.0864243731837));
#51084=CARTESIAN_POINT('Ctrl Pts',(-6.99999673579089,-7.42635372591251,
-22.9929740292688));
#51085=CARTESIAN_POINT('Ctrl Pts',(-6.9999976453721,-7.34831082403186,-22.8985319939186));
#51086=CARTESIAN_POINT('Ctrl Pts',(-6.99999847632113,-7.27213997300368,
-22.8031750086351));
#51087=CARTESIAN_POINT('Ctrl Pts',(-6.99999902465851,-7.22187536817392,
-22.7402496097675));
#51088=CARTESIAN_POINT('Ctrl Pts',(-6.99999953897951,-7.17242592969274,
-22.6769257410983));
#51089=CARTESIAN_POINT('Ctrl Pts',(-6.9999999627666,-7.12379334406456,-22.6132249099148));
#51090=CARTESIAN_POINT('Ctrl Pts',(-7.00000126736881,-6.97408094982872,
-22.4171258576411));
#51091=CARTESIAN_POINT('Ctrl Pts',(-7.00000171385125,-6.83211151967692,
-22.2174579363025));
#51092=CARTESIAN_POINT('Ctrl Pts',(-7.00000170643198,-6.69789034495963,
-22.014913879793));
#51093=CARTESIAN_POINT('Ctrl Pts',(-7.00000169893338,-6.56223404405374,
-21.810204171847));
#51094=CARTESIAN_POINT('Ctrl Pts',(-7.00000122940867,-6.4344925417275,-21.6025564694009));
#51095=CARTESIAN_POINT('Ctrl Pts',(-7.00000072341992,-6.31464617992324,
-21.392638892529));
#51096=CARTESIAN_POINT('Ctrl Pts',(-7.00000046988391,-6.25459471218963,
-21.2874554025634));
#51097=CARTESIAN_POINT('Ctrl Pts',(-7.00000020716497,-6.19652510160297,
-21.1817012804143));
#51098=CARTESIAN_POINT('Ctrl Pts',(-6.99999998766523,-6.14043258691257,
-21.0754562422842));
#51099=CARTESIAN_POINT('Ctrl Pts',(-6.99999993929019,-6.12807048608338,
-21.0520411416916));
#51100=CARTESIAN_POINT('Ctrl Pts',(-6.99999989300829,-6.11580440838993,
-21.0286021859978));
#51101=CARTESIAN_POINT('Ctrl Pts',(-6.99999984878697,-6.10363415345454,
-21.0051402391711));
#51102=CARTESIAN_POINT('Ctrl Pts',(-6.99999965374735,-6.0499568442152,-20.9016605518631));
#51103=CARTESIAN_POINT('Ctrl Pts',(-6.99999949863779,-5.99814361467508,
-20.7977338296875));
#51104=CARTESIAN_POINT('Ctrl Pts',(-6.9999993818455,-5.94817680819026,-20.6934325636233));
#51105=CARTESIAN_POINT('Ctrl Pts',(-6.99999932344936,-5.92319340494786,
-20.6412819305913));
#51106=CARTESIAN_POINT('Ctrl Pts',(-6.99999927466384,-5.89867160746928,
-20.5890376615871));
#51107=CARTESIAN_POINT('Ctrl Pts',(-6.99999923547135,-5.8746091259089,-20.5367085252783));
#51108=CARTESIAN_POINT('Ctrl Pts',(-6.9999992158751,-5.86257788512872,-20.5105439571239));
#51109=CARTESIAN_POINT('Ctrl Pts',(-6.99999919867913,-5.85066147332808,
-20.4843581721434));
#51110=CARTESIAN_POINT('Ctrl Pts',(-6.99999918389319,-5.83885960187496,
-20.4581522577767));
#51111=CARTESIAN_POINT('Ctrl Pts',(-6.99999917282788,-5.8300274615195,-20.4385405957831));
#51112=CARTESIAN_POINT('Ctrl Pts',(-6.99999916268463,-5.82084773603849,
-20.4179924260146));
#51113=CARTESIAN_POINT('Ctrl Pts',(-6.99999915445597,-5.81224570769022,
-20.3985849979498));
#51114=CARTESIAN_POINT('Ctrl Pts',(-6.99999915168916,-5.80935334977234,
-20.3920594174755));
#51115=CARTESIAN_POINT('Ctrl Pts',(-6.99999914912877,-5.80652589333689,
-20.3856629904652));
#51116=CARTESIAN_POINT('Ctrl Pts',(-6.99999914678332,-5.80379731854171,
-20.3794752090212));
#51117=CARTESIAN_POINT('Ctrl Pts',(-6.99999907528831,-5.72062372100036,
-20.1908565776373));
#51118=CARTESIAN_POINT('Ctrl Pts',(-6.99999912491173,-5.64168485177726,
-19.9974675568945));
#51119=CARTESIAN_POINT('Ctrl Pts',(-6.99999933315401,-5.56752053115335,
-19.799448619423));
#51120=CARTESIAN_POINT('Ctrl Pts',(-6.99999947285253,-5.51776768741775,
-19.6666083915368));
#51121=CARTESIAN_POINT('Ctrl Pts',(-6.99999968442923,-5.47016412906179,
-19.5316853935006));
#51122=CARTESIAN_POINT('Ctrl Pts',(-6.99999998816759,-5.42488006699747,
-19.3947330698664));
#51123=CARTESIAN_POINT('Ctrl Pts',(-7.00000042904109,-5.35915065807392,
-19.1959480034915));
#51124=CARTESIAN_POINT('Ctrl Pts',(-7.00000106781889,-5.29830713940259,
-18.9928852940146));
#51125=CARTESIAN_POINT('Ctrl Pts',(-7.0000015333283,-5.24286447796379,-18.7857677797069));
#51126=CARTESIAN_POINT('Ctrl Pts',(-7.00000199136861,-5.18831139407053,
-18.581973466076));
#51127=CARTESIAN_POINT('Ctrl Pts',(-7.00000228134199,-5.13898725835631,
-18.374253365063));
#51128=CARTESIAN_POINT('Ctrl Pts',(-7.00000202664206,-5.09540487226898,
-18.1628646067693));
#51129=CARTESIAN_POINT('Ctrl Pts',(-7.00000181210231,-5.05869440086198,
-17.9848068714367));
#51130=CARTESIAN_POINT('Ctrl Pts',(-7.0000012106348,-5.02605811693811,-17.8041468995805));
#51131=CARTESIAN_POINT('Ctrl Pts',(-6.99999998662388,-4.99781498742711,
-17.621064245929));
#51132=CARTESIAN_POINT('Ctrl Pts',(-6.99999852879686,-4.96417672770832,
-17.4030083165697));
#51133=CARTESIAN_POINT('Ctrl Pts',(-6.99999617281986,-4.93677080969977,
-17.1815144133228));
#51134=CARTESIAN_POINT('Ctrl Pts',(-6.99999449839166,-4.91605443570459,
-16.9569257573727));
#51135=CARTESIAN_POINT('Ctrl Pts',(-6.99999284818615,-4.89563774996922,
-16.735586057224));
#51136=CARTESIAN_POINT('Ctrl Pts',(-6.99999186150181,-4.88171848710305,
-16.5112404439615));
#51137=CARTESIAN_POINT('Ctrl Pts',(-6.99999320063151,-4.87474450353124,
-16.2842667780983));
#51138=CARTESIAN_POINT('Ctrl Pts',(-6.99999413392965,-4.86988402894972,
-16.1260788898933));
#51139=CARTESIAN_POINT('Ctrl Pts',(-6.9999962001064,-4.86839730041592,-15.9666154928942));
#51140=CARTESIAN_POINT('Ctrl Pts',(-6.9999999996549,-4.87043884390324,-15.8060192338875));
#51141=CARTESIAN_POINT('Ctrl Pts',(-7.00000506889263,-4.87316260680444,
-15.5917567726317));
#51142=CARTESIAN_POINT('Ctrl Pts',(-7.00001329864277,-4.88216671047696,
-15.3754753996994));
#51143=CARTESIAN_POINT('Ctrl Pts',(-7.00001657746181,-4.89779557086446,
-15.1576383695357));
#51144=CARTESIAN_POINT('Ctrl Pts',(-7.00001838122561,-4.90639341427219,
-15.0378005421243));
#51145=CARTESIAN_POINT('Ctrl Pts',(-7.00001867170191,-4.91699624108351,
-14.917492806888));
#51146=CARTESIAN_POINT('Ctrl Pts',(-7.00001598754129,-4.92966193716263,
-14.7967990229923));
#51147=CARTESIAN_POINT('Origin',(-5.9999949808,-9.33250914740362,-24.7867195890602));
#51148=CARTESIAN_POINT('Origin',(-6.,-9.33251101143268,-24.7867243677925));
#51149=CARTESIAN_POINT('Ctrl Pts',(-7.10572058681599,-7.15917451980105,
-14.3583562946813));
#51150=CARTESIAN_POINT('Ctrl Pts',(-7.10645540380474,-7.20568112961659,
-14.3348966367294));
#51151=CARTESIAN_POINT('Ctrl Pts',(-7.10076650948181,-7.33448368577117,
-14.271997245283));
#51152=CARTESIAN_POINT('Ctrl Pts',(-7.05594826294389,-7.55240332663308,
-14.1748898295926));
#51153=CARTESIAN_POINT('Ctrl Pts',(-6.95114004312909,-7.80056170268336,
-14.0785538117247));
#51154=CARTESIAN_POINT('Ctrl Pts',(-6.79944482822535,-8.0256849068933,-14.0064757496486));
#51155=CARTESIAN_POINT('Ctrl Pts',(-6.6208277696206,-8.20816691621563,-13.9635191964736));
#51156=CARTESIAN_POINT('Ctrl Pts',(-6.43625208840588,-8.34296075927564,
-13.94674598393));
#51157=CARTESIAN_POINT('Ctrl Pts',(-6.30967320710823,-8.40903533450593,
-13.9489256328214));
#51158=CARTESIAN_POINT('Ctrl Pts',(-6.24787426415866,-8.43565318561558,
-13.9529403897452));
#51159=CARTESIAN_POINT('Ctrl Pts',(-6.24577684234737,-8.4365502147327,-13.9530799785798));
#51160=CARTESIAN_POINT('Ctrl Pts',(-6.81553757384515,-6.90211824706944,
-13.8389932456361));
#51161=CARTESIAN_POINT('Ctrl Pts',(-6.81619657719427,-6.94305640662117,
-13.8183320344138));
#51162=CARTESIAN_POINT('Ctrl Pts',(-6.81109453262395,-7.0566538750647,-13.7629367837621));
#51163=CARTESIAN_POINT('Ctrl Pts',(-6.77074846063708,-7.2494690894213,-13.6776278902152));
#51164=CARTESIAN_POINT('Ctrl Pts',(-6.67638498400727,-7.4692644419055,-13.5936470267869));
#51165=CARTESIAN_POINT('Ctrl Pts',(-6.5401230543666,-7.6684107429182,-13.5316591804317));
#51166=CARTESIAN_POINT('Ctrl Pts',(-6.38028567734501,-7.82939787216426,
-13.4955946842181));
#51167=CARTESIAN_POINT('Ctrl Pts',(-6.21586083447959,-7.94790647752958,
-13.4824388050648));
#51168=CARTESIAN_POINT('Ctrl Pts',(-6.10363915270979,-8.00579354685784,
-13.4852140513868));
#51169=CARTESIAN_POINT('Ctrl Pts',(-6.04899678238557,-8.02908142810832,
-13.4890768959804));
#51170=CARTESIAN_POINT('Ctrl Pts',(-6.04714241757874,-8.02986619471148,
-13.4892108277678));
#51171=CARTESIAN_POINT('Ctrl Pts',(-7.05965280425926,-6.62889424957639,
-13.3045937670833));
#51172=CARTESIAN_POINT('Ctrl Pts',(-7.060521616384,-6.68192398646321,-13.2778453838265));
#51173=CARTESIAN_POINT('Ctrl Pts',(-7.05379562531041,-6.82834107794673,
-13.2063351599417));
#51174=CARTESIAN_POINT('Ctrl Pts',(-7.00126479150212,-7.07498363172971,
-13.0963249144846));
#51175=CARTESIAN_POINT('Ctrl Pts',(-6.87846148914097,-7.35614255519393,
-12.9869832809918));
#51176=CARTESIAN_POINT('Ctrl Pts',(-6.69976369750449,-7.6127989981063,-12.9046724354872));
#51177=CARTESIAN_POINT('Ctrl Pts',(-6.48751180965009,-7.82290039043415,
-12.8552879569376));
#51178=CARTESIAN_POINT('Ctrl Pts',(-6.26592339562598,-7.97997497096265,
-12.8360886525733));
#51179=CARTESIAN_POINT('Ctrl Pts',(-6.11233174024832,-8.05802853807378,
-12.8390651949399));
#51180=CARTESIAN_POINT('Ctrl Pts',(-6.03689908271419,-8.08970313051234,
-12.8440931022415));
#51181=CARTESIAN_POINT('Ctrl Pts',(-6.03433843459531,-8.0907708844276,-12.8442677853705));
#51182=CARTESIAN_POINT('Ctrl Pts',(-7.67146636779035,-6.52533423325674,
-13.1186084728563));
#51183=CARTESIAN_POINT('Ctrl Pts',(-7.67268761324267,-6.59987309890137,
-13.0810367414559));
#51184=CARTESIAN_POINT('Ctrl Pts',(-7.66323370103255,-6.80476224377587,
-12.9807776285539));
#51185=CARTESIAN_POINT('Ctrl Pts',(-7.59016592525227,-7.14747102909554,
-12.8264048102834));
#51186=CARTESIAN_POINT('Ctrl Pts',(-7.41942193955388,-7.53789024560707,
-12.6712749171081));
#51187=CARTESIAN_POINT('Ctrl Pts',(-7.16934195304591,-7.89634143968295,
-12.5520822507266));
#51188=CARTESIAN_POINT('Ctrl Pts',(-6.86920496992593,-8.19268769913783,
-12.4782464203487));
#51189=CARTESIAN_POINT('Ctrl Pts',(-6.55209859046718,-8.41689177268628,
-12.447463467991));
#51190=CARTESIAN_POINT('Ctrl Pts',(-6.32960538007574,-8.52972012494187,
-12.4501105372351));
#51191=CARTESIAN_POINT('Ctrl Pts',(-6.2196050747502,-8.57578171275077,-12.4568267120036));
#51192=CARTESIAN_POINT('Ctrl Pts',(-6.2158701662133,-8.57733481926968,-12.4570607901429));
#51193=CARTESIAN_POINT('',(-6.26383832463082,-8.42072097704164,-13.9442592301454));
#51194=CARTESIAN_POINT('',(-6.24991285392751,-8.55170704998985,-12.4626562658216));
#51195=CARTESIAN_POINT('Origin',(-6.527651908718,-9.09524965967693,-13.2547563604596));
#51196=CARTESIAN_POINT('',(-6.99999988440685,-8.04449912265075,-12.5220505110564));
#51197=CARTESIAN_POINT('Ctrl Pts',(-6.99999985665133,-8.04449905185795,
-12.5220503391613));
#51198=CARTESIAN_POINT('Ctrl Pts',(-6.96289538607134,-8.08112540801169,
-12.5129574216944));
#51199=CARTESIAN_POINT('Ctrl Pts',(-6.92537693594424,-8.11580955524739,
-12.5049945056296));
#51200=CARTESIAN_POINT('Ctrl Pts',(-6.88761335220619,-8.14868195423147,
-12.4980582408632));
#51201=CARTESIAN_POINT('Ctrl Pts',(-6.87240071834141,-8.16192422947395,
-12.4952640448194));
#51202=CARTESIAN_POINT('Ctrl Pts',(-6.85714770636048,-8.17487251418294,
-12.4926365701431));
#51203=CARTESIAN_POINT('Ctrl Pts',(-6.84186306168057,-8.1875353341046,-12.4901695537855));
#51204=CARTESIAN_POINT('Ctrl Pts',(-6.81126970633746,-8.2128809118149,-12.4852316367028));
#51205=CARTESIAN_POINT('Ctrl Pts',(-6.78055089186904,-8.23708299873428,
-12.4809361823432));
#51206=CARTESIAN_POINT('Ctrl Pts',(-6.74977181316329,-8.26021088679133,
-12.4772329615929));
#51207=CARTESIAN_POINT('Ctrl Pts',(-6.70541234527646,-8.2935432947352,-12.4718958004802));
#51208=CARTESIAN_POINT('Ctrl Pts',(-6.66093157460354,-8.32464562527117,
-12.4677866114349));
#51209=CARTESIAN_POINT('Ctrl Pts',(-6.61657594962318,-8.35365273204861,
-12.464775146045));
#51210=CARTESIAN_POINT('Ctrl Pts',(-6.58742401213129,-8.37271713174924,
-12.4627959145305));
#51211=CARTESIAN_POINT('Ctrl Pts',(-6.55832498198079,-8.3908767719984,-12.4612909391321));
#51212=CARTESIAN_POINT('Ctrl Pts',(-6.52933699125688,-8.40817228213706,
-12.4602244920139));
#51213=CARTESIAN_POINT('Ctrl Pts',(-6.51858346639462,-8.41458830800284,
-12.4598288776469));
#51214=CARTESIAN_POINT('Ctrl Pts',(-6.50784513713682,-8.42088543195715,
-12.4594936210241));
#51215=CARTESIAN_POINT('Ctrl Pts',(-6.49712495711951,-8.42706586839688,
-12.4592167863404));
#51216=CARTESIAN_POINT('Ctrl Pts',(-6.45533111070439,-8.45116100587812,
-12.4581375147016));
#51217=CARTESIAN_POINT('Ctrl Pts',(-6.41381168142764,-8.47347393917319,
-12.4579532736844));
#51218=CARTESIAN_POINT('Ctrl Pts',(-6.37260897169576,-8.49418774960732,
-12.4585576701757));
#51219=CARTESIAN_POINT('Ctrl Pts',(-6.33140626196388,-8.51490156004145,
-12.459162066667));
#51220=CARTESIAN_POINT('Ctrl Pts',(-6.29051957134565,-8.53401642514046,
-12.4605551619981));
#51221=CARTESIAN_POINT('Ctrl Pts',(-6.24994618220503,-8.5516924285248,-12.4626545731639));
#51222=CARTESIAN_POINT('',(-7.000009545786,-6.97711952667737,-13.9487142983806));
#51223=CARTESIAN_POINT('Ctrl Pts',(-7.000009545786,-6.97711952667737,-13.9487142983806));
#51224=CARTESIAN_POINT('Ctrl Pts',(-7.,-7.01445409933478,-13.8623191189325));
#51225=CARTESIAN_POINT('Ctrl Pts',(-7.,-7.07990718347488,-13.7190290853873));
#51226=CARTESIAN_POINT('Ctrl Pts',(-7.,-7.14556603609682,-13.589566730198));
#51227=CARTESIAN_POINT('Ctrl Pts',(-7.,-7.18313577273348,-13.518974611728));
#51228=CARTESIAN_POINT('Ctrl Pts',(-7.,-7.1919711816871,-13.5026286632352));
#51229=CARTESIAN_POINT('Ctrl Pts',(-7.,-7.28162969860235,-13.3396969995268));
#51230=CARTESIAN_POINT('Ctrl Pts',(-7.,-7.36735477671998,-13.2056608545378));
#51231=CARTESIAN_POINT('Ctrl Pts',(-7.,-7.63341057490925,-12.8482930275621));
#51232=CARTESIAN_POINT('Ctrl Pts',(-7.,-7.82956349063113,-12.660130291256));
#51233=CARTESIAN_POINT('Ctrl Pts',(-6.999999792337,-8.04449878994872,-12.5220500366276));
#51234=CARTESIAN_POINT('Ctrl Pts',(-7.00001601661457,-6.97711952672703,
-13.9487142980922));
#51235=CARTESIAN_POINT('Ctrl Pts',(-7.00001543846632,-7.01692337104545,
-13.9425963489463));
#51236=CARTESIAN_POINT('Ctrl Pts',(-6.99868096797267,-7.05610076819487,
-13.9368182972979));
#51237=CARTESIAN_POINT('Ctrl Pts',(-6.99616776089911,-7.09452829561729,
-13.9314343716914));
#51238=CARTESIAN_POINT('Ctrl Pts',(-6.99356689649137,-7.13429612430183,
-13.9258626618902));
#51239=CARTESIAN_POINT('Ctrl Pts',(-6.9897046355072,-7.17326074439687,-13.9207129642798));
#51240=CARTESIAN_POINT('Ctrl Pts',(-6.98475617023165,-7.21131869021076,
-13.9160002389077));
#51241=CARTESIAN_POINT('Ctrl Pts',(-6.9797033920153,-7.25017889208334,-13.9111881699584));
#51242=CARTESIAN_POINT('Ctrl Pts',(-6.97351904010826,-7.28809395023687,
-13.9068312712364));
#51243=CARTESIAN_POINT('Ctrl Pts',(-6.9663780349945,-7.32498745762988,-13.9029032827295));
#51244=CARTESIAN_POINT('Ctrl Pts',(-6.95898554961068,-7.36318022038742,
-13.8988369647304));
#51245=CARTESIAN_POINT('Ctrl Pts',(-6.95056864272973,-7.40027848783653,
-13.8952297705182));
#51246=CARTESIAN_POINT('Ctrl Pts',(-6.94129566725109,-7.43623003030209,
-13.8920150836015));
#51247=CARTESIAN_POINT('Ctrl Pts',(-6.93784226353682,-7.44961895714337,
-13.8908178830089));
#51248=CARTESIAN_POINT('Ctrl Pts',(-6.93426982004788,-7.46284913304693,
-13.8896747998003));
#51249=CARTESIAN_POINT('Ctrl Pts',(-6.93058586859352,-7.47591881634163,
-13.8885813742623));
#51250=CARTESIAN_POINT('Ctrl Pts',(-6.91970525354453,-7.51452035452792,
-13.8853519228128));
#51251=CARTESIAN_POINT('Ctrl Pts',(-6.90786941662626,-7.55171553530684,
-13.8826092506353));
#51252=CARTESIAN_POINT('Ctrl Pts',(-6.89530214052475,-7.58746826104597,
-13.8803240339689));
#51253=CARTESIAN_POINT('Ctrl Pts',(-6.88388401452961,-7.6199517621533,-13.8782477772198));
#51254=CARTESIAN_POINT('Ctrl Pts',(-6.87186213916831,-7.65124527796107,
-13.8765482707761));
#51255=CARTESIAN_POINT('Ctrl Pts',(-6.859384598782,-7.68134460616923,-13.8751816781369));
#51256=CARTESIAN_POINT('Ctrl Pts',(-6.84627917222293,-7.7129585719907,-13.8737463167664));
#51257=CARTESIAN_POINT('Ctrl Pts',(-6.83267337671324,-7.74325449253608,
-13.8726829358396));
#51258=CARTESIAN_POINT('Ctrl Pts',(-6.81872866685287,-7.77224538414329,
-13.8719470606914));
#51259=CARTESIAN_POINT('Ctrl Pts',(-6.81175631192269,-7.78674082994689,
-13.8715791231173));
#51260=CARTESIAN_POINT('Ctrl Pts',(-6.80469903051961,-7.80091023832986,
-13.8712930411406));
#51261=CARTESIAN_POINT('Ctrl Pts',(-6.79757576494785,-7.81475652551018,
-13.871083086116));
#51262=CARTESIAN_POINT('Ctrl Pts',(-6.79401413216197,-7.82167966910034,
-13.8709781086038));
#51263=CARTESIAN_POINT('Ctrl Pts',(-6.79043600023178,-7.82852203040168,
-13.8708921649966));
#51264=CARTESIAN_POINT('Ctrl Pts',(-6.78684364094681,-7.83528407274267,
-13.8708245202887));
#51265=CARTESIAN_POINT('Ctrl Pts',(-6.7844031629649,-7.83987788258651,-13.8707785656925));
#51266=CARTESIAN_POINT('Ctrl Pts',(-6.78226604253571,-7.84386068729018,
-13.8707466372644));
#51267=CARTESIAN_POINT('Ctrl Pts',(-6.77980273810643,-7.84840303797618,
-13.8707160597476));
#51268=CARTESIAN_POINT('Ctrl Pts',(-6.77864008294754,-7.8505469822633,-13.8707016274642));
#51269=CARTESIAN_POINT('Ctrl Pts',(-6.77740428166745,-7.85281534857401,
-13.870687857321));
#51270=CARTESIAN_POINT('Ctrl Pts',(-6.77602613363967,-7.85532970183153,
-13.8706757544928));
#51271=CARTESIAN_POINT('Ctrl Pts',(-6.75125394113064,-7.90052516826551,
-13.8704582063179));
#51272=CARTESIAN_POINT('Ctrl Pts',(-6.72490412475708,-7.94384710910138,
-13.8710746067399));
#51273=CARTESIAN_POINT('Ctrl Pts',(-6.69725567797657,-7.98518156062326,
-13.8725531445371));
#51274=CARTESIAN_POINT('Ctrl Pts',(-6.66792060847387,-8.02903751455356,
-13.8741218767479));
#51275=CARTESIAN_POINT('Ctrl Pts',(-6.63712435813431,-8.07065602654574,
-13.8766608669807));
#51276=CARTESIAN_POINT('Ctrl Pts',(-6.60519224452536,-8.10994500446146,
-13.8801627385162));
#51277=CARTESIAN_POINT('Ctrl Pts',(-6.57239250576793,-8.15030150035343,
-13.8837597591497));
#51278=CARTESIAN_POINT('Ctrl Pts',(-6.53839480749624,-8.18820041717145,
-13.8883721273538));
#51279=CARTESIAN_POINT('Ctrl Pts',(-6.50353422891246,-8.22358513606488,
-13.8939568293774));
#51280=CARTESIAN_POINT('Ctrl Pts',(-6.46687694718795,-8.26079357212403,
-13.8998293651684));
#51281=CARTESIAN_POINT('Ctrl Pts',(-6.42926589159602,-8.29522210847277,
-13.906776585492));
#51282=CARTESIAN_POINT('Ctrl Pts',(-6.39106504384856,-8.32684898034795,
-13.9147183184548));
#51283=CARTESIAN_POINT('Ctrl Pts',(-6.35949181868436,-8.35298877581938,
-13.9212822074209));
#51284=CARTESIAN_POINT('Ctrl Pts',(-6.32751518914135,-8.37721562678356,
-13.9285247897248));
#51285=CARTESIAN_POINT('Ctrl Pts',(-6.29532684358237,-8.39953711567565,
-13.9363895287864));
#51286=CARTESIAN_POINT('Ctrl Pts',(-6.28485853259168,-8.40679652225402,
-13.9389473034383));
#51287=CARTESIAN_POINT('Ctrl Pts',(-6.27436773210387,-8.41385453303562,
-13.9415708157395));
#51288=CARTESIAN_POINT('Ctrl Pts',(-6.2638607595696,-8.42071177891138,-13.9442579405079));
#51289=CARTESIAN_POINT('Ctrl Pts',(-6.22267017867758,-7.49367493044375,
-13.1134074242241));
#51290=CARTESIAN_POINT('Ctrl Pts',(-6.22400572031555,-7.81349993090739,
-13.3673840000309));
#51291=CARTESIAN_POINT('Ctrl Pts',(-6.22726530830951,-8.61699726505343,
-14.0755228901556));
#51292=CARTESIAN_POINT('Ctrl Pts',(-6.23205383335972,-9.75631816520924,
-15.3875907763663));
#51293=CARTESIAN_POINT('Ctrl Pts',(-6.2357076456412,-10.7961446862802,-17.0892605390954));
#51294=CARTESIAN_POINT('Ctrl Pts',(-6.23759681166444,-11.5416365780555,
-18.9411597533656));
#51295=CARTESIAN_POINT('Ctrl Pts',(-6.23804400737905,-11.9701361487446,
-20.8893389967195));
#51296=CARTESIAN_POINT('Ctrl Pts',(-6.23649715758559,-12.0627637107556,
-22.726022856573));
#51297=CARTESIAN_POINT('Ctrl Pts',(-6.23490937071487,-11.9504775464553,
-23.8924618957293));
#51298=CARTESIAN_POINT('Ctrl Pts',(-6.23413407861479,-11.8700328552509,
-24.3933786980252));
#51299=CARTESIAN_POINT('Ctrl Pts',(-6.71589117748943,-7.42368469516801,
-13.2016814708845));
#51300=CARTESIAN_POINT('Ctrl Pts',(-6.71707990387349,-7.74006673352331,
-13.4537919778345));
#51301=CARTESIAN_POINT('Ctrl Pts',(-6.71993443015081,-8.53486089184209,
-14.1564716232462));
#51302=CARTESIAN_POINT('Ctrl Pts',(-6.72416527772874,-9.6612568988981,-15.4574021509406));
#51303=CARTESIAN_POINT('Ctrl Pts',(-6.72736893457949,-10.6891558328984,
-17.1431718671125));
#51304=CARTESIAN_POINT('Ctrl Pts',(-6.72902498583597,-11.4262572324651,
-18.976798290278));
#51305=CARTESIAN_POINT('Ctrl Pts',(-6.72941998203574,-11.8502291076773,
-20.9054815431427));
#51306=CARTESIAN_POINT('Ctrl Pts',(-6.72805245035654,-11.9427115601072,
-22.7235295090814));
#51307=CARTESIAN_POINT('Ctrl Pts',(-6.72668417717144,-11.8323436962498,
-23.8785261271082));
#51308=CARTESIAN_POINT('Ctrl Pts',(-6.72599103236445,-11.7530854106976,
-24.3745537247135));
#51309=CARTESIAN_POINT('Ctrl Pts',(-7.02184860947709,-7.17355734656295,
-13.5171494444303));
#51310=CARTESIAN_POINT('Ctrl Pts',(-7.02249156717522,-7.47887520271202,
-13.7610265541486));
#51311=CARTESIAN_POINT('Ctrl Pts',(-7.02397822748931,-8.24599816030359,
-14.4407082883408));
#51312=CARTESIAN_POINT('Ctrl Pts',(-7.02622826305931,-9.33267501545243,
-15.6982405691599));
#51313=CARTESIAN_POINT('Ctrl Pts',(-7.02790160720142,-10.3242144174604,
-17.326828018892));
#51314=CARTESIAN_POINT('Ctrl Pts',(-7.02876614498039,-11.0353387540962,
-19.0974438565416));
#51315=CARTESIAN_POINT('Ctrl Pts',(-7.02897606416112,-11.4446315866814,
-20.9601358899923));
#51316=CARTESIAN_POINT('Ctrl Pts',(-7.02824776303995,-11.5344312606834,
-22.715199240432));
#51317=CARTESIAN_POINT('Ctrl Pts',(-7.02756281917417,-11.4283599706227,
-23.8309174048354));
#51318=CARTESIAN_POINT('Ctrl Pts',(-7.02718413556234,-11.3520773735171,
-24.3100040140441));
#51319=CARTESIAN_POINT('Ctrl Pts',(-6.99898915817327,-6.85988136608093,
-13.9127665215165));
#51320=CARTESIAN_POINT('Ctrl Pts',(-6.99894180086011,-7.15167011659703,
-14.1458817646929));
#51321=CARTESIAN_POINT('Ctrl Pts',(-6.99873531791728,-7.88504935784626,
-14.7957491612715));
#51322=CARTESIAN_POINT('Ctrl Pts',(-6.99850468722686,-8.92372185170608,
-15.9978535584084));
#51323=CARTESIAN_POINT('Ctrl Pts',(-6.99828080837736,-9.87141300061994,
-17.5546303803054));
#51324=CARTESIAN_POINT('Ctrl Pts',(-6.9981643412379,-10.5510791282796,-19.2468664456477));
#51325=CARTESIAN_POINT('Ctrl Pts',(-6.99814257227861,-10.9423826236159,
-21.0278289503835));
#51326=CARTESIAN_POINT('Ctrl Pts',(-6.99821545942191,-11.0282139102074,
-22.7049145045068));
#51327=CARTESIAN_POINT('Ctrl Pts',(-6.99835922294982,-10.9268166228346,
-23.7718253449984));
#51328=CARTESIAN_POINT('Ctrl Pts',(-6.99838072371096,-10.8539128981486,
-24.2298152697073));
#51329=CARTESIAN_POINT('',(-7.00000355772223,-10.9277699390017,-24.1259406808672));
#51330=CARTESIAN_POINT('Ctrl Pts',(-7.00001601661457,-6.97711952672703,
-13.9487142980922));
#51331=CARTESIAN_POINT('Ctrl Pts',(-7.00002088999339,-7.14852816441581,
-14.0875641829895));
#51332=CARTESIAN_POINT('Ctrl Pts',(-7.0000159830912,-7.3142134747507,-14.2303294324432));
#51333=CARTESIAN_POINT('Ctrl Pts',(-7.00000988157515,-7.47407280375667,
-14.3764170928589));
#51334=CARTESIAN_POINT('Ctrl Pts',(-7.00000652467619,-7.56202334106749,
-14.4567908083494));
#51335=CARTESIAN_POINT('Ctrl Pts',(-7.00000279094438,-7.64821100818324,
-14.5381709027261));
#51336=CARTESIAN_POINT('Ctrl Pts',(-6.99999999965531,-7.73262304327109,
-14.6204637380433));
#51337=CARTESIAN_POINT('Ctrl Pts',(-6.99999455422802,-7.89729950162332,
-14.7810059243999));
#51338=CARTESIAN_POINT('Ctrl Pts',(-6.99999266081079,-8.05521661797847,
-14.9450193659817));
#51339=CARTESIAN_POINT('Ctrl Pts',(-6.99999257345288,-8.20640348779146,
-15.1118936930631));
#51340=CARTESIAN_POINT('Ctrl Pts',(-6.99999248483003,-8.35977953074498,
-15.281184346345));
#51341=CARTESIAN_POINT('Ctrl Pts',(-6.99999425319322,-8.50622906277903,
-15.4534193548216));
#51342=CARTESIAN_POINT('Ctrl Pts',(-6.99999619757759,-8.6458124013378,-15.6280063527474));
#51343=CARTESIAN_POINT('Ctrl Pts',(-6.99999754424624,-8.74248696251648,
-15.7489242329634));
#51344=CARTESIAN_POINT('Ctrl Pts',(-6.99999897835358,-8.83586853326925,
-15.8709712717052));
#51345=CARTESIAN_POINT('Ctrl Pts',(-6.99999998662288,-8.92598514844779,
-15.9939628974921));
#51346=CARTESIAN_POINT('Ctrl Pts',(-7.00000143709196,-9.05562448575202,
-16.1708953402985));
#51347=CARTESIAN_POINT('Ctrl Pts',(-7.00000201442316,-9.17850663798034,
-16.3497801253261));
#51348=CARTESIAN_POINT('Ctrl Pts',(-7.00000210876032,-9.29479658368068,
-16.5300359468127));
#51349=CARTESIAN_POINT('Ctrl Pts',(-7.00000220461162,-9.4129530146951,-16.7131849233487));
#51350=CARTESIAN_POINT('Ctrl Pts',(-7.00000180217023,-9.52430397773151,
-16.8977493304543));
#51351=CARTESIAN_POINT('Ctrl Pts',(-7.00000129011944,-9.6290403473303,-17.0831707166954));
#51352=CARTESIAN_POINT('Ctrl Pts',(-7.00000086167034,-9.71667658275699,
-17.2383186592871));
#51353=CARTESIAN_POINT('Ctrl Pts',(-7.00000035619251,-9.79968215285438,
-17.3940675430476));
#51354=CARTESIAN_POINT('Ctrl Pts',(-6.9999999881668,-9.87817778643373,-17.5501167577466));
#51355=CARTESIAN_POINT('Ctrl Pts',(-6.99999970373346,-9.93884413335317,
-17.6707213743825));
#51356=CARTESIAN_POINT('Ctrl Pts',(-6.99999950019769,-9.99681685740602,
-17.7915058719012));
#51357=CARTESIAN_POINT('Ctrl Pts',(-6.99999936067301,-10.0521635852022,
-17.9123403180643));
#51358=CARTESIAN_POINT('Ctrl Pts',(-6.99999924478733,-10.0981331762724,
-18.0127023502653));
#51359=CARTESIAN_POINT('Ctrl Pts',(-6.99999917321297,-10.1422912472031,
-18.1130989925497));
#51360=CARTESIAN_POINT('Ctrl Pts',(-6.99999913936348,-10.1846774398662,
-18.2134600445155));
#51361=CARTESIAN_POINT('Ctrl Pts',(-6.99999912243874,-10.2058705361977,
-18.2636405704984));
#51362=CARTESIAN_POINT('Ctrl Pts',(-6.99999911498655,-10.2266206629623,
-18.3138121989017));
#51363=CARTESIAN_POINT('Ctrl Pts',(-6.99999911639989,-10.2469328611172,
-18.3639665749347));
#51364=CARTESIAN_POINT('Ctrl Pts',(-6.99999911710655,-10.2570889601946,
-18.3890437629512));
#51365=CARTESIAN_POINT('Ctrl Pts',(-6.9999991200318,-10.2671355771195,-18.4141166378752));
#51366=CARTESIAN_POINT('Ctrl Pts',(-6.99999912511194,-10.2770733440966,
-18.4391841663968));
#51367=CARTESIAN_POINT('Ctrl Pts',(-6.99999912765202,-10.2820422275851,
-18.4517179306576));
#51368=CARTESIAN_POINT('Ctrl Pts',(-6.99999913073094,-10.2869838985867,
-18.4642503583179));
#51369=CARTESIAN_POINT('Ctrl Pts',(-6.99999913434145,-10.2918984364191,
-18.4767813216805));
#51370=CARTESIAN_POINT('Ctrl Pts',(-6.99999913749775,-10.2961947269233,
-18.4877358937565));
#51371=CARTESIAN_POINT('Ctrl Pts',(-6.99999914056827,-10.2999248799151,
-18.4972872811118));
#51372=CARTESIAN_POINT('Ctrl Pts',(-6.99999914483355,-10.3045195397806,
-18.5091123716368));
#51373=CARTESIAN_POINT('Ctrl Pts',(-6.99999914544734,-10.3051807232324,
-18.5108140327825));
#51374=CARTESIAN_POINT('Ctrl Pts',(-6.99999914608781,-10.3058597282213,
-18.5125628090823));
#51375=CARTESIAN_POINT('Ctrl Pts',(-6.9999991467609,-10.3065607298115,-18.5143696916144));
#51376=CARTESIAN_POINT('Ctrl Pts',(-6.99999923697261,-10.4005127250538,
-18.756537785691));
#51377=CARTESIAN_POINT('Ctrl Pts',(-6.99999952144542,-10.4851669254592,
-19.0001638726786));
#51378=CARTESIAN_POINT('Ctrl Pts',(-6.99999999018441,-10.5606727034661,
-19.2445345426536));
#51379=CARTESIAN_POINT('Ctrl Pts',(-7.00000044364527,-10.6337174393521,
-19.4809401730273));
#51380=CARTESIAN_POINT('Ctrl Pts',(-7.00000106797182,-10.6982012753055,
-19.7180425300442));
#51381=CARTESIAN_POINT('Ctrl Pts',(-7.00000142593368,-10.7543687395633,
-19.9551823301155));
#51382=CARTESIAN_POINT('Ctrl Pts',(-7.000001787659,-10.8111267256216,-20.194815321282));
#51383=CARTESIAN_POINT('Ctrl Pts',(-7.00000187627587,-10.8593925727004,
-20.4344865835451));
#51384=CARTESIAN_POINT('Ctrl Pts',(-7.00000131559613,-10.899424908229,-20.6735687764459));
#51385=CARTESIAN_POINT('Ctrl Pts',(-7.00000103873707,-10.919192546995,-20.7916256013166));
#51386=CARTESIAN_POINT('Ctrl Pts',(-7.00000060481242,-10.9369527001568,
-20.9095395989653));
#51387=CARTESIAN_POINT('Ctrl Pts',(-6.99999997635826,-10.9527370390027,
-21.0272398759844));
#51388=CARTESIAN_POINT('Ctrl Pts',(-6.99999887928051,-10.9802913904854,
-21.2327064992163));
#51389=CARTESIAN_POINT('Ctrl Pts',(-6.99999719586421,-11.0018248530504,
-21.4375204977235));
#51390=CARTESIAN_POINT('Ctrl Pts',(-6.99999590263484,-11.017557252248,-21.6413538404685));
#51391=CARTESIAN_POINT('Ctrl Pts',(-6.99999568171157,-11.0202448288404,
-21.6761748308222));
#51392=CARTESIAN_POINT('Ctrl Pts',(-6.99999546001773,-11.0229065623117,
-21.7128795454964));
#51393=CARTESIAN_POINT('Ctrl Pts',(-6.99999525388096,-11.0254108578281,
-21.7501378180189));
#51394=CARTESIAN_POINT('Ctrl Pts',(-6.99999512029513,-11.0270337530759,
-21.7742828412477));
#51395=CARTESIAN_POINT('Ctrl Pts',(-6.99999499323631,-11.0285915172457,
-21.7986602431002));
#51396=CARTESIAN_POINT('Ctrl Pts',(-6.99999487630838,-11.0300601234091,
-21.8229071175643));
#51397=CARTESIAN_POINT('Ctrl Pts',(-6.99999457894853,-11.0337949410457,
-21.8845694315598));
#51398=CARTESIAN_POINT('Ctrl Pts',(-6.99999434327763,-11.0369990630641,
-21.9460663067667));
#51399=CARTESIAN_POINT('Ctrl Pts',(-6.99999419420638,-11.0396820529461,
-22.0073884932679));
#51400=CARTESIAN_POINT('Ctrl Pts',(-6.99999365474403,-11.0493913156715,
-22.2293025689177));
#51401=CARTESIAN_POINT('Ctrl Pts',(-6.99999426201427,-11.0522757589082,
-22.4489298924521));
#51402=CARTESIAN_POINT('Ctrl Pts',(-6.99999708881797,-11.0487792584282,
-22.665896946056));
#51403=CARTESIAN_POINT('Ctrl Pts',(-6.99999738657107,-11.0484109647727,
-22.6887505363071));
#51404=CARTESIAN_POINT('Ctrl Pts',(-6.99999770879678,-11.0479718686333,
-22.7115746583192));
#51405=CARTESIAN_POINT('Ctrl Pts',(-6.99999805664087,-11.0474624838517,
-22.734368908558));
#51406=CARTESIAN_POINT('Ctrl Pts',(-6.99999863108936,-11.0466212583313,
-22.7720125636346));
#51407=CARTESIAN_POINT('Ctrl Pts',(-6.99999927541492,-11.0455883348251,
-22.809574746992));
#51408=CARTESIAN_POINT('Ctrl Pts',(-6.99999999465529,-11.0443660217701,
-22.8470536786943));
#51409=CARTESIAN_POINT('Ctrl Pts',(-7.00000393353041,-11.0376721003838,
-23.0523047160112));
#51410=CARTESIAN_POINT('Ctrl Pts',(-7.00001006486665,-11.0252993377964,
-23.2550548353964));
#51411=CARTESIAN_POINT('Ctrl Pts',(-7.00001375755606,-11.0076805209828,
-23.4549602553255));
#51412=CARTESIAN_POINT('Ctrl Pts',(-7.00001750473177,-10.9898017353607,
-23.6578153156528));
#51413=CARTESIAN_POINT('Ctrl Pts',(-7.00001874206597,-10.9665209565483,
-23.8577411890485));
#51414=CARTESIAN_POINT('Ctrl Pts',(-7.00001328550256,-10.9382750849474,
-24.054429846901));
#51415=CARTESIAN_POINT('Ctrl Pts',(-7.00001262289278,-10.9348450889235,
-24.0783144458225));
#51416=CARTESIAN_POINT('Ctrl Pts',(-7.00001186234173,-10.9313418586631,
-24.102151368649));
#51417=CARTESIAN_POINT('Ctrl Pts',(-7.00001099698758,-10.9277661612435,
-24.1259401133012));
#51418=CARTESIAN_POINT('',(-6.271594443024,-11.8794941632625,-24.2690120587724));
#51419=CARTESIAN_POINT('Origin',(-5.99998362344205,-10.9277594519405,-24.1259473036685));
#51420=CARTESIAN_POINT('Ctrl Pts',(-6.26386063113558,-8.42071912122325,
-13.9442659510471));
#51421=CARTESIAN_POINT('Ctrl Pts',(-6.26455155145855,-8.59292897217472,
-14.1129997319506));
#51422=CARTESIAN_POINT('Ctrl Pts',(-6.2652098889244,-8.75835742010234,-14.2852520702197));
#51423=CARTESIAN_POINT('Ctrl Pts',(-6.2658356434991,-8.91700591634091,-14.4604178426464));
#51424=CARTESIAN_POINT('Ctrl Pts',(-6.2664706971121,-9.07801201171459,-14.6381866695197));
#51425=CARTESIAN_POINT('Ctrl Pts',(-6.2670721922411,-9.23203520058945,-14.8189561782818));
#51426=CARTESIAN_POINT('Ctrl Pts',(-6.26764012885049,-9.37910898118983,
-15.0021375673763));
#51427=CARTESIAN_POINT('Ctrl Pts',(-6.26812470388292,-9.50459531333848,
-15.1584316433261));
#51428=CARTESIAN_POINT('Ctrl Pts',(-6.26858484882168,-9.62502315723059,
-15.3164822997201));
#51429=CARTESIAN_POINT('Ctrl Pts',(-6.26902056364464,-9.74043079708379,
-15.4759481443977));
#51430=CARTESIAN_POINT('Ctrl Pts',(-6.26953467308444,-9.87660279295714,
-15.6641053787974));
#51431=CARTESIAN_POINT('Ctrl Pts',(-6.27001477053663,-10.0057860138603,
-15.8542312106714));
#51432=CARTESIAN_POINT('Ctrl Pts',(-6.27046085596489,-10.1281597369355,
-16.0457357401779));
#51433=CARTESIAN_POINT('Ctrl Pts',(-6.27062083627522,-10.1720468154061,
-16.1144153071855));
#51434=CARTESIAN_POINT('Ctrl Pts',(-6.27077644207497,-10.2150582315774,
-16.1832726641688));
#51435=CARTESIAN_POINT('Ctrl Pts',(-6.27092767336246,-10.2572027535103,
-16.2522821457338));
#51436=CARTESIAN_POINT('Ctrl Pts',(-6.27136815356596,-10.3799539904141,
-16.4532809667355));
#51437=CARTESIAN_POINT('Ctrl Pts',(-6.27177152312615,-10.4953497486126,
-16.6555662199662));
#51438=CARTESIAN_POINT('Ctrl Pts',(-6.27213778204303,-10.6036186334423,
-16.8585417460444));
#51439=CARTESIAN_POINT('Ctrl Pts',(-6.2725040409599,-10.711887518272,-17.0615172721226));
#51440=CARTESIAN_POINT('Ctrl Pts',(-6.27283318923347,-10.8130296334295,
-17.265183259542));
#51441=CARTESIAN_POINT('Ctrl Pts',(-6.27312522686372,-10.9072901272152,
-17.4689978455677));
#51442=CARTESIAN_POINT('Ctrl Pts',(-6.27334042001379,-10.9767476576266,
-17.6191822678916));
#51443=CARTESIAN_POINT('Ctrl Pts',(-6.27353526248212,-11.0423478968138,
-17.7691758821825));
#51444=CARTESIAN_POINT('Ctrl Pts',(-6.2737099759448,-11.1043414808216,-17.9190756114325));
#51445=CARTESIAN_POINT('Ctrl Pts',(-6.27388468940749,-11.1663350648294,
-18.0689753406825));
#51446=CARTESIAN_POINT('Ctrl Pts',(-6.27403927386453,-11.2247220378057,
-18.2187816105632));
#51447=CARTESIAN_POINT('Ctrl Pts',(-6.27417395099203,-11.279707421021,-18.368626212332));
#51448=CARTESIAN_POINT('Ctrl Pts',(-6.27427013615269,-11.3189774738988,
-18.4756438430332));
#51449=CARTESIAN_POINT('Ctrl Pts',(-6.27435616721267,-11.3565115886943,
-18.5826817408085));
#51450=CARTESIAN_POINT('Ctrl Pts',(-6.2744321249255,-11.3923814106472,-18.6897928669546));
#51451=CARTESIAN_POINT('Ctrl Pts',(-6.27457884404932,-11.4616671836455,
-18.8966875981714));
#51452=CARTESIAN_POINT('Ctrl Pts',(-6.27469165391534,-11.5261459268611,
-19.1080568290295));
#51453=CARTESIAN_POINT('Ctrl Pts',(-6.27477055452358,-11.5853121282286,
-19.3236963875817));
#51454=CARTESIAN_POINT('Ctrl Pts',(-6.27484862770157,-11.6438578539663,
-19.5370745352639));
#51455=CARTESIAN_POINT('Ctrl Pts',(-6.27489349910493,-11.6972018816246,
-19.7546340252876));
#51456=CARTESIAN_POINT('Ctrl Pts',(-6.27490516873366,-11.7448338103361,
-19.9761311914299));
#51457=CARTESIAN_POINT('Ctrl Pts',(-6.27491664477165,-11.791675559668,-20.1939538791694));
#51458=CARTESIAN_POINT('Ctrl Pts',(-6.27489601148479,-11.8329931384633,
-20.4155847332407));
#51459=CARTESIAN_POINT('Ctrl Pts',(-6.27484326887307,-11.8682812257124,
-20.6407463058143));
#51460=CARTESIAN_POINT('Ctrl Pts',(-6.27479056635055,-11.9035424907943,
-20.8657367350417));
#51461=CARTESIAN_POINT('Ctrl Pts',(-6.27470580329666,-11.9327834609942,
-21.0942526911029));
#51462=CARTESIAN_POINT('Ctrl Pts',(-6.27458897971139,-11.9554797335007,
-21.3259694684535));
#51463=CARTESIAN_POINT('Ctrl Pts',(-6.27454781352703,-11.963477424515,-21.4076216070384));
#51464=CARTESIAN_POINT('Ctrl Pts',(-6.27450266640086,-11.9706622677186,
-21.4896707456406));
#51465=CARTESIAN_POINT('Ctrl Pts',(-6.27445353832076,-11.9770107062944,
-21.5721011963521));
#51466=CARTESIAN_POINT('Ctrl Pts',(-6.27431624074768,-11.9947526006979,
-21.8024684488204));
#51467=CARTESIAN_POINT('Ctrl Pts',(-6.27414785084326,-12.0059621178477,
-22.0358175491883));
#51468=CARTESIAN_POINT('Ctrl Pts',(-6.27394836834336,-12.0102364733222,
-22.271764620327));
#51469=CARTESIAN_POINT('Ctrl Pts',(-6.27375072689948,-12.014471380084,-22.5055340980757));
#51470=CARTESIAN_POINT('Ctrl Pts',(-6.27352256412883,-12.0118985210674,
-22.7418539062483));
#51471=CARTESIAN_POINT('Ctrl Pts',(-6.27326387977453,-12.0021219113766,
-22.9803002635899));
#51472=CARTESIAN_POINT('Ctrl Pts',(-6.27300884338782,-11.9924831714667,
-23.215384049643));
#51473=CARTESIAN_POINT('Ctrl Pts',(-6.27272414017866,-11.9758423964283,
-23.4525348737001));
#51474=CARTESIAN_POINT('Ctrl Pts',(-6.27240976990089,-11.951816352854,-23.6912964437234));
#51475=CARTESIAN_POINT('Ctrl Pts',(-6.27215746684018,-11.932533854605,-23.8829184867648));
#51476=CARTESIAN_POINT('Ctrl Pts',(-6.27188605483419,-11.908494333709,-24.0755771130839));
#51477=CARTESIAN_POINT('Ctrl Pts',(-6.27159553375568,-11.8794980525036,
-24.2690121689631));
#51478=CARTESIAN_POINT('Origin',(-5.999994993365,-10.9277770074801,-24.1259380195517));
#51479=CARTESIAN_POINT('',(-5.98852246669736,-11.3308498388635,-25.0410395151954));
#51480=CARTESIAN_POINT('Origin',(-5.999994993365,-10.9277770074801,-24.1259380195517));
#51481=CARTESIAN_POINT('Origin',(-6.,-10.9277790633915,-24.1259427050578));
#51482=CARTESIAN_POINT('Ctrl Pts',(-5.98841833134383,-11.3313022800093,
-25.0408390134412));
#51483=CARTESIAN_POINT('Ctrl Pts',(-5.98810627250749,-11.2108442555167,
-25.0938945834082));
#51484=CARTESIAN_POINT('Ctrl Pts',(-5.9872640505444,-10.7897532280987,-25.2768814426322));
#51485=CARTESIAN_POINT('Ctrl Pts',(-5.98726405054346,-10.2439465927857,
-25.5029619533741));
#51486=CARTESIAN_POINT('Ctrl Pts',(-5.98810627252732,-9.8167990201698,-25.6713270262117));
#51487=CARTESIAN_POINT('Ctrl Pts',(-5.98841833138136,-9.69410637653267,
-25.7189877605115));
#51488=CARTESIAN_POINT('Ctrl Pts',(-6.58019637611207,-11.334065277118,-25.0471116847692));
#51489=CARTESIAN_POINT('Ctrl Pts',(-6.57988216872294,-11.2136609913595,
-25.1003453887717));
#51490=CARTESIAN_POINT('Ctrl Pts',(-6.57903377743291,-10.7926927015607,
-25.2838224191463));
#51491=CARTESIAN_POINT('Ctrl Pts',(-6.57903377743206,-10.2467760827226,
-25.5099484865553));
#51492=CARTESIAN_POINT('Ctrl Pts',(-6.57988216874175,-9.81936869536461,
-25.6778801674394));
#51493=CARTESIAN_POINT('Ctrl Pts',(-6.58019637614898,-9.69658809095763,
-25.7253769429152));
#51494=CARTESIAN_POINT('Ctrl Pts',(-7.00079677429184,-11.1662377629886,
-24.6661026395446));
#51495=CARTESIAN_POINT('Ctrl Pts',(-7.0006124896366,-11.0471442760462,-24.7189023979519));
#51496=CARTESIAN_POINT('Ctrl Pts',(-7.00011448915241,-10.6307100868985,
-24.9007955995176));
#51497=CARTESIAN_POINT('Ctrl Pts',(-7.00011448915238,-10.0904742265319,
-25.1245686197181));
#51498=CARTESIAN_POINT('Ctrl Pts',(-7.00061248964771,-9.66739286861664,
-25.2904141433636));
#51499=CARTESIAN_POINT('Ctrl Pts',(-7.00079677431298,-9.54584598485692,
-25.3372908899495));
#51500=CARTESIAN_POINT('Ctrl Pts',(-6.99999917318423,-10.9276780868235,
-24.1245144806664));
#51501=CARTESIAN_POINT('Ctrl Pts',(-6.99999957776486,-10.8103725307965,
-24.1765264252412));
#51502=CARTESIAN_POINT('Ctrl Pts',(-7.00000004362129,-10.4001860019773,
-24.3557042159038));
#51503=CARTESIAN_POINT('Ctrl Pts',(-7.0000000436221,-9.86804155661048,-24.576125662278));
#51504=CARTESIAN_POINT('Ctrl Pts',(-6.99999957776511,-9.45129804718398,
-24.7394735083839));
#51505=CARTESIAN_POINT('Ctrl Pts',(-6.99999917318347,-9.33157249006586,
-24.7856430653755));
#51506=CARTESIAN_POINT('Origin',(-5.98852353414945,4.75229019615101,11.4730434493167));
#51507=CARTESIAN_POINT('Origin',(-7.00021006963517,4.74293535319878,11.4504589429759));
#51508=CARTESIAN_POINT('Ctrl Pts',(-6.05505067658424,-11.6467908023141,
-24.9010149462025));
#51509=CARTESIAN_POINT('Ctrl Pts',(-4.03670045105583,-12.172766115143,-24.6398353500469));
#51510=CARTESIAN_POINT('Ctrl Pts',(7.59697248924746E-7,-12.7121382468122,
-24.4085103636044));
#51511=CARTESIAN_POINT('Ctrl Pts',(4.03670197045045,-12.1727659121264,-24.6398354371181));
#51512=CARTESIAN_POINT('Ctrl Pts',(6.05505295567616,-11.6467902083882,-24.9010152411215));
#51513=CARTESIAN_POINT('Ctrl Pts',(-6.05505067658424,-10.8984856531672,
-25.2386153210465));
#51514=CARTESIAN_POINT('Ctrl Pts',(-4.03670045105583,-11.0706898476697,
-25.1429607074797));
#51515=CARTESIAN_POINT('Ctrl Pts',(7.59697248924746E-7,-11.3017449371971,
-25.1800056309795));
#51516=CARTESIAN_POINT('Ctrl Pts',(4.03670197045045,-11.0706897606967,-25.1429606935417));
#51517=CARTESIAN_POINT('Ctrl Pts',(6.05505295567616,-10.8984854587184,-25.2386154290685));
#51518=CARTESIAN_POINT('Ctrl Pts',(-6.05505067658424,-10.1393891149069,
-25.5530359782357));
#51519=CARTESIAN_POINT('Ctrl Pts',(-4.03670045105583,-9.94969139606472,
-25.6072809456058));
#51520=CARTESIAN_POINT('Ctrl Pts',(7.59697248924746E-7,-9.81219809096102,
-25.7969458341962));
#51521=CARTESIAN_POINT('Ctrl Pts',(4.03670197045045,-9.94969144781643,-25.6072808742153));
#51522=CARTESIAN_POINT('Ctrl Pts',(6.05505295567616,-10.1393893291101,-25.5530359169843));
#51523=CARTESIAN_POINT('Ctrl Pts',(-6.05505067658424,-9.37153325114741,
-25.8434352094466));
#51524=CARTESIAN_POINT('Ctrl Pts',(-4.03670045105583,-8.81463489221611,
-26.0307812750284));
#51525=CARTESIAN_POINT('Ctrl Pts',(7.59697248924746E-7,-8.26934125243994,
-26.2486262267072));
#51526=CARTESIAN_POINT('Ctrl Pts',(4.03670197045045,-8.81463509746334,-26.0307811930261));
#51527=CARTESIAN_POINT('Ctrl Pts',(6.05505295567616,-9.37153387998869,-25.8434349978963));
#51528=CARTESIAN_POINT('Ctrl Pts',(-5.98852262888498,-11.3308502499308,
-25.0410393032242));
#51529=CARTESIAN_POINT('Ctrl Pts',(-5.93914474648228,-11.3464662790723,
-25.0335418651297));
#51530=CARTESIAN_POINT('Ctrl Pts',(-5.88279573443552,-11.3641427248077,
-25.025075083296));
#51531=CARTESIAN_POINT('Ctrl Pts',(-5.81940484978196,-11.3837118309506,
-25.0157333886925));
#51532=CARTESIAN_POINT('Ctrl Pts',(-5.75829929351482,-11.4025754439613,
-25.0067284749995));
#51533=CARTESIAN_POINT('Ctrl Pts',(-5.6906501886918,-11.4231976271372,-24.9969107663179));
#51534=CARTESIAN_POINT('Ctrl Pts',(-5.61638362618853,-11.4453877159357,
-24.9863837755093));
#51535=CARTESIAN_POINT('Ctrl Pts',(-5.54072805448531,-11.4679928264674,
-24.9756598981533));
#51536=CARTESIAN_POINT('Ctrl Pts',(-5.45820496082235,-11.4922253843586,
-24.9641999665009));
#51537=CARTESIAN_POINT('Ctrl Pts',(-5.36872850713851,-11.517838641789,-24.9521323326467));
#51538=CARTESIAN_POINT('Ctrl Pts',(-5.32399028029659,-11.5306452705042,
-24.9460985157196));
#51539=CARTESIAN_POINT('Ctrl Pts',(-5.27751361435665,-11.5437963423677,
-24.9399130655401));
#51540=CARTESIAN_POINT('Ctrl Pts',(-5.22928736241266,-11.557256449084,-24.9335937406877));
#51541=CARTESIAN_POINT('Ctrl Pts',(-5.20517423644066,-11.5639865024422,
-24.9304340782615));
#51542=CARTESIAN_POINT('Ctrl Pts',(-5.18062371398836,-11.5707938128604,
-24.9272409434839));
#51543=CARTESIAN_POINT('Ctrl Pts',(-5.15563438617454,-11.5776735871523,
-24.9240166902759));
#51544=CARTESIAN_POINT('Ctrl Pts',(-5.13189984807928,-11.5842079071722,
-24.9209543365718));
#51545=CARTESIAN_POINT('Ctrl Pts',(-5.10666091671902,-11.5911088858746,
-24.917722934394));
#51546=CARTESIAN_POINT('Ctrl Pts',(-5.08307503754699,-11.5975138749284,
-24.9147262027041));
#51547=CARTESIAN_POINT('Ctrl Pts',(-5.08182810707926,-11.5978524917736,
-24.9145677724831));
#51548=CARTESIAN_POINT('Ctrl Pts',(-5.0805858005279,-11.5981897325559,-24.9144099927714));
#51549=CARTESIAN_POINT('Ctrl Pts',(-5.07934858564891,-11.5985254731791,
-24.9142529214491));
#51550=CARTESIAN_POINT('Ctrl Pts',(-5.06433554014817,-11.6025995344745,
-24.9123469316755));
#51551=CARTESIAN_POINT('Ctrl Pts',(-5.04943318285377,-11.6066254144498,
-24.9104644360685));
#51552=CARTESIAN_POINT('Ctrl Pts',(-5.03464184082257,-11.610603820394,-24.9086050215558));
#51553=CARTESIAN_POINT('Ctrl Pts',(-4.91702209136905,-11.6422398348539,
-24.8938190833598));
#51554=CARTESIAN_POINT('Ctrl Pts',(-4.8064247394437,-11.6708766576423,-24.880490587538));
#51555=CARTESIAN_POINT('Ctrl Pts',(-4.70298901342678,-11.6968548640577,
-24.8684336938881));
#51556=CARTESIAN_POINT('Ctrl Pts',(-4.59988945574151,-11.7227486407442,
-24.8564159854017));
#51557=CARTESIAN_POINT('Ctrl Pts',(-4.50390473923413,-11.7460013235489,
-24.8456616465603));
#51558=CARTESIAN_POINT('Ctrl Pts',(-4.41514467568984,-11.7669144905269,
-24.836011384925));
#51559=CARTESIAN_POINT('Ctrl Pts',(-4.38360632213252,-11.7743453871241,
-24.8325824400682));
#51560=CARTESIAN_POINT('Ctrl Pts',(-4.35297986818637,-11.7814805642034,
-24.8292931152813));
#51561=CARTESIAN_POINT('Ctrl Pts',(-4.32326949058923,-11.7883323671655,
-24.8261370134803));
#51562=CARTESIAN_POINT('Ctrl Pts',(-4.28864225633674,-11.7963180948946,
-24.8224585992282));
#51563=CARTESIAN_POINT('Ctrl Pts',(-4.25525940838751,-11.8039189234467,
-24.8189611357159));
#51564=CARTESIAN_POINT('Ctrl Pts',(-4.22312693762557,-11.8111532657858,
-24.8156351724646));
#51565=CARTESIAN_POINT('Ctrl Pts',(-4.2070607022446,-11.8147704369554,-24.8139721908389));
#51566=CARTESIAN_POINT('Ctrl Pts',(-4.19130706116087,-11.8182959875239,
-24.8123520863462));
#51567=CARTESIAN_POINT('Ctrl Pts',(-4.17586669210795,-11.8217320788189,
-24.8107737565214));
#51568=CARTESIAN_POINT('Ctrl Pts',(-4.16814650758149,-11.8234501244665,
-24.8099845916091));
#51569=CARTESIAN_POINT('Ctrl Pts',(-4.16050464106272,-11.8251458053497,
-24.8092058704814));
#51570=CARTESIAN_POINT('Ctrl Pts',(-4.15294117552302,-11.8268193877146,
-24.8084374579634));
#51571=CARTESIAN_POINT('Ctrl Pts',(-4.14915944275316,-11.827656178897,-24.8080532517044));
#51572=CARTESIAN_POINT('Ctrl Pts',(-4.14539731022808,-11.828487445453,-24.8076716226047));
#51573=CARTESIAN_POINT('Ctrl Pts',(-4.14165478808721,-11.8293132201818,
-24.8072925540389));
#51574=CARTESIAN_POINT('Ctrl Pts',(-4.13978352701677,-11.8297261075463,
-24.807103019756));
#51575=CARTESIAN_POINT('Ctrl Pts',(-4.13791716854239,-11.8301376219541,
-24.806914125607));
#51576=CARTESIAN_POINT('Ctrl Pts',(-4.13605571391661,-11.8305477674734,
-24.8067258695314));
#51577=CARTESIAN_POINT('Ctrl Pts',(-4.13419425929082,-11.8309579129926,
-24.8065376134559));
#51578=CARTESIAN_POINT('Ctrl Pts',(-4.13409016851678,-11.8309811013436,
-24.8065269615135));
#51579=CARTESIAN_POINT('Ctrl Pts',(-4.13048606283315,-11.8317741014242,
-24.806163013471));
#51580=CARTESIAN_POINT('Ctrl Pts',(-4.08691193608046,-11.8413615799999,
-24.8017628322536));
#51581=CARTESIAN_POINT('Ctrl Pts',(-4.04447551158591,-11.8505510334919,
-24.7975506165548));
#51582=CARTESIAN_POINT('Ctrl Pts',(-4.00318382527373,-11.859363884762,-24.7935152675936));
#51583=CARTESIAN_POINT('Ctrl Pts',(-3.90005318300528,-11.8813749744723,
-24.7834365285712));
#51584=CARTESIAN_POINT('Ctrl Pts',(-3.80406510876868,-11.9010396405033,
-24.7744594735136));
#51585=CARTESIAN_POINT('Ctrl Pts',(-3.71531264757601,-11.9186665884889,
-24.7664288201101));
#51586=CARTESIAN_POINT('Ctrl Pts',(-3.6270765161079,-11.9361909892655,-24.758444886144));
#51587=CARTESIAN_POINT('Ctrl Pts',(-3.54599178802324,-11.9517014694679,
-24.7513963839144));
#51588=CARTESIAN_POINT('Ctrl Pts',(-3.4721292318734,-11.9654603838603,-24.7451537349961));
#51589=CARTESIAN_POINT('Ctrl Pts',(-3.41383650114598,-11.9763189938731,
-24.7402270025435));
#51590=CARTESIAN_POINT('Ctrl Pts',(-3.36004163248443,-11.986085873297,-24.7358026394847));
#51591=CARTESIAN_POINT('Ctrl Pts',(-3.3107717495728,-11.9948708904099,-24.7318271128458));
#51592=CARTESIAN_POINT('Ctrl Pts',(-3.27749896763286,-12.0008035604602,
-24.7291423727341));
#51593=CARTESIAN_POINT('Ctrl Pts',(-3.24628968207182,-12.0062880984038,
-24.726662511234));
#51594=CARTESIAN_POINT('Ctrl Pts',(-3.21715071542865,-12.0113537837853,
-24.7243733815959));
#51595=CARTESIAN_POINT('Ctrl Pts',(-3.20258123210707,-12.013886626476,-24.7232288167768));
#51596=CARTESIAN_POINT('Ctrl Pts',(-3.18852932852064,-12.0163147568122,
-24.7221319365904));
#51597=CARTESIAN_POINT('Ctrl Pts',(-3.17499573068162,-12.0186414143701,
-24.7210811821799));
#51598=CARTESIAN_POINT('Ctrl Pts',(-3.16822893176211,-12.019804743149,-24.7205558049746));
#51599=CARTESIAN_POINT('Ctrl Pts',(-3.16159170927972,-12.0209427037737,
-24.7200419592991));
#51600=CARTESIAN_POINT('Ctrl Pts',(-3.15508415103286,-12.0220556892655,
-24.7195394565085));
#51601=CARTESIAN_POINT('Ctrl Pts',(-3.15183037190943,-12.0226121820114,
-24.7192882051131));
#51602=CARTESIAN_POINT('Ctrl Pts',(-3.14860900884489,-12.0231624309762,
-24.7190397894436));
#51603=CARTESIAN_POINT('Ctrl Pts',(-3.14542007238591,-12.0237064837776,
-24.7187941866655));
#51604=CARTESIAN_POINT('Ctrl Pts',(-3.14223113592693,-12.024250536579,-24.7185485838875));
#51605=CARTESIAN_POINT('Ctrl Pts',(-3.13737712873962,-12.0250773021456,
-24.7181753876997));
#51606=CARTESIAN_POINT('Ctrl Pts',(-3.13595055324829,-12.0253201008564,
-24.7180657944062));
#51607=CARTESIAN_POINT('Ctrl Pts',(-3.12014621424304,-12.0280099501904,
-24.7168516633817));
#51608=CARTESIAN_POINT('Ctrl Pts',(-3.09726104736722,-12.031904238561,-24.7150939460526));
#51609=CARTESIAN_POINT('Ctrl Pts',(-3.06727915293222,-12.0369286672949,
-24.7128278062112));
#51610=CARTESIAN_POINT('Ctrl Pts',(-3.03741245210651,-12.0419337916422,
-24.7105703731186));
#51611=CARTESIAN_POINT('Ctrl Pts',(-3.00050337107899,-12.0480604207122,
-24.7078084254843));
#51612=CARTESIAN_POINT('Ctrl Pts',(-2.95652738924272,-12.0551889523713,
-24.7045982342559));
#51613=CARTESIAN_POINT('Ctrl Pts',(-2.93861217079074,-12.0580930194684,
-24.7032904458966));
#51614=CARTESIAN_POINT('Ctrl Pts',(-2.91952400847139,-12.0611628292699,
-24.7019085134711));
#51615=CARTESIAN_POINT('Ctrl Pts',(-2.89926087788367,-12.0643880612036,
-24.7004572665812));
#51616=CARTESIAN_POINT('Ctrl Pts',(-2.84967927860436,-12.0722798406417,
-24.6969062288261));
#51617=CARTESIAN_POINT('Ctrl Pts',(-2.79306320304649,-12.081105438518,-24.692938717703));
#51618=CARTESIAN_POINT('Ctrl Pts',(-2.72937889016979,-12.0906809535796,
-24.688640353631));
#51619=CARTESIAN_POINT('Ctrl Pts',(-2.66611327954161,-12.1001935129539,
-24.6843702498105));
#51620=CARTESIAN_POINT('Ctrl Pts',(-2.59587189460584,-12.1104462002574,
-24.679773650128));
#51621=CARTESIAN_POINT('Ctrl Pts',(-2.51861770667281,-12.1212119874621,
-24.6749552284126));
#51622=CARTESIAN_POINT('Ctrl Pts',(-2.46588273788183,-12.1285608894109,
-24.6716660951555));
#51623=CARTESIAN_POINT('Ctrl Pts',(-2.40987996295885,-12.1361479142357,
-24.6682740289955));
#51624=CARTESIAN_POINT('Ctrl Pts',(-2.35059722570636,-12.1438880278938,
-24.6648178614771));
#51625=CARTESIAN_POINT('Ctrl Pts',(-2.31881048271695,-12.1480381905711,
-24.6629647029738));
#51626=CARTESIAN_POINT('Ctrl Pts',(-2.28608075398001,-12.1522321864854,
-24.6610931921645));
#51627=CARTESIAN_POINT('Ctrl Pts',(-2.25240618558163,-12.1564556378308,
-24.6592098515184));
#51628=CARTESIAN_POINT('Ctrl Pts',(-2.23556890138244,-12.1585673635036,
-24.6582681811953));
#51629=CARTESIAN_POINT('Ctrl Pts',(-2.21849540726422,-12.1606864526718,
-24.6573235526666));
#51630=CARTESIAN_POINT('Ctrl Pts',(-2.20118547572961,-12.1628110079849,
-24.6563768240204));
#51631=CARTESIAN_POINT('Ctrl Pts',(-2.19253050996231,-12.1638732856414,
-24.6559034596973));
#51632=CARTESIAN_POINT('Ctrl Pts',(-2.18381643484066,-12.16493692981,-24.6554295702951));
#51633=CARTESIAN_POINT('Ctrl Pts',(-2.1750432221839,-12.1660017003922,-24.6549552641153));
#51634=CARTESIAN_POINT('Ctrl Pts',(-2.16846331269133,-12.1668002783289,
-24.6545995344804));
#51635=CARTESIAN_POINT('Ctrl Pts',(-2.16185013833523,-12.1675994898712,
-24.6542435704039));
#51636=CARTESIAN_POINT('Ctrl Pts',(-2.1552036872966,-12.1683992325303,-24.6538874180593));
#51637=CARTESIAN_POINT('Ctrl Pts',(-2.15298820361706,-12.1686658134167,
-24.6537687006112));
#51638=CARTESIAN_POINT('Ctrl Pts',(-2.14946255514892,-12.1690891997327,
-24.6535801640996));
#51639=CARTESIAN_POINT('Ctrl Pts',(-2.14854614359989,-12.1691991483266,
-24.6535312047162));
#51640=CARTESIAN_POINT('Ctrl Pts',(-2.01285727760659,-12.1854787336713,
-24.6462820127763));
#51641=CARTESIAN_POINT('Ctrl Pts',(-1.87311902797097,-12.200646089438,-24.6395546412827));
#51642=CARTESIAN_POINT('Ctrl Pts',(-1.72934488862509,-12.2144325023485,
-24.6334653588438));
#51643=CARTESIAN_POINT('Ctrl Pts',(-1.55033452716363,-12.2315976947092,
-24.6258837126911));
#51644=CARTESIAN_POINT('Ctrl Pts',(-1.3650667468862,-12.2466229246189,-24.6192915670951));
#51645=CARTESIAN_POINT('Ctrl Pts',(-1.17358542883385,-12.2589711971898,
-24.613901599077));
#51646=CARTESIAN_POINT('Ctrl Pts',(-0.995034417419455,-12.2704856184357,
-24.6088756035861));
#51647=CARTESIAN_POINT('Ctrl Pts',(-0.811080765511128,-12.279672079365,
-24.6048950353104));
#51648=CARTESIAN_POINT('Ctrl Pts',(-0.621784930580049,-12.2860629160544,
-24.6021354957624));
#51649=CARTESIAN_POINT('Ctrl Pts',(-0.437714167124175,-12.2922773485535,
-24.5994521268886));
#51650=CARTESIAN_POINT('Ctrl Pts',(-0.248590430429552,-12.2958477298752,
-24.5979230997908));
#51651=CARTESIAN_POINT('Ctrl Pts',(-0.0545586007863394,-12.2963375937408,
-24.5977237909786));
#51652=CARTESIAN_POINT('Ctrl Pts',(0.0790391870814224,-12.2966748823647,
-24.5975865598012));
#51653=CARTESIAN_POINT('Ctrl Pts',(0.214962940974409,-12.2955512908672,
-24.5980798261454));
#51654=CARTESIAN_POINT('Ctrl Pts',(0.353152334498822,-12.2928182131356,
-24.5992620301425));
#51655=CARTESIAN_POINT('Ctrl Pts',(0.484530631885856,-12.2902198436815,
-24.600385965521));
#51656=CARTESIAN_POINT('Ctrl Pts',(0.617956409124449,-12.286166616767,-24.6021323416886));
#51657=CARTESIAN_POINT('Ctrl Pts',(0.753387341602309,-12.2805320625146,
-24.6045701077575));
#51658=CARTESIAN_POINT('Ctrl Pts',(0.832599513683294,-12.2772364691603,
-24.6059959322853));
#51659=CARTESIAN_POINT('Ctrl Pts',(0.912497523784989,-12.2733998517983,
-24.6076583513174));
#51660=CARTESIAN_POINT('Ctrl Pts',(0.993071860718278,-12.2689964190193,
-24.6095717929907));
#51661=CARTESIAN_POINT('Ctrl Pts',(1.03335902918492,-12.2667947026297,-24.6105285138274));
#51662=CARTESIAN_POINT('Ctrl Pts',(1.07381527937235,-12.2644512842182,-24.6115479940166));
#51663=CARTESIAN_POINT('Ctrl Pts',(1.11443933315437,-12.2619628983529,-24.6126320861955));
#51664=CARTESIAN_POINT('Ctrl Pts',(1.13475136004538,-12.2607187054203,-24.613174132285));
#51665=CARTESIAN_POINT('Ctrl Pts',(1.1551053378358,-12.2594382707433,-24.6137323316115));
#51666=CARTESIAN_POINT('Ctrl Pts',(1.17550110411703,-12.258121185405,-24.6143069179415));
#51667=CARTESIAN_POINT('Ctrl Pts',(1.18569898725765,-12.2574626427358,-24.6145942111066));
#51668=CARTESIAN_POINT('Ctrl Pts',(1.19590731752102,-12.2567949374089,-24.6148856010378));
#51669=CARTESIAN_POINT('Ctrl Pts',(1.20612607429678,-12.2561180181637,-24.6151811171442));
#51670=CARTESIAN_POINT('Ctrl Pts',(1.21003383986061,-12.2558591567607,-24.6152941257703));
#51671=CARTESIAN_POINT('Ctrl Pts',(1.21394313017906,-12.2555989479443,-24.6154077377951));
#51672=CARTESIAN_POINT('Ctrl Pts',(1.21785394409128,-12.2553373888361,-24.6155219548719));
#51673=CARTESIAN_POINT('Ctrl Pts',(1.21905649426289,-12.2552569610894,-24.6155570758897));
#51674=CARTESIAN_POINT('Ctrl Pts',(1.22025918849377,-12.2551764056696,-24.6155922541167));
#51675=CARTESIAN_POINT('Ctrl Pts',(1.22146202675023,-12.2550957224978,-24.6156274895932));
#51676=CARTESIAN_POINT('Ctrl Pts',(1.22401932127499,-12.2549241860237,-24.6157024019855));
#51677=CARTESIAN_POINT('Ctrl Pts',(1.22657726680809,-12.254752072081,-24.6157775731603));
#51678=CARTESIAN_POINT('Ctrl Pts',(1.22913586302588,-12.2545793799462,-24.615853003491));
#51679=CARTESIAN_POINT('Ctrl Pts',(1.23169445924366,-12.2544066878115,-24.6159284338216));
#51680=CARTESIAN_POINT('Ctrl Pts',(1.23563112026502,-12.2541398736881,-24.6160449895183));
#51681=CARTESIAN_POINT('Ctrl Pts',(1.23681360340771,-12.2540595681746,-24.6160800723573));
#51682=CARTESIAN_POINT('Ctrl Pts',(1.30415698594497,-12.2494861034709,-24.6180780687402));
#51683=CARTESIAN_POINT('Ctrl Pts',(1.37864973085997,-12.2440404697575,-24.6204626949177));
#51684=CARTESIAN_POINT('Ctrl Pts',(1.46026015657689,-12.2374742450696,-24.6233466830752));
#51685=CARTESIAN_POINT('Ctrl Pts',(1.54192304891292,-12.2309037990141,-24.6262325253231));
#51686=CARTESIAN_POINT('Ctrl Pts',(1.63071299872235,-12.2232112393102,-24.6296183548054));
#51687=CARTESIAN_POINT('Ctrl Pts',(1.72658504127951,-12.2141023251319,-24.6336393175605));
#51688=CARTESIAN_POINT('Ctrl Pts',(1.81123505362126,-12.2060596290858,-24.6371896179166));
#51689=CARTESIAN_POINT('Ctrl Pts',(1.90140617161389,-12.1969120518504,-24.6412353762544));
#51690=CARTESIAN_POINT('Ctrl Pts',(1.99705663526021,-12.1864285395999,-24.6458841574754));
#51691=CARTESIAN_POINT('Ctrl Pts',(2.1063311141233,-12.1744518037413,-24.6511950898631));
#51692=CARTESIAN_POINT('Ctrl Pts',(2.22275766737551,-12.1607320046081,-24.6572926544663));
#51693=CARTESIAN_POINT('Ctrl Pts',(2.34625419832298,-12.1448874689547,-24.6643580022169));
#51694=CARTESIAN_POINT('Ctrl Pts',(2.46249284595542,-12.1299741156598,-24.6710081199268));
#51695=CARTESIAN_POINT('Ctrl Pts',(2.58499494385502,-12.113177944025,-24.6785157979436));
#51696=CARTESIAN_POINT('Ctrl Pts',(2.71367114819397,-12.0941490502631,-24.6870505947827));
#51697=CARTESIAN_POINT('Ctrl Pts',(2.74257980860118,-12.0898739798994,-24.6889680397736));
#51698=CARTESIAN_POINT('Ctrl Pts',(2.77180000479066,-12.0854860993413,-24.6909373986732));
#51699=CARTESIAN_POINT('Ctrl Pts',(2.80133057466338,-12.0809812862044,-24.692960694511));
#51700=CARTESIAN_POINT('Ctrl Pts',(2.82674885367853,-12.0771037925522,-24.6947022355093));
#51701=CARTESIAN_POINT('Ctrl Pts',(2.85519249015935,-12.0727095378522,-24.6966769976858));
#51702=CARTESIAN_POINT('Ctrl Pts',(2.8838692040386,-12.0682098270556,-24.6987006235588));
#51703=CARTESIAN_POINT('Ctrl Pts',(2.89904593783843,-12.0658284205519,-24.6997715981242));
#51704=CARTESIAN_POINT('Ctrl Pts',(2.91428809658606,-12.0634182291851,-24.7008559061583));
#51705=CARTESIAN_POINT('Ctrl Pts',(2.92918282625697,-12.0610456032668,-24.7019236870447));
#51706=CARTESIAN_POINT('Ctrl Pts',(3.02452065291981,-12.0458589564775,-24.708758313205));
#51707=CARTESIAN_POINT('Ctrl Pts',(3.11288303257106,-12.031070308535,-24.7154292262998));
#51708=CARTESIAN_POINT('Ctrl Pts',(3.19431902969002,-12.0169622138921,-24.7218050079397));
#51709=CARTESIAN_POINT('Ctrl Pts',(3.25134055683339,-12.0070837187538,-24.7262693335292));
#51710=CARTESIAN_POINT('Ctrl Pts',(3.3049662326169,-11.9975378488254,-24.7305893943761));
#51711=CARTESIAN_POINT('Ctrl Pts',(3.35521234116895,-11.9884076807588,-24.7347260891693));
#51712=CARTESIAN_POINT('Ctrl Pts',(3.42777530415416,-11.9752223403105,-24.7407001006861));
#51713=CARTESIAN_POINT('Ctrl Pts',(3.49329025741202,-11.9629060207124,-24.7462907649862));
#51714=CARTESIAN_POINT('Ctrl Pts',(3.55180244408811,-11.9516685494414,-24.7513984144608));
#51715=CARTESIAN_POINT('Ctrl Pts',(3.61060203492046,-11.9403758811912,-24.756531152037));
#51716=CARTESIAN_POINT('Ctrl Pts',(3.66233004929159,-11.9301726003974,-24.7611761093311));
#51717=CARTESIAN_POINT('Ctrl Pts',(3.7070253556445,-11.9212240723819,-24.7652538073756));
#51718=CARTESIAN_POINT('Ctrl Pts',(3.75194669933796,-11.9122302890221,-24.7693521275411));
#51719=CARTESIAN_POINT('Ctrl Pts',(3.78976414426838,-11.9045039244158,-24.7728774247372));
#51720=CARTESIAN_POINT('Ctrl Pts',(3.82050797835506,-11.8981660086328,-24.7757709934024));
#51721=CARTESIAN_POINT('Ctrl Pts',(3.82703718787525,-11.8968199962925,-24.7763855138953));
#51722=CARTESIAN_POINT('Ctrl Pts',(3.83324732017357,-11.8955364413545,-24.7769716204608));
#51723=CARTESIAN_POINT('Ctrl Pts',(3.83913860511669,-11.894316236168,-24.7775288783472));
#51724=CARTESIAN_POINT('Ctrl Pts',(3.85140018573146,-11.8917766129102,-24.7786887038459));
#51725=CARTESIAN_POINT('Ctrl Pts',(3.86228059655449,-11.8895115217444,-24.7797235077149));
#51726=CARTESIAN_POINT('Ctrl Pts',(3.87178159558094,-11.8875277080389,-24.7806299973009));
#51727=CARTESIAN_POINT('Ctrl Pts',(3.87653209509417,-11.8865358011862,-24.781083242094));
#51728=CARTESIAN_POINT('Ctrl Pts',(3.88093774165891,-11.8856142138884,-24.781504408725));
#51729=CARTESIAN_POINT('Ctrl Pts',(3.88499870666068,-11.8847635947793,-24.7818931792817));
#51730=CARTESIAN_POINT('Ctrl Pts',(3.88702918916156,-11.8843382852248,-24.78208756456));
#51731=CARTESIAN_POINT('Ctrl Pts',(3.88897350127174,-11.8839307177306,-24.7822738508481));
#51732=CARTESIAN_POINT('Ctrl Pts',(3.89083166298951,-11.8835409680762,-24.7824520010861));
#51733=CARTESIAN_POINT('Ctrl Pts',(3.89176074384839,-11.8833460932489,-24.7825410762051));
#51734=CARTESIAN_POINT('Ctrl Pts',(3.89266828710916,-11.8831556728825,-24.7826281173135));
#51735=CARTESIAN_POINT('Ctrl Pts',(3.89355429510512,-11.8829697157939,-24.7827131200975));
#51736=CARTESIAN_POINT('Ctrl Pts',(3.89399729910309,-11.8828767372495,-24.7827556214894));
#51737=CARTESIAN_POINT('Ctrl Pts',(3.89443491926945,-11.8827848744668,-24.7827976133288));
#51738=CARTESIAN_POINT('Ctrl Pts',(3.89486446602496,-11.8826946941185,-24.7828388365331));
#51739=CARTESIAN_POINT('Ctrl Pts',(3.89529401278048,-11.8826045137702,-24.7828800597375));
#51740=CARTESIAN_POINT('Ctrl Pts',(3.89572088452154,-11.8825149548244,-24.7829209970462));
#51741=CARTESIAN_POINT('Ctrl Pts',(3.89744544075142,-11.8821526702451,-24.7830866116476));
#51742=CARTESIAN_POINT('Ctrl Pts',(3.90615289621541,-11.880323459469,-24.7839228161979));
#51743=CARTESIAN_POINT('Ctrl Pts',(3.91484190904383,-11.878492241168,-24.7847601238004));
#51744=CARTESIAN_POINT('Ctrl Pts',(3.92351248770123,-11.8766590889184,-24.7855985015432));
#51745=CARTESIAN_POINT('Ctrl Pts',(4.08352426403357,-11.8428290575766,-24.8010703999214));
#51746=CARTESIAN_POINT('Ctrl Pts',(4.23725683184937,-11.808344456804,-24.8169055229193));
#51747=CARTESIAN_POINT('Ctrl Pts',(4.38477077580503,-11.773645900217,-24.8329066121935));
#51748=CARTESIAN_POINT('Ctrl Pts',(4.40473563417751,-11.7689497220158,-24.8350722344567));
#51749=CARTESIAN_POINT('Ctrl Pts',(4.42458660093341,-11.7642495521737,-24.8372409190368));
#51750=CARTESIAN_POINT('Ctrl Pts',(4.44432384241394,-11.7595464156776,-24.8394121977579));
#51751=CARTESIAN_POINT('Ctrl Pts',(4.59308111763143,-11.7240994272611,-24.8557768709375));
#51752=CARTESIAN_POINT('Ctrl Pts',(4.73537748962768,-11.6884880158654,-24.8722877337365));
#51753=CARTESIAN_POINT('Ctrl Pts',(4.87128883771487,-11.6531251539034,-24.8887562362082));
#51754=CARTESIAN_POINT('Ctrl Pts',(4.89544337944055,-11.6468403679984,-24.8916830641421));
#51755=CARTESIAN_POINT('Ctrl Pts',(4.91939627029786,-11.6405633068695,-24.8946085907191));
#51756=CARTESIAN_POINT('Ctrl Pts',(4.94314796326616,-11.634296127747,-24.8975318051419));
#51757=CARTESIAN_POINT('Ctrl Pts',(5.07995159612902,-11.5981987904793,-24.914368767173));
#51758=CARTESIAN_POINT('Ctrl Pts',(5.21008001675493,-11.562433404087,-24.931127948449));
#51759=CARTESIAN_POINT('Ctrl Pts',(5.33362132823233,-11.5273836985521,-24.947629563727));
#51760=CARTESIAN_POINT('Ctrl Pts',(5.3698064122361,-11.5171176869329,-24.9524628646519));
#51761=CARTESIAN_POINT('Ctrl Pts',(5.40542643050983,-11.5069127441063,-24.9572741575169));
#51762=CARTESIAN_POINT('Ctrl Pts',(5.44048367932361,-11.4967777094823,-24.9620591479588));
#51763=CARTESIAN_POINT('Ctrl Pts',(5.5634076792632,-11.46124043723,-24.9788371378094));
#51764=CARTESIAN_POINT('Ctrl Pts',(5.67941229692956,-11.426566627261,-24.9952908229024));
#51765=CARTESIAN_POINT('Ctrl Pts',(5.78859481050879,-11.3931049741266,-25.0112500391612));
#51766=CARTESIAN_POINT('Ctrl Pts',(5.84240057663458,-11.3766148803953,-25.0191148320609));
#51767=CARTESIAN_POINT('Ctrl Pts',(5.89454960328078,-11.3604183740888,-25.0268597295277));
#51768=CARTESIAN_POINT('Ctrl Pts',(5.94505368243095,-11.3445527218703,-25.0344655498479));
#51769=CARTESIAN_POINT('Ctrl Pts',(5.95968231208449,-11.3399571970251,-25.0366685942464));
#51770=CARTESIAN_POINT('Ctrl Pts',(5.97417293278451,-11.3353894121292,-25.0388599757614));
#51771=CARTESIAN_POINT('Ctrl Pts',(5.98852581858904,-11.3308502293444,-25.0410392599613));
#51772=CARTESIAN_POINT('Ctrl Pts',(-6.39567215542467,-11.8440001024728,
-24.2657748968686));
#51773=CARTESIAN_POINT('Ctrl Pts',(-6.35564925618098,-11.8565901643257,
-24.2594187494307));
#51774=CARTESIAN_POINT('Ctrl Pts',(-5.98524940757696,-11.9719910115992,
-24.2012637897805));
#51775=CARTESIAN_POINT('Ctrl Pts',(-5.25616631904133,-12.1789676278653,
-24.0987566446471));
#51776=CARTESIAN_POINT('Ctrl Pts',(-4.1757614528087,-12.4300245021709,-23.9769546135746));
#51777=CARTESIAN_POINT('Ctrl Pts',(-3.01936948336144,-12.6350408997157,
-23.8792988421013));
#51778=CARTESIAN_POINT('Ctrl Pts',(-1.83578686335412,-12.7756187619401,
-23.8136687413269));
#51779=CARTESIAN_POINT('Ctrl Pts',(-0.697923544232415,-12.8441382007264,
-23.782558252307));
#51780=CARTESIAN_POINT('Ctrl Pts',(0.331409741550182,-12.8512034879543,
-23.7794557881091));
#51781=CARTESIAN_POINT('Ctrl Pts',(1.24580985113917,-12.8144571656071,-23.7959567162203));
#51782=CARTESIAN_POINT('Ctrl Pts',(2.0703011525311,-12.7465811278717,-23.8272319476035));
#51783=CARTESIAN_POINT('Ctrl Pts',(2.81706942635404,-12.6564395388812,-23.8693929263403));
#51784=CARTESIAN_POINT('Ctrl Pts',(3.49018596890746,-12.5517033164802,-23.9189811921973));
#51785=CARTESIAN_POINT('Ctrl Pts',(4.09497305511126,-12.4387782665359,-23.9729948461712));
#51786=CARTESIAN_POINT('Ctrl Pts',(4.65005393633298,-12.3195528639124,-24.0305544994279));
#51787=CARTESIAN_POINT('Ctrl Pts',(5.18050287209621,-12.1916401414439,-24.0928853069425));
#51788=CARTESIAN_POINT('Ctrl Pts',(5.70542267295585,-12.0514960850741,-24.1618790928945));
#51789=CARTESIAN_POINT('Ctrl Pts',(6.10978283806977,-11.9329730134373,-24.2209473269322));
#51790=CARTESIAN_POINT('Ctrl Pts',(6.34031611249689,-11.8614128328345,-24.2569837007452));
#51791=CARTESIAN_POINT('Ctrl Pts',(6.39541677164253,-11.8440802209038,-24.2657356729641));
#51792=CARTESIAN_POINT('Ctrl Pts',(-6.33018795450903,-11.8153030248918,
-24.6384814580648));
#51793=CARTESIAN_POINT('Ctrl Pts',(-6.29063921510137,-11.8278586316894,
-24.6322059111688));
#51794=CARTESIAN_POINT('Ctrl Pts',(-5.9246003059131,-11.9429535886473,-24.5747847388569));
#51795=CARTESIAN_POINT('Ctrl Pts',(-5.20363640375749,-12.1495431753517,
-24.4735093872846));
#51796=CARTESIAN_POINT('Ctrl Pts',(-4.13466319834969,-12.400333149385,-24.3531155353953));
#51797=CARTESIAN_POINT('Ctrl Pts',(-2.99013101626481,-12.6052506194047,
-24.2565628937697));
#51798=CARTESIAN_POINT('Ctrl Pts',(-1.81835018697561,-12.7458213587748,
-24.1916588641543));
#51799=CARTESIAN_POINT('Ctrl Pts',(-0.691526419463407,-12.8143591144599,
-24.1608816865859));
#51800=CARTESIAN_POINT('Ctrl Pts',(0.328410955103737,-12.8214279221244,
-24.1578109793223));
#51801=CARTESIAN_POINT('Ctrl Pts',(1.23410624365119,-12.7846688139739,-24.1741376713656));
#51802=CARTESIAN_POINT('Ctrl Pts',(2.05052545184689,-12.7167848350623,-24.2050718889341));
#51803=CARTESIAN_POINT('Ctrl Pts',(2.78983578881101,-12.6266522506618,-24.2467655952706));
#51804=CARTESIAN_POINT('Ctrl Pts',(3.45611831470981,-12.5219522866885,-24.2957971475504));
#51805=CARTESIAN_POINT('Ctrl Pts',(4.05467056771375,-12.4090965633996,-24.3491974594818));
#51806=CARTESIAN_POINT('Ctrl Pts',(4.60393606416149,-12.2899790555555,-24.4060956630845));
#51807=CARTESIAN_POINT('Ctrl Pts',(5.12872017337514,-12.1622243332721,-24.4676997961477));
#51808=CARTESIAN_POINT('Ctrl Pts',(5.64789136142997,-12.022309291172,-24.5358734405517));
#51809=CARTESIAN_POINT('Ctrl Pts',(6.04766215329681,-11.904040942247,-24.5942191807346));
#51810=CARTESIAN_POINT('Ctrl Pts',(6.27548786378983,-11.8326680689264,-24.6298017767411));
#51811=CARTESIAN_POINT('Ctrl Pts',(6.32993527380381,-11.8153829807007,-24.6384426479982));
#51812=CARTESIAN_POINT('Ctrl Pts',(-6.21932914003729,-11.6046077138231,
-24.933941067311));
#51813=CARTESIAN_POINT('Ctrl Pts',(-6.18048424948508,-11.6170331460216,
-24.9278367279444));
#51814=CARTESIAN_POINT('Ctrl Pts',(-5.82094614637916,-11.7309405707257,
-24.871982184622));
#51815=CARTESIAN_POINT('Ctrl Pts',(-5.11256398456841,-11.9354888600937,
-24.7734733502725));
#51816=CARTESIAN_POINT('Ctrl Pts',(-4.06219748998055,-12.1838752205529,
-24.656435331966));
#51817=CARTESIAN_POINT('Ctrl Pts',(-2.93773430970566,-12.3868544707923,
-24.5626392307631));
#51818=CARTESIAN_POINT('Ctrl Pts',(-1.78661004834439,-12.5261043229835,
-24.4996240375242));
#51819=CARTESIAN_POINT('Ctrl Pts',(-0.679627595412669,-12.5940042619886,
-24.469747090831));
#51820=CARTESIAN_POINT('Ctrl Pts',(0.32279241813113,-12.6010084102561,-24.4667652656686));
#51821=CARTESIAN_POINT('Ctrl Pts',(1.21265278063735,-12.5645895081712,-24.4826158046806));
#51822=CARTESIAN_POINT('Ctrl Pts',(2.01469390807635,-12.4973407985779,-24.5126460662249));
#51823=CARTESIAN_POINT('Ctrl Pts',(2.74097574449004,-12.40805553802,-24.5531296341404));
#51824=CARTESIAN_POINT('Ctrl Pts',(3.39554807864259,-12.3043438963876,-24.6007526810749));
#51825=CARTESIAN_POINT('Ctrl Pts',(3.98362077418606,-12.192558706476,-24.652636935921));
#51826=CARTESIAN_POINT('Ctrl Pts',(4.5233025684579,-12.0745788464337,-24.7079386489045));
#51827=CARTESIAN_POINT('Ctrl Pts',(5.03894734293331,-11.9480565297811,-24.7678332938225));
#51828=CARTESIAN_POINT('Ctrl Pts',(5.54906664696171,-11.8095120106988,-24.8341333987973));
#51829=CARTESIAN_POINT('Ctrl Pts',(5.94181973580656,-11.6924305250497,-24.8908864048995));
#51830=CARTESIAN_POINT('Ctrl Pts',(6.16560267824642,-11.6217926877057,-24.9254982178085));
#51831=CARTESIAN_POINT('Ctrl Pts',(6.21908066379017,-11.6046868956139,-24.9339032360192));
#51832=CARTESIAN_POINT('Ctrl Pts',(-6.09478101909931,-11.2722125663433,
-25.0678681419845));
#51833=CARTESIAN_POINT('Ctrl Pts',(-6.05666854227872,-11.2844493451113,
-25.0619766664134));
#51834=CARTESIAN_POINT('Ctrl Pts',(-5.70391349769389,-11.3966273350641,
-25.0080736685403));
#51835=CARTESIAN_POINT('Ctrl Pts',(-5.00898011870794,-11.5980641644672,
-24.9130750297103));
#51836=CARTESIAN_POINT('Ctrl Pts',(-3.97907763477767,-11.8425981319446,
-24.8003808773973));
#51837=CARTESIAN_POINT('Ctrl Pts',(-2.8771566178203,-12.0423546994034,-24.7102064331904));
#51838=CARTESIAN_POINT('Ctrl Pts',(-1.74963938185109,-12.1793480627038,
-24.6497026624673));
#51839=CARTESIAN_POINT('Ctrl Pts',(-0.66562847075,-12.2461366725668,-24.6210354030492));
#51840=CARTESIAN_POINT('Ctrl Pts',(0.316160263864133,-12.2530264963728,
-24.6181741642278));
#51841=CARTESIAN_POINT('Ctrl Pts',(1.18758201207714,-12.2172033812172,-24.6333828131016));
#51842=CARTESIAN_POINT('Ctrl Pts',(1.97304891122712,-12.1510512680947,-24.662204699665));
#51843=CARTESIAN_POINT('Ctrl Pts',(2.68445564141552,-12.0632090701854,-24.7010813430047));
#51844=CARTESIAN_POINT('Ctrl Pts',(3.32578864566661,-11.961154888898,-24.7468468918969));
#51845=CARTESIAN_POINT('Ctrl Pts',(3.90213225627227,-11.8511350032299,-24.7967459194263));
#51846=CARTESIAN_POINT('Ctrl Pts',(4.43120108774589,-11.7349969248286,-24.849972634402));
#51847=CARTESIAN_POINT('Ctrl Pts',(4.93684397707271,-11.6104287119617,-24.9076638088831));
#51848=CARTESIAN_POINT('Ctrl Pts',(5.43719497822094,-11.4740040324212,-24.9715726993592));
#51849=CARTESIAN_POINT('Ctrl Pts',(5.82250744905605,-11.3587019609412,-25.0263181394208));
#51850=CARTESIAN_POINT('Ctrl Pts',(6.04206764945466,-11.2891366012123,-25.0597197276758));
#51851=CARTESIAN_POINT('Ctrl Pts',(6.09453704716553,-11.2722905841804,-25.0678315745393));
#51852=CARTESIAN_POINT('',(6.27159454870591,-11.879492346709,-24.2690137147315));
#51853=CARTESIAN_POINT('Origin',(5.999999949022,-10.92778026693,-24.1259420051984));
#51854=CARTESIAN_POINT('Ctrl Pts',(-6.2715938732803,-11.8794984953269,-24.269012375374));
#51855=CARTESIAN_POINT('Ctrl Pts',(-6.13239663762701,-11.9224692223419,
-24.2474082712106));
#51856=CARTESIAN_POINT('Ctrl Pts',(-5.98564490228836,-11.9663158806333,
-24.2255025400386));
#51857=CARTESIAN_POINT('Ctrl Pts',(-5.8313286107345,-12.0105539104888,-24.2035349755448));
#51858=CARTESIAN_POINT('Ctrl Pts',(-5.67907405556145,-12.0542008999905,
-24.1818609077807));
#51859=CARTESIAN_POINT('Ctrl Pts',(-5.51945543077222,-12.0982289054275,
-24.1601268768661));
#51860=CARTESIAN_POINT('Ctrl Pts',(-5.35247238148756,-12.1421228678868,
-24.1385689856038));
#51861=CARTESIAN_POINT('Ctrl Pts',(-5.32566688848742,-12.1491690878984,
-24.1351083355211));
#51862=CARTESIAN_POINT('Ctrl Pts',(-5.29867164443853,-12.1562117478511,
-24.1316522325387));
#51863=CARTESIAN_POINT('Ctrl Pts',(-5.27148667848168,-12.1632485947852,
-24.1282016614138));
#51864=CARTESIAN_POINT('Ctrl Pts',(-5.14595415318808,-12.1957427743678,
-24.1122678946509));
#51865=CARTESIAN_POINT('Ctrl Pts',(-5.01637573150645,-12.2281142363005,
-24.0964517500017));
#51866=CARTESIAN_POINT('Ctrl Pts',(-4.882757385002,-12.26013253772,-24.0808623957014));
#51867=CARTESIAN_POINT('Ctrl Pts',(-4.711064069478,-12.301274555055,-24.0608308057534));
#51868=CARTESIAN_POINT('Ctrl Pts',(-4.5326954979539,-12.3418362421708,-24.0411729378986));
#51869=CARTESIAN_POINT('Ctrl Pts',(-4.34764548374925,-12.3812950798105,
-24.0221340537593));
#51870=CARTESIAN_POINT('Ctrl Pts',(-4.2958405153995,-12.3923416276523,-24.0168040958315));
#51871=CARTESIAN_POINT('Ctrl Pts',(-4.24351200589396,-12.4033014559238,
-24.0115227210219));
#51872=CARTESIAN_POINT('Ctrl Pts',(-4.19066006814981,-12.4141624244733,
-24.0062954756857));
#51873=CARTESIAN_POINT('Ctrl Pts',(-4.14338502638451,-12.4238773519424,
-24.0016198052726));
#51874=CARTESIAN_POINT('Ctrl Pts',(-4.09569119111324,-12.4335131772699,
-23.996987443632));
#51875=CARTESIAN_POINT('Ctrl Pts',(-4.04757899088175,-12.4430611425052,
-23.9924025353514));
#51876=CARTESIAN_POINT('Ctrl Pts',(-3.90056247343951,-12.4722368732097,
-23.978392424715));
#51877=CARTESIAN_POINT('Ctrl Pts',(-3.749635972985,-12.5005941111466,-23.9648249555871));
#51878=CARTESIAN_POINT('Ctrl Pts',(-3.59479966513697,-12.5278747715792,
-23.9518214668319));
#51879=CARTESIAN_POINT('Ctrl Pts',(-3.51738151121296,-12.5415151017955,
-23.9453197224542));
#51880=CARTESIAN_POINT('Ctrl Pts',(-3.43898589682887,-12.5548860374477,
-23.9389590687969));
#51881=CARTESIAN_POINT('Ctrl Pts',(-3.35961279462372,-12.5679537431773,
-23.9327552486077));
#51882=CARTESIAN_POINT('Ctrl Pts',(-3.31992624352115,-12.5744875960422,
-23.9296533385131));
#51883=CARTESIAN_POINT('Ctrl Pts',(-3.27999531807212,-12.5809456256128,
-23.926590634974));
#51884=CARTESIAN_POINT('Ctrl Pts',(-3.23982001430566,-12.5873234964514,
-23.9235691505921));
#51885=CARTESIAN_POINT('Ctrl Pts',(-3.21973236242243,-12.5905124318707,
-23.9220584084011));
#51886=CARTESIAN_POINT('Ctrl Pts',(-3.19958361581005,-12.5936813265724,
-23.9205579708818));
#51887=CARTESIAN_POINT('Ctrl Pts',(-3.17937377348063,-12.5968296320843,
-23.9190680904652));
#51888=CARTESIAN_POINT('Ctrl Pts',(-3.16169016144239,-12.5995843994072,
-23.9177644451007));
#51889=CARTESIAN_POINT('Ctrl Pts',(-3.14395977298706,-12.6023234030703,
-23.916468882511));
#51890=CARTESIAN_POINT('Ctrl Pts',(-3.12618260735964,-12.6050462727838,
-23.9151815725702));
#51891=CARTESIAN_POINT('Ctrl Pts',(-3.12364301227001,-12.6054352541714,
-23.9149976711501));
#51892=CARTESIAN_POINT('Ctrl Pts',(-3.11986203723764,-12.6060134334648,
-23.9147243465347));
#51893=CARTESIAN_POINT('Ctrl Pts',(-3.11856095818475,-12.606212228053,-23.9146303740971));
#51894=CARTESIAN_POINT('Ctrl Pts',(-3.09161304666525,-12.6103296557857,
-23.9126840196999));
#51895=CARTESIAN_POINT('Ctrl Pts',(-3.06343997575514,-12.6145807550419,
-23.9106767095399));
#51896=CARTESIAN_POINT('Ctrl Pts',(-3.03404177228778,-12.618950273952,-23.9086156635078));
#51897=CARTESIAN_POINT('Ctrl Pts',(-2.96197568736319,-12.6296616128679,
-23.9035632623108));
#51898=CARTESIAN_POINT('Ctrl Pts',(-2.88254751287245,-12.641087839082,-23.8981864399));
#51899=CARTESIAN_POINT('Ctrl Pts',(-2.79575688315666,-12.6529718125133,
-23.8926067538628));
#51900=CARTESIAN_POINT('Ctrl Pts',(-2.70929650814212,-12.6648105651863,
-23.8870482995824));
#51901=CARTESIAN_POINT('Ctrl Pts',(-2.61552935566523,-12.6771036167269,
-23.8812885584487));
#51902=CARTESIAN_POINT('Ctrl Pts',(-2.51445615805138,-12.6895496271244,
-23.8754690386501));
#51903=CARTESIAN_POINT('Ctrl Pts',(-2.50259521508505,-12.6910101668418,
-23.8747861178159));
#51904=CARTESIAN_POINT('Ctrl Pts',(-2.49063366414967,-12.6924727591018,
-23.8741023976447));
#51905=CARTESIAN_POINT('Ctrl Pts',(-2.4785715099771,-12.6939368738316,-23.8734181258235));
#51906=CARTESIAN_POINT('Ctrl Pts',(-2.37688568616911,-12.706279587274,-23.8676496086209));
#51907=CARTESIAN_POINT('Ctrl Pts',(-2.26804987401106,-12.7187343062723,
-23.8618405787172));
#51908=CARTESIAN_POINT('Ctrl Pts',(-2.15206286682857,-12.7309579443555,
-23.856152503585));
#51909=CARTESIAN_POINT('Ctrl Pts',(-2.11969742264863,-12.734368873611,-23.8545652820276));
#51910=CARTESIAN_POINT('Ctrl Pts',(-2.08677519359464,-12.7377615266798,
-23.852987599166));
#51911=CARTESIAN_POINT('Ctrl Pts',(-2.05329627361692,-12.7411277873687,
-23.8514232425027));
#51912=CARTESIAN_POINT('Ctrl Pts',(-1.97656814623441,-12.748842698098,-23.8478379966998));
#51913=CARTESIAN_POINT('Ctrl Pts',(-1.89691554157196,-12.7564195700983,
-23.8443225621781));
#51914=CARTESIAN_POINT('Ctrl Pts',(-1.81433841441059,-12.7637550184018,
-23.8409252171504));
#51915=CARTESIAN_POINT('Ctrl Pts',(-1.81240161146196,-12.7639270674714,
-23.8408455342153));
#51916=CARTESIAN_POINT('Ctrl Pts',(-1.8104631997204,-12.7640989833751,-23.8407659162187));
#51917=CARTESIAN_POINT('Ctrl Pts',(-1.80852317916683,-12.7642707647223,
-23.8406863638458));
#51918=CARTESIAN_POINT('Ctrl Pts',(-1.7691060435725,-12.7677610002474,-23.8390700270161));
#51919=CARTESIAN_POINT('Ctrl Pts',(-1.72902475054208,-12.7711957218126,
-23.8374807696023));
#51920=CARTESIAN_POINT('Ctrl Pts',(-1.68827932336461,-12.7745632602754,
-23.8359241929636));
#51921=CARTESIAN_POINT('Ctrl Pts',(-1.66690391177416,-12.7763299007471,
-23.8351075990872));
#51922=CARTESIAN_POINT('Ctrl Pts',(-1.64534571982271,-12.7780780454456,
-23.8342999985264));
#51923=CARTESIAN_POINT('Ctrl Pts',(-1.62360474836943,-12.7798059674892,
-23.8335022087749));
#51924=CARTESIAN_POINT('Ctrl Pts',(-1.61273426264279,-12.7806699285111,
-23.8331033138992));
#51925=CARTESIAN_POINT('Ctrl Pts',(-1.60181808200573,-12.781528833429,-23.8327068716795));
#51926=CARTESIAN_POINT('Ctrl Pts',(-1.5908562065608,-12.7823824635436,-23.8323129856623));
#51927=CARTESIAN_POINT('Ctrl Pts',(-1.58537526883834,-12.7828092786009,
-23.8321160426538));
#51928=CARTESIAN_POINT('Ctrl Pts',(-1.57988290741174,-12.7832347749296,
-23.8319197386929));
#51929=CARTESIAN_POINT('Ctrl Pts',(-1.57437912229396,-12.7836589250135,
-23.8317240868131));
#51930=CARTESIAN_POINT('Ctrl Pts',(-1.56887533717618,-12.7840830750973,
-23.8315284349333));
#51931=CARTESIAN_POINT('Ctrl Pts',(-1.56205961010252,-12.7846050491578,
-23.8312877046057));
#51932=CARTESIAN_POINT('Ctrl Pts',(-1.55783349587533,-12.7849273088989,
-23.8311391004704));
#51933=CARTESIAN_POINT('Ctrl Pts',(-1.33210031738351,-12.8021404535854,
-23.8232015763092));
#51934=CARTESIAN_POINT('Ctrl Pts',(-1.1100537646997,-12.8153351589271,-23.8171220363203));
#51935=CARTESIAN_POINT('Ctrl Pts',(-0.89169689626609,-12.8248709187615,
-23.8127291065153));
#51936=CARTESIAN_POINT('Ctrl Pts',(-0.848420677506258,-12.8267608141039,
-23.8118584703287));
#51937=CARTESIAN_POINT('Ctrl Pts',(-0.805289281811483,-12.8285068906274,
-23.8110541625113));
#51938=CARTESIAN_POINT('Ctrl Pts',(-0.762302580912269,-12.8301118030515,
-23.810314964591));
#51939=CARTESIAN_POINT('Ctrl Pts',(-0.724716128547589,-12.8315150967009,
-23.80966862917));
#51940=CARTESIAN_POINT('Ctrl Pts',(-0.687240284721794,-12.8328104687764,
-23.8090720400251));
#51941=CARTESIAN_POINT('Ctrl Pts',(-0.649875247251341,-12.833999670689,
-23.8085242653197));
#51942=CARTESIAN_POINT('Ctrl Pts',(-0.558064364505217,-12.8369216984653,
-23.8071783097778));
#51943=CARTESIAN_POINT('Ctrl Pts',(-0.466922522056544,-12.8392027905172,
-23.8061270352528));
#51944=CARTESIAN_POINT('Ctrl Pts',(-0.376448954449454,-12.8408704269592,
-23.8053581701341));
#51945=CARTESIAN_POINT('Ctrl Pts',(-0.312801781035167,-12.8420435911068,
-23.8048172818633));
#51946=CARTESIAN_POINT('Ctrl Pts',(-0.249485494921159,-12.8429131418327,
-23.8044160904582));
#51947=CARTESIAN_POINT('Ctrl Pts',(-0.186500096427085,-12.8434883989062,
-23.8041502796551));
#51948=CARTESIAN_POINT('Ctrl Pts',(-0.155007397180047,-12.843776027443,
-23.8040173742536));
#51949=CARTESIAN_POINT('Ctrl Pts',(-0.123597419714937,-12.8439900795261,
-23.8039183136937));
#51950=CARTESIAN_POINT('Ctrl Pts',(-0.0922701636528899,-12.8441317019992,
-23.8038525594803));
#51951=CARTESIAN_POINT('Ctrl Pts',(-0.0647192958780385,-12.8442562523914,
-23.8037947317013));
#51952=CARTESIAN_POINT('Ctrl Pts',(-0.038338203916619,-12.8443236937568,
-23.8037631767086));
#51953=CARTESIAN_POINT('Ctrl Pts',(-0.0102093991919666,-12.8443378682957,
-23.8037560881866));
#51954=CARTESIAN_POINT('Ctrl Pts',(-0.0063537932791852,-12.844339811195,
-23.8037551165653));
#51955=CARTESIAN_POINT('Ctrl Pts',(-0.00246535106877531,-12.8443406806773,
-23.8037546373443));
#51956=CARTESIAN_POINT('Ctrl Pts',(0.00146344077723272,-12.8443404157055,
-23.8037546778085));
#51957=CARTESIAN_POINT('Ctrl Pts',(0.123997928659108,-12.8443321515412,
-23.8037559398407));
#51958=CARTESIAN_POINT('Ctrl Pts',(0.246529019799122,-12.8432200162837,
-23.8042792014033));
#51959=CARTESIAN_POINT('Ctrl Pts',(0.369061817155031,-12.8410040026569,
-23.8053128196795));
#51960=CARTESIAN_POINT('Ctrl Pts',(0.644876546147541,-12.8360158753058,
-23.8076394387636));
#51961=CARTESIAN_POINT('Ctrl Pts',(0.920699733133829,-12.825437781153,-23.8125503711935));
#51962=CARTESIAN_POINT('Ctrl Pts',(1.19652079061211,-12.8092724576358,-23.8200737229866));
#51963=CARTESIAN_POINT('Ctrl Pts',(1.22211852101468,-12.8077722255758,-23.8207719319365));
#51964=CARTESIAN_POINT('Ctrl Pts',(1.2477162348584,-12.8062238382288,-23.8214926578109));
#51965=CARTESIAN_POINT('Ctrl Pts',(1.27331392444618,-12.8046272774463,-23.8222359333602));
#51966=CARTESIAN_POINT('Ctrl Pts',(1.37082860577193,-12.7985451615041,-23.8250674497781));
#51967=CARTESIAN_POINT('Ctrl Pts',(1.46834293639484,-12.7917639892806,-23.8282261876786));
#51968=CARTESIAN_POINT('Ctrl Pts',(1.56585686947366,-12.7842847835651,-23.83171014081));
#51969=CARTESIAN_POINT('Ctrl Pts',(1.74018067037264,-12.7709143499577,-23.8379383374672));
#51970=CARTESIAN_POINT('Ctrl Pts',(1.91450485624828,-12.7553132735693,-23.8452071705032));
#51971=CARTESIAN_POINT('Ctrl Pts',(2.08882858929884,-12.7374808031892,-23.8535163666922));
#51972=CARTESIAN_POINT('Ctrl Pts',(2.17523695513979,-12.7286416474558,-23.8576350489368));
#51973=CARTESIAN_POINT('Ctrl Pts',(2.26164519251036,-12.7192541347995,-23.8620094030456));
#51974=CARTESIAN_POINT('Ctrl Pts',(2.34805359245555,-12.709318748311,-23.8666392626566));
#51975=CARTESIAN_POINT('Ctrl Pts',(2.47841969335505,-12.6943290297391,-23.8736244255063));
#51976=CARTESIAN_POINT('Ctrl Pts',(2.60878583338074,-12.6780923255439,-23.8811913884885));
#51977=CARTESIAN_POINT('Ctrl Pts',(2.7391519852192,-12.6606086884026,-23.8893399953968));
#51978=CARTESIAN_POINT('Ctrl Pts',(2.77254675020636,-12.656130056908,-23.8914273532641));
#51979=CARTESIAN_POINT('Ctrl Pts',(2.80594152189464,-12.651569593432,-23.8935528679851));
#51980=CARTESIAN_POINT('Ctrl Pts',(2.83933628185077,-12.6469272782789,-23.8957165518898));
#51981=CARTESIAN_POINT('Ctrl Pts',(2.87112458799384,-12.6425082815413,-23.8977761518525));
#51982=CARTESIAN_POINT('Ctrl Pts',(2.90291288348001,-12.6380151185757,-23.8998703371182));
#51983=CARTESIAN_POINT('Ctrl Pts',(2.93470118431995,-12.6334478148393,-23.9019990914454));
#51984=CARTESIAN_POINT('Ctrl Pts',(2.98358847573866,-12.6264237492911,-23.9052729069815));
#51985=CARTESIAN_POINT('Ctrl Pts',(3.03247576368835,-12.6192243319166,-23.9086285031247));
#51986=CARTESIAN_POINT('Ctrl Pts',(3.08136305406435,-12.6118496261618,-23.9120658770569));
#51987=CARTESIAN_POINT('Ctrl Pts',(3.09765881752302,-12.6093913909102,-23.9132116683676));
#51988=CARTESIAN_POINT('Ctrl Pts',(3.11203760771907,-12.607207438777,-23.9142296216478));
#51989=CARTESIAN_POINT('Ctrl Pts',(3.13025034526784,-12.6044164915618,-23.9155305099189));
#51990=CARTESIAN_POINT('Ctrl Pts',(3.25877318570469,-12.5847214587502,-23.9247105607072));
#51991=CARTESIAN_POINT('Ctrl Pts',(3.38587636788282,-12.5640249808262,-23.9344227860646));
#51992=CARTESIAN_POINT('Ctrl Pts',(3.51154612818603,-12.5424083497868,-23.9446281308574));
#51993=CARTESIAN_POINT('Ctrl Pts',(3.71380564173032,-12.5076174082911,-23.9610531488439));
#51994=CARTESIAN_POINT('Ctrl Pts',(3.91235133346752,-12.4704440589107,-23.9787552448699));
#51995=CARTESIAN_POINT('Ctrl Pts',(4.10714944138902,-12.4312193029833,-23.9975754628997));
#51996=CARTESIAN_POINT('Ctrl Pts',(4.29250029057756,-12.3938968572064,-24.0154829437831));
#51997=CARTESIAN_POINT('Ctrl Pts',(4.47445852096732,-12.3547170216527,-24.0344028076301));
#51998=CARTESIAN_POINT('Ctrl Pts',(4.65301431239387,-12.3139520128374,-24.0542053141028));
#51999=CARTESIAN_POINT('Ctrl Pts',(4.83065430931525,-12.2733960836087,-24.0739062555326));
#52000=CARTESIAN_POINT('Ctrl Pts',(5.00492682818613,-12.2312711675382,-24.0944809142273));
#52001=CARTESIAN_POINT('Ctrl Pts',(5.17583782751897,-12.1878310093366,-24.1158115156527));
#52002=CARTESIAN_POINT('Ctrl Pts',(5.35320999676605,-12.1427486265601,-24.1379485054366));
#52003=CARTESIAN_POINT('Ctrl Pts',(5.52696176320015,-12.0962497351854,-24.1608998542789));
#52004=CARTESIAN_POINT('Ctrl Pts',(5.69711466993369,-12.0485999934587,-24.1845484510568));
#52005=CARTESIAN_POINT('Ctrl Pts',(5.87744654476362,-11.9980997262243,-24.2096117654364));
#52006=CARTESIAN_POINT('Ctrl Pts',(6.05373611657599,-11.9463068999075,-24.2354586152215));
#52007=CARTESIAN_POINT('Ctrl Pts',(6.22602222360087,-11.8935144278621,-24.2619713031445));
#52008=CARTESIAN_POINT('Ctrl Pts',(6.2412447323608,-11.8888498969719,-24.2643138578121));
#52009=CARTESIAN_POINT('Ctrl Pts',(6.25643599311294,-11.8841775483418,-24.2666616081869));
#52010=CARTESIAN_POINT('Ctrl Pts',(6.27159604017512,-11.8794975712383,-24.269014496721));
#52011=CARTESIAN_POINT('Origin',(5.999999999061,-10.9277802195584,-24.1259421376201));
#52012=CARTESIAN_POINT('Origin',(5.99996968604348,-10.92775528448,-24.1259230378048));
#52013=CARTESIAN_POINT('Ctrl Pts',(6.2506839997157,-8.43293793822341,-13.9512886376407));
#52014=CARTESIAN_POINT('Ctrl Pts',(6.30609107903449,-8.4089443361267,-13.9477561522565));
#52015=CARTESIAN_POINT('Ctrl Pts',(6.42571412640754,-8.34736363641913,-13.9452436913382));
#52016=CARTESIAN_POINT('Ctrl Pts',(6.60616709762988,-8.21875062808475,-13.9600011874018));
#52017=CARTESIAN_POINT('Ctrl Pts',(6.78564627982441,-8.04020051785475,-14.0007025637708));
#52018=CARTESIAN_POINT('Ctrl Pts',(6.94040491966306,-7.81754299922649,-14.0706916391873));
#52019=CARTESIAN_POINT('Ctrl Pts',(7.04958588954151,-7.56911744843866,-14.1659910151057));
#52020=CARTESIAN_POINT('Ctrl Pts',(7.09856303838754,-7.34590570822213,-14.2646458549881));
#52021=CARTESIAN_POINT('Ctrl Pts',(7.10550422945416,-7.21206930956354,-14.3297283067357));
#52022=CARTESIAN_POINT('Ctrl Pts',(7.10486447840068,-7.1618629058329,-14.35501317323));
#52023=CARTESIAN_POINT('Ctrl Pts',(6.05255921110257,-8.02911577078493,-13.4884779979374));
#52024=CARTESIAN_POINT('Ctrl Pts',(6.10163826062474,-8.00808629630007,-13.4850681496603));
#52025=CARTESIAN_POINT('Ctrl Pts',(6.20784989591504,-7.95404975929016,-13.4820617786761));
#52026=CARTESIAN_POINT('Ctrl Pts',(6.36880447954209,-7.84082091740601,-13.4935329138248));
#52027=CARTESIAN_POINT('Ctrl Pts',(6.52960557358651,-7.68309717847588,-13.527681476833));
#52028=CARTESIAN_POINT('Ctrl Pts',(6.66878769581625,-7.48587125691864,-13.5878974252917));
#52029=CARTESIAN_POINT('Ctrl Pts',(6.76721838514569,-7.26552280866674,-13.6710447620323));
#52030=CARTESIAN_POINT('Ctrl Pts',(6.81137640333751,-7.06770393936238,-13.7578157172582));
#52031=CARTESIAN_POINT('Ctrl Pts',(6.81761281966829,-6.94946218721919,-13.8152192041817));
#52032=CARTESIAN_POINT('Ctrl Pts',(6.81703837246853,-6.90519492478787,-13.8375220044062));
#52033=CARTESIAN_POINT('Ctrl Pts',(6.04144506586559,-8.08851582223875,-12.8459991592576));
#52034=CARTESIAN_POINT('Ctrl Pts',(6.10905976426781,-8.05997102346696,-12.8415739201359));
#52035=CARTESIAN_POINT('Ctrl Pts',(6.25426772822431,-7.98718898283285,-12.8382171896667));
#52036=CARTESIAN_POINT('Ctrl Pts',(6.47106155741839,-7.83717256794907,-12.8550776491995));
#52037=CARTESIAN_POINT('Ctrl Pts',(6.68448599491058,-7.63141480041554,-12.9018927977333));
#52038=CARTESIAN_POINT('Ctrl Pts',(6.86688747126734,-7.37739371601871,-12.9818716205382));
#52039=CARTESIAN_POINT('Ctrl Pts',(6.99483563759271,-7.09583628609421,-13.0900818015455));
#52040=CARTESIAN_POINT('Ctrl Pts',(7.05222134159964,-6.84322738167346,-13.2018442365124));
#52041=CARTESIAN_POINT('Ctrl Pts',(7.06042125079301,-6.69113539618814,-13.2758159416857));
#52042=CARTESIAN_POINT('Ctrl Pts',(7.05966442080613,-6.63389340780036,-13.304642630965));
#52043=CARTESIAN_POINT('Ctrl Pts',(6.22476564159013,-8.57073749841051,-12.4584449885852));
#52044=CARTESIAN_POINT('Ctrl Pts',(6.3232318544767,-8.52928566176545,-12.4525535946661));
#52045=CARTESIAN_POINT('Ctrl Pts',(6.53344505259971,-8.42415889175985,-12.4492269301855));
#52046=CARTESIAN_POINT('Ctrl Pts',(6.84361485042466,-8.21008811643112,-12.4765033513155));
#52047=CARTESIAN_POINT('Ctrl Pts',(7.14534003904336,-7.91995501597388,-12.5466286666515));
#52048=CARTESIAN_POINT('Ctrl Pts',(7.40049874768094,-7.56536280118761,-12.6625262804813));
#52049=CARTESIAN_POINT('Ctrl Pts',(7.57824979202421,-7.17474961980343,-12.8160459785316));
#52050=CARTESIAN_POINT('Ctrl Pts',(7.65795529133822,-6.82426150287073,-12.9727554779674));
#52051=CARTESIAN_POINT('Ctrl Pts',(7.66945774630811,-6.61179150649196,-13.0763256360123));
#52052=CARTESIAN_POINT('Ctrl Pts',(7.66839431346161,-6.53144498495453,-13.1167654130957));
#52053=CARTESIAN_POINT('',(7.00000000000021,-6.97709949620137,-13.9487329104921));
#52054=CARTESIAN_POINT('',(6.99999983297877,-8.0445005512629,-12.5220497591224));
#52055=CARTESIAN_POINT('Ctrl Pts',(7.,-6.97709949620152,-13.9487329104919));
#52056=CARTESIAN_POINT('Ctrl Pts',(7.,-7.02099172054913,-13.8471553853057));
#52057=CARTESIAN_POINT('Ctrl Pts',(7.,-7.06243364082271,-13.7568553945143));
#52058=CARTESIAN_POINT('Ctrl Pts',(7.,-7.10051939710644,-13.6792399036818));
#52059=CARTESIAN_POINT('Ctrl Pts',(7.,-7.1195622752483,-13.6404321582655));
#52060=CARTESIAN_POINT('Ctrl Pts',(7.,-7.13772767823402,-13.6047694443452));
#52061=CARTESIAN_POINT('Ctrl Pts',(7.,-7.15473399319081,-13.572301993779));
#52062=CARTESIAN_POINT('Ctrl Pts',(7.,-7.1632371506692,-13.5560682684958));
#52063=CARTESIAN_POINT('Ctrl Pts',(7.,-7.17144937268595,-13.5406322757568));
#52064=CARTESIAN_POINT('Ctrl Pts',(7.,-7.17933119800859,-13.5259946169535));
#52065=CARTESIAN_POINT('Ctrl Pts',(7.,-7.18327211066991,-13.5186757875519));
#52066=CARTESIAN_POINT('Ctrl Pts',(7.,-7.1871304241577,-13.5115565416342));
#52067=CARTESIAN_POINT('Ctrl Pts',(7.,-7.19090112056253,-13.5046366132084));
#52068=CARTESIAN_POINT('Ctrl Pts',(7.,-7.19278646876494,-13.5011766489955));
#52069=CARTESIAN_POINT('Ctrl Pts',(7.,-7.19464991269662,-13.4977665141556));
#52070=CARTESIAN_POINT('Ctrl Pts',(7.,-7.19649083259167,-13.4944061694443));
#52071=CARTESIAN_POINT('Ctrl Pts',(7.,-7.19833175248671,-13.4910458247329));
#52072=CARTESIAN_POINT('Ctrl Pts',(7.,-7.19934688844232,-13.4891942737903));
#52073=CARTESIAN_POINT('Ctrl Pts',(7.,-7.20194540134434,-13.4844744618343));
#52074=CARTESIAN_POINT('Ctrl Pts',(7.,-7.2435216077767,-13.4089574705386));
#52075=CARTESIAN_POINT('Ctrl Pts',(7.,-7.28577339769281,-13.3377261163259));
#52076=CARTESIAN_POINT('Ctrl Pts',(7.,-7.32833005782022,-13.2712688299823));
#52077=CARTESIAN_POINT('Ctrl Pts',(7.,-7.37088671794763,-13.2048115436386));
#52078=CARTESIAN_POINT('Ctrl Pts',(7.,-7.41277533743944,-13.1444121047124));
#52079=CARTESIAN_POINT('Ctrl Pts',(7.,-7.45594679397945,-13.0864207383147));
#52080=CARTESIAN_POINT('Ctrl Pts',(7.,-7.54228970705945,-12.9704380055194));
#52081=CARTESIAN_POINT('Ctrl Pts',(7.,-7.63586349310065,-12.8624797720249));
#52082=CARTESIAN_POINT('Ctrl Pts',(7.,-7.73523562504603,-12.7671941670015));
#52083=CARTESIAN_POINT('Ctrl Pts',(7.,-7.83460775699141,-12.6719085619781));
#52084=CARTESIAN_POINT('Ctrl Pts',(7.,-7.93958121382532,-12.589452238568));
#52085=CARTESIAN_POINT('Ctrl Pts',(7.,-8.04450023478728,-12.5220492664956));
#52086=CARTESIAN_POINT('',(6.24988067607176,-8.55172528393766,-12.4626549972234));
#52087=CARTESIAN_POINT('Ctrl Pts',(6.24994482956932,-8.55169717381052,-12.4626517783794));
#52088=CARTESIAN_POINT('Ctrl Pts',(6.29048458262229,-8.53403513767215,-12.4605545886541));
#52089=CARTESIAN_POINT('Ctrl Pts',(6.33134363509387,-8.51493349436176,-12.4591623965491));
#52090=CARTESIAN_POINT('Ctrl Pts',(6.37251646586922,-8.49423690369723,-12.4585572396575));
#52091=CARTESIAN_POINT('Ctrl Pts',(6.41368929664456,-8.47354031303271,-12.457952082766));
#52092=CARTESIAN_POINT('Ctrl Pts',(6.45517658069543,-8.45124860872904,-12.4581338983597));
#52093=CARTESIAN_POINT('Ctrl Pts',(6.49692908775461,-8.42718486597987,-12.4592076157083));
#52094=CARTESIAN_POINT('Ctrl Pts',(6.50031160745528,-8.4252353762449,-12.4592946013851));
#52095=CARTESIAN_POINT('Ctrl Pts',(6.50369585137872,-8.42327429550722,-12.4593874157455));
#52096=CARTESIAN_POINT('Ctrl Pts',(6.50708174191544,-8.42130154727401,-12.459486119114));
#52097=CARTESIAN_POINT('Ctrl Pts',(6.54999952146535,-8.39629602129426,-12.4607372314472));
#52098=CARTESIAN_POINT('Ctrl Pts',(6.59318572013806,-8.3694158784028,-12.4629336731219));
#52099=CARTESIAN_POINT('Ctrl Pts',(6.63647569728123,-8.34051133705735,-12.4661941145981));
#52100=CARTESIAN_POINT('Ctrl Pts',(6.67408360229115,-8.31540069212261,-12.46902660335));
#52101=CARTESIAN_POINT('Ctrl Pts',(6.71176939123371,-8.28876205909622,-12.4726622916301));
#52102=CARTESIAN_POINT('Ctrl Pts',(6.74939368103051,-8.26049889249528,-12.4771850108168));
#52103=CARTESIAN_POINT('Ctrl Pts',(6.77237300104314,-8.24323694938883,-12.4799472958214));
#52104=CARTESIAN_POINT('Ctrl Pts',(6.7953286993857,-8.22536928626321,-12.4830404776204));
#52105=CARTESIAN_POINT('Ctrl Pts',(6.818232101135,-8.20686687586236,-12.4864861196393));
#52106=CARTESIAN_POINT('Ctrl Pts',(6.85639403896923,-8.1760379255069,-12.4922272919754));
#52107=CARTESIAN_POINT('Ctrl Pts',(6.89441333319197,-8.14344663938261,-12.4989465132712));
#52108=CARTESIAN_POINT('Ctrl Pts',(6.9321382534014,-8.10896156348281,-12.5067449032162));
#52109=CARTESIAN_POINT('Ctrl Pts',(6.9548806557229,-8.08817229565011,-12.511446148987));
#52110=CARTESIAN_POINT('Ctrl Pts',(6.97751518344798,-8.06669475313748,-12.5165397978753));
#52111=CARTESIAN_POINT('Ctrl Pts',(6.99999949893631,-8.04450053061514,-12.5220497269843));
#52112=CARTESIAN_POINT('',(6.26382947399266,-8.42073790614957,-13.9442724045435));
#52113=CARTESIAN_POINT('Origin',(6.527587443497,-9.09528625386695,-13.2547537415242));
#52114=CARTESIAN_POINT('Ctrl Pts',(6.26386081927195,-8.42073287768038,-13.9442638625882));
#52115=CARTESIAN_POINT('Ctrl Pts',(6.30364635770537,-8.39476059044689,-13.9340836131071));
#52116=CARTESIAN_POINT('Ctrl Pts',(6.34318219371725,-8.36594610635673,-13.9248487614566));
#52117=CARTESIAN_POINT('Ctrl Pts',(6.38210302545369,-8.33427173662188,-13.9166477645883));
#52118=CARTESIAN_POINT('Ctrl Pts',(6.42102385719013,-8.30259736688704,-13.9084467677199));
#52119=CARTESIAN_POINT('Ctrl Pts',(6.4593294825228,-8.26806279443629,-13.9012800888418));
#52120=CARTESIAN_POINT('Ctrl Pts',(6.49663260666941,-8.230695113355,-13.8952081854052));
#52121=CARTESIAN_POINT('Ctrl Pts',(6.51075077335915,-8.21655251370995,-13.8929101434368));
#52122=CARTESIAN_POINT('Ctrl Pts',(6.52472513260001,-8.2020045811677,-13.8907685937496));
#52123=CARTESIAN_POINT('Ctrl Pts',(6.53853398200339,-8.1870546194782,-13.8887855340391));
#52124=CARTESIAN_POINT('Ctrl Pts',(6.57276742070081,-8.14999225591147,-13.8838693421791));
#52125=CARTESIAN_POINT('Ctrl Pts',(6.60598682438523,-8.11045658124235,-13.8799312016209));
#52126=CARTESIAN_POINT('Ctrl Pts',(6.6378660093174,-8.06853116995194,-13.8770019875818));
#52127=CARTESIAN_POINT('Ctrl Pts',(6.64639311847277,-8.05731687575912,-13.8762184754592));
#52128=CARTESIAN_POINT('Ctrl Pts',(6.65482425905276,-8.04593181774124,-13.8755069788649));
#52129=CARTESIAN_POINT('Ctrl Pts',(6.66315302408082,-8.0343780801965,-13.8748676892266));
#52130=CARTESIAN_POINT('Ctrl Pts',(6.68288623746992,-8.00700398960277,-13.8733530302335));
#52131=CARTESIAN_POINT('Ctrl Pts',(6.70204494706761,-7.97868286949254,-13.872244398396));
#52132=CARTESIAN_POINT('Ctrl Pts',(6.72054559570175,-7.9494469599469,-13.8715439793987));
#52133=CARTESIAN_POINT('Ctrl Pts',(6.72979592001882,-7.93482900517408,-13.8711937699));
#52134=CARTESIAN_POINT('Ctrl Pts',(6.73888182638716,-7.91998235042525,-13.8709456115201));
#52135=CARTESIAN_POINT('Ctrl Pts',(6.74779278023998,-7.90491194370508,-13.8707996343));
#52136=CARTESIAN_POINT('Ctrl Pts',(6.75224825716639,-7.89737674034499,-13.8707266456899));
#52137=CARTESIAN_POINT('Ctrl Pts',(6.75665999697761,-7.88978560334353,-13.8706791978952));
#52138=CARTESIAN_POINT('Ctrl Pts',(6.7610266857108,-7.88213918461823,-13.8706572814865));
#52139=CARTESIAN_POINT('Ctrl Pts',(6.76400979685793,-7.87691552011436,-13.8706423092532));
#52140=CARTESIAN_POINT('Ctrl Pts',(6.767263976232,-7.87114466561447,-13.8706383101171));
#52141=CARTESIAN_POINT('Ctrl Pts',(6.77018874126757,-7.86589465086422,-13.8706483529515));
#52142=CARTESIAN_POINT('Ctrl Pts',(6.77154525771907,-7.86345967530456,-13.870653010854));
#52143=CARTESIAN_POINT('Ctrl Pts',(6.77283150170764,-7.86113705674444,-13.8706602095793));
#52144=CARTESIAN_POINT('Ctrl Pts',(6.77399028875956,-7.85903475791193,-13.8706681031229));
#52145=CARTESIAN_POINT('Ctrl Pts',(6.79031634658572,-7.82941563828974,-13.8707793146253));
#52146=CARTESIAN_POINT('Ctrl Pts',(6.80638197979347,-7.79820326450054,-13.8712236235775));
#52147=CARTESIAN_POINT('Ctrl Pts',(6.8219998728032,-7.76535612977931,-13.8720923025352));
#52148=CARTESIAN_POINT('Ctrl Pts',(6.83722489386632,-7.73333527282491,-13.8729391296597));
#52149=CARTESIAN_POINT('Ctrl Pts',(6.85202408371635,-7.69976039894808,-13.8741898593545));
#52150=CARTESIAN_POINT('Ctrl Pts',(6.86618710318874,-7.66461800682303,-13.8759100776536));
#52151=CARTESIAN_POINT('Ctrl Pts',(6.87985159490252,-7.63071260078081,-13.8775697455472));
#52152=CARTESIAN_POINT('Ctrl Pts',(6.89292332203614,-7.59534777689527,-13.8796669331209));
#52153=CARTESIAN_POINT('Ctrl Pts',(6.90518551397339,-7.55854047945062,-13.8822346286123));
#52154=CARTESIAN_POINT('Ctrl Pts',(6.9139051923643,-7.53236670906778,-13.8840605239339));
#52155=CARTESIAN_POINT('Ctrl Pts',(6.92221488481856,-7.50546412122659,-13.8861238258106));
#52156=CARTESIAN_POINT('Ctrl Pts',(6.93003048544214,-7.47784944293239,-13.8884258882348));
#52157=CARTESIAN_POINT('Ctrl Pts',(6.94050147980807,-7.44085252423582,-13.89151008916));
#52158=CARTESIAN_POINT('Ctrl Pts',(6.95007987425218,-7.40257560652634,-13.8949948880792));
#52159=CARTESIAN_POINT('Ctrl Pts',(6.95858300270777,-7.36306946515618,-13.8989690474034));
#52160=CARTESIAN_POINT('Ctrl Pts',(6.96639277933585,-7.32678468583649,-13.9026191506294));
#52161=CARTESIAN_POINT('Ctrl Pts',(6.97329457265961,-7.28946289945377,-13.9066823481282));
#52162=CARTESIAN_POINT('Ctrl Pts',(6.97912057043595,-7.25117104072324,-13.9111965112778));
#52163=CARTESIAN_POINT('Ctrl Pts',(6.98481751717041,-7.21372738078283,-13.9156106816914));
#52164=CARTESIAN_POINT('Ctrl Pts',(6.98948502380683,-7.17535595748036,-13.9204564887435));
#52165=CARTESIAN_POINT('Ctrl Pts',(6.99295170328696,-7.13614918333898,-13.9257329552367));
#52166=CARTESIAN_POINT('Ctrl Pts',(6.99632248551628,-7.09802696918501,-13.9308634611258));
#52167=CARTESIAN_POINT('Ctrl Pts',(6.99855707282768,-7.05911499469893,-13.9364013240573));
#52168=CARTESIAN_POINT('Ctrl Pts',(6.99949624089758,-7.01952796744627,-13.942306371551));
#52169=CARTESIAN_POINT('Ctrl Pts',(6.99982980142646,-7.00546800291992,-13.9444036434113));
#52170=CARTESIAN_POINT('Ctrl Pts',(7.00000000252704,-6.99132316217677,-13.9465468520234));
#52171=CARTESIAN_POINT('Ctrl Pts',(7.00000000000032,-6.97709949620138,-13.9487329104922));
#52172=CARTESIAN_POINT('Ctrl Pts',(6.99990204209712,-6.87914456964441,-13.8881650018953));
#52173=CARTESIAN_POINT('Ctrl Pts',(6.99990204209712,-7.13651843302261,-14.0922367193011));
#52174=CARTESIAN_POINT('Ctrl Pts',(6.99990204209712,-7.80837710098112,-14.676030897134));
#52175=CARTESIAN_POINT('Ctrl Pts',(6.99990204209712,-8.78348255721519,-15.7555643069836));
#52176=CARTESIAN_POINT('Ctrl Pts',(6.99990204209712,-9.70999001325044,-17.1681336842782));
#52177=CARTESIAN_POINT('Ctrl Pts',(6.99990204209712,-10.4111885651775,-18.7078378782952));
#52178=CARTESIAN_POINT('Ctrl Pts',(6.99990204209712,-10.8675485943344,-20.3372599925577));
#52179=CARTESIAN_POINT('Ctrl Pts',(6.99990204209712,-11.0696762981163,-22.0150948612855));
#52180=CARTESIAN_POINT('Ctrl Pts',(6.99990204209712,-11.0250216793473,-23.3220419082231));
#52181=CARTESIAN_POINT('Ctrl Pts',(6.99990204209712,-10.9251645215214,-24.0577229990154));
#52182=CARTESIAN_POINT('Ctrl Pts',(6.99990204209712,-10.8963439108589,-24.2367456800396));
#52183=CARTESIAN_POINT('Ctrl Pts',(7.00657867940667,-7.1754747309625,-13.5144113065886));
#52184=CARTESIAN_POINT('Ctrl Pts',(7.00657867940667,-7.44407566709084,-13.7273830362199));
#52185=CARTESIAN_POINT('Ctrl Pts',(7.00657867940667,-8.14504949431156,-14.3364946131352));
#52186=CARTESIAN_POINT('Ctrl Pts',(7.00657867940667,-9.16238026129488,-15.4627618448717));
#52187=CARTESIAN_POINT('Ctrl Pts',(7.00657867940667,-10.1293833823756,-16.9370083185477));
#52188=CARTESIAN_POINT('Ctrl Pts',(7.00657867940667,-10.8609672539439,-18.5435648618307));
#52189=CARTESIAN_POINT('Ctrl Pts',(7.00657867940667,-11.3371716152691,-20.2436461281815));
#52190=CARTESIAN_POINT('Ctrl Pts',(7.00657867940667,-11.5480935350588,-21.9947648368347));
#52191=CARTESIAN_POINT('Ctrl Pts',(7.00657867940667,-11.5014977799429,-23.3582205168238));
#52192=CARTESIAN_POINT('Ctrl Pts',(7.00657867940667,-11.3973240256672,-24.1257634459938));
#52193=CARTESIAN_POINT('Ctrl Pts',(7.00657867940667,-11.3672534070212,-24.3125554713659));
#52194=CARTESIAN_POINT('Ctrl Pts',(6.71861277733521,-7.41191640291053,-13.2161934396482));
#52195=CARTESIAN_POINT('Ctrl Pts',(6.71861277733521,-7.68947541419458,-13.43626648412));
#52196=CARTESIAN_POINT('Ctrl Pts',(6.71861277733521,-8.41368021089695,-14.0655787997737));
#52197=CARTESIAN_POINT('Ctrl Pts',(6.71861277733521,-9.4647025299881,-15.2291349221608));
#52198=CARTESIAN_POINT('Ctrl Pts',(6.71861277733521,-10.4640171198348,-16.7525935169619));
#52199=CARTESIAN_POINT('Ctrl Pts',(6.71861277733521,-11.2198454211492,-18.4124915127807));
#52200=CARTESIAN_POINT('Ctrl Pts',(6.71861277733521,-11.7118835641508,-20.1689516775356));
#52201=CARTESIAN_POINT('Ctrl Pts',(6.71861277733521,-11.9298223840338,-21.978543521564));
#52202=CARTESIAN_POINT('Ctrl Pts',(6.71861277733521,-11.8816777972994,-23.3870874086374));
#52203=CARTESIAN_POINT('Ctrl Pts',(6.71861277733521,-11.7740598330902,-24.1800528810343));
#52204=CARTESIAN_POINT('Ctrl Pts',(6.71861277733521,-11.7429918337667,-24.3730440619698));
#52205=CARTESIAN_POINT('Ctrl Pts',(6.25720741184697,-7.48821447986154,-13.1199606158348));
#52206=CARTESIAN_POINT('Ctrl Pts',(6.25720741184697,-7.76866419946435,-13.3423252050321));
#52207=CARTESIAN_POINT('Ctrl Pts',(6.25720741184697,-8.50036546784203,-13.9781561580555));
#52208=CARTESIAN_POINT('Ctrl Pts',(6.25720741184697,-9.56225981559318,-15.1537451451436));
#52209=CARTESIAN_POINT('Ctrl Pts',(6.25720741184697,-10.5720010908474,-16.6930841478832));
#52210=CARTESIAN_POINT('Ctrl Pts',(6.25720741184697,-11.3356529003941,-18.3701950580588));
#52211=CARTESIAN_POINT('Ctrl Pts',(6.25720741184697,-11.8328004942073,-20.1448482997505));
#52212=CARTESIAN_POINT('Ctrl Pts',(6.25720741184697,-12.0530036187637,-21.973309016367));
#52213=CARTESIAN_POINT('Ctrl Pts',(6.25720741184697,-12.0043592348795,-23.3964025531034));
#52214=CARTESIAN_POINT('Ctrl Pts',(6.25720741184697,-11.8956298481708,-24.1975717027368));
#52215=CARTESIAN_POINT('Ctrl Pts',(6.25720741184697,-11.8642400010606,-24.392563307896));
#52216=CARTESIAN_POINT('Ctrl Pts',(7.00000000000032,-6.9770994962013,-13.9487329104922));
#52217=CARTESIAN_POINT('Ctrl Pts',(7.00000000000032,-7.10629915106168,-14.0533893975594));
#52218=CARTESIAN_POINT('Ctrl Pts',(6.99999999999072,-7.23274383645403,-14.1606500554492));
#52219=CARTESIAN_POINT('Ctrl Pts',(6.99999999940502,-7.35653276712002,-14.2705333166525));
#52220=CARTESIAN_POINT('Ctrl Pts',(6.99999999896232,-7.45009804601583,-14.353588060927));
#52221=CARTESIAN_POINT('Ctrl Pts',(6.99999999822524,-7.54214550930935,-14.4381420517995));
#52222=CARTESIAN_POINT('Ctrl Pts',(6.99999999797672,-7.63270518127864,-14.5242182514032));
#52223=CARTESIAN_POINT('Ctrl Pts',(6.99999999764697,-7.75286173493317,-14.6384260358524));
#52224=CARTESIAN_POINT('Ctrl Pts',(6.99999999919547,-7.8704006665934,-14.7553125453204));
#52225=CARTESIAN_POINT('Ctrl Pts',(6.99999999987686,-7.98538150041516,-14.874987097388));
#52226=CARTESIAN_POINT('Ctrl Pts',(6.99999999995253,-7.99815034808622,-14.8882771916991));
#52227=CARTESIAN_POINT('Ctrl Pts',(7.00000000000035,-8.01088760691926,-14.9016017031286));
#52228=CARTESIAN_POINT('Ctrl Pts',(7.00000000000035,-8.02359332727153,-14.9149608060427));
#52229=CARTESIAN_POINT('Ctrl Pts',(7.00000000000035,-8.16375185897403,-15.0623268897741));
#52230=CARTESIAN_POINT('Ctrl Pts',(6.99999999555914,-8.30011589105752,-15.2138319381572));
#52231=CARTESIAN_POINT('Ctrl Pts',(6.99999999493194,-8.43226901989482,-15.3691238080779));
#52232=CARTESIAN_POINT('Ctrl Pts',(6.99999999439975,-8.54440376184542,-15.500892264215));
#52233=CARTESIAN_POINT('Ctrl Pts',(6.99999999610764,-8.65350711581379,-15.6353863891432));
#52234=CARTESIAN_POINT('Ctrl Pts',(6.99999999794456,-8.75934547301326,-15.7723701876197));
#52235=CARTESIAN_POINT('Ctrl Pts',(6.99999999900022,-8.82017040022465,-15.8510942890886));
#52236=CARTESIAN_POINT('Ctrl Pts',(7.00000000000035,-8.87991734635779,-15.9306403281046));
#52237=CARTESIAN_POINT('Ctrl Pts',(7.00000000000035,-8.93855257173526,-16.0109543539319));
#52238=CARTESIAN_POINT('Ctrl Pts',(7.00000000000035,-9.09298167451233,-16.222479471625));
#52239=CARTESIAN_POINT('Ctrl Pts',(6.99999999747293,-9.23963260823544,-16.4393930418639));
#52240=CARTESIAN_POINT('Ctrl Pts',(6.99999999839252,-9.37832622087594,-16.6612166909058));
#52241=CARTESIAN_POINT('Ctrl Pts',(6.99999999909985,-9.48500722655949,-16.8318400492108));
#52242=CARTESIAN_POINT('Ctrl Pts',(6.99999999994394,-9.586979807279,-17.0053694008068));
#52243=CARTESIAN_POINT('Ctrl Pts',(6.9999999999955,-9.68414867194944,-17.1816028684607));
#52244=CARTESIAN_POINT('Ctrl Pts',(6.99999999999884,-9.69044102029951,-17.1930151904342));
#52245=CARTESIAN_POINT('Ctrl Pts',(7.00000000000035,-9.69671321993812,-17.2044388563421));
#52246=CARTESIAN_POINT('Ctrl Pts',(7.00000000000035,-9.70296524696087,-17.2158738099789));
#52247=CARTESIAN_POINT('Ctrl Pts',(7.00000000000035,-9.87477532000824,-17.5301143294911));
#52248=CARTESIAN_POINT('Ctrl Pts',(7.00000000000863,-10.0313678420663,-17.8528586248414));
#52249=CARTESIAN_POINT('Ctrl Pts',(6.99999999997898,-10.1718235720896,-18.1825334426912));
#52250=CARTESIAN_POINT('Ctrl Pts',(6.99999999996923,-10.2180173474565,-18.2909585277864));
#52251=CARTESIAN_POINT('Ctrl Pts',(7.00000000000035,-10.2624658168571,-18.4001328570506));
#52252=CARTESIAN_POINT('Ctrl Pts',(7.00000000000035,-10.3051367476958,-18.5099993257218));
#52253=CARTESIAN_POINT('Ctrl Pts',(7.00000000000035,-10.3319482521631,-18.5790319260819));
#52254=CARTESIAN_POINT('Ctrl Pts',(6.99999999997254,-10.3580605209726,-18.6483371267314));
#52255=CARTESIAN_POINT('Ctrl Pts',(6.99999999993318,-10.3834664693262,-18.717900541163));
#52256=CARTESIAN_POINT('Ctrl Pts',(6.99999999971942,-10.5214370739838,-19.0956745261202));
#52257=CARTESIAN_POINT('Ctrl Pts',(7.00000000000035,-10.6385722836543,-19.481064067169));
#52258=CARTESIAN_POINT('Ctrl Pts',(7.00000000000035,-10.7343171771693,-19.8715547121628));
#52259=CARTESIAN_POINT('Ctrl Pts',(7.00000000000035,-10.7726966551624,-20.0280834477003));
#52260=CARTESIAN_POINT('Ctrl Pts',(6.999999999624,-10.8076376867947,-20.1854325756873));
#52261=CARTESIAN_POINT('Ctrl Pts',(6.99999999912793,-10.8391038800975,-20.3434795187503));
#52262=CARTESIAN_POINT('Ctrl Pts',(6.99999999825573,-10.8944274489208,-20.621356186185));
#52263=CARTESIAN_POINT('Ctrl Pts',(6.99999999886898,-10.9390123595612,-20.901390595644));
#52264=CARTESIAN_POINT('Ctrl Pts',(6.99999999982073,-10.9726762049677,-21.1829159345384));
#52265=CARTESIAN_POINT('Ctrl Pts',(6.99999999992676,-10.9764265412553,-21.2142793952952));
#52266=CARTESIAN_POINT('Ctrl Pts',(7.00000000000035,-10.9800412819873,-21.2456613499309));
#52267=CARTESIAN_POINT('Ctrl Pts',(7.00000000000035,-10.9835201357179,-21.2770608676747));
#52268=CARTESIAN_POINT('Ctrl Pts',(7.00000000000035,-11.0078795682481,-21.4969247921714));
#52269=CARTESIAN_POINT('Ctrl Pts',(6.99999999634688,-11.0256228522879,-21.7176517758152));
#52270=CARTESIAN_POINT('Ctrl Pts',(6.99999999542235,-11.0366757131641,-21.9386334390376));
#52271=CARTESIAN_POINT('Ctrl Pts',(6.99999999531207,-11.0379941427253,-21.9649930178432));
#52272=CARTESIAN_POINT('Ctrl Pts',(6.99999999523666,-11.0392174373876,-21.991356219691));
#52273=CARTESIAN_POINT('Ctrl Pts',(6.99999999520114,-11.0403455207274,-22.0177220124615));
#52274=CARTESIAN_POINT('Ctrl Pts',(6.99999999489308,-11.050129574066,-22.2463968928441));
#52275=CARTESIAN_POINT('Ctrl Pts',(7.00000000000035,-11.0527466392745,-22.4752660514269));
#52276=CARTESIAN_POINT('Ctrl Pts',(7.00000000000035,-11.0482983184102,-22.7036608217722));
#52277=CARTESIAN_POINT('Ctrl Pts',(7.00000000000035,-11.044983466985,-22.8738586903776));
#52278=CARTESIAN_POINT('Ctrl Pts',(6.99999999741464,-11.0376888388909,-23.0437848171676));
#52279=CARTESIAN_POINT('Ctrl Pts',(6.99999999745767,-11.0264497943418,-23.2135396730414));
#52280=CARTESIAN_POINT('Ctrl Pts',(6.99999999749874,-11.0157217260455,-23.3755767287237));
#52281=CARTESIAN_POINT('Ctrl Pts',(6.99999999865165,-11.0013993941378,-23.5374580702059));
#52282=CARTESIAN_POINT('Ctrl Pts',(6.99999999924098,-10.9834692586181,-23.699270698839));
#52283=CARTESIAN_POINT('Ctrl Pts',(6.9999999997591,-10.9677053432543,-23.8415340174717));
#52284=CARTESIAN_POINT('Ctrl Pts',(6.99999999990897,-10.9491520894197,-23.9837444084844));
#52285=CARTESIAN_POINT('Ctrl Pts',(6.99999999989431,-10.9277733094969,-24.1259362010628));
#52286=CARTESIAN_POINT('Ctrl Pts',(6.26386085547009,-8.4207418582818,-13.9442726607693));
#52287=CARTESIAN_POINT('Ctrl Pts',(6.264607194611,-8.60590534760794,-14.1256751686954));
#52288=CARTESIAN_POINT('Ctrl Pts',(6.26531572513606,-8.78359556684554,-14.3114975773241));
#52289=CARTESIAN_POINT('Ctrl Pts',(6.26598642940395,-8.95375584024701,-14.5010992765559));
#52290=CARTESIAN_POINT('Ctrl Pts',(6.26666478024275,-9.12585607834021,-14.6928625884524));
#52291=CARTESIAN_POINT('Ctrl Pts',(6.26730443743229,-9.29025374785374,-14.8884918847937));
#52292=CARTESIAN_POINT('Ctrl Pts',(6.26790538606772,-9.44692290708507,-15.0873663300705));
#52293=CARTESIAN_POINT('Ctrl Pts',(6.26800179595848,-9.4720572623971,-15.1192716584363));
#52294=CARTESIAN_POINT('Ctrl Pts',(6.26809720958945,-9.49699277082847,-15.1512605953605));
#52295=CARTESIAN_POINT('Ctrl Pts',(6.26819162690635,-9.52172940099684,-15.1833306754945));
#52296=CARTESIAN_POINT('Ctrl Pts',(6.26876871801906,-9.67292295210862,-15.37934724149));
#52297=CARTESIAN_POINT('Ctrl Pts',(6.2693085884704,-9.81668511809778,-15.5783911664421));
#52298=CARTESIAN_POINT('Ctrl Pts',(6.26981122734859,-9.95309248242574,-15.7798081313912));
#52299=CARTESIAN_POINT('Ctrl Pts',(6.27017912980239,-10.0529347473803,-15.9272336467207));
#52300=CARTESIAN_POINT('Ctrl Pts',(6.27052708590838,-10.1488372020054,-16.0759315329076));
#52301=CARTESIAN_POINT('Ctrl Pts',(6.27085509217591,-10.2408366896114,-16.2256615039805));
#52302=CARTESIAN_POINT('Ctrl Pts',(6.27121137691842,-10.3407677488555,-16.3883001772955));
#52303=CARTESIAN_POINT('Ctrl Pts',(6.27154412300116,-10.4360937721226,-16.5521563516628));
#52304=CARTESIAN_POINT('Ctrl Pts',(6.27185332634397,-10.5268692976001,-16.7169398447424));
#52305=CARTESIAN_POINT('Ctrl Pts',(6.27227096778314,-10.6494799419672,-16.9395131668055));
#52306=CARTESIAN_POINT('Ctrl Pts',(6.2726456578957,-10.7637883511822,-17.1637762381474));
#52307=CARTESIAN_POINT('Ctrl Pts',(6.27297738874874,-10.869998798733,-17.3890720441409));
#52308=CARTESIAN_POINT('Ctrl Pts',(6.27330911960178,-10.9762092462838,-17.6143678501343));
#52309=CARTESIAN_POINT('Ctrl Pts',(6.27359789121449,-11.0743218171509,-17.8406965676868));
#52310=CARTESIAN_POINT('Ctrl Pts',(6.27384369779657,-11.1645575170758,-18.0674572453059));
#52311=CARTESIAN_POINT('Ctrl Pts',(6.27395596405333,-11.2057705072685,-18.171024742323));
#52312=CARTESIAN_POINT('Ctrl Pts',(6.27405926792789,-11.2453406153195,-18.2746831003251));
#52313=CARTESIAN_POINT('Ctrl Pts',(6.27415361604604,-11.2832899881317,-18.3783788192582));
#52314=CARTESIAN_POINT('Ctrl Pts',(6.27415652027611,-11.2844581482576,-18.381570787797));
#52315=CARTESIAN_POINT('Ctrl Pts',(6.27415941595948,-11.2856247726996,-18.384762791782));
#52316=CARTESIAN_POINT('Ctrl Pts',(6.27416230310198,-11.2867898621169,-18.3879548296995));
#52317=CARTESIAN_POINT('Ctrl Pts',(6.27420631246129,-11.3045495808973,-18.4366117781816));
#52318=CARTESIAN_POINT('Ctrl Pts',(6.27424833729733,-11.3219526271923,-18.4852766012743));
#52319=CARTESIAN_POINT('Ctrl Pts',(6.27428839822284,-11.3390022188445,-18.533943700428));
#52320=CARTESIAN_POINT('Ctrl Pts',(6.2743178500858,-11.3515366830508,-18.5697226225751));
#52321=CARTESIAN_POINT('Ctrl Pts',(6.27434670121203,-11.3640964164529,-18.6061334871817));
#52322=CARTESIAN_POINT('Ctrl Pts',(6.27437398744428,-11.3762332615428,-18.6418692456922));
#52323=CARTESIAN_POINT('Ctrl Pts',(6.27438625127513,-11.3816881815887,-18.6579307265802));
#52324=CARTESIAN_POINT('Ctrl Pts',(6.27439819898716,-11.387058352707,-18.673855597911));
#52325=CARTESIAN_POINT('Ctrl Pts',(6.27440974304166,-11.3923063239685,-18.6895241035388));
#52326=CARTESIAN_POINT('Ctrl Pts',(6.27456064715992,-11.4609079124125,-18.8943431318955));
#52327=CARTESIAN_POINT('Ctrl Pts',(6.27467736520998,-11.5248693955755,-19.1037511979344));
#52328=CARTESIAN_POINT('Ctrl Pts',(6.27475989545213,-11.5836609481629,-19.3175727645897));
#52329=CARTESIAN_POINT('Ctrl Pts',(6.27484107220331,-11.6414883228561,-19.5278876705287));
#52330=CARTESIAN_POINT('Ctrl Pts',(6.27488917331302,-11.6943139378734,-19.7424725854378));
#52331=CARTESIAN_POINT('Ctrl Pts',(6.27490419809794,-11.741610311925,-19.9611156276329));
#52332=CARTESIAN_POINT('Ctrl Pts',(6.27490863211128,-11.7555680993114,-20.025640089765));
#52333=CARTESIAN_POINT('Ctrl Pts',(6.2749101854529,-11.769044178975,-20.0905176757685));
#52334=CARTESIAN_POINT('Ctrl Pts',(6.2749088581209,-11.7820245987158,-20.155742159142));
#52335=CARTESIAN_POINT('Ctrl Pts',(6.27490450942711,-11.8245519171822,-20.369434969669));
#52336=CARTESIAN_POINT('Ctrl Pts',(6.27486923973871,-11.8617601976141,-20.5868549744431));
#52337=CARTESIAN_POINT('Ctrl Pts',(6.2748030495234,-11.8931694348145,-20.8077262448279));
#52338=CARTESIAN_POINT('Ctrl Pts',(6.27475277095458,-11.9170281197666,-20.9755016677541));
#52339=CARTESIAN_POINT('Ctrl Pts',(6.27468465115883,-11.9375403794305,-21.1452675639377));
#52340=CARTESIAN_POINT('Ctrl Pts',(6.27459869066247,-11.9544887837,-21.3168841110458));
#52341=CARTESIAN_POINT('Ctrl Pts',(6.27448994645919,-11.9759293383426,-21.5339873791369));
#52342=CARTESIAN_POINT('Ctrl Pts',(6.27435264982169,-11.9916670083741,-21.7540538870482));
#52343=CARTESIAN_POINT('Ctrl Pts',(6.27418680323014,-12.0012473071029,-21.9767610896342));
#52344=CARTESIAN_POINT('Ctrl Pts',(6.27401315364896,-12.0112783535429,-22.2099465418742));
#52345=CARTESIAN_POINT('Ctrl Pts',(6.27380820438329,-12.0145579268997,-22.4460271421446));
#52346=CARTESIAN_POINT('Ctrl Pts',(6.27357195921121,-12.0106606948055,-22.6846229983359));
#52347=CARTESIAN_POINT('Ctrl Pts',(6.2733393070839,-12.0068227355811,-22.9195900582934));
#52348=CARTESIAN_POINT('Ctrl Pts',(6.27307630376345,-11.9960245832477,-23.1569965027566));
#52349=CARTESIAN_POINT('Ctrl Pts',(6.27278295384919,-11.9778555569011,-23.3964293197048));
#52350=CARTESIAN_POINT('Ctrl Pts',(6.27261682316355,-11.9675660266934,-23.5320255346988));
#52351=CARTESIAN_POINT('Ctrl Pts',(6.2724409596977,-11.9549124215193,-23.6682707312012));
#52352=CARTESIAN_POINT('Ctrl Pts',(6.27225536444075,-11.9398195551922,-23.8050824682305));
#52353=CARTESIAN_POINT('Ctrl Pts',(6.27204648914279,-11.9228335233136,-23.9590551117422));
#52354=CARTESIAN_POINT('Ctrl Pts',(6.27182528752745,-11.9027579548588,-24.1137456145766));
#52355=CARTESIAN_POINT('Ctrl Pts',(6.27159176118789,-11.8794807211417,-24.2690119676562));
#52356=CARTESIAN_POINT('Ctrl Pts',(-6.390310997295,-8.1390337018704,-13.724647000479));
#52357=CARTESIAN_POINT('Ctrl Pts',(-4.26020733153,-9.11395737648274,-13.8218516500125));
#52358=CARTESIAN_POINT('Ctrl Pts',(0.0001535201484502,-10.0899905443268,
-13.9179732725499));
#52359=CARTESIAN_POINT('Ctrl Pts',(4.260514371827,-9.11388703213361,-13.8218447223658));
#52360=CARTESIAN_POINT('Ctrl Pts',(6.39077155774,-8.13882290112087,-13.7246259826053));
#52361=CARTESIAN_POINT('Ctrl Pts',(-6.390310997295,-8.71288713243719,-14.2540934475748));
#52362=CARTESIAN_POINT('Ctrl Pts',(-4.26020733153,-9.62694691866724,-14.3565346513067));
#52363=CARTESIAN_POINT('Ctrl Pts',(0.0001535201484502,-10.5423893454478,
-14.457603967021));
#52364=CARTESIAN_POINT('Ctrl Pts',(4.260514371827,-9.62688094118782,-14.3565273670688));
#52365=CARTESIAN_POINT('Ctrl Pts',(6.39077155774,-8.71268949185425,-14.2540712974373));
#52366=CARTESIAN_POINT('Ctrl Pts',(-6.390310997295,-9.96965830570771,-15.6639820761747));
#52367=CARTESIAN_POINT('Ctrl Pts',(-4.26020733153,-10.7489237306763,-15.7525575365657));
#52368=CARTESIAN_POINT('Ctrl Pts',(0.0001535201484502,-11.5272448903699,
-15.8420463049841));
#52369=CARTESIAN_POINT('Ctrl Pts',(4.260514371827,-10.7488676357646,-15.7525510869549));
#52370=CARTESIAN_POINT('Ctrl Pts',(6.39077155774,-9.96948981072532,-15.663962924145));
#52371=CARTESIAN_POINT('Ctrl Pts',(-6.390310997295,-11.3879809584937,-18.3168609125011));
#52372=CARTESIAN_POINT('Ctrl Pts',(-4.26020733153,-12.0191857141868,-18.3050659003902));
#52373=CARTESIAN_POINT('Ctrl Pts',(0.0001535201484502,-12.6510838649568,
-18.2929947853426));
#52374=CARTESIAN_POINT('Ctrl Pts',(4.260514371827,-12.019140172221,-18.3050667703783));
#52375=CARTESIAN_POINT('Ctrl Pts',(6.39077155774,-11.3878444776174,-18.3168634628551));
#52376=CARTESIAN_POINT('Ctrl Pts',(-6.390310997295,-12.0713625046932,-21.4528944523568));
#52377=CARTESIAN_POINT('Ctrl Pts',(-4.26020733153,-12.6592431520397,-21.2792418550437));
#52378=CARTESIAN_POINT('Ctrl Pts',(0.0001535201484502,-13.2456895514566,
-21.1056367718251));
#52379=CARTESIAN_POINT('Ctrl Pts',(4.260514371827,-12.6592008858621,-21.2792543670473));
#52380=CARTESIAN_POINT('Ctrl Pts',(6.39077155774,-12.0712353914676,-21.4529320000167));
#52381=CARTESIAN_POINT('Ctrl Pts',(-6.390310997295,-11.972049918498,-23.5459013792421));
#52382=CARTESIAN_POINT('Ctrl Pts',(-4.26020733153,-12.6077624045725,-23.2652611808828));
#52383=CARTESIAN_POINT('Ctrl Pts',(0.0001535201484502,-13.2461450674405,
-22.9846436057981));
#52384=CARTESIAN_POINT('Ctrl Pts',(4.260514371827,-12.6077163952593,-23.2652814054656));
#52385=CARTESIAN_POINT('Ctrl Pts',(6.39077155774,-11.9719124629745,-23.545962060063));
#52386=CARTESIAN_POINT('Ctrl Pts',(-6.390310997295,-11.8061921255752,-24.5118553802274));
#52387=CARTESIAN_POINT('Ctrl Pts',(-4.26020733153,-12.4817967099141,-24.1870632940561));
#52388=CARTESIAN_POINT('Ctrl Pts',(0.0001535201484502,-13.1582598604799,
-23.8622686316189));
#52389=CARTESIAN_POINT('Ctrl Pts',(4.260514371827,-12.4817479560743,-24.1870867025552));
#52390=CARTESIAN_POINT('Ctrl Pts',(6.39077155774,-11.8060460444555,-24.5119256076905));
#52391=CARTESIAN_POINT('Ctrl Pts',(-6.26383832463082,-8.42072097704164,
-13.9442592301454));
#52392=CARTESIAN_POINT('Ctrl Pts',(-5.97538166530715,-8.54511327803086,
-13.9555611456819));
#52393=CARTESIAN_POINT('Ctrl Pts',(-5.68507720580592,-8.66086372588226,
-13.9652304145446));
#52394=CARTESIAN_POINT('Ctrl Pts',(-5.39341281594673,-8.76784094219661,
-13.9735236289449));
#52395=CARTESIAN_POINT('Ctrl Pts',(-5.11950005635845,-8.86830718200011,
-13.9813120917165));
#52396=CARTESIAN_POINT('Ctrl Pts',(-4.8443878682284,-8.96103497709053,-13.9878870849323));
#52397=CARTESIAN_POINT('Ctrl Pts',(-4.56848035310862,-9.04595730735802,
-13.9934724196174));
#52398=CARTESIAN_POINT('Ctrl Pts',(-4.31195848006228,-9.12491287772086,
-13.9986653209937));
#52399=CARTESIAN_POINT('Ctrl Pts',(-4.05474911530607,-9.19712104882665,
-14.00300287132));
#52400=CARTESIAN_POINT('Ctrl Pts',(-3.79717702676898,-9.26257108423024,
-14.0066729478108));
#52401=CARTESIAN_POINT('Ctrl Pts',(-3.5773823659106,-9.3184217333297,-14.0098047437371));
#52402=CARTESIAN_POINT('Ctrl Pts',(-3.35732357810741,-9.36935171683099,
-14.0124506324332));
#52403=CARTESIAN_POINT('Ctrl Pts',(-3.13720246660799,-9.41538425106597,
-14.0147316531077));
#52404=CARTESIAN_POINT('Ctrl Pts',(-2.89762459074644,-9.46548565523124,
-14.0172142958869));
#52405=CARTESIAN_POINT('Ctrl Pts',(-2.65797161578867,-9.50979849671482,
-14.019280061851));
#52406=CARTESIAN_POINT('Ctrl Pts',(-2.41848996164712,-9.54830494866256,
-14.0209850915276));
#52407=CARTESIAN_POINT('Ctrl Pts',(-2.18234700883573,-9.58627456808007,
-14.0226663507619));
#52408=CARTESIAN_POINT('Ctrl Pts',(-1.94637063324644,-9.61859853128913,
-14.0239968819857));
#52409=CARTESIAN_POINT('Ctrl Pts',(-1.71079709151736,-9.64531020662259,
-14.0250352679962));
#52410=CARTESIAN_POINT('Ctrl Pts',(-1.47670514184955,-9.67185388428608,
-14.0260671232884));
#52411=CARTESIAN_POINT('Ctrl Pts',(-1.24301097489225,-9.69285557808708,
-14.0268105104645));
#52412=CARTESIAN_POINT('Ctrl Pts',(-1.0099464175956,-9.70839908468116,-14.0273274013437));
#52413=CARTESIAN_POINT('Ctrl Pts',(-0.778428527975858,-9.72383944114588,
-14.0278408620214));
#52414=CARTESIAN_POINT('Ctrl Pts',(-0.54753191928796,-9.73389378123307,
-14.0281308355323));
#52415=CARTESIAN_POINT('Ctrl Pts',(-0.317483833678931,-9.73869552910469,
-14.0282623090293));
#52416=CARTESIAN_POINT('Ctrl Pts',(-0.211730793665827,-9.74090289124577,
-14.0283227473587));
#52417=CARTESIAN_POINT('Ctrl Pts',(-0.106157066799982,-9.74200097364583,
-14.0283497487973));
#52418=CARTESIAN_POINT('Ctrl Pts',(-0.000784728634572568,-9.74200642998883,
-14.0283499195312));
#52419=CARTESIAN_POINT('Ctrl Pts',(-0.000523153662346578,-9.74200644353359,
-14.028349919955));
#52420=CARTESIAN_POINT('Ctrl Pts',(-0.000261577451239455,-9.74200645034681,
-14.0283499202138));
#52421=CARTESIAN_POINT('Ctrl Pts',(-1.58450436742064E-12,-9.74200645042823,
-14.0283499203075));
#52422=CARTESIAN_POINT('Ctrl Pts',(0.229838637557164,-9.74200652196735,
-14.0283500025861));
#52423=CARTESIAN_POINT('Ctrl Pts',(0.460633496507224,-9.73680495785485,
-14.0282222464573));
#52424=CARTESIAN_POINT('Ctrl Pts',(0.692159238285023,-9.72624319253679,
-14.0278992860365));
#52425=CARTESIAN_POINT('Ctrl Pts',(0.925512241714882,-9.71559807100703,
-14.0275737767278));
#52426=CARTESIAN_POINT('Ctrl Pts',(1.15960771013407,-9.69950781444332,-14.0270499565804));
#52427=CARTESIAN_POINT('Ctrl Pts',(1.39421492746824,-9.67786301061442,-14.0262631113473));
#52428=CARTESIAN_POINT('Ctrl Pts',(1.63029378402774,-9.65608243371467,-14.0254713304079));
#52429=CARTESIAN_POINT('Ctrl Pts',(1.86689082981409,-9.6286774638351,-14.0244132003187));
#52430=CARTESIAN_POINT('Ctrl Pts',(2.10377097976868,-9.59558948956167,-14.0230272818018));
#52431=CARTESIAN_POINT('Ctrl Pts',(2.34348947075129,-9.56210504916419,-14.0216247569571));
#52432=CARTESIAN_POINT('Ctrl Pts',(2.58349789095941,-9.52280064216678,-14.0198865221185));
#52433=CARTESIAN_POINT('Ctrl Pts',(2.82355260317888,-9.47766881045565,-14.017753756889));
#52434=CARTESIAN_POINT('Ctrl Pts',(2.92765742358338,-9.45809643384462,-14.0168288379857));
#52435=CARTESIAN_POINT('Ctrl Pts',(3.03177095016019,-9.43742875781944,-14.0158297824754));
#52436=CARTESIAN_POINT('Ctrl Pts',(3.13587331164792,-9.41566819115963,-14.0147520852401));
#52437=CARTESIAN_POINT('Ctrl Pts',(3.39867956582585,-9.36073367352787,-14.0120314401991));
#52438=CARTESIAN_POINT('Ctrl Pts',(3.66140879823393,-9.29881450311919,-14.0087907922733));
#52439=CARTESIAN_POINT('Ctrl Pts',(3.92371691757782,-9.2298741376027,-14.004824436216));
#52440=CARTESIAN_POINT('Ctrl Pts',(4.19327232811746,-9.15902902394007,-14.0007484940071));
#52441=CARTESIAN_POINT('Ctrl Pts',(4.4623830343311,-9.08076995842586,-13.9959061304099));
#52442=CARTESIAN_POINT('Ctrl Pts',(4.73067562905621,-8.99511737496303,-13.9900830109841));
#52443=CARTESIAN_POINT('Ctrl Pts',(5.02417182687565,-8.90141852499846,-13.9837128634492));
#52444=CARTESIAN_POINT('Ctrl Pts',(5.31668898549974,-8.79887209713146,-13.9761688159281));
#52445=CARTESIAN_POINT('Ctrl Pts',(5.60773826797885,-8.68756970498058,-13.9671831253586));
#52446=CARTESIAN_POINT('Ctrl Pts',(5.82734099413855,-8.60358973933271,-13.9604032352703));
#52447=CARTESIAN_POINT('Ctrl Pts',(6.04610805609104,-8.51462651729644,-13.9528028757534));
#52448=CARTESIAN_POINT('Ctrl Pts',(6.26382947399266,-8.42073790614957,-13.9442724045435));
#52449=CARTESIAN_POINT('Ctrl Pts',(-6.38263471220914,-8.36841944701316,
-13.9389824198947));
#52450=CARTESIAN_POINT('Ctrl Pts',(-6.32602239780459,-8.394139193293,-13.9420683564949));
#52451=CARTESIAN_POINT('Ctrl Pts',(-5.68511490691572,-8.68097899639166,
-13.976093651889));
#52452=CARTESIAN_POINT('Ctrl Pts',(-4.3452434520593,-9.18098161005785,-14.0268456230749));
#52453=CARTESIAN_POINT('Ctrl Pts',(-2.26201825060707,-9.6636131923873,-14.0637937745164));
#52454=CARTESIAN_POINT('Ctrl Pts',(-0.00125756887690166,-9.84171456782906,
-14.0745454197917));
#52455=CARTESIAN_POINT('Ctrl Pts',(2.25978796677181,-9.66398535327025,-14.0638181801999));
#52456=CARTESIAN_POINT('Ctrl Pts',(4.34366867832048,-9.18148899332632,-14.026891442955));
#52457=CARTESIAN_POINT('Ctrl Pts',(5.68433680181859,-8.68130836760525,-13.9761309988622));
#52458=CARTESIAN_POINT('Ctrl Pts',(6.32575507084932,-8.39426070532174,-13.942082936579));
#52459=CARTESIAN_POINT('Ctrl Pts',(6.38264695375981,-8.36841389164203,-13.938981748398));
#52460=CARTESIAN_POINT('Ctrl Pts',(-6.17942050080956,-7.96893940221161,
-13.4711461915673));
#52461=CARTESIAN_POINT('Ctrl Pts',(-6.12458159000237,-7.99369183810001,
-13.4742878091345));
#52462=CARTESIAN_POINT('Ctrl Pts',(-5.50375880491641,-8.2697463021422,-13.5089464493689));
#52463=CARTESIAN_POINT('Ctrl Pts',(-4.20607327283165,-8.75099127862432,
-13.5610724671584));
#52464=CARTESIAN_POINT('Ctrl Pts',(-2.18922025325704,-9.21546154338672,
-13.5997349748739));
#52465=CARTESIAN_POINT('Ctrl Pts',(-0.00121700010307547,-9.38682514547008,
-13.6112156728877));
#52466=CARTESIAN_POINT('Ctrl Pts',(2.18706140901595,-9.21581965563337,-13.5997608378893));
#52467=CARTESIAN_POINT('Ctrl Pts',(4.20454828183471,-8.75147962203571,-13.5611198620646));
#52468=CARTESIAN_POINT('Ctrl Pts',(5.5030051176246,-8.2700633023372,-13.5089845778398));
#52469=CARTESIAN_POINT('Ctrl Pts',(6.12432263701548,-7.99380877974493,-13.4743026523511));
#52470=CARTESIAN_POINT('Ctrl Pts',(6.17943235891975,-7.96893405529369,-13.4711455083109));
#52471=CARTESIAN_POINT('Ctrl Pts',(-6.17609323028145,-8.03335433234395,
-12.8276174364743));
#52472=CARTESIAN_POINT('Ctrl Pts',(-6.12140911242363,-8.05780395121941,
-12.8307280019944));
#52473=CARTESIAN_POINT('Ctrl Pts',(-5.50230415439753,-8.33050515234243,
-12.8650456140325));
#52474=CARTESIAN_POINT('Ctrl Pts',(-4.20735980031929,-8.80645453110351,
-12.916693548388));
#52475=CARTESIAN_POINT('Ctrl Pts',(-2.19139790985851,-9.26683779944148,
-12.955028315275));
#52476=CARTESIAN_POINT('Ctrl Pts',(-0.00121862788615356,-9.43699416114887,
-12.9664097316442));
#52477=CARTESIAN_POINT('Ctrl Pts',(2.18923837210851,-9.26719317059794,-12.9550539597772));
#52478=CARTESIAN_POINT('Ctrl Pts',(4.20583716474793,-8.80693793478961,-12.916740528662));
#52479=CARTESIAN_POINT('Ctrl Pts',(5.50155240772465,-8.33081840437701,-12.8650833759042));
#52480=CARTESIAN_POINT('Ctrl Pts',(6.12115089105302,-8.05791946224448,-12.8307426976662));
#52481=CARTESIAN_POINT('Ctrl Pts',(6.17610505478834,-8.03334905141697,-12.8276167590171));
#52482=CARTESIAN_POINT('Ctrl Pts',(-6.37328423761647,-8.51437156949978,
-12.4447843264679));
#52483=CARTESIAN_POINT('Ctrl Pts',(-6.31704477490063,-8.53938216381777,
-12.4477987971532));
#52484=CARTESIAN_POINT('Ctrl Pts',(-5.68027830641508,-8.81836853175587,
-12.4810393968647));
#52485=CARTESIAN_POINT('Ctrl Pts',(-4.34709680890174,-9.30595474822533,
-12.5306952467038));
#52486=CARTESIAN_POINT('Ctrl Pts',(-2.26647258115335,-9.7789738787803,-12.5668982241231));
#52487=CARTESIAN_POINT('Ctrl Pts',(-0.0012610105169752,-9.954224760735,
-12.5774258330699));
#52488=CARTESIAN_POINT('Ctrl Pts',(2.26424126928097,-9.7793395776048,-12.566922135523));
#52489=CARTESIAN_POINT('Ctrl Pts',(4.34552789319493,-9.30645053700893,-12.5307401190399));
#52490=CARTESIAN_POINT('Ctrl Pts',(5.67950489339072,-8.81868912212491,-12.4810759011191));
#52491=CARTESIAN_POINT('Ctrl Pts',(6.31677921013562,-8.53950032554409,-12.4478130376531));
#52492=CARTESIAN_POINT('Ctrl Pts',(6.37329639823823,-8.51436616865024,-12.4447836683068));
#52493=CARTESIAN_POINT('Ctrl Pts',(-6.24991282163701,-8.55170697043111,
-12.4626563115405));
#52494=CARTESIAN_POINT('Ctrl Pts',(-5.9951518486516,-8.66268534979844,-12.4758442934149));
#52495=CARTESIAN_POINT('Ctrl Pts',(-5.73646706502544,-8.76784866932984,
-12.4876291065261));
#52496=CARTESIAN_POINT('Ctrl Pts',(-5.47399786209961,-8.86673420580976,
-12.4981941489829));
#52497=CARTESIAN_POINT('Ctrl Pts',(-5.27446010051969,-8.94191025839756,
-12.5062260433892));
#52498=CARTESIAN_POINT('Ctrl Pts',(-5.07273572700998,-9.01345851273478,
-12.5135524815385));
#52499=CARTESIAN_POINT('Ctrl Pts',(-4.86889821251265,-9.0811859245181,-12.5202415502398));
#52500=CARTESIAN_POINT('Ctrl Pts',(-4.63291108368157,-9.1595954238162,-12.527985630721));
#52501=CARTESIAN_POINT('Ctrl Pts',(-4.3940912290919,-9.23288409034135,-12.5348755534569));
#52502=CARTESIAN_POINT('Ctrl Pts',(-4.15257087682656,-9.30077330239881,
-12.5409921785991));
#52503=CARTESIAN_POINT('Ctrl Pts',(-4.03181070069389,-9.33471790842754,
-12.5440504911702));
#52504=CARTESIAN_POINT('Ctrl Pts',(-3.91037570869951,-9.36731298118346,
-12.5469150648855));
#52505=CARTESIAN_POINT('Ctrl Pts',(-3.78828430791232,-9.39852576868662,
-12.5495933701623));
#52506=CARTESIAN_POINT('Ctrl Pts',(-3.72723860751873,-9.41413216243819,
-12.5509325228007));
#52507=CARTESIAN_POINT('Ctrl Pts',(-3.66602880391475,-9.42939298126246,
-12.5522251035111));
#52508=CARTESIAN_POINT('Ctrl Pts',(-3.60465734051059,-9.44430429742624,
-12.553471843025));
#52509=CARTESIAN_POINT('Ctrl Pts',(-3.57397160880851,-9.45175995550813,
-12.554095212782));
#52510=CARTESIAN_POINT('Ctrl Pts',(-3.54324546208646,-9.45912823768745,
-12.5547071219219));
#52511=CARTESIAN_POINT('Ctrl Pts',(-3.51247920955523,-9.46640865724988,
-12.5553076546463));
#52512=CARTESIAN_POINT('Ctrl Pts',(-3.49709608328961,-9.4700488670311,-12.5556079210085));
#52513=CARTESIAN_POINT('Ctrl Pts',(-3.48170293056752,-9.47366711114212,
-12.5559053432456));
#52514=CARTESIAN_POINT('Ctrl Pts',(-3.46629979054523,-9.47726332934056,
-12.5561999311267));
#52515=CARTESIAN_POINT('Ctrl Pts',(-3.45089665052293,-9.480859547539,-12.5564945190078));
#52516=CARTESIAN_POINT('Ctrl Pts',(-3.43752301160335,-9.4839640228018,-12.5567480657857));
#52517=CARTESIAN_POINT('Ctrl Pts',(-3.42006044787704,-9.48798584610345,
-12.557075201193));
#52518=CARTESIAN_POINT('Ctrl Pts',(-3.16496428844448,-9.54673733839557,
-12.5618540519572));
#52519=CARTESIAN_POINT('Ctrl Pts',(-2.9083995259039,-9.5990949307777,-12.5658854025021));
#52520=CARTESIAN_POINT('Ctrl Pts',(-2.65057545024978,-9.64488223466745,
-12.5693035076391));
#52521=CARTESIAN_POINT('Ctrl Pts',(-2.39508555341555,-9.69025500878651,
-12.5726906673782));
#52522=CARTESIAN_POINT('Ctrl Pts',(-2.13835912217894,-9.72917596851338,
-12.5754757356453));
#52523=CARTESIAN_POINT('Ctrl Pts',(-1.8806090149955,-9.76150571997245,-12.5777508730779));
#52524=CARTESIAN_POINT('Ctrl Pts',(-1.70382302984741,-9.78368009275444,
-12.5793113473558));
#52525=CARTESIAN_POINT('Ctrl Pts',(-1.5265556646053,-9.80275440615707,-12.5806311333328));
#52526=CARTESIAN_POINT('Ctrl Pts',(-1.34887783893452,-9.81869245723344,
-12.5817290231167));
#52527=CARTESIAN_POINT('Ctrl Pts',(-1.09250470695069,-9.84168963235498,
-12.5833131793917));
#52528=CARTESIAN_POINT('Ctrl Pts',(-0.835276744086408,-9.85815719512418,
-12.5844360222734));
#52529=CARTESIAN_POINT('Ctrl Pts',(-0.577412891913281,-9.86802180172397,
-12.5851131549729));
#52530=CARTESIAN_POINT('Ctrl Pts',(-0.385525226552946,-9.87536248291747,
-12.5856170387541));
#52531=CARTESIAN_POINT('Ctrl Pts',(-0.193285590508025,-9.87904741916114,
-12.5858732856714));
#52532=CARTESIAN_POINT('Ctrl Pts',(-0.00078636143307452,-9.87905785432159,
-12.5858736475182));
#52533=CARTESIAN_POINT('Ctrl Pts',(0.257720844642301,-9.8790718676981,-12.5858741334423));
#52534=CARTESIAN_POINT('Ctrl Pts',(0.515777038007509,-9.87245589781863,
-12.5854163540354));
#52535=CARTESIAN_POINT('Ctrl Pts',(0.773154488727125,-9.85925949667269,
-12.5845132529827));
#52536=CARTESIAN_POINT('Ctrl Pts',(1.03174709470167,-9.84600079140433,-12.5836058881221));
#52537=CARTESIAN_POINT('Ctrl Pts',(1.28965444445947,-9.82609939635818,-12.5822489670534));
#52538=CARTESIAN_POINT('Ctrl Pts',(1.54665177143313,-9.79963821643248,-12.5804148452328));
#52539=CARTESIAN_POINT('Ctrl Pts',(1.60560439865932,-9.79356828529937,-12.5799941159542));
#52540=CARTESIAN_POINT('Ctrl Pts',(1.66450916949929,-9.7871533139504,-12.579548108785));
#52541=CARTESIAN_POINT('Ctrl Pts',(1.72336342415286,-9.78039454216238,-12.5790761922448));
#52542=CARTESIAN_POINT('Ctrl Pts',(1.98197035651968,-9.75069634533781,-12.5770025802428));
#52543=CARTESIAN_POINT('Ctrl Pts',(2.23960128133811,-9.71435892567672,-12.574430876114));
#52544=CARTESIAN_POINT('Ctrl Pts',(2.49603560817474,-9.67151459029893,-12.5712774729064));
#52545=CARTESIAN_POINT('Ctrl Pts',(2.52259643111958,-9.66707688174331,-12.5709508513292));
#52546=CARTESIAN_POINT('Ctrl Pts',(2.54914442427194,-9.66256939409518,-12.5706179541918));
#52547=CARTESIAN_POINT('Ctrl Pts',(2.57567934791689,-9.65799229447821,-12.5702786645519));
#52548=CARTESIAN_POINT('Ctrl Pts',(2.71703894936703,-9.63360869397081,-12.56847116554));
#52549=CARTESIAN_POINT('Ctrl Pts',(2.85802756534812,-9.60724934697013,-12.5664824530093));
#52550=CARTESIAN_POINT('Ctrl Pts',(2.99860947845435,-9.57894193118977,-12.5642922890289));
#52551=CARTESIAN_POINT('Ctrl Pts',(3.06890043500747,-9.5647882232996,-12.5631972070388));
#52552=CARTESIAN_POINT('Ctrl Pts',(3.1390897140937,-9.55014749051982,-12.5620517520799));
#52553=CARTESIAN_POINT('Ctrl Pts',(3.20917295407369,-9.53502358563055,-12.5608529863025));
#52554=CARTESIAN_POINT('Ctrl Pts',(3.24421457406368,-9.52746163318592,-12.5602536034138));
#52555=CARTESIAN_POINT('Ctrl Pts',(3.27922968418995,-9.51977888728932,-12.559640892266));
#52556=CARTESIAN_POINT('Ctrl Pts',(3.31421774203385,-9.51197583874081,-12.5590144729994));
#52557=CARTESIAN_POINT('Ctrl Pts',(3.33171177095581,-9.50807431446657,-12.5587012633661));
#52558=CARTESIAN_POINT('Ctrl Pts',(3.34919903680103,-9.50414271450498,-12.558384626671));
#52559=CARTESIAN_POINT('Ctrl Pts',(3.36667947214295,-9.50018110159169,-12.5580645140084));
#52560=CARTESIAN_POINT('Ctrl Pts',(3.38415990748487,-9.49621948867839,-12.5577444013458));
#52561=CARTESIAN_POINT('Ctrl Pts',(3.40367174990795,-9.49175857405086,-12.5573826410032));
#52562=CARTESIAN_POINT('Ctrl Pts',(3.41910021933437,-9.48820628709549,-12.5570936987225));
#52563=CARTESIAN_POINT('Ctrl Pts',(3.68468645188544,-9.42705709054576,-12.5521198358181));
#52564=CARTESIAN_POINT('Ctrl Pts',(3.94732104507969,-9.35935398742538,-12.5463133571322));
#52565=CARTESIAN_POINT('Ctrl Pts',(4.20681520902679,-9.28542097652985,-12.5396050120407));
#52566=CARTESIAN_POINT('Ctrl Pts',(4.47313973337084,-9.20954191373872,-12.5327200910528));
#52567=CARTESIAN_POINT('Ctrl Pts',(4.7361562409857,-9.12710073431103,-12.5248850533555));
#52568=CARTESIAN_POINT('Ctrl Pts',(4.99568992142244,-9.03847547006321,-12.5159872135925));
#52569=CARTESIAN_POINT('Ctrl Pts',(5.13446019343343,-8.99108835635211,-12.5112296205042));
#52570=CARTESIAN_POINT('Ctrl Pts',(5.27223524686326,-8.9419337085792,-12.506167554481));
#52571=CARTESIAN_POINT('Ctrl Pts',(5.40899176766102,-8.89107233748081,-12.5007797956799));
#52572=CARTESIAN_POINT('Ctrl Pts',(5.67488604643662,-8.79218310348412,-12.4903044323681));
#52573=CARTESIAN_POINT('Ctrl Pts',(5.93692802123922,-8.68684255488974,-12.478598163806));
#52574=CARTESIAN_POINT('Ctrl Pts',(6.194971318514,-8.57552812461383,-12.4654727479179));
#52575=CARTESIAN_POINT('Ctrl Pts',(6.21329458554215,-8.56762385408414,-12.4645407318465));
#52576=CARTESIAN_POINT('Ctrl Pts',(6.23159770394303,-8.55968947309391,-12.4636015474238));
#52577=CARTESIAN_POINT('Ctrl Pts',(6.24988062747952,-8.55172515761025,-12.4626551215893));
#52578=CARTESIAN_POINT('Ctrl Pts',(7.10864015812303,-14.3702857527608,-7.14961345992433));
#52579=CARTESIAN_POINT('Ctrl Pts',(7.10873195145162,-14.3685405421865,-7.15305333563911));
#52580=CARTESIAN_POINT('Ctrl Pts',(7.11056295294098,-14.3266947300623,-7.23573122197125));
#52581=CARTESIAN_POINT('Ctrl Pts',(7.09575328823177,-14.2427614361485,-7.41145149599964));
#52582=CARTESIAN_POINT('Ctrl Pts',(7.015653292201,-14.1296722279313,-7.67994912051664));
#52583=CARTESIAN_POINT('Ctrl Pts',(6.86753480235506,-14.0345787862568,-7.94877408540477));
#52584=CARTESIAN_POINT('Ctrl Pts',(6.65756610531993,-13.97131600051,-8.18823799362193));
#52585=CARTESIAN_POINT('Ctrl Pts',(6.43827730135439,-13.9506144748102,-8.34979252916423));
#52586=CARTESIAN_POINT('Ctrl Pts',(6.29372111382291,-13.954903661422,-8.42179428876983));
#52587=CARTESIAN_POINT('Ctrl Pts',(6.24006895947315,-13.9586807624534,-8.44434194376808));
#52588=CARTESIAN_POINT('Ctrl Pts',(6.8141141961259,-13.8514991507047,-6.8948240391595));
#52589=CARTESIAN_POINT('Ctrl Pts',(6.81419627684994,-13.8499675766328,-6.89784015081079));
#52590=CARTESIAN_POINT('Ctrl Pts',(6.81583363961584,-13.8132441297087,-6.97034394335527));
#52591=CARTESIAN_POINT('Ctrl Pts',(6.80258372349459,-13.7395910455641,-7.12497917479021));
#52592=CARTESIAN_POINT('Ctrl Pts',(6.73069216203656,-13.6408694233877,-7.36194197355014));
#52593=CARTESIAN_POINT('Ctrl Pts',(6.59792593852943,-13.5588146206345,-7.59913721838558));
#52594=CARTESIAN_POINT('Ctrl Pts',(6.41046234837585,-13.5054525382864,-7.80983934257711));
#52595=CARTESIAN_POINT('Ctrl Pts',(6.21582986261128,-13.4892779790566,-7.95132463382177));
#52596=CARTESIAN_POINT('Ctrl Pts',(6.08830244526732,-13.4939767162925,-8.01411538505492));
#52597=CARTESIAN_POINT('Ctrl Pts',(6.04108479443307,-13.4975659796289,-8.03375561024937));
#52598=CARTESIAN_POINT('Ctrl Pts',(7.05418145102173,-13.3159705186763,-6.61710193690136));
#52599=CARTESIAN_POINT('Ctrl Pts',(7.0542892633488,-13.3139898936888,-6.62100630655558));
#52600=CARTESIAN_POINT('Ctrl Pts',(7.05643951679178,-13.2665094508432,-6.71482650170777));
#52601=CARTESIAN_POINT('Ctrl Pts',(7.03906592225061,-13.1717458506828,-6.91317869534412));
#52602=CARTESIAN_POINT('Ctrl Pts',(6.94574282526344,-13.0442863141664,-7.21546230643042));
#52603=CARTESIAN_POINT('Ctrl Pts',(6.77268167770971,-12.9366350636699,-7.51934219641006));
#52604=CARTESIAN_POINT('Ctrl Pts',(6.52525483088428,-12.8644440066539,-7.79272044859093));
#52605=CARTESIAN_POINT('Ctrl Pts',(6.26358458306018,-12.8408370822447,-7.97995451406243));
#52606=CARTESIAN_POINT('Ctrl Pts',(6.08889668952107,-12.8463947505128,-8.06469804500965));
#52607=CARTESIAN_POINT('Ctrl Pts',(6.02373779604539,-12.8510945065208,-8.09140233501099));
#52608=CARTESIAN_POINT('Ctrl Pts',(7.66687013380095,-13.1298707134944,-6.50628245672557));
#52609=CARTESIAN_POINT('Ctrl Pts',(7.66702167078277,-13.1270827140161,-6.5117850556935));
#52610=CARTESIAN_POINT('Ctrl Pts',(7.67004350237204,-13.0602569178355,-6.64396416362557));
#52611=CARTESIAN_POINT('Ctrl Pts',(7.64565946499919,-12.9272996711648,-6.92120542958822));
#52612=CARTESIAN_POINT('Ctrl Pts',(7.51579922451643,-12.7474722240711,-7.34139335357857));
#52613=CARTESIAN_POINT('Ctrl Pts',(7.27412336431642,-12.5929349937385,-7.76507343272806));
#52614=CARTESIAN_POINT('Ctrl Pts',(6.92493246816672,-12.4859435512758,-8.15007988493282));
#52615=CARTESIAN_POINT('Ctrl Pts',(6.54999801644743,-12.4479784492041,-8.4178655165686));
#52616=CARTESIAN_POINT('Ctrl Pts',(6.29594779154568,-12.4542588737833,-8.54084107185101));
#52617=CARTESIAN_POINT('Ctrl Pts',(6.20064104132926,-12.4606133626168,-8.57979107217853));
#52618=CARTESIAN_POINT('',(6.26385988969939,-13.9442649557967,-8.42071839556295));
#52619=CARTESIAN_POINT('',(6.24994527954487,-12.4626513729877,-8.55169284846167));
#52620=CARTESIAN_POINT('Ctrl Pts',(6.26385592204643,-13.9442753243737,-8.42070825250184));
#52621=CARTESIAN_POINT('Ctrl Pts',(6.25433094938681,-13.9218720248115,-8.4015324156922));
#52622=CARTESIAN_POINT('Ctrl Pts',(6.24498622483379,-13.8980075092444,-8.38293048695047));
#52623=CARTESIAN_POINT('Ctrl Pts',(6.23592366206991,-13.8726980683743,-8.36513067103791));
#52624=CARTESIAN_POINT('Ctrl Pts',(6.22708766500422,-13.8480213680756,-8.34777585372286));
#52625=CARTESIAN_POINT('Ctrl Pts',(6.21852019074842,-13.8219708232343,-8.3311842415144));
#52626=CARTESIAN_POINT('Ctrl Pts',(6.21032173905935,-13.7946096914538,-8.31557592497331));
#52627=CARTESIAN_POINT('Ctrl Pts',(6.20224970289332,-13.7676704529668,-8.30020827991192));
#52628=CARTESIAN_POINT('Ctrl Pts',(6.19453572189864,-13.7394606139546,-8.28579459549095));
#52629=CARTESIAN_POINT('Ctrl Pts',(6.18727710741677,-13.7100907636814,-8.27254267655098));
#52630=CARTESIAN_POINT('Ctrl Pts',(6.18014608857456,-13.6812371916651,-8.25952370662328));
#52631=CARTESIAN_POINT('Ctrl Pts',(6.1734549049804,-13.6512641756783,-8.24762677146337));
#52632=CARTESIAN_POINT('Ctrl Pts',(6.16729227922977,-13.6203252002813,-8.23703555362394));
#52633=CARTESIAN_POINT('Ctrl Pts',(6.16649544171368,-13.6163247405255,-8.23566609195988));
#52634=CARTESIAN_POINT('Ctrl Pts',(6.16570743204194,-13.612308196355,-8.23431843270015));
#52635=CARTESIAN_POINT('Ctrl Pts',(6.16492843297263,-13.608275957326,-8.23299294604334));
#52636=CARTESIAN_POINT('Ctrl Pts',(6.15899612350256,-13.5775692585389,-8.22289897115123));
#52637=CARTESIAN_POINT('Ctrl Pts',(6.15358731359049,-13.5459490871413,-8.21409328094374));
#52638=CARTESIAN_POINT('Ctrl Pts',(6.14877659384877,-13.5136112831753,-8.20672369077255));
#52639=CARTESIAN_POINT('Ctrl Pts',(6.14402750491138,-13.4816877633448,-8.19944851345313));
#52640=CARTESIAN_POINT('Ctrl Pts',(6.13986155259341,-13.4490654654329,-8.19357343054227));
#52641=CARTESIAN_POINT('Ctrl Pts',(6.13633723326726,-13.4159680839301,-8.1892066760389));
#52642=CARTESIAN_POINT('Ctrl Pts',(6.13283360983156,-13.383065060463,-8.18486556446525));
#52643=CARTESIAN_POINT('Ctrl Pts',(6.1299643255585,-13.3496932358894,-8.18201553851788));
#52644=CARTESIAN_POINT('Ctrl Pts',(6.12776995560997,-13.316097801226,-8.18072180153648));
#52645=CARTESIAN_POINT('Ctrl Pts',(6.1255830317919,-13.282616365567,-8.179432454578));
#52646=CARTESIAN_POINT('Ctrl Pts',(6.12406658849042,-13.2489136651176,-8.17968907655454));
#52647=CARTESIAN_POINT('Ctrl Pts',(6.12324125283879,-13.2152460979091,-8.18151036836834));
#52648=CARTESIAN_POINT('Ctrl Pts',(6.12241666034082,-13.1816088458528,-8.18333002024368));
#52649=CARTESIAN_POINT('Ctrl Pts',(6.12228197612596,-13.1480075395908,-8.18671153080457));
#52650=CARTESIAN_POINT('Ctrl Pts',(6.122836841893,-13.1146987316703,-8.19162595594638));
#52651=CARTESIAN_POINT('Ctrl Pts',(6.1233944112646,-13.0812276253159,-8.19656432681168));
#52652=CARTESIAN_POINT('Ctrl Pts',(6.12464822342135,-13.0480527410839,-8.20305039378025));
#52653=CARTESIAN_POINT('Ctrl Pts',(6.12657672595882,-13.0154220523358,-8.21100805179854));
#52654=CARTESIAN_POINT('Ctrl Pts',(6.12851268953151,-12.9826651212245,-8.21899649658821));
#52655=CARTESIAN_POINT('Ctrl Pts',(6.13112842257139,-12.9504573700935,-8.22846751325802));
#52656=CARTESIAN_POINT('Ctrl Pts',(6.13438230274582,-12.9190248592522,-8.2393018492621));
#52657=CARTESIAN_POINT('Ctrl Pts',(6.13767357069664,-12.8872311821651,-8.25026067409498));
#52658=CARTESIAN_POINT('Ctrl Pts',(6.14161751179079,-12.8562313109216,-8.26261375045333));
#52659=CARTESIAN_POINT('Ctrl Pts',(6.1461536325471,-12.8262230153038,-8.27620209831034));
#52660=CARTESIAN_POINT('Ctrl Pts',(6.1494575947754,-12.8043659527202,-8.2860994071512));
#52661=CARTESIAN_POINT('Ctrl Pts',(6.15307533149207,-12.7830341718204,-8.29665125444258));
#52662=CARTESIAN_POINT('Ctrl Pts',(6.15697892940399,-12.7622897446298,-8.3077874826303));
#52663=CARTESIAN_POINT('Ctrl Pts',(6.16243382819168,-12.7333014232692,-8.32334927946783));
#52664=CARTESIAN_POINT('Ctrl Pts',(6.16844710131043,-12.7054621437925,-8.34005240550776));
#52665=CARTESIAN_POINT('Ctrl Pts',(6.17493397014691,-12.6788987311741,-8.35769073070605));
#52666=CARTESIAN_POINT('Ctrl Pts',(6.18156923382221,-12.6517276489029,-8.37573255356872));
#52667=CARTESIAN_POINT('Ctrl Pts',(6.18869965656706,-12.625891567721,-8.39475204203223));
#52668=CARTESIAN_POINT('Ctrl Pts',(6.19622899598039,-12.6014723181196,-8.41452203315139));
#52669=CARTESIAN_POINT('Ctrl Pts',(6.20386985882546,-12.5766913743021,-8.43458485437609));
#52670=CARTESIAN_POINT('Ctrl Pts',(6.21192118959142,-12.5533693081249,-8.45541979900906));
#52671=CARTESIAN_POINT('Ctrl Pts',(6.22028225574658,-12.5315379646513,-8.47679504363041));
#52672=CARTESIAN_POINT('Ctrl Pts',(6.22884384657957,-12.5091830368603,-8.49868293388352));
#52673=CARTESIAN_POINT('Ctrl Pts',(6.23772988080328,-12.4883907997429,-8.52113665235221));
#52674=CARTESIAN_POINT('Ctrl Pts',(6.2468373203672,-12.4691443274329,-8.54392454922704));
#52675=CARTESIAN_POINT('Ctrl Pts',(6.24787065114139,-12.4669606212449,-8.54651006571107));
#52676=CARTESIAN_POINT('Ctrl Pts',(6.24890684035735,-12.4647967651974,-8.5490999082433));
#52677=CARTESIAN_POINT('Ctrl Pts',(6.24994574427476,-12.4626526982907,-8.55169375781615));
#52678=CARTESIAN_POINT('',(7.00000122821582,-12.5220660378628,-8.0444743030066));
#52679=CARTESIAN_POINT('Ctrl Pts',(7.00000132931107,-12.5220647920326,-8.04447409604749));
#52680=CARTESIAN_POINT('Ctrl Pts',(6.96887878389782,-12.5144347474821,-8.07520189714783));
#52681=CARTESIAN_POINT('Ctrl Pts',(6.93707075291002,-12.5075043810512,-8.10494973687714));
#52682=CARTESIAN_POINT('Ctrl Pts',(6.90460107002341,-12.5012608134835,-8.13374300551672));
#52683=CARTESIAN_POINT('Ctrl Pts',(6.86312146827392,-12.4932847363192,-8.17052603540976));
#52684=CARTESIAN_POINT('Ctrl Pts',(6.8205633372368,-12.4864286234133,-8.20575222368633));
#52685=CARTESIAN_POINT('Ctrl Pts',(6.77697281918209,-12.4806721578446,-8.23946237925169));
#52686=CARTESIAN_POINT('Ctrl Pts',(6.7350679148999,-12.4751382906317,-8.27186898750836));
#52687=CARTESIAN_POINT('Ctrl Pts',(6.69220821568608,-12.4706207026436,-8.30287475268951));
#52688=CARTESIAN_POINT('Ctrl Pts',(6.64840148631274,-12.4671221440221,-8.33249307237288));
#52689=CARTESIAN_POINT('Ctrl Pts',(6.60341126484273,-12.4635290675826,-8.36291156700114));
#52690=CARTESIAN_POINT('Ctrl Pts',(6.55744030090632,-12.4610077121262,-8.39186122162719));
#52691=CARTESIAN_POINT('Ctrl Pts',(6.51046156859088,-12.4595840347784,-8.41933237390026));
#52692=CARTESIAN_POINT('Ctrl Pts',(6.49869811470617,-12.4592275465974,-8.42621113833253));
#52693=CARTESIAN_POINT('Ctrl Pts',(6.48687134569449,-12.4589400147176,-8.43299702468925));
#52694=CARTESIAN_POINT('Ctrl Pts',(6.47498059517163,-12.4587221158036,-8.43968951496237));
#52695=CARTESIAN_POINT('Ctrl Pts',(6.42823118731504,-12.4578654293242,-8.46600155950091));
#52696=CARTESIAN_POINT('Ctrl Pts',(6.38049401611387,-12.4580829756919,-8.49087309509549));
#52697=CARTESIAN_POINT('Ctrl Pts',(6.33175355644512,-12.4594129782019,-8.51426069387726));
#52698=CARTESIAN_POINT('Ctrl Pts',(6.30479295496598,-12.4601486640753,-8.5271974559553));
#52699=CARTESIAN_POINT('Ctrl Pts',(6.27752508279713,-12.4612252038702,-8.53967947586593));
#52700=CARTESIAN_POINT('Ctrl Pts',(6.2499457442928,-12.4626526982629,-8.55169375784748));
#52701=CARTESIAN_POINT('',(6.99999966028467,-13.9486981671726,-6.97711506156621));
#52702=CARTESIAN_POINT('Ctrl Pts',(6.999999755579,-13.9486981671724,-6.97711506157905));
#52703=CARTESIAN_POINT('Ctrl Pts',(7.,-13.8626463334129,-7.01419856109545));
#52704=CARTESIAN_POINT('Ctrl Pts',(7.,-13.7400684821722,-7.07011204123475));
#52705=CARTESIAN_POINT('Ctrl Pts',(7.,-13.6272404800293,-7.12645786767111));
#52706=CARTESIAN_POINT('Ctrl Pts',(7.,-13.5541884450668,-7.1641178289169));
#52707=CARTESIAN_POINT('Ctrl Pts',(7.,-13.520579782048,-7.1819856114406));
#52708=CARTESIAN_POINT('Ctrl Pts',(7.,-13.339612670826,-7.28166708221286));
#52709=CARTESIAN_POINT('Ctrl Pts',(7.,-13.2055611610638,-7.36745032586629));
#52710=CARTESIAN_POINT('Ctrl Pts',(7.,-12.8482255802639,-7.63349426885588));
#52711=CARTESIAN_POINT('Ctrl Pts',(7.,-12.6600978814924,-7.8296083475282));
#52712=CARTESIAN_POINT('Ctrl Pts',(7.000002769617,-12.5220662044828,-8.04447387621312));
#52713=CARTESIAN_POINT('Ctrl Pts',(6.99999922604724,-13.9486981671804,-6.97711506153452));
#52714=CARTESIAN_POINT('Ctrl Pts',(6.99999541671456,-13.9418949807255,-7.02119365462051));
#52715=CARTESIAN_POINT('Ctrl Pts',(6.99835381561817,-13.9356151148029,-7.06425756057063));
#52716=CARTESIAN_POINT('Ctrl Pts',(6.9953485697528,-13.9298432802271,-7.10615136253393));
#52717=CARTESIAN_POINT('Ctrl Pts',(6.99234332388744,-13.9240714456514,-7.14804516449724));
#52718=CARTESIAN_POINT('Ctrl Pts',(6.98797379154531,-13.9188076897555,-7.18876918020147));
#52719=CARTESIAN_POINT('Ctrl Pts',(6.98248007277824,-13.9140314092665,-7.22820843471191));
#52720=CARTESIAN_POINT('Ctrl Pts',(6.97660699910893,-13.9089253147672,-7.27037106753371));
#52721=CARTESIAN_POINT('Ctrl Pts',(6.96944999946155,-13.9043759886361,-7.31106590392677));
#52722=CARTESIAN_POINT('Ctrl Pts',(6.96130496881929,-13.900335688588,-7.35021802520771));
#52723=CARTESIAN_POINT('Ctrl Pts',(6.9554290548961,-13.8974209720756,-7.3784627924359));
#52724=CARTESIAN_POINT('Ctrl Pts',(6.94903794299284,-13.8947711282211,-7.4059054976004));
#52725=CARTESIAN_POINT('Ctrl Pts',(6.94223029680783,-13.8923674055314,-7.43252906388036));
#52726=CARTESIAN_POINT('Ctrl Pts',(6.93362366105249,-13.8893284747345,-7.46618817765514));
#52727=CARTESIAN_POINT('Ctrl Pts',(6.92435173757794,-13.8866830002541,-7.49853750694693));
#52728=CARTESIAN_POINT('Ctrl Pts',(6.91459419318944,-13.8843912896279,-7.52956122924081));
#52729=CARTESIAN_POINT('Ctrl Pts',(6.90281862571623,-13.8816256149834,-7.56700117525552));
#52730=CARTESIAN_POINT('Ctrl Pts',(6.89033747519103,-13.8793747431416,-7.60251052333689));
#52731=CARTESIAN_POINT('Ctrl Pts',(6.87745399509062,-13.87755326155,-7.63611118024047));
#52732=CARTESIAN_POINT('Ctrl Pts',(6.86947771174407,-13.8764255652154,-7.65691366202369));
#52733=CARTESIAN_POINT('Ctrl Pts',(6.86134622163443,-13.8754624935046,-7.67698512013817));
#52734=CARTESIAN_POINT('Ctrl Pts',(6.8531229005019,-13.8746441171068,-7.69633557749649));
#52735=CARTESIAN_POINT('Ctrl Pts',(6.84770422519965,-13.8741048561557,-7.70908636804509));
#52736=CARTESIAN_POINT('Ctrl Pts',(6.84224554756976,-13.8736284270604,-7.72152417125158));
#52737=CARTESIAN_POINT('Ctrl Pts',(6.8367636178037,-13.8732091805885,-7.7336526079316));
#52738=CARTESIAN_POINT('Ctrl Pts',(6.83402265292067,-13.8729995573526,-7.73971682627161));
#52739=CARTESIAN_POINT('Ctrl Pts',(6.83127586601031,-13.8728042342134,-7.74570369902245));
#52740=CARTESIAN_POINT('Ctrl Pts',(6.82852524644297,-13.872622504644,-7.75161374361826));
#52741=CARTESIAN_POINT('Ctrl Pts',(6.82714993665931,-13.8725316398593,-7.75456876591616));
#52742=CARTESIAN_POINT('Ctrl Pts',(6.82577366815407,-13.8724441737331,-7.75750458093883));
#52743=CARTESIAN_POINT('Ctrl Pts',(6.82439668502147,-13.8723600188195,-7.76042125420104));
#52744=CARTESIAN_POINT('Ctrl Pts',(6.82331719844689,-13.8722940455355,-7.76270778157706));
#52745=CARTESIAN_POINT('Ctrl Pts',(6.82270593100578,-13.8722577027424,-7.76399798722328));
#52746=CARTESIAN_POINT('Ctrl Pts',(6.82146136860573,-13.8721857550262,-7.76660776827813));
#52747=CARTESIAN_POINT('Ctrl Pts',(6.82111837867054,-13.8721659268982,-7.76732699990109));
#52748=CARTESIAN_POINT('Ctrl Pts',(6.82072709486732,-13.8721434920848,-7.7681463433998));
#52749=CARTESIAN_POINT('Ctrl Pts',(6.82026383294919,-13.8721174008885,-7.76911391468128));
#52750=CARTESIAN_POINT('Ctrl Pts',(6.80986980584361,-13.8715320028847,-7.79082293442298));
#52751=CARTESIAN_POINT('Ctrl Pts',(6.79910043570059,-13.8711237960025,-7.81218975557005));
#52752=CARTESIAN_POINT('Ctrl Pts',(6.78797479033902,-13.8708967998656,-7.83319651415722));
#52753=CARTESIAN_POINT('Ctrl Pts',(6.75802589931483,-13.8702857537334,-7.88974416629362));
#52754=CARTESIAN_POINT('Ctrl Pts',(6.7254993938176,-13.8709862004088,-7.9436820906596));
#52755=CARTESIAN_POINT('Ctrl Pts',(6.69085594874757,-13.8730137832032,-7.99475942931483));
#52756=CARTESIAN_POINT('Ctrl Pts',(6.66371766412754,-13.8746021101971,-8.03477136667432));
#52757=CARTESIAN_POINT('Ctrl Pts',(6.63527897360461,-13.8770054109227,-8.07302800792033));
#52758=CARTESIAN_POINT('Ctrl Pts',(6.6057412909821,-13.8802385643642,-8.10941412831148));
#52759=CARTESIAN_POINT('Ctrl Pts',(6.56617721821083,-13.8845691924528,-8.1581513001952));
#52760=CARTESIAN_POINT('Ctrl Pts',(6.5246436408946,-13.8903876497457,-8.20353270811691));
#52761=CARTESIAN_POINT('Ctrl Pts',(6.4816917663355,-13.8976560231946,-8.24539866607507));
#52762=CARTESIAN_POINT('Ctrl Pts',(6.44899683080048,-13.9031887037539,-8.2772670026868));
#52763=CARTESIAN_POINT('Ctrl Pts',(6.41547887539951,-13.9095620771806,-8.30709844682416));
#52764=CARTESIAN_POINT('Ctrl Pts',(6.3813625868749,-13.9167654813743,-8.33482743069761));
#52765=CARTESIAN_POINT('Ctrl Pts',(6.34283815341129,-13.924899633053,-8.36613925975182));
#52766=CARTESIAN_POINT('Ctrl Pts',(6.30355145233289,-13.9340917614948,-8.39477063371972));
#52767=CARTESIAN_POINT('Ctrl Pts',(6.26385592205553,-13.9442753243951,-8.42070825252017));
#52768=CARTESIAN_POINT('Ctrl Pts',(6.99933866941448,-24.2330493766941,-10.874321862056));
#52769=CARTESIAN_POINT('Ctrl Pts',(6.99933866941448,-24.1955798273609,-10.8803485970913));
#52770=CARTESIAN_POINT('Ctrl Pts',(6.99933866941448,-23.5851351123061,-10.9752955968351));
#52771=CARTESIAN_POINT('Ctrl Pts',(6.99933866941448,-22.3847684638752,-11.0599204357608));
#52772=CARTESIAN_POINT('Ctrl Pts',(6.99933866941448,-20.6450473295107,-10.9047318327807));
#52773=CARTESIAN_POINT('Ctrl Pts',(6.99933866941448,-18.9490871085038,-10.4757466588859));
#52774=CARTESIAN_POINT('Ctrl Pts',(6.99933866941448,-17.342462236957,-9.7823271357614));
#52775=CARTESIAN_POINT('Ctrl Pts',(6.99933866941448,-15.8669670639865,-8.8443674600905));
#52776=CARTESIAN_POINT('Ctrl Pts',(6.99933866941448,-14.734489189311,-7.83889823066968));
#52777=CARTESIAN_POINT('Ctrl Pts',(6.99933866941448,-14.1224323389474,-7.13859596735225));
#52778=CARTESIAN_POINT('Ctrl Pts',(6.99933866941448,-13.9057057528166,-6.86526372147669));
#52779=CARTESIAN_POINT('Ctrl Pts',(7.01704755924886,-24.310389917853,-11.3548276333142));
#52780=CARTESIAN_POINT('Ctrl Pts',(7.01704755924886,-24.2712580736605,-11.3611213667568));
#52781=CARTESIAN_POINT('Ctrl Pts',(7.01704755924886,-23.6337446446486,-11.4602748689665));
#52782=CARTESIAN_POINT('Ctrl Pts',(7.01704755924886,-22.3805064854811,-11.5486515701702));
#52783=CARTESIAN_POINT('Ctrl Pts',(7.01704755924886,-20.5629013815418,-11.3865346008396));
#52784=CARTESIAN_POINT('Ctrl Pts',(7.01704755924886,-18.7919623591938,-10.9385361771176));
#52785=CARTESIAN_POINT('Ctrl Pts',(7.01704755924886,-17.1138140330456,-10.2143156875747));
#52786=CARTESIAN_POINT('Ctrl Pts',(7.01704755924886,-15.5725993502725,-9.23452321255108));
#52787=CARTESIAN_POINT('Ctrl Pts',(7.01704755924886,-14.3899029550477,-8.18446712170575));
#52788=CARTESIAN_POINT('Ctrl Pts',(7.01704755924886,-13.7507244922113,-7.45315527481836));
#52789=CARTESIAN_POINT('Ctrl Pts',(7.01704755924886,-13.5243359009936,-7.1676330973788));
#52790=CARTESIAN_POINT('Ctrl Pts',(6.72711815520593,-24.3727491957856,-11.7422569490181));
#52791=CARTESIAN_POINT('Ctrl Pts',(6.72711815520593,-24.3322770518609,-11.7487659618967));
#52792=CARTESIAN_POINT('Ctrl Pts',(6.72711815520593,-23.6729382589067,-11.8513111452604));
#52793=CARTESIAN_POINT('Ctrl Pts',(6.72711815520593,-22.3770700743642,-11.9427129535966));
#52794=CARTESIAN_POINT('Ctrl Pts',(6.72711815520593,-20.4966675289803,-11.7750096783504));
#52795=CARTESIAN_POINT('Ctrl Pts',(6.72711815520593,-18.6652734872849,-11.3116809697256));
#52796=CARTESIAN_POINT('Ctrl Pts',(6.72711815520593,-16.9294561699855,-10.562625820423));
#52797=CARTESIAN_POINT('Ctrl Pts',(6.72711815520593,-15.335252186698,-9.54910377585614));
#52798=CARTESIAN_POINT('Ctrl Pts',(6.72711815520593,-14.1120648583422,-8.46309752947625));
#52799=CARTESIAN_POINT('Ctrl Pts',(6.72711815520593,-13.451018379787,-7.70678281590056));
#52800=CARTESIAN_POINT('Ctrl Pts',(6.72711815520593,-13.216839363892,-7.41143195975148));
#52801=CARTESIAN_POINT('Ctrl Pts',(6.25441317313844,-24.3925105190614,-11.865031237121));
#52802=CARTESIAN_POINT('Ctrl Pts',(6.25441317313844,-24.3516136412845,-11.8716084709059));
#52803=CARTESIAN_POINT('Ctrl Pts',(6.25441317313844,-23.6853585066674,-11.975228459979));
#52804=CARTESIAN_POINT('Ctrl Pts',(6.25441317313844,-22.3759810939704,-12.0675889086622));
#52805=CARTESIAN_POINT('Ctrl Pts',(6.25441317313844,-20.4756783736281,-11.8981153628051));
#52806=CARTESIAN_POINT('Ctrl Pts',(6.25441317313844,-18.6251264580638,-11.4299285684873));
#52807=CARTESIAN_POINT('Ctrl Pts',(6.25441317313844,-16.8710341444066,-10.6730034476867));
#52808=CARTESIAN_POINT('Ctrl Pts',(6.25441317313844,-15.2600381338117,-9.64879268205177));
#52809=CARTESIAN_POINT('Ctrl Pts',(6.25441317313844,-14.0240194442555,-8.55139402272411));
#52810=CARTESIAN_POINT('Ctrl Pts',(6.25441317313844,-13.3560431079106,-7.78715603376997));
#52811=CARTESIAN_POINT('Ctrl Pts',(6.25441317313844,-13.1193953478972,-7.48869052164871));
#52812=CARTESIAN_POINT('',(7.00000000000001,-24.1259420764689,-10.9277801898196));
#52813=CARTESIAN_POINT('Ctrl Pts',(7.00000000000006,-24.1259420781412,-10.9277802009505));
#52814=CARTESIAN_POINT('Ctrl Pts',(7.00000000000006,-23.9636071725167,-10.9521697295806));
#52815=CARTESIAN_POINT('Ctrl Pts',(7.00000000006077,-23.8012468908441,-10.9728907817485));
#52816=CARTESIAN_POINT('Ctrl Pts',(6.99999999867347,-23.6387646052866,-10.9899916559832));
#52817=CARTESIAN_POINT('Ctrl Pts',(6.99999999728333,-23.4759487464894,-11.0071276380083));
#52818=CARTESIAN_POINT('Ctrl Pts',(6.99999999422996,-23.3130099247608,-11.0206285810807));
#52819=CARTESIAN_POINT('Ctrl Pts',(6.99999999314807,-23.1498445645076,-11.0304911277965));
#52820=CARTESIAN_POINT('Ctrl Pts',(6.99999999206999,-22.9872534292042,-11.0403189654271));
#52821=CARTESIAN_POINT('Ctrl Pts',(6.9999999947222,-22.8244368951336,-11.0465339705941));
#52822=CARTESIAN_POINT('Ctrl Pts',(6.99999999803545,-22.66129298247,-11.0490812192144));
#52823=CARTESIAN_POINT('Ctrl Pts',(6.99999999907237,-22.6102350557993,-11.0498784125092));
#52824=CARTESIAN_POINT('Ctrl Pts',(7.00000000000006,-22.5591450946315,-11.0503159841132));
#52825=CARTESIAN_POINT('Ctrl Pts',(7.00000000000006,-22.508020091487,-11.0503912041561));
#52826=CARTESIAN_POINT('Ctrl Pts',(7.00000000000006,-22.4670935981955,-11.0504514191662));
#52827=CARTESIAN_POINT('Ctrl Pts',(6.99999999938403,-22.4261442171024,-11.050284473563));
#52828=CARTESIAN_POINT('Ctrl Pts',(6.99999999847206,-22.3851771719375,-11.0498891036845));
#52829=CARTESIAN_POINT('Ctrl Pts',(6.99999999416113,-22.1915245001741,-11.0480201762823));
#52830=CARTESIAN_POINT('Ctrl Pts',(6.99999998574668,-21.9974766397739,-11.0410429983301));
#52831=CARTESIAN_POINT('Ctrl Pts',(6.99999998500523,-21.8035275617183,-11.0289287826417));
#52832=CARTESIAN_POINT('Ctrl Pts',(6.99999998426222,-21.6091684925747,-11.0167889585797));
#52833=CARTESIAN_POINT('Ctrl Pts',(6.99999998984227,-21.4149090420865,-10.9994903474823));
#52834=CARTESIAN_POINT('Ctrl Pts',(6.99999999473006,-21.2212489723544,-10.9770562251537));
#52835=CARTESIAN_POINT('Ctrl Pts',(6.99999999759815,-21.1076118068151,-10.9638921791203));
#52836=CARTESIAN_POINT('Ctrl Pts',(7.00000000000006,-20.9941810379534,-10.948960864708));
#52837=CARTESIAN_POINT('Ctrl Pts',(7.00000000000006,-20.8810571711621,-10.9322753272691));
#52838=CARTESIAN_POINT('Ctrl Pts',(7.00000000000006,-20.803036582786,-10.9207674511217));
#52839=CARTESIAN_POINT('Ctrl Pts',(6.99999999890224,-20.7251635517596,-10.908419020453));
#52840=CARTESIAN_POINT('Ctrl Pts',(6.99999999758216,-20.6474486195687,-10.8952326698618));
#52841=CARTESIAN_POINT('Ctrl Pts',(6.9999999934628,-20.4049366467525,-10.8540842340856));
#52842=CARTESIAN_POINT('Ctrl Pts',(6.99999998925875,-20.1639637186277,-10.8047802508425));
#52843=CARTESIAN_POINT('Ctrl Pts',(6.99999999152164,-19.9248987558909,-10.7474287548476));
#52844=CARTESIAN_POINT('Ctrl Pts',(6.99999999354319,-19.7113312431013,-10.6961940769836));
#52845=CARTESIAN_POINT('Ctrl Pts',(7.00000000000006,-19.4992861507214,-10.6385361910376));
#52846=CARTESIAN_POINT('Ctrl Pts',(7.00000000000006,-19.2890339655977,-10.5744977405065));
#52847=CARTESIAN_POINT('Ctrl Pts',(7.00000000000006,-19.17655249537,-10.5402382199093));
#52848=CARTESIAN_POINT('Ctrl Pts',(6.99999999803034,-19.0645775028502,-10.504167106816));
#52849=CARTESIAN_POINT('Ctrl Pts',(6.99999999636317,-18.9531879180019,-10.4662992290709));
#52850=CARTESIAN_POINT('Ctrl Pts',(6.99999999271532,-18.7094607695301,-10.3834420223219));
#52851=CARTESIAN_POINT('Ctrl Pts',(6.99999999204987,-18.4685373676012,-10.2919792986757));
#52852=CARTESIAN_POINT('Ctrl Pts',(6.99999999506641,-18.2311614386956,-10.1922299012747));
#52853=CARTESIAN_POINT('Ctrl Pts',(6.99999999705723,-18.0745004696608,-10.1263983010382));
#52854=CARTESIAN_POINT('Ctrl Pts',(7.00000000000006,-17.9193843979218,-10.0569584114509));
#52855=CARTESIAN_POINT('Ctrl Pts',(7.00000000000006,-17.766022595808,-9.98401350658058));
#52856=CARTESIAN_POINT('Ctrl Pts',(7.00000000000006,-17.6246293972524,-9.91676134029285));
#52857=CARTESIAN_POINT('Ctrl Pts',(6.99999999722481,-17.4847350708803,-9.84651938455048));
#52858=CARTESIAN_POINT('Ctrl Pts',(6.9999999944647,-17.3464252545365,-9.77332652209554));
#52859=CARTESIAN_POINT('Ctrl Pts',(6.99999999008274,-17.1268437480598,-9.65712508805378));
#52860=CARTESIAN_POINT('Ctrl Pts',(6.99999998784249,-16.9112542265341,-9.53348786405889));
#52861=CARTESIAN_POINT('Ctrl Pts',(6.99999999262698,-16.7000150345023,-9.4025775854068));
#52862=CARTESIAN_POINT('Ctrl Pts',(6.99999999531406,-16.5813783940284,-9.32905545386764));
#52863=CARTESIAN_POINT('Ctrl Pts',(7.00000000000006,-16.4641144961371,-9.25323851298255));
#52864=CARTESIAN_POINT('Ctrl Pts',(7.00000000000006,-16.3482917008713,-9.17515026984984));
#52865=CARTESIAN_POINT('Ctrl Pts',(7.00000000000006,-16.1866110203611,-9.06614443675301));
#52866=CARTESIAN_POINT('Ctrl Pts',(6.99999999014838,-16.0276937644611,-8.95275813318587));
#52867=CARTESIAN_POINT('Ctrl Pts',(6.99999998525279,-15.8719395759788,-8.83523425985909));
#52868=CARTESIAN_POINT('Ctrl Pts',(6.99999998003402,-15.705902863785,-8.70995173794678));
#52869=CARTESIAN_POINT('Ctrl Pts',(6.99999998145005,-15.5434613041719,-8.57996719362684));
#52870=CARTESIAN_POINT('Ctrl Pts',(6.99999998835937,-15.3850002943582,-8.4456794914934));
#52871=CARTESIAN_POINT('Ctrl Pts',(6.99999999308637,-15.2765894902534,-8.35380681071988));
#52872=CARTESIAN_POINT('Ctrl Pts',(7.00000000000006,-15.170041121258,-8.25992084727754));
#52873=CARTESIAN_POINT('Ctrl Pts',(7.00000000000006,-15.0654684222749,-8.16415901392044));
#52874=CARTESIAN_POINT('Ctrl Pts',(7.00000000000006,-14.942478127508,-8.05153137566937));
#52875=CARTESIAN_POINT('Ctrl Pts',(6.99999999283358,-14.8222826731093,-7.93626853663342));
#52876=CARTESIAN_POINT('Ctrl Pts',(6.99999999157264,-14.704766055738,-7.81832398014723));
#52877=CARTESIAN_POINT('Ctrl Pts',(6.99999999107903,-14.6587635315272,-7.77215393682353));
#52878=CARTESIAN_POINT('Ctrl Pts',(6.99999999110877,-14.6131718473932,-7.72557250510986));
#52879=CARTESIAN_POINT('Ctrl Pts',(6.99999999149981,-14.567985422531,-7.67857521349894));
#52880=CARTESIAN_POINT('Ctrl Pts',(6.99999999249449,-14.4530460284897,-7.55902957040342));
#52881=CARTESIAN_POINT('Ctrl Pts',(6.99999999551018,-14.3407261040585,-7.43679567026283));
#52882=CARTESIAN_POINT('Ctrl Pts',(6.9999999971704,-14.2309835397531,-7.31180056414431));
#52883=CARTESIAN_POINT('Ctrl Pts',(6.99999999862377,-14.1349138626647,-7.20237866792347));
#52884=CARTESIAN_POINT('Ctrl Pts',(6.99999999923222,-14.0408196901903,-7.09084007133104));
#52885=CARTESIAN_POINT('Ctrl Pts',(6.99999999922778,-13.948698167165,-6.97711506158508));
#52886=CARTESIAN_POINT('',(6.27159471697238,-24.269013917935,-11.8794981306075));
#52887=CARTESIAN_POINT('Origin',(5.999999877384,-24.1259420367214,-10.9277801432445));
#52888=CARTESIAN_POINT('Ctrl Pts',(6.27159470456973,-24.2690136413581,-11.8794980693512));
#52889=CARTESIAN_POINT('Ctrl Pts',(6.27193966908722,-24.0395180543602,-11.9138782815514));
#52890=CARTESIAN_POINT('Ctrl Pts',(6.27225782582989,-23.8113318046113,-11.9412742082228));
#52891=CARTESIAN_POINT('Ctrl Pts',(6.27254917050926,-23.5849162071069,-11.962037041859));
#52892=CARTESIAN_POINT('Ctrl Pts',(6.27284515847502,-23.3548921261236,-11.983130781771));
#52893=CARTESIAN_POINT('Ctrl Pts',(6.27311347294071,-23.1266955387491,-11.9973783462536));
#52894=CARTESIAN_POINT('Ctrl Pts',(6.27335411034387,-22.9007559497552,-12.005146606458));
#52895=CARTESIAN_POINT('Ctrl Pts',(6.27354178947188,-22.7245400145422,-12.0112052668415));
#52896=CARTESIAN_POINT('Ctrl Pts',(6.27371263313229,-22.5496958596412,-12.0133226529662));
#52897=CARTESIAN_POINT('Ctrl Pts',(6.27386663999438,-22.3764053057352,-12.0116720606327));
#52898=CARTESIAN_POINT('Ctrl Pts',(6.27406869011557,-22.1490558425905,-12.0095065572487));
#52899=CARTESIAN_POINT('Ctrl Pts',(6.27424176026293,-21.9243820277569,-12.0008567702672));
#52900=CARTESIAN_POINT('Ctrl Pts',(6.27438584818351,-21.7027300644865,-11.9862080166945));
#52901=CARTESIAN_POINT('Ctrl Pts',(6.27447252049793,-21.5694011318745,-11.9773964426885));
#52902=CARTESIAN_POINT('Ctrl Pts',(6.27454870616355,-21.4371646133612,-11.9664139402272));
#52903=CARTESIAN_POINT('Ctrl Pts',(6.27461440482897,-21.3060872704049,-11.9533633073105));
#52904=CARTESIAN_POINT('Ctrl Pts',(6.27472591390497,-21.0836122276783,-11.9312127201056));
#52905=CARTESIAN_POINT('Ctrl Pts',(6.27480721239585,-20.8644791517284,-11.9031052711444));
#52906=CARTESIAN_POINT('Ctrl Pts',(6.27485829924009,-20.6489740686427,-11.8695298232301));
#52907=CARTESIAN_POINT('Ctrl Pts',(6.27487121344989,-20.594496680279,-11.8610423078113));
#52908=CARTESIAN_POINT('Ctrl Pts',(6.27488219706538,-20.5402508831747,-11.8522052883625));
#52909=CARTESIAN_POINT('Ctrl Pts',(6.27489125007749,-20.4862408043715,-11.8430264891903));
#52910=CARTESIAN_POINT('Ctrl Pts',(6.27492812753947,-20.2662306459103,-11.8056366333501));
#52911=CARTESIAN_POINT('Ctrl Pts',(6.27493296962422,-20.0501355961709,-11.76257741312));
#52912=CARTESIAN_POINT('Ctrl Pts',(6.27490577626535,-19.8381798151852,-11.7143926828644));
#52913=CARTESIAN_POINT('Ctrl Pts',(6.27488257692671,-19.6573550055141,-11.6732850771318));
#52914=CARTESIAN_POINT('Ctrl Pts',(6.27483606148424,-19.4795419596773,-11.6284465854906));
#52915=CARTESIAN_POINT('Ctrl Pts',(6.27476623040389,-19.3048532627893,-11.5802011728913));
#52916=CARTESIAN_POINT('Ctrl Pts',(6.27472435242991,-19.2000917631089,-11.5512682089009));
#52917=CARTESIAN_POINT('Ctrl Pts',(6.2746740891859,-19.0964534576399,-11.5211097231509));
#52918=CARTESIAN_POINT('Ctrl Pts',(6.27461544218523,-18.9939586105461,-11.4897934549333));
#52919=CARTESIAN_POINT('Ctrl Pts',(6.27458611868489,-18.9427111869992,-11.4741353208245));
#52920=CARTESIAN_POINT('Ctrl Pts',(6.27455469661342,-18.8917496307821,-11.4581877322973));
#52921=CARTESIAN_POINT('Ctrl Pts',(6.27452117941578,-18.8410761475086,-11.4419589915794));
#52922=CARTESIAN_POINT('Ctrl Pts',(6.27450442081696,-18.8157394058718,-11.4338446212205));
#52923=CARTESIAN_POINT('Ctrl Pts',(6.27448713825884,-18.7904746826481,-11.4256599622173));
#52924=CARTESIAN_POINT('Ctrl Pts',(6.27446933174197,-18.7652822447661,-11.417406045708));
#52925=CARTESIAN_POINT('Ctrl Pts',(6.27445391981117,-18.7434776373593,-11.4102620999773));
#52926=CARTESIAN_POINT('Ctrl Pts',(6.27443873004181,-18.7225443122958,-11.4033384872226));
#52927=CARTESIAN_POINT('Ctrl Pts',(6.27442216619727,-18.7003606182323,-11.3959293058135));
#52928=CARTESIAN_POINT('Ctrl Pts',(6.27441959263581,-18.6969138882179,-11.3947781247761));
#52929=CARTESIAN_POINT('Ctrl Pts',(6.27441698590347,-18.6934370056222,-11.3936151253547));
#52930=CARTESIAN_POINT('Ctrl Pts',(6.27441434001319,-18.6899220490416,-11.3924375508251));
#52931=CARTESIAN_POINT('Ctrl Pts',(6.27440279689551,-18.6745874912887,-11.3873001944403));
#52932=CARTESIAN_POINT('Ctrl Pts',(6.2743910639149,-18.659253820605,-11.3821284442931));
#52933=CARTESIAN_POINT('Ctrl Pts',(6.27437914107232,-18.6439212023062,-11.376922213299));
#52934=CARTESIAN_POINT('Ctrl Pts',(6.2742001082632,-18.4136873710926,-11.2987457085033));
#52935=CARTESIAN_POINT('Ctrl Pts',(6.27397826546618,-18.1836867138033,-11.2127933414718));
#52936=CARTESIAN_POINT('Ctrl Pts',(6.27371361695892,-17.9544888171664,-11.1188672514994));
#52937=CARTESIAN_POINT('Ctrl Pts',(6.27345239043039,-17.7282545130149,-11.0261556519674));
#52938=CARTESIAN_POINT('Ctrl Pts',(6.27314945800378,-17.5028023070296,-10.9256751677364));
#52939=CARTESIAN_POINT('Ctrl Pts',(6.27280482563134,-17.2787286637382,-10.8172494411368));
#52940=CARTESIAN_POINT('Ctrl Pts',(6.27260798186139,-17.1507444573198,-10.7553198881097));
#52941=CARTESIAN_POINT('Ctrl Pts',(6.27239753412351,-17.0232108844582,-10.6907985735669));
#52942=CARTESIAN_POINT('Ctrl Pts',(6.27217348382512,-16.8962464406854,-10.6236547826323));
#52943=CARTESIAN_POINT('Ctrl Pts',(6.2717701365263,-16.6676782762649,-10.5027789485001));
#52944=CARTESIAN_POINT('Ctrl Pts',(6.27132270436512,-16.4409512945987,-10.3734023863807));
#52945=CARTESIAN_POINT('Ctrl Pts',(6.27083119754382,-16.2167888769591,-10.2354143091808));
#52946=CARTESIAN_POINT('Ctrl Pts',(6.2703673283612,-16.0052312078906,-10.1051853605504));
#52947=CARTESIAN_POINT('Ctrl Pts',(6.26986420337956,-15.7959581779868,-9.96728626862293));
#52948=CARTESIAN_POINT('Ctrl Pts',(6.2693218323302,-15.5896259522535,-9.82164365060285));
#52949=CARTESIAN_POINT('Ctrl Pts',(6.26905885839949,-15.4895837459165,-9.75102739668692));
#52950=CARTESIAN_POINT('Ctrl Pts',(6.26878665818488,-15.3902336026562,-9.67859101895923));
#52951=CARTESIAN_POINT('Ctrl Pts',(6.26850523301692,-15.2916544059507,-9.60432785433404));
#52952=CARTESIAN_POINT('Ctrl Pts',(6.26791731255527,-15.0857143073545,-9.44918595872037));
#52953=CARTESIAN_POINT('Ctrl Pts',(6.26728913172618,-14.8831364031573,-9.28606925080027));
#52954=CARTESIAN_POINT('Ctrl Pts',(6.26662070494602,-14.684553681111,-9.11503058970898));
#52955=CARTESIAN_POINT('Ctrl Pts',(6.26595959126037,-14.4881436042373,-8.94586322093109));
#52956=CARTESIAN_POINT('Ctrl Pts',(6.26525910742267,-14.2956417419887,-8.76894625204622));
#52957=CARTESIAN_POINT('Ctrl Pts',(6.26451927074089,-14.1077007982857,-8.58436221949173));
#52958=CARTESIAN_POINT('Ctrl Pts',(6.26430325540102,-14.0528263539262,-8.53046791618305));
#52959=CARTESIAN_POINT('Ctrl Pts',(6.26408388523087,-13.9983409961619,-8.4759201993414));
#52960=CARTESIAN_POINT('Ctrl Pts',(6.26386116072122,-13.9442616342258,-8.4207216444605));
#52961=CARTESIAN_POINT('Ctrl Pts',(6.99999999998952,-24.7867299440625,-9.33248386897489));
#52962=CARTESIAN_POINT('Ctrl Pts',(6.99999999998952,-24.7867268022291,-9.33249195735394));
#52963=CARTESIAN_POINT('Ctrl Pts',(6.99999999998952,-24.6819075264287,-9.6023398658611));
#52964=CARTESIAN_POINT('Ctrl Pts',(6.99999999998952,-24.467486837193,-10.1365881548782));
#52965=CARTESIAN_POINT('Ctrl Pts',(6.99999999998952,-24.2412740854125,-10.6659288230027));
#52966=CARTESIAN_POINT('Ctrl Pts',(6.99999999998952,-24.1259369152881,-10.9277807259463));
#52967=CARTESIAN_POINT('Ctrl Pts',(7.00000270572501,-25.3377021368351,-9.5465023705352));
#52968=CARTESIAN_POINT('Ctrl Pts',(7.00000270572501,-25.3376989472236,-9.54651058191452));
#52969=CARTESIAN_POINT('Ctrl Pts',(7.00000270572501,-25.2312856813305,-9.82046207694803));
#52970=CARTESIAN_POINT('Ctrl Pts',(7.00000270572501,-25.0136075533826,-10.362826432265));
#52971=CARTESIAN_POINT('Ctrl Pts',(7.00000270572501,-24.7839582727123,-10.9002087469914));
#52972=CARTESIAN_POINT('Ctrl Pts',(7.00000270572501,-24.6668671666083,-11.1660426394912));
#52973=CARTESIAN_POINT('Ctrl Pts',(6.57967197783315,-25.7251433388993,-9.69699923153138));
#52974=CARTESIAN_POINT('Ctrl Pts',(6.57967197783315,-25.7251401156906,-9.69700752940395));
#52975=CARTESIAN_POINT('Ctrl Pts',(6.57967197783315,-25.6176059630351,-9.97384464828113));
#52976=CARTESIAN_POINT('Ctrl Pts',(6.57967197783315,-25.397637218632,-10.5219161854199));
#52977=CARTESIAN_POINT('Ctrl Pts',(6.57967197783315,-25.1655713860881,-11.0649533503668));
#52978=CARTESIAN_POINT('Ctrl Pts',(6.57967197783315,-25.0472469199922,-11.3335873602638));
#52979=CARTESIAN_POINT('Ctrl Pts',(5.98852435812724,-25.7188194279219,-9.69454278460152));
#52980=CARTESIAN_POINT('Ctrl Pts',(5.98852435812724,-25.7188162052615,-9.69455108106231));
#52981=CARTESIAN_POINT('Ctrl Pts',(5.98852435812724,-25.6113003479907,-9.97134110007211));
#52982=CARTESIAN_POINT('Ctrl Pts',(5.98852435812724,-25.3913689915969,-10.5193194831806));
#52983=CARTESIAN_POINT('Ctrl Pts',(5.98852435812724,-25.1593426026096,-11.0622643482657));
#52984=CARTESIAN_POINT('Ctrl Pts',(5.98852435812724,-25.0410382677198,-11.330852653955));
#52985=CARTESIAN_POINT('',(6.99999999994035,-24.7867180660544,-9.33250873275177));
#52986=CARTESIAN_POINT('',(5.98852583803482,-25.7188097331028,-9.69456766152955));
#52987=CARTESIAN_POINT('Origin',(5.999999999061,-24.7867247845918,-9.33250979146072));
#52988=CARTESIAN_POINT('',(5.98852581355281,-25.041038964337,-11.3308503205395));
#52989=CARTESIAN_POINT('Origin',(5.98846855882151,11.4751154998608,4.75314843379863));
#52990=CARTESIAN_POINT('Origin',(6.,-24.1259421517584,-10.9277801936246));
#52991=CARTESIAN_POINT('Origin',(6.99999997874242,11.4664777701405,4.74946019467707));
#52992=CARTESIAN_POINT('Origin',(5.999999877384,-24.1259420367214,-10.9277801432445));
#52993=CARTESIAN_POINT('Origin',(5.99999764418935,-24.1259401205898,-10.92777920691));
#52994=CARTESIAN_POINT('Ctrl Pts',(-6.09469640286227,-25.067939639332,-11.2720340325188));
#52995=CARTESIAN_POINT('Ctrl Pts',(-6.05660168672299,-25.0620362475116,
-11.2843010058053));
#52996=CARTESIAN_POINT('Ctrl Pts',(-5.71257762289918,-25.0092998243332,
-11.394110688857));
#52997=CARTESIAN_POINT('Ctrl Pts',(-5.02644182487932,-24.9143124203008,
-11.5957010011836));
#52998=CARTESIAN_POINT('Ctrl Pts',(-3.98600488126534,-24.7973050957913,
-11.8498309399477));
#52999=CARTESIAN_POINT('Ctrl Pts',(-2.81238881479937,-24.6981603854715,
-12.0695365650579));
#53000=CARTESIAN_POINT('Ctrl Pts',(-1.52056314267948,-24.6290900858772,
-12.2259244827651));
#53001=CARTESIAN_POINT('Ctrl Pts',(-0.189421525832001,-24.6021758282813,
-12.2891015458096));
#53002=CARTESIAN_POINT('Ctrl Pts',(1.08612112074885,-24.6169125737592,-12.2542343899029));
#53003=CARTESIAN_POINT('Ctrl Pts',(2.24134091410634,-24.6645165608675,-12.14542388015));
#53004=CARTESIAN_POINT('Ctrl Pts',(3.27311180230409,-24.7349519813417,-11.987723359583));
#53005=CARTESIAN_POINT('Ctrl Pts',(4.20014655760399,-24.8207557066891,-11.7987497778676));
#53006=CARTESIAN_POINT('Ctrl Pts',(5.05723014150755,-24.9193545614888,-11.5851573172023));
#53007=CARTESIAN_POINT('Ctrl Pts',(5.68071122101956,-25.0048784218136,-11.4035074456581));
#53008=CARTESIAN_POINT('Ctrl Pts',(6.0226216716602,-25.0567655494879,-11.2952493912532));
#53009=CARTESIAN_POINT('Ctrl Pts',(6.09456166898787,-25.0679141839452,-11.2720852989104));
#53010=CARTESIAN_POINT('Ctrl Pts',(-6.21867431468926,-24.9346968833895,
-11.6029424921361));
#53011=CARTESIAN_POINT('Ctrl Pts',(-6.17985088684529,-24.9285688314149,
-11.6153919480189));
#53012=CARTESIAN_POINT('Ctrl Pts',(-5.82924224889114,-24.8737915981942,
-11.726821457879));
#53013=CARTESIAN_POINT('Ctrl Pts',(-5.12989137209224,-24.7745387685011,
-11.9311466147024));
#53014=CARTESIAN_POINT('Ctrl Pts',(-4.06887094871852,-24.6510530267549,
-12.1882783777638));
#53015=CARTESIAN_POINT('Ctrl Pts',(-2.87132776031619,-24.5453674748488,
-12.410182967047));
#53016=CARTESIAN_POINT('Ctrl Pts',(-1.5524869166459,-24.4708982597995,-12.5677689267365));
#53017=CARTESIAN_POINT('Ctrl Pts',(-0.193358844396399,-24.4413460965294,
-12.6311563952282));
#53018=CARTESIAN_POINT('Ctrl Pts',(1.10887434912825,-24.4575903644852,-12.5962055595565));
#53019=CARTESIAN_POINT('Ctrl Pts',(2.28838573686662,-24.5091665685093,-12.4866859321996));
#53020=CARTESIAN_POINT('Ctrl Pts',(3.34148469913762,-24.5846570400626,-12.3275787096358));
#53021=CARTESIAN_POINT('Ctrl Pts',(4.2872641910569,-24.6758354477742,-12.1366054642574));
#53022=CARTESIAN_POINT('Ctrl Pts',(5.16125575332339,-24.7797709394588,-11.9204468212989));
#53023=CARTESIAN_POINT('Ctrl Pts',(5.7967639608332,-24.8691764112112,-11.7363471153343));
#53024=CARTESIAN_POINT('Ctrl Pts',(6.14522058488246,-24.9230952791029,-11.6265024693038));
#53025=CARTESIAN_POINT('Ctrl Pts',(6.21853693433094,-24.9346678113508,-11.6029935132844));
#53026=CARTESIAN_POINT('Ctrl Pts',(-6.3291976151697,-24.6411127990943,-11.8134744744563));
#53027=CARTESIAN_POINT('Ctrl Pts',(-6.28967065041395,-24.6348054639139,
-11.8260431665115));
#53028=CARTESIAN_POINT('Ctrl Pts',(-5.93271715869416,-24.5784070111057,
-11.9385075897552));
#53029=CARTESIAN_POINT('Ctrl Pts',(-5.22084676033754,-24.4758901456533,
-12.1441734830564));
#53030=CARTESIAN_POINT('Ctrl Pts',(-4.14083391228667,-24.3476616660051,
-12.4019308785022));
#53031=CARTESIAN_POINT('Ctrl Pts',(-2.92182478818763,-24.2373538322188,
-12.6234624893178));
#53032=CARTESIAN_POINT('Ctrl Pts',(-1.57942699565776,-24.1591923694902,
-12.7800117355765));
#53033=CARTESIAN_POINT('Ctrl Pts',(-0.196627641794983,-24.127897596587,
-12.8424645128103));
#53034=CARTESIAN_POINT('Ctrl Pts',(1.12798366959883,-24.1451325507698,-12.8080890569226));
#53035=CARTESIAN_POINT('Ctrl Pts',(2.32846860310748,-24.1993949614146,-12.6995305381204));
#53036=CARTESIAN_POINT('Ctrl Pts',(3.40040463563438,-24.2783987537493,-12.5410590148184));
#53037=CARTESIAN_POINT('Ctrl Pts',(4.36313923304952,-24.3734142612292,-12.3501602884885));
#53038=CARTESIAN_POINT('Ctrl Pts',(5.25277086485876,-24.4812739291955,-12.1333723566152));
#53039=CARTESIAN_POINT('Ctrl Pts',(5.89966040938067,-24.5736432781445,-11.9480989079523));
#53040=CARTESIAN_POINT('Ctrl Pts',(6.25441184400203,-24.6291702577748,-11.8372584494335));
#53041=CARTESIAN_POINT('Ctrl Pts',(6.32905697483992,-24.6410811304521,-11.8135238830363));
#53042=CARTESIAN_POINT('Ctrl Pts',(-6.39488356493844,-24.2701531239778,
-11.8436584886566));
#53043=CARTESIAN_POINT('Ctrl Pts',(-6.35487788284077,-24.2637628370598,
-11.8562492151803));
#53044=CARTESIAN_POINT('Ctrl Pts',(-5.99361978154214,-24.2066235446642,
-11.9688688499429));
#53045=CARTESIAN_POINT('Ctrl Pts',(-5.27347862166588,-24.1027720674649,
-12.1740981846543));
#53046=CARTESIAN_POINT('Ctrl Pts',(-4.18145578449957,-23.9728855570156,
-12.4299227229637));
#53047=CARTESIAN_POINT('Ctrl Pts',(-2.9495367877123,-23.8611892252005,-12.6486100257343));
#53048=CARTESIAN_POINT('Ctrl Pts',(-1.59373038381807,-23.7820931269272,
-12.8021774001287));
#53049=CARTESIAN_POINT('Ctrl Pts',(-0.198299206200222,-23.7504472304135,
-12.8628132462037));
#53050=CARTESIAN_POINT('Ctrl Pts',(1.13802038684705,-23.7678739310925,-12.8295103268418));
#53051=CARTESIAN_POINT('Ctrl Pts',(2.35020389927267,-23.8227718588654,-12.7233138532897));
#53052=CARTESIAN_POINT('Ctrl Pts',(3.43313687196658,-23.9027473925422,-12.5673442125066));
#53053=CARTESIAN_POINT('Ctrl Pts',(4.40622315044349,-23.9989707201674,-12.3785772414031));
#53054=CARTESIAN_POINT('Ctrl Pts',(5.30578728126644,-24.1082259561267,-12.1632793605793));
#53055=CARTESIAN_POINT('Ctrl Pts',(5.96018217331522,-24.2017987382936,-11.9784438330912));
#53056=CARTESIAN_POINT('Ctrl Pts',(6.31919070559268,-24.2580531221787,-11.8674820485747));
#53057=CARTESIAN_POINT('Ctrl Pts',(6.39473997476331,-24.2701206174988,-11.8437053720656));
#53058=CARTESIAN_POINT('',(-5.98852245733355,-25.0410395152723,-11.3308498383555));
#53059=CARTESIAN_POINT('Ctrl Pts',(-5.98852261948751,-25.0410393033441,
-11.3308502493374));
#53060=CARTESIAN_POINT('Ctrl Pts',(-5.87205076796215,-25.0233544613059,
-11.367685096755));
#53061=CARTESIAN_POINT('Ctrl Pts',(-5.74888355754614,-25.005242019761,-11.4056286998378));
#53062=CARTESIAN_POINT('Ctrl Pts',(-5.61901871664054,-24.9868831667565,
-11.444317480895));
#53063=CARTESIAN_POINT('Ctrl Pts',(-5.51146429395196,-24.9716783136003,
-11.4763596370485));
#53064=CARTESIAN_POINT('Ctrl Pts',(-5.39931579719988,-24.9563046811778,
-11.5089121550632));
#53065=CARTESIAN_POINT('Ctrl Pts',(-5.28257497430164,-24.9408702526267,
-11.5417420021001));
#53066=CARTESIAN_POINT('Ctrl Pts',(-5.21037293125216,-24.9313243436034,
-11.5620466562067));
#53067=CARTESIAN_POINT('Ctrl Pts',(-5.13641382817025,-24.921756434098,-11.5824542767675));
#53068=CARTESIAN_POINT('Ctrl Pts',(-5.0606977888326,-24.9121959426248,-11.6028979719004));
#53069=CARTESIAN_POINT('Ctrl Pts',(-5.00129388439626,-24.9046951471949,
-11.6189373120801));
#53070=CARTESIAN_POINT('Ctrl Pts',(-4.940808549391,-24.8971989135736,-11.6349987771992));
#53071=CARTESIAN_POINT('Ctrl Pts',(-4.87924165182869,-24.8897228456719,
-11.6510488119178));
#53072=CARTESIAN_POINT('Ctrl Pts',(-4.80922171108662,-24.8812203248014,
-11.6693024924573));
#53073=CARTESIAN_POINT('Ctrl Pts',(-4.73780290838212,-24.8727440062738,
-11.6875411426127));
#53074=CARTESIAN_POINT('Ctrl Pts',(-4.66498524290714,-24.8643182000375,
-11.7057116411845));
#53075=CARTESIAN_POINT('Ctrl Pts',(-4.62857641016964,-24.8601052969194,
-11.7147968904705));
#53076=CARTESIAN_POINT('Ctrl Pts',(-4.59181786178269,-24.8559050168986,
-11.723865099662));
#53077=CARTESIAN_POINT('Ctrl Pts',(-4.55470959781019,-24.8517205219723,
-11.7329092764268));
#53078=CARTESIAN_POINT('Ctrl Pts',(-4.53615546582394,-24.8496282745091,
-11.7374313648091));
#53079=CARTESIAN_POINT('Ctrl Pts',(-4.51751390494272,-24.8475399729966,
-11.7419474449398));
#53080=CARTESIAN_POINT('Ctrl Pts',(-4.49878491518002,-24.8454560142994,
-11.7464566339608));
#53081=CARTESIAN_POINT('Ctrl Pts',(-4.48942042029867,-24.8444140349508,
-11.7487112284712));
#53082=CARTESIAN_POINT('Ctrl Pts',(-4.480034068197,-24.8433731412847,-11.7509641001946));
#53083=CARTESIAN_POINT('Ctrl Pts',(-4.47062585887677,-24.8423333832995,
-11.7532151375777));
#53084=CARTESIAN_POINT('Ctrl Pts',(-4.46121764955655,-24.8412936253143,
-11.7554661749609));
#53085=CARTESIAN_POINT('Ctrl Pts',(-4.45054315234059,-24.8401184151216,
-11.7580112496464));
#53086=CARTESIAN_POINT('Ctrl Pts',(-4.4423356592623,-24.8392175664482,-11.7599626347848));
#53087=CARTESIAN_POINT('Ctrl Pts',(-4.30838925350436,-24.8245157030693,
-11.7918092684698));
#53088=CARTESIAN_POINT('Ctrl Pts',(-4.17012435782523,-24.8100104719952,
-11.8233568462962));
#53089=CARTESIAN_POINT('Ctrl Pts',(-4.02753309951211,-24.7958400284994,
-11.8542867658105));
#53090=CARTESIAN_POINT('Ctrl Pts',(-3.89053390305902,-24.7822253132968,
-11.8840036935517));
#53091=CARTESIAN_POINT('Ctrl Pts',(-3.74954081408819,-24.7689196049158,
-11.9131501841802));
#53092=CARTESIAN_POINT('Ctrl Pts',(-3.60456156835002,-24.756055028871,-11.941428033939));
#53093=CARTESIAN_POINT('Ctrl Pts',(-3.4566234260213,-24.7429278983482,-11.9702830092913));
#53094=CARTESIAN_POINT('Ctrl Pts',(-3.30453072099736,-24.730260574804,-11.9982326013014));
#53095=CARTESIAN_POINT('Ctrl Pts',(-3.14828345340735,-24.7181990088325,
-12.024941127055));
#53096=CARTESIAN_POINT('Ctrl Pts',(-3.07015981961235,-24.7121682258468,
-12.0382953899319));
#53097=CARTESIAN_POINT('Ctrl Pts',(-2.99099754506532,-24.7062889446006,
-12.0513391359894));
#53098=CARTESIAN_POINT('Ctrl Pts',(-2.91079662890743,-24.7005796605404,
-12.0640290816424));
#53099=CARTESIAN_POINT('Ctrl Pts',(-2.89466050069938,-24.6994309736676,
-12.0665822518532));
#53100=CARTESIAN_POINT('Ctrl Pts',(-2.87848233128174,-24.6982891659728,
-12.0691211031326));
#53101=CARTESIAN_POINT('Ctrl Pts',(-2.86226211536665,-24.6971543919734,
-12.0716452719487));
#53102=CARTESIAN_POINT('Ctrl Pts',(-2.83817290389319,-24.6954690993121,
-12.0753940035764));
#53103=CARTESIAN_POINT('Ctrl Pts',(-2.81399095318337,-24.6937993201618,
-12.0791103517112));
#53104=CARTESIAN_POINT('Ctrl Pts',(-2.7897162732971,-24.6921455557091,-12.0827931595367));
#53105=CARTESIAN_POINT('Ctrl Pts',(-2.76940638379877,-24.690761901076,-12.0858744533099));
#53106=CARTESIAN_POINT('Ctrl Pts',(-2.74903157918974,-24.6893894585293,
-12.0889322650775));
#53107=CARTESIAN_POINT('Ctrl Pts',(-2.7285918594789,-24.6880285241487,-12.0919659100489));
#53108=CARTESIAN_POINT('Ctrl Pts',(-2.71837199962347,-24.6873480569584,
-12.0934827325346));
#53109=CARTESIAN_POINT('Ctrl Pts',(-2.70813591099257,-24.6866704667983,
-12.0949935133159));
#53110=CARTESIAN_POINT('Ctrl Pts',(-2.69788359358737,-24.6859957907078,
-12.0964981665553));
#53111=CARTESIAN_POINT('Ctrl Pts',(-2.68763127618217,-24.6853211146172,
-12.0980028197947));
#53112=CARTESIAN_POINT('Ctrl Pts',(-2.67595577372556,-24.6845578593136,
-12.0997054936876));
#53113=CARTESIAN_POINT('Ctrl Pts',(-2.66707795505005,-24.6839805416632,
-12.1009936577339));
#53114=CARTESIAN_POINT('Ctrl Pts',(-2.48139215791761,-24.6719055385544,
-12.1279365112102));
#53115=CARTESIAN_POINT('Ctrl Pts',(-2.29080876534563,-24.6607939753664,
-12.1528481905792));
#53116=CARTESIAN_POINT('Ctrl Pts',(-2.09532194002464,-24.6508433076934,
-12.1752575839113));
#53117=CARTESIAN_POINT('Ctrl Pts',(-1.99172347344666,-24.6455699399835,
-12.1871334675281));
#53118=CARTESIAN_POINT('Ctrl Pts',(-1.88674823654334,-24.6406228500151,
-12.1983058558354));
#53119=CARTESIAN_POINT('Ctrl Pts',(-1.78039790893332,-24.6360331099419,
-12.2086994875532));
#53120=CARTESIAN_POINT('Ctrl Pts',(-1.69972470639523,-24.6325515124814,
-12.2165836904091));
#53121=CARTESIAN_POINT('Ctrl Pts',(-1.61826034679528,-24.6292749693734,
-12.2240209290589));
#53122=CARTESIAN_POINT('Ctrl Pts',(-1.53600337413355,-24.6262160050007,
-12.2309799669966));
#53123=CARTESIAN_POINT('Ctrl Pts',(-1.46173164272138,-24.6234539950101,
-12.2372634440061));
#53124=CARTESIAN_POINT('Ctrl Pts',(-1.38681370628058,-24.6208693844213,
-12.2431570369601));
#53125=CARTESIAN_POINT('Ctrl Pts',(-1.31125082907904,-24.6184705634025,
-12.2486374451097));
#53126=CARTESIAN_POINT('Ctrl Pts',(-1.23162592321267,-24.6159427891185,
-12.254412463203));
#53127=CARTESIAN_POINT('Ctrl Pts',(-1.15128415257726,-24.6136213373792,
-12.2597286510634));
#53128=CARTESIAN_POINT('Ctrl Pts',(-1.07022551562338,-24.611515578708,-12.2645590549739));
#53129=CARTESIAN_POINT('Ctrl Pts',(-1.02969619714645,-24.6104626993724,
-12.2669742569292));
#53130=CARTESIAN_POINT('Ctrl Pts',(-0.988987662088587,-24.6094637393483,
-12.2692680108946));
#53131=CARTESIAN_POINT('Ctrl Pts',(-0.948099910353172,-24.6085198307991,
-12.2714369651261));
#53132=CARTESIAN_POINT('Ctrl Pts',(-0.927656034485465,-24.6080478765245,
-12.2725214422418));
#53133=CARTESIAN_POINT('Ctrl Pts',(-0.907167354448814,-24.6075896848596,
-12.2735747192932));
#53134=CARTESIAN_POINT('Ctrl Pts',(-0.886633870240808,-24.6071453945875,
-12.2745963788644));
#53135=CARTESIAN_POINT('Ctrl Pts',(-0.876367128136804,-24.6069232494515,
-12.2751072086499));
#53136=CARTESIAN_POINT('Ctrl Pts',(-0.866089184989999,-24.6067045796472,
-12.2756101340571));
#53137=CARTESIAN_POINT('Ctrl Pts',(-0.855800040800765,-24.6064894023357,
-12.276105103034));
#53138=CARTESIAN_POINT('Ctrl Pts',(-0.845510896611531,-24.6062742250242,
-12.2766000720109));
#53139=CARTESIAN_POINT('Ctrl Pts',(-0.833523570709159,-24.6060284825045,
-12.2771654501541));
#53140=CARTESIAN_POINT('Ctrl Pts',(-0.824899005106446,-24.6058543649454,
-12.2775660886454));
#53141=CARTESIAN_POINT('Ctrl Pts',(-0.603175520772098,-24.6013780871043,
-12.287865849392));
#53142=CARTESIAN_POINT('Ctrl Pts',(-0.379356108691484,-24.5986972392275,
-12.294099179569));
#53143=CARTESIAN_POINT('Ctrl Pts',(-0.153436083501442,-24.5978636227735,
-12.2960197642684));
#53144=CARTESIAN_POINT('Ctrl Pts',(-0.0981464448159366,-24.5976596109667,
-12.296489790925));
#53145=CARTESIAN_POINT('Ctrl Pts',(-0.0427310282098727,-24.5975662928513,
-12.2967012973707));
#53146=CARTESIAN_POINT('Ctrl Pts',(0.0128096103566303,-24.5975847248816,
-12.2966530210514));
#53147=CARTESIAN_POINT('Ctrl Pts',(0.154052749885538,-24.5976315986283,
-12.2965302515068));
#53148=CARTESIAN_POINT('Ctrl Pts',(0.29610840766086,-24.5984033807796,-12.2947229752056));
#53149=CARTESIAN_POINT('Ctrl Pts',(0.438976597831794,-24.5999235338914,
-12.2911986428102));
#53150=CARTESIAN_POINT('Ctrl Pts',(0.510410692917262,-24.6006836104473,
-12.2894364766125));
#53151=CARTESIAN_POINT('Ctrl Pts',(0.582047920626159,-24.6016307834336,
-12.2872450479625));
#53152=CARTESIAN_POINT('Ctrl Pts',(0.653888280922487,-24.6027673887545,
-12.2846215674522));
#53153=CARTESIAN_POINT('Ctrl Pts',(0.689808461070652,-24.603335691415,-12.2833098271971));
#53154=CARTESIAN_POINT('Ctrl Pts',(0.725779424351655,-24.6039513526094,
-12.2818900742089));
#53155=CARTESIAN_POINT('Ctrl Pts',(0.761801170691137,-24.6046146482615,
-12.2803620000399));
#53156=CARTESIAN_POINT('Ctrl Pts',(0.779812043860877,-24.6049462960875,
-12.2795979629554));
#53157=CARTESIAN_POINT('Ctrl Pts',(0.797835612794589,-24.6052898525645,
-12.2788068455948));
#53158=CARTESIAN_POINT('Ctrl Pts',(0.815871877480789,-24.6056453501107,
-12.2779886141642));
#53159=CARTESIAN_POINT('Ctrl Pts',(0.833908142166988,-24.6060008476568,
-12.2771703827336));
#53160=CARTESIAN_POINT('Ctrl Pts',(0.853574764290539,-24.6064022678434,
-12.2762468935398));
#53161=CARTESIAN_POINT('Ctrl Pts',(0.870018758783986,-24.6067476978381,
-12.2754525453828));
#53162=CARTESIAN_POINT('Ctrl Pts',(0.954872427152908,-24.6085301724204,
-12.2713535805536));
#53163=CARTESIAN_POINT('Ctrl Pts',(1.03910591013512,-24.6105606431458,-12.2666936617127));
#53164=CARTESIAN_POINT('Ctrl Pts',(1.12271338003206,-24.6128292922613,-12.2614998270138));
#53165=CARTESIAN_POINT('Ctrl Pts',(1.34022823043383,-24.6187314547544,-12.2479874437431));
#53166=CARTESIAN_POINT('Ctrl Pts',(1.55350464283,-24.6262446722061,-12.2308647797843));
#53167=CARTESIAN_POINT('Ctrl Pts',(1.76254241975356,-24.6351856038298,-12.2106161409963));
#53168=CARTESIAN_POINT('Ctrl Pts',(1.93919399330944,-24.6427413177473,-12.1935046219354));
#53169=CARTESIAN_POINT('Ctrl Pts',(2.11281902534721,-24.6513168882403,-12.1741597888555));
#53170=CARTESIAN_POINT('Ctrl Pts',(2.28342873010899,-24.6608091507357,-12.1528483689007));
#53171=CARTESIAN_POINT('Ctrl Pts',(2.31456109991636,-24.6625412715827,-12.1489595220846));
#53172=CARTESIAN_POINT('Ctrl Pts',(2.34559309142697,-24.6643039339464,-12.1450051321266));
#53173=CARTESIAN_POINT('Ctrl Pts',(2.37652480039739,-24.6660964943325,-12.140986795155));
#53174=CARTESIAN_POINT('Ctrl Pts',(2.47723059042409,-24.6719326157711,-12.1279041103377));
#53175=CARTESIAN_POINT('Ctrl Pts',(2.57774645010243,-24.6781345523141,-12.1140335534561));
#53176=CARTESIAN_POINT('Ctrl Pts',(2.67730193212354,-24.6846447806991,-12.0995100861891));
#53177=CARTESIAN_POINT('Ctrl Pts',(2.77899779962591,-24.6912949752419,-12.084674372747));
#53178=CARTESIAN_POINT('Ctrl Pts',(2.8796914022943,-24.6982668480994,-12.0691574773542));
#53179=CARTESIAN_POINT('Ctrl Pts',(2.97857178221497,-24.7054759893512,-12.0531516948572));
#53180=CARTESIAN_POINT('Ctrl Pts',(3.01268321914448,-24.7079629758224,-12.047630071249));
#53181=CARTESIAN_POINT('Ctrl Pts',(3.04657896440391,-24.7104780025605,-12.0420506729313));
#53182=CARTESIAN_POINT('Ctrl Pts',(3.0802260433282,-24.7130169985012,-12.036422638873));
#53183=CARTESIAN_POINT('Ctrl Pts',(3.15883688464465,-24.7189489430674,-12.0232736670624));
#53184=CARTESIAN_POINT('Ctrl Pts',(3.23630489540883,-24.7250268680016,-12.0098255651543));
#53185=CARTESIAN_POINT('Ctrl Pts',(3.31262859491132,-24.7312313779075,-11.9961225004861));
#53186=CARTESIAN_POINT('Ctrl Pts',(3.45637318405417,-24.7429166700654,-11.9703147708611));
#53187=CARTESIAN_POINT('Ctrl Pts',(3.59605850742905,-24.7550505065092,-11.9436041773303));
#53188=CARTESIAN_POINT('Ctrl Pts',(3.73168881449518,-24.7675089492556,-11.9162751283198));
#53189=CARTESIAN_POINT('Ctrl Pts',(3.8355116079042,-24.7770456844841,-11.8953551859349));
#53190=CARTESIAN_POINT('Ctrl Pts',(3.93695723414212,-24.7867726890048,-11.8740725457157));
#53191=CARTESIAN_POINT('Ctrl Pts',(4.03602569255836,-24.7966365496557,-11.8525471646707));
#53192=CARTESIAN_POINT('Ctrl Pts',(4.06079280716241,-24.7991025148184,-11.8471658194094));
#53193=CARTESIAN_POINT('Ctrl Pts',(4.08642489230921,-24.8016767052159,-11.8415516114812));
#53194=CARTESIAN_POINT('Ctrl Pts',(4.11438437314248,-24.8045167746375,-11.8353623819252));
#53195=CARTESIAN_POINT('Ctrl Pts',(4.14234385397576,-24.807356844059,-11.8291731523692));
#53196=CARTESIAN_POINT('Ctrl Pts',(4.17012474470698,-24.8102092676449,-11.822961572623));
#53197=CARTESIAN_POINT('Ctrl Pts',(4.19772704535576,-24.813072857578,-11.8167302722123));
#53198=CARTESIAN_POINT('Ctrl Pts',(4.20554193314355,-24.8138836100685,-11.81496603835));
#53199=CARTESIAN_POINT('Ctrl Pts',(4.21334250585392,-24.8146952579057,-11.8132002230615));
#53200=CARTESIAN_POINT('Ctrl Pts',(4.2211287629001,-24.8155077747819,-11.8114328844504));
#53201=CARTESIAN_POINT('Ctrl Pts',(4.26834485873559,-24.8204349014448,-11.8007156902017));
#53202=CARTESIAN_POINT('Ctrl Pts',(4.31503452256417,-24.8253939764717,-11.7899425107744));
#53203=CARTESIAN_POINT('Ctrl Pts',(4.36119776853383,-24.8303793321254,-11.7791263095482));
#53204=CARTESIAN_POINT('Ctrl Pts',(4.51915676200642,-24.8474379627442,-11.7421159948919));
#53205=CARTESIAN_POINT('Ctrl Pts',(4.67095309053977,-24.8648025159746,-11.7046073810182));
#53206=CARTESIAN_POINT('Ctrl Pts',(4.81658449887707,-24.8822581001067,-11.6670799571238));
#53207=CARTESIAN_POINT('Ctrl Pts',(4.86926930145242,-24.8885729741736,-11.6535037310774));
#53208=CARTESIAN_POINT('Ctrl Pts',(4.92114738769541,-24.8948998902692,-11.6399245763458));
#53209=CARTESIAN_POINT('Ctrl Pts',(4.97221904055577,-24.901229111514,-11.6263636369502));
#53210=CARTESIAN_POINT('Ctrl Pts',(5.00451866410746,-24.9052319477673,-11.6177871916434));
#53211=CARTESIAN_POINT('Ctrl Pts',(5.0364956863611,-24.9092353290269,-11.6092188631595));
#53212=CARTESIAN_POINT('Ctrl Pts',(5.0681500716503,-24.9132371031204,-11.6006632531542));
#53213=CARTESIAN_POINT('Ctrl Pts',(5.21038871655004,-24.9312190326083,-11.5622187102472));
#53214=CARTESIAN_POINT('Ctrl Pts',(5.34611257555511,-24.9491678527347,-11.5240350807026));
#53215=CARTESIAN_POINT('Ctrl Pts',(5.47532119490194,-24.9669053701192,-11.4865038210347));
#53216=CARTESIAN_POINT('Ctrl Pts',(5.60704624394362,-24.9849883382614,-11.44824161341));
#53217=CARTESIAN_POINT('Ctrl Pts',(5.73199999775446,-25.0028515439196,-11.4106573120967));
#53218=CARTESIAN_POINT('Ctrl Pts',(5.85018400307863,-25.0203164124304,-11.374112915196));
#53219=CARTESIAN_POINT('Ctrl Pts',(5.86232336329831,-25.022110329716,-11.370359229604));
#53220=CARTESIAN_POINT('Ctrl Pts',(5.87439129930192,-25.0239000542431,-11.366616471453));
#53221=CARTESIAN_POINT('Ctrl Pts',(5.88638781265971,-25.0256853994385,-11.3628850030951));
#53222=CARTESIAN_POINT('Ctrl Pts',(5.92102951903959,-25.0308408477093,-11.3521098363977));
#53223=CARTESIAN_POINT('Ctrl Pts',(5.95507566020921,-25.0359597807444,-11.3414288309808));
#53224=CARTESIAN_POINT('Ctrl Pts',(5.98852582161071,-25.041038287801,-11.3308501130812));
#53225=CARTESIAN_POINT('',(-6.27159361731003,-24.2690120888649,-11.8794975616074));
#53226=CARTESIAN_POINT('Origin',(-5.9999949808,-24.1259380084106,-10.9277770011797));
#53227=CARTESIAN_POINT('Ctrl Pts',(-6.27159386307111,-24.2690123724984,
-11.8794985003173));
#53228=CARTESIAN_POINT('Ctrl Pts',(-6.19708065351306,-24.2574475543624,
-11.9025009389632));
#53229=CARTESIAN_POINT('Ctrl Pts',(-6.11543895257566,-24.2450493566266,
-11.9272858537852));
#53230=CARTESIAN_POINT('Ctrl Pts',(-6.02658472781102,-24.2319368753586,
-11.9536191373682));
#53231=CARTESIAN_POINT('Ctrl Pts',(-5.93855997637016,-24.2189468019272,
-11.9797065940779));
#53232=CARTESIAN_POINT('Ctrl Pts',(-5.843456579914,-24.2052557378526,-12.0073137787139));
#53233=CARTESIAN_POINT('Ctrl Pts',(-5.74118385812537,-24.190999674031,-12.036167269489));
#53234=CARTESIAN_POINT('Ctrl Pts',(-5.64049537709834,-24.1769644416982,
-12.0645738094507));
#53235=CARTESIAN_POINT('Ctrl Pts',(-5.53285779290229,-24.1623816149949,
-12.0941884455386));
#53236=CARTESIAN_POINT('Ctrl Pts',(-5.41817822128907,-24.1474001878375,
-12.1247039897279));
#53237=CARTESIAN_POINT('Ctrl Pts',(-5.37925192931951,-24.1423149629849,
-12.1350620418729));
#53238=CARTESIAN_POINT('Ctrl Pts',(-5.33951424232753,-24.1371839758268,
-12.145523488055));
#53239=CARTESIAN_POINT('Ctrl Pts',(-5.29896141200715,-24.1320135572971,
-12.1560750390864));
#53240=CARTESIAN_POINT('Ctrl Pts',(-5.21821295353835,-24.1217182629216,
-12.1770851997462));
#53241=CARTESIAN_POINT('Ctrl Pts',(-5.13423258229018,-24.1112662697748,
-12.1984532839905));
#53242=CARTESIAN_POINT('Ctrl Pts',(-5.0469909527127,-24.1007138190865,-12.2200666252813));
#53243=CARTESIAN_POINT('Ctrl Pts',(-4.92201111320241,-24.0855966829228,
-12.2510292739491));
#53244=CARTESIAN_POINT('Ctrl Pts',(-4.79033819728022,-24.0702723180806,
-12.2824973998057));
#53245=CARTESIAN_POINT('Ctrl Pts',(-4.65188628790323,-24.0549258574929,
-12.3140999820478));
#53246=CARTESIAN_POINT('Ctrl Pts',(-4.51343437852624,-24.0395793969053,
-12.34570256429));
#53247=CARTESIAN_POINT('Ctrl Pts',(-4.36820327813878,-24.0242107182453,
-12.3774398645895));
#53248=CARTESIAN_POINT('Ctrl Pts',(-4.21611007767937,-24.0090298594609,
-12.4088906061113));
#53249=CARTESIAN_POINT('Ctrl Pts',(-4.07082690496949,-23.9945287290882,
-12.4389331293704));
#53250=CARTESIAN_POINT('Ctrl Pts',(-3.919281825186,-23.9801990076705,-12.4687138657733));
#53251=CARTESIAN_POINT('Ctrl Pts',(-3.76141964906482,-23.9662475292409,
-12.4978250150864));
#53252=CARTESIAN_POINT('Ctrl Pts',(-3.73054601994573,-23.9635189923533,
-12.503518379065));
#53253=CARTESIAN_POINT('Ctrl Pts',(-3.69943080463875,-23.960804995437,-12.5091859945926));
#53254=CARTESIAN_POINT('Ctrl Pts',(-3.66807364565266,-23.9581071929869,
-12.5148246080531));
#53255=CARTESIAN_POINT('Ctrl Pts',(-3.58017499593443,-23.9505448627174,
-12.5306304567171));
#53256=CARTESIAN_POINT('Ctrl Pts',(-3.490375146284,-23.9431096165281,-12.546208731638));
#53257=CARTESIAN_POINT('Ctrl Pts',(-3.39866712296084,-23.9358394501584,
-12.5614848710859));
#53258=CARTESIAN_POINT('Ctrl Pts',(-3.35281311129926,-23.9322043669735,
-12.5691229408098));
#53259=CARTESIAN_POINT('Ctrl Pts',(-3.30648204726695,-23.9286105470841,
-12.5766854190333));
#53260=CARTESIAN_POINT('Ctrl Pts',(-3.25967322938304,-23.9250630078039,
-12.5841625636959));
#53261=CARTESIAN_POINT('Ctrl Pts',(-3.23626882044109,-23.9232892381638,
-12.5879011360272));
#53262=CARTESIAN_POINT('Ctrl Pts',(-3.21274497244039,-23.9215270382459,
-12.5916183712853));
#53263=CARTESIAN_POINT('Ctrl Pts',(-3.1891016016632,-23.9197770417985,-12.5953130271372));
#53264=CARTESIAN_POINT('Ctrl Pts',(-3.17727991627461,-23.9189020435748,
-12.5971603550631));
#53265=CARTESIAN_POINT('Ctrl Pts',(-3.1654283501572,-23.9180300961918,-12.5990020379013));
#53266=CARTESIAN_POINT('Ctrl Pts',(-3.15354689347884,-23.9171612798269,
-12.6008379186848));
#53267=CARTESIAN_POINT('Ctrl Pts',(-3.14166543680048,-23.9162924634619,
-12.6026737994683));
#53268=CARTESIAN_POINT('Ctrl Pts',(-3.12814004811533,-23.9153102015369,
-12.6047504356254));
#53269=CARTESIAN_POINT('Ctrl Pts',(-3.11781284205288,-23.9145643041974,
-12.6063279968725));
#53270=CARTESIAN_POINT('Ctrl Pts',(-3.07662019693105,-23.9115891060443,
-12.6126204945932));
#53271=CARTESIAN_POINT('Ctrl Pts',(-3.03568681537497,-23.9086932554489,
-12.6187484873184));
#53272=CARTESIAN_POINT('Ctrl Pts',(-2.99501443262714,-23.9058746076504,
-12.6247163285268));
#53273=CARTESIAN_POINT('Ctrl Pts',(-2.79739858312814,-23.8921795782105,
-12.6537124170365));
#53274=CARTESIAN_POINT('Ctrl Pts',(-2.6059481172625,-23.8803065355462,-12.6789294120371));
#53275=CARTESIAN_POINT('Ctrl Pts',(-2.42085608552228,-23.8700051487675,
-12.700877549924));
#53276=CARTESIAN_POINT('Ctrl Pts',(-2.23092814035405,-23.859434616882,-12.7233991284594));
#53277=CARTESIAN_POINT('Ctrl Pts',(-2.04769490737325,-23.8505187444206,
-12.7424791212769));
#53278=CARTESIAN_POINT('Ctrl Pts',(-1.87131615446196,-23.8429959123325,
-12.7586449499604));
#53279=CARTESIAN_POINT('Ctrl Pts',(-1.78117031097362,-23.8391510498827,
-12.7669071824476));
#53280=CARTESIAN_POINT('Ctrl Pts',(-1.69281421885882,-23.8356702303762,
-12.7744077811853));
#53281=CARTESIAN_POINT('Ctrl Pts',(-1.60626489566071,-23.8325196335033,
-12.7812144424466));
#53282=CARTESIAN_POINT('Ctrl Pts',(-1.43907112315413,-23.826433390915,-12.7943633768622));
#53283=CARTESIAN_POINT('Ctrl Pts',(-1.27862186952989,-23.8215784079356,
-12.804925193892));
#53284=CARTESIAN_POINT('Ctrl Pts',(-1.12501669320035,-23.8177150204011,
-12.8133804302271));
#53285=CARTESIAN_POINT('Ctrl Pts',(-0.969939790398224,-23.8138146168634,
-12.8219166781235));
#53286=CARTESIAN_POINT('Ctrl Pts',(-0.821838349560999,-23.8109247887991,
-12.8283059141215));
#53287=CARTESIAN_POINT('Ctrl Pts',(-0.680782441978169,-23.808815889581,
-12.8330036984709));
#53288=CARTESIAN_POINT('Ctrl Pts',(-0.538388175208224,-23.8066869808172,
-12.8377460560887));
#53289=CARTESIAN_POINT('Ctrl Pts',(-0.403173390274244,-23.8053537794222,
-12.8407648496665));
#53290=CARTESIAN_POINT('Ctrl Pts',(-0.275183236026138,-23.8045989488871,
-12.8424872290624));
#53291=CARTESIAN_POINT('Ctrl Pts',(-0.236228074657881,-23.8043692082052,
-12.8430114535053));
#53292=CARTESIAN_POINT('Ctrl Pts',(-0.197942004448109,-23.8041931828349,
-12.8434152878692));
#53293=CARTESIAN_POINT('Ctrl Pts',(-0.160325891526743,-23.804065111692,
-12.8437099928471));
#53294=CARTESIAN_POINT('Ctrl Pts',(-0.154008551789045,-23.8040436031187,
-12.8437594863041));
#53295=CARTESIAN_POINT('Ctrl Pts',(-0.147710107568991,-23.804023447473,
-12.8438059009661));
#53296=CARTESIAN_POINT('Ctrl Pts',(-0.141430562185521,-23.8040046167472,
-12.843849290145));
#53297=CARTESIAN_POINT('Ctrl Pts',(-0.103047991455955,-23.8038895173851,
-12.8441144985521));
#53298=CARTESIAN_POINT('Ctrl Pts',(-0.0662560608545565,-23.8038251207424,
-12.8442644001821));
#53299=CARTESIAN_POINT('Ctrl Pts',(-0.0289816147159557,-23.8038019492759,
-12.8443170148345));
#53300=CARTESIAN_POINT('Ctrl Pts',(-0.0185593893001033,-23.8037954703535,
-12.844331726301));
#53301=CARTESIAN_POINT('Ctrl Pts',(-0.00809943928968467,-23.8037923580938,
-12.8443385552721));
#53302=CARTESIAN_POINT('Ctrl Pts',(0.0024435548564048,-23.803792739344,
-12.8443372522127));
#53303=CARTESIAN_POINT('Ctrl Pts',(0.127127989417073,-23.8037972481167,
-12.8443218418633));
#53304=CARTESIAN_POINT('Ctrl Pts',(0.25898642404739,-23.8042924746921,-12.8431696762975));
#53305=CARTESIAN_POINT('Ctrl Pts',(0.397985640324334,-23.8054910550641,
-12.8404650160666));
#53306=CARTESIAN_POINT('Ctrl Pts',(0.535666720384046,-23.8066782692412,
-12.837786004258));
#53307=CARTESIAN_POINT('Ctrl Pts',(0.680354116090917,-23.8085556434041,
-12.8335836901914));
#53308=CARTESIAN_POINT('Ctrl Pts',(0.831993591445606,-23.8113495705492,
-12.8274126495319));
#53309=CARTESIAN_POINT('Ctrl Pts',(0.942261582564669,-23.8133812363334,
-12.8229252411242));
#53310=CARTESIAN_POINT('Ctrl Pts',(1.05620525936726,-23.815897968114,-12.8173959531631));
#53311=CARTESIAN_POINT('Ctrl Pts',(1.17379482851288,-23.818993100867,-12.8106400419382));
#53312=CARTESIAN_POINT('Ctrl Pts',(1.33435500185533,-23.8232192839796,-12.8014153268106));
#53313=CARTESIAN_POINT('Ctrl Pts',(1.50171435296593,-23.8285235621057,-12.7899045033718));
#53314=CARTESIAN_POINT('Ctrl Pts',(1.67576187127814,-23.8351487432857,-12.7756218976607));
#53315=CARTESIAN_POINT('Ctrl Pts',(1.84377414908803,-23.8415441908723,-12.7618345530215));
#53316=CARTESIAN_POINT('Ctrl Pts',(2.01801903026665,-23.8491706974574,-12.7454640321563));
#53317=CARTESIAN_POINT('Ctrl Pts',(2.19835996716835,-23.85825712127,-12.7260475830157));
#53318=CARTESIAN_POINT('Ctrl Pts',(2.26108100521229,-23.8614173018892,-12.7192947077887));
#53319=CARTESIAN_POINT('Ctrl Pts',(2.32453906546292,-23.8647541557383,-12.7121731843065));
#53320=CARTESIAN_POINT('Ctrl Pts',(2.38872722788395,-23.8682775611684,-12.7046628694941));
#53321=CARTESIAN_POINT('Ctrl Pts',(2.47499317115351,-23.8730128562988,-12.6945693512018));
#53322=CARTESIAN_POINT('Ctrl Pts',(2.56257789012541,-23.87808510115,-12.6837736012509));
#53323=CARTESIAN_POINT('Ctrl Pts',(2.65146471615966,-23.8835179367988,-12.6722277411706));
#53324=CARTESIAN_POINT('Ctrl Pts',(2.72897727448682,-23.8882555678843,-12.6621593295416));
#53325=CARTESIAN_POINT('Ctrl Pts',(2.80748002688193,-23.8932674685411,-12.651520474965));
#53326=CARTESIAN_POINT('Ctrl Pts',(2.88696068491028,-23.89856938809,-12.6402790265889));
#53327=CARTESIAN_POINT('Ctrl Pts',(2.92670101392446,-23.9012203478645,-12.6346583024009));
#53328=CARTESIAN_POINT('Ctrl Pts',(2.96668581815838,-23.9039438114799,-12.6288869221067));
#53329=CARTESIAN_POINT('Ctrl Pts',(3.00691344054863,-23.9067417736369,-12.6229608336922));
#53330=CARTESIAN_POINT('Ctrl Pts',(3.02702725174375,-23.9081407547155,-12.619997789485));
#53331=CARTESIAN_POINT('Ctrl Pts',(3.04720176742329,-23.9095583603789,-12.6169960677866));
#53332=CARTESIAN_POINT('Ctrl Pts',(3.06743677586502,-23.9109948393404,-12.6139551599589));
#53333=CARTESIAN_POINT('Ctrl Pts',(3.07755428008588,-23.9117130788211,-12.6124347060451));
#53334=CARTESIAN_POINT('Ctrl Pts',(3.08768690749317,-23.9124360366231,-12.6109044555701));
#53335=CARTESIAN_POINT('Ctrl Pts',(3.09783463114383,-23.9131637438721,-12.6093643448404));
#53336=CARTESIAN_POINT('Ctrl Pts',(3.1079823547945,-23.913891451121,-12.6078242341107));
#53337=CARTESIAN_POINT('Ctrl Pts',(3.11649244074334,-23.9145041917183,-12.6065275662883));
#53338=CARTESIAN_POINT('Ctrl Pts',(3.12832306372687,-23.9153611450882,-12.6047143680975));
#53339=CARTESIAN_POINT('Ctrl Pts',(3.24396685480677,-23.9237378245419,-12.5869904398604));
#53340=CARTESIAN_POINT('Ctrl Pts',(3.35681912039119,-23.9324154957705,-12.5687089038458));
#53341=CARTESIAN_POINT('Ctrl Pts',(3.4668879598054,-23.9413241010436,-12.5500064110851));
#53342=CARTESIAN_POINT('Ctrl Pts',(3.63912660786559,-23.9552645235693,-12.5207402528736));
#53343=CARTESIAN_POINT('Ctrl Pts',(3.80454906756701,-23.9697690124171,-12.4904460839916));
#53344=CARTESIAN_POINT('Ctrl Pts',(3.96321157890833,-23.9845899397826,-12.459612244304));
#53345=CARTESIAN_POINT('Ctrl Pts',(4.12187409024965,-23.9994108671481,-12.4287784046164));
#53346=CARTESIAN_POINT('Ctrl Pts',(4.27377692443362,-24.0145483743825,-12.3974046276365));
#53347=CARTESIAN_POINT('Ctrl Pts',(4.4189885867178,-24.0297823945403,-12.3659264725924));
#53348=CARTESIAN_POINT('Ctrl Pts',(4.56351829145772,-24.0449448711678,-12.3345961484111));
#53349=CARTESIAN_POINT('Ctrl Pts',(4.70142003690318,-24.0602031912136,-12.3031622817141));
#53350=CARTESIAN_POINT('Ctrl Pts',(4.8327746454666,-24.0753671449434,-12.2720086542693));
#53351=CARTESIAN_POINT('Ctrl Pts',(4.90532346446221,-24.0837423892264,-12.254802110066));
#53352=CARTESIAN_POINT('Ctrl Pts',(4.97587515091848,-24.0920892595714,-12.2376801962019));
#53353=CARTESIAN_POINT('Ctrl Pts',(5.04444362554569,-24.1003786527912,-12.2207014861673));
#53354=CARTESIAN_POINT('Ctrl Pts',(5.13538826924481,-24.1113731501452,-12.1981820595218));
#53355=CARTESIAN_POINT('Ctrl Pts',(5.22284414698212,-24.1222663281055,-12.1759149756777));
#53356=CARTESIAN_POINT('Ctrl Pts',(5.30684382899792,-24.1329956869054,-12.1540257892894));
#53357=CARTESIAN_POINT('Ctrl Pts',(5.42689862544594,-24.1483303995594,-12.1227411254289));
#53358=CARTESIAN_POINT('Ctrl Pts',(5.53989391654885,-24.1633297986691,-12.0922303547407));
#53359=CARTESIAN_POINT('Ctrl Pts',(5.64592674944952,-24.1778361923838,-12.0628174732137));
#53360=CARTESIAN_POINT('Ctrl Pts',(5.75378605730955,-24.1925924668584,-12.0328979383218));
#53361=CARTESIAN_POINT('Ctrl Pts',(5.85444112642878,-24.2068385834764,-12.0041143447075));
#53362=CARTESIAN_POINT('Ctrl Pts',(5.94798675722919,-24.2204298947769,-11.9767582307012));
#53363=CARTESIAN_POINT('Ctrl Pts',(6.02496392816279,-24.2316139627471,-11.9542473315183));
#53364=CARTESIAN_POINT('Ctrl Pts',(6.09712692397713,-24.2423550377847,-11.9327020733305));
#53365=CARTESIAN_POINT('Ctrl Pts',(6.16452391351239,-24.2525831812488,-11.9122611829523));
#53366=CARTESIAN_POINT('Ctrl Pts',(6.20165874427759,-24.258218750125,-11.9009985284907));
#53367=CARTESIAN_POINT('Ctrl Pts',(6.23734659769671,-24.2636988047476,-11.8900707716899));
#53368=CARTESIAN_POINT('Ctrl Pts',(6.27159479316353,-24.2690136880217,-11.879498379804));
#53369=CARTESIAN_POINT('Ctrl Pts',(-6.390311350267,-24.5118463360737,-11.8061935774203));
#53370=CARTESIAN_POINT('Ctrl Pts',(-4.260207566844,-24.1870546297901,-12.4817978606254));
#53371=CARTESIAN_POINT('Ctrl Pts',(0.00016633772734,-23.8622593703069,-13.1582627624527));
#53372=CARTESIAN_POINT('Ctrl Pts',(4.260540242299,-24.1870799927345,-12.4817450361405));
#53373=CARTESIAN_POINT('Ctrl Pts',(6.390810363449,-24.5119224270561,-11.8060352994126));
#53374=CARTESIAN_POINT('Ctrl Pts',(-6.390311350267,-23.545895230188,-11.9720501088178));
#53375=CARTESIAN_POINT('Ctrl Pts',(-4.260207566844,-23.2652553174244,-12.6077625233822));
#53376=CARTESIAN_POINT('Ctrl Pts',(0.00016633772734,-22.9846371837595,-13.2461470236444));
#53377=CARTESIAN_POINT('Ctrl Pts',(4.260540242299,-23.2652772306214,-12.6077126725587));
#53378=CARTESIAN_POINT('Ctrl Pts',(6.390810363449,-23.5459609774455,-11.9719011765393));
#53379=CARTESIAN_POINT('Ctrl Pts',(-6.390311350267,-21.4528914442104,-12.0713617472543));
#53380=CARTESIAN_POINT('Ctrl Pts',(-4.260207566844,-21.2792389843666,-12.659242501556));
#53381=CARTESIAN_POINT('Ctrl Pts',(0.0001663377273399,-21.1056335160082,
-13.2456907741115));
#53382=CARTESIAN_POINT('Ctrl Pts',(4.260540242299,-21.2792525410423,-12.65919670638));
#53383=CARTESIAN_POINT('Ctrl Pts',(6.390810363449,-21.4529321268594,-12.0712240207621));
#53384=CARTESIAN_POINT('Ctrl Pts',(-6.390311350267,-18.3168609136217,-11.3879808552382));
#53385=CARTESIAN_POINT('Ctrl Pts',(-4.260207566844,-18.3050659001792,-12.0191856806231));
#53386=CARTESIAN_POINT('Ctrl Pts',(0.0001663377273402,-18.2929947474288,
-12.6510858023083));
#53387=CARTESIAN_POINT('Ctrl Pts',(4.260540242299,-18.3050668428013,-12.0191363361582));
#53388=CARTESIAN_POINT('Ctrl Pts',(6.390810363449,-18.3168636769148,-11.3878329789646));
#53389=CARTESIAN_POINT('Ctrl Pts',(-6.390311350267,-15.6641217900945,-9.96973288195603));
#53390=CARTESIAN_POINT('Ctrl Pts',(-4.260207566844,-15.7526919735633,-10.7489905945888));
#53391=CARTESIAN_POINT('Ctrl Pts',(0.0001663377273394,-15.8421756717823,
-11.5273064696613));
#53392=CARTESIAN_POINT('Ctrl Pts',(4.260540242299,-15.7526849858726,-10.7489298166621));
#53393=CARTESIAN_POINT('Ctrl Pts',(6.390810363449,-15.6641010402186,-9.96955032039603));
#53394=CARTESIAN_POINT('Ctrl Pts',(-6.390311350267,-14.2543287641255,-8.71309675413792));
#53395=CARTESIAN_POINT('Ctrl Pts',(-4.260207566844,-14.3567676644292,-9.62713414228719));
#53396=CARTESIAN_POINT('Ctrl Pts',(0.0001663377273409,-14.4578353619718,
-10.5425565369485));
#53397=CARTESIAN_POINT('Ctrl Pts',(4.260540242299,-14.3567597721566,-9.62706265784722));
#53398=CARTESIAN_POINT('Ctrl Pts',(6.390810363449,-14.2543047651132,-8.71288261692475));
#53399=CARTESIAN_POINT('Ctrl Pts',(-6.390311350267,-13.7249660384067,-8.13937934281661));
#53400=CARTESIAN_POINT('Ctrl Pts',(-4.260207566844,-13.8221738529227,-9.11426644869758));
#53401=CARTESIAN_POINT('Ctrl Pts',(0.0001663377273409,-13.9182987555376,
-10.0902661487876));
#53402=CARTESIAN_POINT('Ctrl Pts',(4.260540242299,-13.8221663466254,-9.11419023383394));
#53403=CARTESIAN_POINT('Ctrl Pts',(6.390810363449,-13.7249432649203,-8.1391509499607));
#53404=CARTESIAN_POINT('',(-6.26385894390912,-13.9442626806115,-8.42070713435433));
#53405=CARTESIAN_POINT('Ctrl Pts',(-6.27159552384312,-24.269012166051,-11.8794980574164));
#53406=CARTESIAN_POINT('Ctrl Pts',(-6.27195777361259,-24.0278185145914,
-11.9156534425328));
#53407=CARTESIAN_POINT('Ctrl Pts',(-6.27229031331253,-23.7878332021302,
-11.9441024507922));
#53408=CARTESIAN_POINT('Ctrl Pts',(-6.27259314318901,-23.5495553100136,
-11.9652318875922));
#53409=CARTESIAN_POINT('Ctrl Pts',(-6.27289863590125,-23.309182198958,-11.9865471192041));
#53410=CARTESIAN_POINT('Ctrl Pts',(-6.27317389400559,-23.0705465785284,
-12.0004135122592));
#53411=CARTESIAN_POINT('Ctrl Pts',(-6.27341891775463,-22.8341072928724,
-12.0072245172161));
#53412=CARTESIAN_POINT('Ctrl Pts',(-6.27366754294784,-22.5941927404691,
-12.0141356326898));
#53413=CARTESIAN_POINT('Ctrl Pts',(-6.27388503846378,-22.3565395172541,
-12.0137824595501));
#53414=CARTESIAN_POINT('Ctrl Pts',(-6.27407140456636,-22.1215730806342,
-12.0065719106687));
#53415=CARTESIAN_POINT('Ctrl Pts',(-6.27421804504213,-21.9366918732854,
-12.0008983557473));
#53416=CARTESIAN_POINT('Ctrl Pts',(-6.274345412718,-21.7534730092084,-11.9909791927894));
#53417=CARTESIAN_POINT('Ctrl Pts',(-6.27445350772255,-21.5721011929363,
-11.9770107164412));
#53418=CARTESIAN_POINT('Ctrl Pts',(-6.27450263019869,-21.4896789500694,
-11.9706629101849));
#53419=CARTESIAN_POINT('Ctrl Pts',(-6.27454777260064,-21.4076378813805,
-11.9634788610596));
#53420=CARTESIAN_POINT('Ctrl Pts',(-6.27458893494047,-21.3259936705028,
-11.9554821150223));
#53421=CARTESIAN_POINT('Ctrl Pts',(-6.27470712676182,-21.0915638974046,
-11.9325205928409));
#53422=CARTESIAN_POINT('Ctrl Pts',(-6.27479250379279,-20.8604098971047,
-11.9028602054795));
#53423=CARTESIAN_POINT('Ctrl Pts',(-6.27484506603337,-20.6328676324398,
-11.867043777871));
#53424=CARTESIAN_POINT('Ctrl Pts',(-6.27489762827396,-20.4053253677749,
-11.8312273502626));
#53425=CARTESIAN_POINT('Ctrl Pts',(-6.27491737572417,-20.1813946486095,
-11.7892548434866));
#53426=CARTESIAN_POINT('Ctrl Pts',(-6.274904308384,-19.9613613260337,-11.7416479058904));
#53427=CARTESIAN_POINT('Ctrl Pts',(-6.27489476877272,-19.8007293735071,
-11.7068931912392));
#53428=CARTESIAN_POINT('Ctrl Pts',(-6.27486754215411,-19.641886015768,-11.6690684550223));
#53429=CARTESIAN_POINT('Ctrl Pts',(-6.27482284572605,-19.4852449189779,
-11.6284287739379));
#53430=CARTESIAN_POINT('Ctrl Pts',(-6.27477793235585,-19.3278435365188,
-11.5875918408694));
#53431=CARTESIAN_POINT('Ctrl Pts',(-6.27471537917892,-19.1726661423447,
-11.5439127568876));
#53432=CARTESIAN_POINT('Ctrl Pts',(-6.27463540657113,-19.0201057129404,
-11.4976958184635));
#53433=CARTESIAN_POINT('Ctrl Pts',(-6.27457693113742,-18.9085545515761,
-11.4639023034869));
#53434=CARTESIAN_POINT('Ctrl Pts',(-6.27450914251616,-18.7984019852882,
-11.4287529048035));
#53435=CARTESIAN_POINT('Ctrl Pts',(-6.27443212685842,-18.6897913755697,
-11.3923809119521));
#53436=CARTESIAN_POINT('Ctrl Pts',(-6.2743563554567,-18.5829354662577,-11.3565965407962));
#53437=CARTESIAN_POINT('Ctrl Pts',(-6.27427024866111,-18.4758579337037,
-11.3190560601371));
#53438=CARTESIAN_POINT('Ctrl Pts',(-6.27417380647165,-18.3686262100889,
-11.2797074657311));
#53439=CARTESIAN_POINT('Ctrl Pts',(-6.27399075729118,-18.1650982806783,
-11.2050230563539));
#53440=CARTESIAN_POINT('Ctrl Pts',(-6.27377047507158,-17.9610120041854,
-11.123823840775));
#53441=CARTESIAN_POINT('Ctrl Pts',(-6.27351295981285,-17.7568367231181,
-11.035841741865));
#53442=CARTESIAN_POINT('Ctrl Pts',(-6.27325823671108,-17.554875250418,-10.9488136051864));
#53443=CARTESIAN_POINT('Ctrl Pts',(-6.2729670836052,-17.3528266037693,-10.8551488043137));
#53444=CARTESIAN_POINT('Ctrl Pts',(-6.27263950049519,-17.1511936567995,
-10.7546017230361));
#53445=CARTESIAN_POINT('Ctrl Pts',(-6.27231700457665,-16.9526919622582,
-10.655616084455));
#53446=CARTESIAN_POINT('Ctrl Pts',(-6.27195920134555,-16.7545931145514,
-10.5499602069169));
#53447=CARTESIAN_POINT('Ctrl Pts',(-6.27156609080189,-16.5574252175733,
-10.4374141472497));
#53448=CARTESIAN_POINT('Ctrl Pts',(-6.2713627573503,-16.4554416160609,-10.379200550225));
#53449=CARTESIAN_POINT('Ctrl Pts',(-6.27114997778991,-16.3537078788031,
-10.319143797673));
#53450=CARTESIAN_POINT('Ctrl Pts',(-6.27092775212072,-16.2523023418362,
-10.2572150776267));
#53451=CARTESIAN_POINT('Ctrl Pts',(-6.27050608517554,-16.0598881929588,
-10.1397070764348));
#53452=CARTESIAN_POINT('Ctrl Pts',(-6.27005040934441,-15.8686527392963,
-10.0154582935042));
#53453=CARTESIAN_POINT('Ctrl Pts',(-6.26956072399719,-15.6791680310297,
-9.88428363945258));
#53454=CARTESIAN_POINT('Ctrl Pts',(-6.2693850560598,-15.6111929771396,-9.83722652196934));
#53455=CARTESIAN_POINT('Ctrl Pts',(-6.26920501137747,-15.543443689627,-9.78927825014016));
#53456=CARTESIAN_POINT('Ctrl Pts',(-6.26902058992111,-15.4759481426865,
-9.74043078842283));
#53457=CARTESIAN_POINT('Ctrl Pts',(-6.26850854403676,-15.2885468624668,
-9.60480588757748));
#53458=CARTESIAN_POINT('Ctrl Pts',(-6.26796275784848,-15.1030987092309,
-9.46224688357658));
#53459=CARTESIAN_POINT('Ctrl Pts',(-6.2673832307336,-14.9201609309892,-9.31269380803585));
#53460=CARTESIAN_POINT('Ctrl Pts',(-6.2668123205751,-14.7399432443758,-9.16536442883974));
#53461=CARTESIAN_POINT('Ctrl Pts',(-6.26620866541429,-14.5621618196626,
-9.01124737044733));
#53462=CARTESIAN_POINT('Ctrl Pts',(-6.26557226465588,-14.387390153543,-8.85031461575968));
#53463=CARTESIAN_POINT('Ctrl Pts',(-6.26502584988123,-14.2373309034618,
-8.71213747859487));
#53464=CARTESIAN_POINT('Ctrl Pts',(-6.26445529515408,-14.0894910489303,
-8.56893625679463));
#53465=CARTESIAN_POINT('Ctrl Pts',(-6.26386060009764,-13.9442583528487,
-8.4207113681085));
#53466=CARTESIAN_POINT('Ctrl Pts',(6.26385988969939,-13.9442649557967,-8.42071839556296));
#53467=CARTESIAN_POINT('Ctrl Pts',(5.97383874386791,-13.9556277753621,-8.54578524258237));
#53468=CARTESIAN_POINT('Ctrl Pts',(5.68187737111666,-13.9653433861138,-8.66214789045299));
#53469=CARTESIAN_POINT('Ctrl Pts',(5.38846823418052,-13.9736716145702,-8.7696610247794));
#53470=CARTESIAN_POINT('Ctrl Pts',(5.11338258670262,-13.9814797426375,-8.87045993130766));
#53471=CARTESIAN_POINT('Ctrl Pts',(4.83702435532471,-13.988068547081,-8.96347945608504));
#53472=CARTESIAN_POINT('Ctrl Pts',(4.55979938137085,-13.9936635247548,-9.0486414964153));
#53473=CARTESIAN_POINT('Ctrl Pts',(4.30239065070984,-13.9988585693446,-9.12771609200192));
#53474=CARTESIAN_POINT('Ctrl Pts',(4.04423465963907,-14.0031969134852,-9.20001611936352));
#53475=CARTESIAN_POINT('Ctrl Pts',(3.78565629268788,-14.0068671085627,-9.26552212090106));
#53476=CARTESIAN_POINT('Ctrl Pts',(3.57067714236566,-14.009918467532,-9.31998307491506));
#53477=CARTESIAN_POINT('Ctrl Pts',(3.35540604275743,-14.0125081378356,-9.36974849325115));
#53478=CARTESIAN_POINT('Ctrl Pts',(3.14002969264849,-14.0147484168714,-9.41483453292874));
#53479=CARTESIAN_POINT('Ctrl Pts',(2.89780153371509,-14.0172680002243,-9.46554162485956));
#53480=CARTESIAN_POINT('Ctrl Pts',(2.65545132443959,-14.019360774289,-9.51033998830773));
#53481=CARTESIAN_POINT('Ctrl Pts',(2.41322275468519,-14.0210847790028,-9.54920642782744));
#53482=CARTESIAN_POINT('Ctrl Pts',(2.17467354086663,-14.0227825967686,-9.5874825015406));
#53483=CARTESIAN_POINT('Ctrl Pts',(1.93624229932215,-14.024122784021,-9.62000545081673));
#53484=CARTESIAN_POINT('Ctrl Pts',(1.69816178307905,-14.0251655159631,-9.64680346661629));
#53485=CARTESIAN_POINT('Ctrl Pts',(1.4617492566177,-14.0262009425354,-9.67341373577774));
#53486=CARTESIAN_POINT('Ctrl Pts',(1.22568255831659,-14.0269430813681,-9.69437893277111));
#53487=CARTESIAN_POINT('Ctrl Pts',(0.990189583399944,-14.0274553092097,
-9.70977763601441));
#53488=CARTESIAN_POINT('Ctrl Pts',(0.75648966765497,-14.0279636369144,-9.72505909250718));
#53489=CARTESIAN_POINT('Ctrl Pts',(0.523354771819489,-14.028245554676,-9.73485846362861));
#53490=CARTESIAN_POINT('Ctrl Pts',(0.291007625024935,-14.0283672016567,
-9.73930374711879));
#53491=CARTESIAN_POINT('Ctrl Pts',(0.193861948610386,-14.0284180629579,
-9.74116234567472));
#53492=CARTESIAN_POINT('Ctrl Pts',(0.0968539805059063,-14.0284409565461,
-9.74208560497615));
#53493=CARTESIAN_POINT('Ctrl Pts',(7.83699083554507E-14,-14.0284409287452,
-9.74208558080452));
#53494=CARTESIAN_POINT('Ctrl Pts',(-7.9714237465531E-7,-14.028440928745,
-9.74208558080432));
#53495=CARTESIAN_POINT('Ctrl Pts',(-1.59428481433331E-6,-14.0284409287448,
-9.74208558080406));
#53496=CARTESIAN_POINT('Ctrl Pts',(-2.39142724503642E-6,-14.0284409287445,
-9.74208558080373));
#53497=CARTESIAN_POINT('Ctrl Pts',(-0.230506176176072,-14.0284408616835,
-9.74208548711302));
#53498=CARTESIAN_POINT('Ctrl Pts',(-0.461891889173131,-14.0283107293459,
-9.73685239088828));
#53499=CARTESIAN_POINT('Ctrl Pts',(-0.693935715395254,-14.0279835403948,
-9.72623762050784));
#53500=CARTESIAN_POINT('Ctrl Pts',(-0.928010413572703,-14.0276534878517,
-9.71552994854139));
#53501=CARTESIAN_POINT('Ctrl Pts',(-1.16275479513849,-14.0271229008488,
-9.69934599832716));
#53502=CARTESIAN_POINT('Ctrl Pts',(-1.39793911692932,-14.0263272827681,
-9.67758619433263));
#53503=CARTESIAN_POINT('Ctrl Pts',(-1.63471589070468,-14.0255262774933,
-9.65567905295272));
#53504=CARTESIAN_POINT('Ctrl Pts',(-1.87193858261666,-14.0244566259444,
-9.62812035587519));
#53505=CARTESIAN_POINT('Ctrl Pts',(-2.10937275100279,-14.0230570272121,
-9.59486143413018));
#53506=CARTESIAN_POINT('Ctrl Pts',(-2.34982868667985,-14.0216396161249,
-9.56117923412431));
#53507=CARTESIAN_POINT('Ctrl Pts',(-2.59050151590398,-14.0198837865677,
-9.52165084198971));
#53508=CARTESIAN_POINT('Ctrl Pts',(-2.83114773156445,-14.0177307442246,
-9.47627906946699));
#53509=CARTESIAN_POINT('Ctrl Pts',(-2.93418571946641,-14.0168088716313,
-9.45685214378084));
#53510=CARTESIAN_POINT('Ctrl Pts',(-3.03721882826862,-14.0158142395614,
-9.43635459918357));
#53511=CARTESIAN_POINT('Ctrl Pts',(-3.14022794330804,-14.0147425141972,
-9.41478954778385));
#53512=CARTESIAN_POINT('Ctrl Pts',(-3.40298087450609,-14.012008785432,-9.3597819839916));
#53513=CARTESIAN_POINT('Ctrl Pts',(-3.66557292847633,-14.0087547923374,
-9.29780917364166));
#53514=CARTESIAN_POINT('Ctrl Pts',(-3.92766534880194,-14.0047774817881,
-9.22884775196303));
#53515=CARTESIAN_POINT('Ctrl Pts',(-4.19885783938051,-14.0006620756565,
-9.15749193146415));
#53516=CARTESIAN_POINT('Ctrl Pts',(-4.46951539858308,-13.9957721838197,
-9.07865430510139));
#53517=CARTESIAN_POINT('Ctrl Pts',(-4.7392627449362,-13.9898918314853,-8.99236905962181));
#53518=CARTESIAN_POINT('Ctrl Pts',(-5.03507315963629,-13.98344331777,-8.89774690821647));
#53519=CARTESIAN_POINT('Ctrl Pts',(-5.32978897414251,-13.9758034680593,
-8.79416873779773));
#53520=CARTESIAN_POINT('Ctrl Pts',(-5.62291527875815,-13.9667005606775,
-8.68174476322627));
#53521=CARTESIAN_POINT('Ctrl Pts',(-5.83748008953337,-13.9600373456432,
-8.59945181151676));
#53522=CARTESIAN_POINT('Ctrl Pts',(-6.05119323169097,-13.952590488428,-8.51242073270881));
#53523=CARTESIAN_POINT('Ctrl Pts',(-6.26386060007216,-13.9442583528048,
-8.42071136807365));
#53524=CARTESIAN_POINT('Ctrl Pts',(6.38247011518717,-13.9383842293975,-8.36786575295797));
#53525=CARTESIAN_POINT('Ctrl Pts',(5.83976911340181,-13.9679622540055,-8.61443012698678));
#53526=CARTESIAN_POINT('Ctrl Pts',(4.5258368467239,-14.0220349167051,-9.12803247901763));
#53527=CARTESIAN_POINT('Ctrl Pts',(2.38629932644282,-14.0625377999656,-9.65166978692595));
#53528=CARTESIAN_POINT('Ctrl Pts',(0.000145959755059722,-14.0741398126941,
-9.84427564872159));
#53529=CARTESIAN_POINT('Ctrl Pts',(-2.38600750188862,-14.0625408462426,
-9.65171698481383));
#53530=CARTESIAN_POINT('Ctrl Pts',(-4.52564624096925,-14.0220410567715,
-9.12809880319294));
#53531=CARTESIAN_POINT('Ctrl Pts',(-5.83967376427529,-13.9679673726684,
-8.6144731341098));
#53532=CARTESIAN_POINT('Ctrl Pts',(-6.38246545188257,-13.9383844561507,
-8.36786779269362));
#53533=CARTESIAN_POINT('Ctrl Pts',(6.177925724167,-13.466791063603,-7.96585293951407));
#53534=CARTESIAN_POINT('Ctrl Pts',(5.65233905480535,-13.4969066625404,-8.20307837018344));
#53535=CARTESIAN_POINT('Ctrl Pts',(4.37999194810445,-13.5523366915063,-8.69728215770289));
#53536=CARTESIAN_POINT('Ctrl Pts',(2.30900032384948,-13.5946978059676,-9.20108707500959));
#53537=CARTESIAN_POINT('Ctrl Pts',(0.000141220875385398,-13.6070941366454,
-9.38635631507042));
#53538=CARTESIAN_POINT('Ctrl Pts',(-2.30871791260755,-13.5947010396693,
-9.20113247851775));
#53539=CARTESIAN_POINT('Ctrl Pts',(-4.3798073931949,-13.5523430345878,-8.69734597758452));
#53540=CARTESIAN_POINT('Ctrl Pts',(-5.65224671339352,-13.496911875029,-8.2031197495587));
#53541=CARTESIAN_POINT('Ctrl Pts',(-6.1779212078179,-13.4667912943994,-7.96585490328432));
#53542=CARTESIAN_POINT('Ctrl Pts',(6.17628879660483,-12.8196117922142,-8.03444678682366));
#53543=CARTESIAN_POINT('Ctrl Pts',(5.65205474344145,-12.8494195568757,-8.26881665925291));
#53544=CARTESIAN_POINT('Ctrl Pts',(4.38232924763575,-12.9043202327645,-8.75753222014369));
#53545=CARTESIAN_POINT('Ctrl Pts',(2.31198089188489,-12.9463013545954,-9.25697094634347));
#53546=CARTESIAN_POINT('Ctrl Pts',(0.000141450441422552,-12.9585829054207,
-9.44098574409741));
#53547=CARTESIAN_POINT('Ctrl Pts',(-2.31169828944397,-12.9463045599124,
-9.25701601862634));
#53548=CARTESIAN_POINT('Ctrl Pts',(-4.38214499322134,-12.9043265148673,
-8.75759539236768));
#53549=CARTESIAN_POINT('Ctrl Pts',(-5.65196263603526,-12.8494247211796,
-8.26885754201286));
#53550=CARTESIAN_POINT('Ctrl Pts',(-6.17628429233524,-12.8196120244309,
-8.03444872628162));
#53551=CARTESIAN_POINT('Ctrl Pts',(6.376125622901,-12.4394717503676,-8.52105869970914));
#53552=CARTESIAN_POINT('Ctrl Pts',(5.83675988447364,-12.4683463754376,-8.76091826903374));
#53553=CARTESIAN_POINT('Ctrl Pts',(4.5293976034514,-12.5212149055004,-9.2616161521347));
#53554=CARTESIAN_POINT('Ctrl Pts',(2.39220470509012,-12.5608645076069,-9.7749319909605));
#53555=CARTESIAN_POINT('Ctrl Pts',(0.000146429844990828,-12.5722117056496,
-9.96455183631497));
#53556=CARTESIAN_POINT('Ctrl Pts',(-2.39191255764638,-12.5608674907541,
-9.77497840220907));
#53557=CARTESIAN_POINT('Ctrl Pts',(-4.52920776688929,-12.5212209074462,
-9.26168095077238));
#53558=CARTESIAN_POINT('Ctrl Pts',(-5.83666511294557,-12.4683513841291,
-8.7609601100695));
#53559=CARTESIAN_POINT('Ctrl Pts',(-6.37612098930916,-12.4394719804615,
-8.52106068240773));
#53560=CARTESIAN_POINT('',(-6.24994532672558,-12.462652132724,-8.55169075504561));
#53561=CARTESIAN_POINT('Origin',(-6.5277204968019,-13.2547548639173,-9.09521590379488));
#53562=CARTESIAN_POINT('Ctrl Pts',(6.24994435006576,-12.4626487224143,-8.5516910297148));
#53563=CARTESIAN_POINT('Ctrl Pts',(5.93520863610954,-12.478935053609,-8.68880231996198));
#53564=CARTESIAN_POINT('Ctrl Pts',(5.61561497397808,-12.4930288863896,-8.81654384237152));
#53565=CARTESIAN_POINT('Ctrl Pts',(5.29150042771701,-12.5052897567797,-8.93429441879265));
#53566=CARTESIAN_POINT('Ctrl Pts',(5.10416783972639,-12.5123763272767,-9.00235221031365));
#53567=CARTESIAN_POINT('Ctrl Pts',(4.9153250937991,-12.5188505341334,-9.06707147399993));
#53568=CARTESIAN_POINT('Ctrl Pts',(4.72503881885995,-12.5247817359611,-9.12832441192078));
#53569=CARTESIAN_POINT('Ctrl Pts',(4.72121098795688,-12.5249010490206,-9.12955658638399));
#53570=CARTESIAN_POINT('Ctrl Pts',(4.71738257406758,-12.5250201403348,-9.13078736032785));
#53571=CARTESIAN_POINT('Ctrl Pts',(4.71355357757958,-12.5251390103775,-9.13201673287128));
#53572=CARTESIAN_POINT('Ctrl Pts',(4.45754789802082,-12.5330866295876,-9.21421225182763));
#53573=CARTESIAN_POINT('Ctrl Pts',(4.19893806746814,-12.5400452191779,-9.29014571126507));
#53574=CARTESIAN_POINT('Ctrl Pts',(3.93791724033779,-12.5461419619073,-9.35956663918277));
#53575=CARTESIAN_POINT('Ctrl Pts',(3.80545482353562,-12.5492359268045,-9.39479625664174));
#53576=CARTESIAN_POINT('Ctrl Pts',(3.67237176886856,-12.5521072046937,-9.42834905312878));
#53577=CARTESIAN_POINT('Ctrl Pts',(3.53869508005236,-12.5547679555686,-9.46019456380016));
#53578=CARTESIAN_POINT('Ctrl Pts',(3.47185673564426,-12.556098331006,-9.47611731913585));
#53579=CARTESIAN_POINT('Ctrl Pts',(3.40486997931727,-12.5573760590713,-9.49161324128445));
#53580=CARTESIAN_POINT('Ctrl Pts',(3.33773832833752,-12.5586023421897,-9.50667870912308));
#53581=CARTESIAN_POINT('Ctrl Pts',(3.30417250284765,-12.5592154837489,-9.51421144304239));
#53582=CARTESIAN_POINT('Ctrl Pts',(3.27057045352523,-12.5598157631269,-9.52163656266291));
#53583=CARTESIAN_POINT('Ctrl Pts',(3.23693262388625,-12.5604033178904,-9.52895361921054));
#53584=CARTESIAN_POINT('Ctrl Pts',(3.20933465675268,-12.5608853738739,-9.53495685688323));
#53585=CARTESIAN_POINT('Ctrl Pts',(3.180755829783,-12.5613750545733,-9.54109103135349));
#53586=CARTESIAN_POINT('Ctrl Pts',(3.15355121784076,-12.5618325282578,-9.54685408039594));
#53587=CARTESIAN_POINT('Ctrl Pts',(3.14759744179454,-12.5619326471593,-9.54811533357665));
#53588=CARTESIAN_POINT('Ctrl Pts',(3.14170952969673,-12.5620312448056,-9.54935900566632));
#53589=CARTESIAN_POINT('Ctrl Pts',(3.13591223970834,-12.5621279382662,-9.55058015248305));
#53590=CARTESIAN_POINT('Ctrl Pts',(2.87755178205346,-12.5664371528765,-9.60500145123953));
#53591=CARTESIAN_POINT('Ctrl Pts',(2.61814577474157,-12.5700203191151,-9.652793457199));
#53592=CARTESIAN_POINT('Ctrl Pts',(2.3578840641493,-12.5730153521193,-9.69382346594162));
#53593=CARTESIAN_POINT('Ctrl Pts',(2.0559289187946,-12.5764901837573,-9.74142640463585));
#53594=CARTESIAN_POINT('Ctrl Pts',(1.75282198464787,-12.5791732609632,-9.77992868385661));
#53595=CARTESIAN_POINT('Ctrl Pts',(1.44895725672518,-12.5811590067854,-9.80926917466022));
#53596=CARTESIAN_POINT('Ctrl Pts',(1.14576931107835,-12.5831403298582,-9.83854431689812));
#53597=CARTESIAN_POINT('Ctrl Pts',(0.841826368189186,-12.5844273449745,
-9.85869852518057));
#53598=CARTESIAN_POINT('Ctrl Pts',(0.537511110199068,-12.5851093061151,
-9.86962038034393));
#53599=CARTESIAN_POINT('Ctrl Pts',(0.358491817075135,-12.5855104828492,
-9.87604537133472));
#53600=CARTESIAN_POINT('Ctrl Pts',(0.179343559716909,-12.5857021945379,
-9.8792744456513));
#53601=CARTESIAN_POINT('Ctrl Pts',(0.000144045323212458,-12.5857020417033,
-9.87927649693224));
#53602=CARTESIAN_POINT('Ctrl Pts',(9.53568818153291E-5,-12.5857020416617,
-9.87927649748958));
#53603=CARTESIAN_POINT('Ctrl Pts',(4.66684366375151E-5,-12.585702041606,
-9.87927649780865));
#53604=CARTESIAN_POINT('Ctrl Pts',(-2.02001232150136E-6,-12.5857020415362,
-9.87927649788946));
#53605=CARTESIAN_POINT('Ctrl Pts',(-0.298119005239199,-12.5857016138055,
-9.87927699270075));
#53606=CARTESIAN_POINT('Ctrl Pts',(-0.596080646488231,-12.5851365239961,
-9.87039237637331));
#53607=CARTESIAN_POINT('Ctrl Pts',(-0.89354275403253,-12.5839683223329,
-9.85270238622077));
#53608=CARTESIAN_POINT('Ctrl Pts',(-1.1210836629543,-12.5830747171929,-9.83917059062046));
#53609=CARTESIAN_POINT('Ctrl Pts',(-1.34833217344988,-12.5818281693976,
-9.82048537709595));
#53610=CARTESIAN_POINT('Ctrl Pts',(-1.57512820480823,-12.5802099836666,
-9.79666281776233));
#53611=CARTESIAN_POINT('Ctrl Pts',(-1.83662850139142,-12.5783441836081,
-9.76919493706882));
#53612=CARTESIAN_POINT('Ctrl Pts',(-2.09753059605828,-12.575973201931,-9.73491182923078));
#53613=CARTESIAN_POINT('Ctrl Pts',(-2.35759908107191,-12.5729990046887,
-9.69389384419149));
#53614=CARTESIAN_POINT('Ctrl Pts',(-2.35774019131026,-12.5729973909227,
-9.69387158829361));
#53615=CARTESIAN_POINT('Ctrl Pts',(-2.35788130130321,-12.572995776979,-9.69384933041219));
#53616=CARTESIAN_POINT('Ctrl Pts',(-2.35802241105073,-12.5729941628576,
-9.69382707054729));
#53617=CARTESIAN_POINT('Ctrl Pts',(-2.48812675613284,-12.5715059297154,
-9.67330329245208));
#53618=CARTESIAN_POINT('Ctrl Pts',(-2.61802246404346,-12.5698659514544,
-9.65109436515554));
#53619=CARTESIAN_POINT('Ctrl Pts',(-2.74768075918299,-12.5680600288683,
-9.6272147285293));
#53620=CARTESIAN_POINT('Ctrl Pts',(-2.81250990675276,-12.5671570675753,
-9.61527491021618));
#53621=CARTESIAN_POINT('Ctrl Pts',(-2.87727970070071,-12.5662126091452,
-9.6029174058796));
#53622=CARTESIAN_POINT('Ctrl Pts',(-2.9419865920507,-12.5652245964307,-9.59014423675178));
#53623=CARTESIAN_POINT('Ctrl Pts',(-2.97434003772569,-12.5647305900734,
-9.58375765218786));
#53624=CARTESIAN_POINT('Ctrl Pts',(-3.00667775770639,-12.564225694429,-9.57726715086189));
#53625=CARTESIAN_POINT('Ctrl Pts',(-3.03899930980661,-12.5637096414949,
-9.57067299017703));
#53626=CARTESIAN_POINT('Ctrl Pts',(-3.06566659180715,-12.5632838658676,
-9.56523239926745));
#53627=CARTESIAN_POINT('Ctrl Pts',(-3.09135655462812,-12.5628663941347,
-9.55992271288502));
#53628=CARTESIAN_POINT('Ctrl Pts',(-3.11846086046902,-12.562417769849,-9.55424587330949));
#53629=CARTESIAN_POINT('Ctrl Pts',(-3.12420779283676,-12.5623226479358,
-9.55304221167379));
#53630=CARTESIAN_POINT('Ctrl Pts',(-3.13001826947044,-12.5622261062038,
-9.55182186515024));
#53631=CARTESIAN_POINT('Ctrl Pts',(-3.13591502092693,-12.5621277362302,
-9.55057978976115));
#53632=CARTESIAN_POINT('Ctrl Pts',(-3.45257930704656,-12.5568451229652,
-9.48387850189209));
#53633=CARTESIAN_POINT('Ctrl Pts',(-3.76614685428018,-12.5505102571087,
-9.40752256927021));
#53634=CARTESIAN_POINT('Ctrl Pts',(-4.07624236026289,-12.5429015342422,
-9.32200266916992));
#53635=CARTESIAN_POINT('Ctrl Pts',(-4.29026496940007,-12.5376501239874,
-9.26297829829228));
#53636=CARTESIAN_POINT('Ctrl Pts',(-4.50263387066465,-12.5317919731508,
-9.19958748653664));
#53637=CARTESIAN_POINT('Ctrl Pts',(-4.71322682841913,-12.5252544390584,
-9.13197721008274));
#53638=CARTESIAN_POINT('Ctrl Pts',(-5.02876448392235,-12.5154590584232,
-9.03067473374325));
#53639=CARTESIAN_POINT('Ctrl Pts',(-5.34031574361354,-12.5041386185149,
-8.91990198233565));
#53640=CARTESIAN_POINT('Ctrl Pts',(-5.64761398272241,-12.4910219758922,
-8.80016008656025));
#53641=CARTESIAN_POINT('Ctrl Pts',(-5.85026677362467,-12.4823719938992,
-8.72119435790141));
#53642=CARTESIAN_POINT('Ctrl Pts',(-6.0510698467664,-12.4729408293642,-8.63832685047973));
#53643=CARTESIAN_POINT('Ctrl Pts',(-6.24994452572252,-12.4626498485398,
-8.55168918768589));
#53644=CARTESIAN_POINT('Ctrl Pts',(-6.24277095337913,-13.9570481133821,
-8.44169435429085));
#53645=CARTESIAN_POINT('Ctrl Pts',(-6.29815583077892,-13.9532401195528,
-8.41824340131205));
#53646=CARTESIAN_POINT('Ctrl Pts',(-6.4447418010428,-13.9493436454455,-8.34436057253389));
#53647=CARTESIAN_POINT('Ctrl Pts',(-6.66526187295068,-13.9714492594668,
-8.17939903115658));
#53648=CARTESIAN_POINT('Ctrl Pts',(-6.87369344496963,-14.036253579378,-7.93773816682672));
#53649=CARTESIAN_POINT('Ctrl Pts',(-7.019185666524,-14.1323671765394,-7.66828606903858));
#53650=CARTESIAN_POINT('Ctrl Pts',(-7.0965183656736,-14.2455227590742,-7.40111221773899));
#53651=CARTESIAN_POINT('Ctrl Pts',(-7.10969901122602,-14.3273043817824,
-7.23055752275661));
#53652=CARTESIAN_POINT('Ctrl Pts',(-7.10784879432356,-14.3669526800853,
-7.15228421614289));
#53653=CARTESIAN_POINT('Ctrl Pts',(-6.04395576815581,-13.495653564219,-8.0326875434042));
#53654=CARTESIAN_POINT('Ctrl Pts',(-6.09276946049994,-13.4920218131833,
-8.01223198182578));
#53655=CARTESIAN_POINT('Ctrl Pts',(-6.22228199799112,-13.4876402372165,
-7.94771003933163));
#53656=CARTESIAN_POINT('Ctrl Pts',(-6.41829649695095,-13.5050515638676,
-7.80303765417474));
#53657=CARTESIAN_POINT('Ctrl Pts',(-6.60464059843952,-13.5598578050206,
-7.59012754325846));
#53658=CARTESIAN_POINT('Ctrl Pts',(-6.73521158016175,-13.6429459389554,
-7.35210380136168));
#53659=CARTESIAN_POINT('Ctrl Pts',(-6.80469368075153,-13.7418688573599,
-7.1160681283494));
#53660=CARTESIAN_POINT('Ctrl Pts',(-6.81649571475142,-13.8137195396554,
-6.96583884061849));
#53661=CARTESIAN_POINT('Ctrl Pts',(-6.81483976643568,-13.8485536822665,
-6.89712306094761));
#53662=CARTESIAN_POINT('Ctrl Pts',(-6.02805601653886,-12.8501482256791,
-8.09057476185638));
#53663=CARTESIAN_POINT('Ctrl Pts',(-6.09538291160628,-12.8454029891221,
-8.06277674238425));
#53664=CARTESIAN_POINT('Ctrl Pts',(-6.27265850281004,-12.8403106482999,
-7.9757587629418));
#53665=CARTESIAN_POINT('Ctrl Pts',(-6.53595054453926,-12.8655837800627,
-7.7844790925534));
#53666=CARTESIAN_POINT('Ctrl Pts',(-6.78171371030984,-12.9396065336219,
-7.50843369672343));
#53667=CARTESIAN_POINT('Ctrl Pts',(-6.95183436866027,-13.0485085954569,
-7.20361737708373));
#53668=CARTESIAN_POINT('Ctrl Pts',(-7.04202608316068,-13.1761754239708,
-6.90252126095774));
#53669=CARTESIAN_POINT('Ctrl Pts',(-7.05751522705347,-13.2686270590318,
-6.7097519791209));
#53670=CARTESIAN_POINT('Ctrl Pts',(-7.05533880391617,-13.313666237071,-6.62082661348952));
#53671=CARTESIAN_POINT('Ctrl Pts',(-6.20650780120442,-12.4602299621517,
-8.57738035221049));
#53672=CARTESIAN_POINT('Ctrl Pts',(-6.30488566866451,-12.453836841744,-8.5368768391189));
#53673=CARTESIAN_POINT('Ctrl Pts',(-6.56239159754601,-12.4482921495602,
-8.41074728563732));
#53674=CARTESIAN_POINT('Ctrl Pts',(-6.9391515270053,-12.4886612913967,-8.13753809672886));
#53675=CARTESIAN_POINT('Ctrl Pts',(-7.28557450517007,-12.5981021554977,
-7.7492384229932));
#53676=CARTESIAN_POINT('Ctrl Pts',(-7.5229153234017,-12.7541756117298,-7.324649770896));
#53677=CARTESIAN_POINT('Ctrl Pts',(-7.64834332712291,-12.9340958564118,
-6.9063608319225));
#53678=CARTESIAN_POINT('Ctrl Pts',(-7.67008672986089,-13.0637272878827,
-6.63699912917934));
#53679=CARTESIAN_POINT('Ctrl Pts',(-7.66702778969363,-13.1270784697037,
-6.51178563799198));
#53680=CARTESIAN_POINT('',(-7.00001043113205,-13.9487143148388,-6.97711954537448));
#53681=CARTESIAN_POINT('',(-7.00000027445394,-12.5220632044943,-8.04447892907881));
#53682=CARTESIAN_POINT('Ctrl Pts',(-7.,-13.9487143149799,-6.97711954518352));
#53683=CARTESIAN_POINT('Ctrl Pts',(-7.,-13.845491146465,-7.02162187524465));
#53684=CARTESIAN_POINT('Ctrl Pts',(-7.,-13.754333549677,-7.0634883841343));
#53685=CARTESIAN_POINT('Ctrl Pts',(-7.,-13.6767079632962,-7.10164870932265));
#53686=CARTESIAN_POINT('Ctrl Pts',(-7.,-13.6378951701058,-7.12072887191683));
#53687=CARTESIAN_POINT('Ctrl Pts',(-7.,-13.6024393883131,-7.13883660024732));
#53688=CARTESIAN_POINT('Ctrl Pts',(-7.,-13.5703851007164,-7.15566494585842));
#53689=CARTESIAN_POINT('Ctrl Pts',(-7.,-13.5543579569181,-7.16407911866396));
#53690=CARTESIAN_POINT('Ctrl Pts',(-7.,-13.5391800633319,-7.17217227343122));
#53691=CARTESIAN_POINT('Ctrl Pts',(-7.,-13.5248512234156,-7.17990207217249));
#53692=CARTESIAN_POINT('Ctrl Pts',(-7.,-13.5176868034574,-7.18376697154313));
#53693=CARTESIAN_POINT('Ctrl Pts',(-7.,-13.5107346469166,-7.18754103190727));
#53694=CARTESIAN_POINT('Ctrl Pts',(-7.,-13.5039943937985,-7.19121892813308));
#53695=CARTESIAN_POINT('Ctrl Pts',(-7.,-13.5006242672395,-7.19305787624598));
#53696=CARTESIAN_POINT('Ctrl Pts',(-7.,-13.4973071165361,-7.19487278332431));
#53697=CARTESIAN_POINT('Ctrl Pts',(-7.,-13.4940428913842,-7.19666299402289));
#53698=CARTESIAN_POINT('Ctrl Pts',(-7.,-13.4907786662322,-7.19845320472147));
#53699=CARTESIAN_POINT('Ctrl Pts',(-7.,-13.4891249577557,-7.19936055090131));
#53700=CARTESIAN_POINT('Ctrl Pts',(-7.,-13.4844089378928,-7.2019588837331));
#53701=CARTESIAN_POINT('Ctrl Pts',(-7.,-13.4089526200857,-7.24353220904171));
#53702=CARTESIAN_POINT('Ctrl Pts',(-7.,-13.3377436713999,-7.28579001561386));
#53703=CARTESIAN_POINT('Ctrl Pts',(-7.,-13.2712863644665,-7.32835269250401));
#53704=CARTESIAN_POINT('Ctrl Pts',(-7.,-13.2048290575331,-7.37091536939417));
#53705=CARTESIAN_POINT('Ctrl Pts',(-7.,-13.1443246620373,-7.41287378405723));
#53706=CARTESIAN_POINT('Ctrl Pts',(-7.,-13.0863576832307,-7.45602150139235));
#53707=CARTESIAN_POINT('Ctrl Pts',(-7.,-12.9704237256174,-7.54231693606261));
#53708=CARTESIAN_POINT('Ctrl Pts',(-7.,-12.8624865278623,-7.63585832171496));
#53709=CARTESIAN_POINT('Ctrl Pts',(-7.,-12.7672163298947,-7.73520842630034));
#53710=CARTESIAN_POINT('Ctrl Pts',(-7.,-12.6719461319271,-7.83455853088573));
#53711=CARTESIAN_POINT('Ctrl Pts',(-7.,-12.5894789845998,-7.93953599603716));
#53712=CARTESIAN_POINT('Ctrl Pts',(-7.,-12.5220635189387,-8.04447812614683));
#53713=CARTESIAN_POINT('Ctrl Pts',(-6.24994591284326,-12.4626538041299,
-8.55169190192368));
#53714=CARTESIAN_POINT('Ctrl Pts',(-6.29984502952175,-12.4600715183856,
-8.5299538017944));
#53715=CARTESIAN_POINT('Ctrl Pts',(-6.34871496710572,-12.4586373900724,
-8.50669099475367));
#53716=CARTESIAN_POINT('Ctrl Pts',(-6.39657992048361,-12.4582954827157,
-8.48197367229514));
#53717=CARTESIAN_POINT('Ctrl Pts',(-6.42793514231834,-12.458071507129,-8.46578192710052));
#53718=CARTESIAN_POINT('Ctrl Pts',(-6.45885896943399,-12.4583168141412,
-8.44896505528031));
#53719=CARTESIAN_POINT('Ctrl Pts',(-6.48935513207306,-12.4590220513095,
-8.43153301532157));
#53720=CARTESIAN_POINT('Ctrl Pts',(-6.53665120488326,-12.4601157937863,
-8.40449790795816));
#53721=CARTESIAN_POINT('Ctrl Pts',(-6.58292002814214,-12.4623144775476,
-8.37598485615482));
#53722=CARTESIAN_POINT('Ctrl Pts',(-6.62819544396853,-12.465585688379,-8.34601162845821));
#53723=CARTESIAN_POINT('Ctrl Pts',(-6.63503349783147,-12.4660797471404,
-8.34148470050637));
#53724=CARTESIAN_POINT('Ctrl Pts',(-6.64184884345374,-12.4665983213324,
-8.3369243973713));
#53725=CARTESIAN_POINT('Ctrl Pts',(-6.64864154412372,-12.467141352241,-8.33233071027927));
#53726=CARTESIAN_POINT('Ctrl Pts',(-6.69594096035842,-12.4709226236704,
-8.30034362173017));
#53727=CARTESIAN_POINT('Ctrl Pts',(-6.74212293424803,-12.4758915212378,
-8.26674704428514));
#53728=CARTESIAN_POINT('Ctrl Pts',(-6.78718061207176,-12.4820430406497,
-8.23152520023946));
#53729=CARTESIAN_POINT('Ctrl Pts',(-6.83223828989548,-12.4881945600615,
-8.19630335619378));
#53730=CARTESIAN_POINT('Ctrl Pts',(-6.87617234032553,-12.4955288522721,
-8.15945574064839));
#53731=CARTESIAN_POINT('Ctrl Pts',(-6.91893148542368,-12.5040687076553,
-8.12093600965497));
#53732=CARTESIAN_POINT('Ctrl Pts',(-6.94644685185362,-12.5095640759464,
-8.09614869197979));
#53733=CARTESIAN_POINT('Ctrl Pts',(-6.97347471723017,-12.5155592318714,
-8.07066836258662));
#53734=CARTESIAN_POINT('Ctrl Pts',(-7.00000082162213,-12.5220620483258,
-8.04447919620794));
#53735=CARTESIAN_POINT('Ctrl Pts',(-6.26385534042556,-13.9442720969407,
-8.42069792283772));
#53736=CARTESIAN_POINT('Ctrl Pts',(-6.30612913172524,-13.9334276586312,
-8.393074980389));
#53737=CARTESIAN_POINT('Ctrl Pts',(-6.34794395424447,-13.9237064047667,
-8.3623944118752));
#53738=CARTESIAN_POINT('Ctrl Pts',(-6.38887223123086,-13.9151877588231,
-8.32867404218946));
#53739=CARTESIAN_POINT('Ctrl Pts',(-6.43384340086241,-13.9058276415651,
-8.29162277649167));
#53740=CARTESIAN_POINT('Ctrl Pts',(-6.47774452173498,-13.897919689472,-8.25090041315255));
#53741=CARTESIAN_POINT('Ctrl Pts',(-6.52005084106735,-13.8914885296134,
-8.2066635433403));
#53742=CARTESIAN_POINT('Ctrl Pts',(-6.53777952753404,-13.8887935181222,
-8.18812584950294));
#53743=CARTESIAN_POINT('Ctrl Pts',(-6.55522760709187,-13.886357991745,-8.16897117842091));
#53744=CARTESIAN_POINT('Ctrl Pts',(-6.57235390700123,-13.8841845943505,
-8.14921175211991));
#53745=CARTESIAN_POINT('Ctrl Pts',(-6.5861973044387,-13.8824278106855,-8.13323996645292));
#53746=CARTESIAN_POINT('Ctrl Pts',(-6.59983046404273,-13.8808423141501,
-8.11687304420284));
#53747=CARTESIAN_POINT('Ctrl Pts',(-6.61323083027859,-13.8794298320133,
-8.10011755820082));
#53748=CARTESIAN_POINT('Ctrl Pts',(-6.64590221527833,-13.8759860643667,
-8.05926606769717));
#53749=CARTESIAN_POINT('Ctrl Pts',(-6.67719137476755,-13.8735702711939,
-8.01610413538155));
#53750=CARTESIAN_POINT('Ctrl Pts',(-6.70681950479909,-13.8721615260151,
-7.97079335835709));
#53751=CARTESIAN_POINT('Ctrl Pts',(-6.72770964821358,-13.8711682507464,
-7.93884572517013));
#53752=CARTESIAN_POINT('Ctrl Pts',(-6.74777362032552,-13.8706757328006,
-7.90583003453161));
#53753=CARTESIAN_POINT('Ctrl Pts',(-6.76690562480041,-13.8706795466101,
-7.87180523652566));
#53754=CARTESIAN_POINT('Ctrl Pts',(-6.77618565666782,-13.870681396509,-7.85530141382417));
#53755=CARTESIAN_POINT('Ctrl Pts',(-6.78524634454529,-13.8708000658958,
-7.8385601337316));
#53756=CARTESIAN_POINT('Ctrl Pts',(-6.79407489018008,-13.8710353077612,
-7.82158832904041));
#53757=CARTESIAN_POINT('Ctrl Pts',(-6.7943469477008,-13.8710425568961,-7.82106533156185));
#53758=CARTESIAN_POINT('Ctrl Pts',(-6.79461878474062,-13.8710499167433,
-7.82054211518253));
#53759=CARTESIAN_POINT('Ctrl Pts',(-6.79489040101669,-13.8710573872386,
-7.82001868017595));
#53760=CARTESIAN_POINT('Ctrl Pts',(-6.7994333225514,-13.8711823351039,-7.81126396121066));
#53761=CARTESIAN_POINT('Ctrl Pts',(-6.80391449395765,-13.8713382356806,
-7.80244807312468));
#53762=CARTESIAN_POINT('Ctrl Pts',(-6.80833258184899,-13.8715247945615,
-7.79357229387828));
#53763=CARTESIAN_POINT('Ctrl Pts',(-6.81054162579466,-13.871618074002,-7.78913440425508));
#53764=CARTESIAN_POINT('Ctrl Pts',(-6.81273489854703,-13.8717190181075,
-7.78468154176765));
#53765=CARTESIAN_POINT('Ctrl Pts',(-6.81491223129425,-13.8718275909203,
-7.78021386629139));
#53766=CARTESIAN_POINT('Ctrl Pts',(-6.81652751824644,-13.8719081372897,
-7.77689945423717));
#53767=CARTESIAN_POINT('Ctrl Pts',(-6.81855728648138,-13.8720156889984,
-7.77269732427786));
#53768=CARTESIAN_POINT('Ctrl Pts',(-6.82005848244088,-13.8720999717879,
-7.76956453127851));
#53769=CARTESIAN_POINT('Ctrl Pts',(-6.82058082980177,-13.8721292983341,
-7.76847446295995));
#53770=CARTESIAN_POINT('Ctrl Pts',(-6.82103962979231,-13.8721555817735,
-7.7675141188402));
#53771=CARTESIAN_POINT('Ctrl Pts',(-6.82139623906195,-13.8721761601389,
-7.76676656116145));
#53772=CARTESIAN_POINT('Ctrl Pts',(-6.83575184946987,-13.8730045597979,
-7.73667298898843));
#53773=CARTESIAN_POINT('Ctrl Pts',(-6.85002639449847,-13.874185312472,-7.70455942481883));
#53774=CARTESIAN_POINT('Ctrl Pts',(-6.86393641265041,-13.8758132973589,
-7.670365998745));
#53775=CARTESIAN_POINT('Ctrl Pts',(-6.87708941310866,-13.8773526832698,
-7.63803346374));
#53776=CARTESIAN_POINT('Ctrl Pts',(-6.88991660308488,-13.8792919442696,
-7.60384113002283));
#53777=CARTESIAN_POINT('Ctrl Pts',(-6.90213804711071,-13.8817125104589,
-7.56776145381844));
#53778=CARTESIAN_POINT('Ctrl Pts',(-6.90769941303009,-13.8828139886707,
-7.55134340361085));
#53779=CARTESIAN_POINT('Ctrl Pts',(-6.91313476695845,-13.8840151483965,
-7.53453488091171));
#53780=CARTESIAN_POINT('Ctrl Pts',(-6.91841458762728,-13.8853237667971,
-7.51733513890366));
#53781=CARTESIAN_POINT('Ctrl Pts',(-6.92704805286015,-13.887463595434,-7.48921043847256));
#53782=CARTESIAN_POINT('Ctrl Pts',(-6.93526621074753,-13.889890883691,-7.46003892947911));
#53783=CARTESIAN_POINT('Ctrl Pts',(-6.94294163685135,-13.8926328856932,
-7.42983414009522));
#53784=CARTESIAN_POINT('Ctrl Pts',(-6.95237988057618,-13.896004644191,-7.39269220686497));
#53785=CARTESIAN_POINT('Ctrl Pts',(-6.96099870250611,-13.8998523152925,
-7.35398679499351));
#53786=CARTESIAN_POINT('Ctrl Pts',(-6.96853214253001,-13.9042238202432,
-7.31377108169759));
#53787=CARTESIAN_POINT('Ctrl Pts',(-6.97439397820933,-13.9076253265419,
-7.28247888287218));
#53788=CARTESIAN_POINT('Ctrl Pts',(-6.97959814398842,-13.9113439203884,
-7.25027282717614));
#53789=CARTESIAN_POINT('Ctrl Pts',(-6.98400299079825,-13.9154010683865,
-7.21719263050833));
#53790=CARTESIAN_POINT('Ctrl Pts',(-6.98927533587738,-13.920257238239,-7.17759756179238));
#53791=CARTESIAN_POINT('Ctrl Pts',(-6.99340294124102,-13.9255988112762,
-7.1367486794794));
#53792=CARTESIAN_POINT('Ctrl Pts',(-6.99614956769376,-13.9314442793002,
-7.09476435678002));
#53793=CARTESIAN_POINT('Ctrl Pts',(-6.99865578183743,-13.9367780933046,
-7.05645492330856));
#53794=CARTESIAN_POINT('Ctrl Pts',(-7.00001226545564,-13.9425313541841,
-7.01720035980972));
#53795=CARTESIAN_POINT('Ctrl Pts',(-7.00001530585652,-13.9487143147908,
-6.97711954573686));
#53796=CARTESIAN_POINT('Ctrl Pts',(-6.23412706809605,-24.3933911327703,
-11.8700326072878));
#53797=CARTESIAN_POINT('Ctrl Pts',(-6.23490236892324,-23.8924704339311,
-11.9504784732052));
#53798=CARTESIAN_POINT('Ctrl Pts',(-6.23649016701325,-22.7260268100557,
-12.0627656084535));
#53799=CARTESIAN_POINT('Ctrl Pts',(-6.23803702240708,-20.8893388269326,
-11.9701378589627));
#53800=CARTESIAN_POINT('Ctrl Pts',(-6.23758982654153,-18.9411592545323,
-11.5416382303731));
#53801=CARTESIAN_POINT('Ctrl Pts',(-6.23570065532116,-17.0892597438815,
-10.7961461814687));
#53802=CARTESIAN_POINT('Ctrl Pts',(-6.23204684345145,-15.3875898374077,
-9.7563195899027));
#53803=CARTESIAN_POINT('Ctrl Pts',(-6.22725829190456,-14.0755224934574,
-8.61699903004171));
#53804=CARTESIAN_POINT('Ctrl Pts',(-6.22399874199105,-13.3673849692544,
-7.81350344253181));
#53805=CARTESIAN_POINT('Ctrl Pts',(-6.22266320381891,-13.1134091391432,
-7.49367959650599));
#53806=CARTESIAN_POINT('Ctrl Pts',(-6.72598859051384,-24.3745664585965,
-11.7530878020866));
#53807=CARTESIAN_POINT('Ctrl Pts',(-6.7266817490657,-23.8785348888993,-11.8323472612636));
#53808=CARTESIAN_POINT('Ctrl Pts',(-6.72805001567041,-22.7235334782936,
-11.9427161005427));
#53809=CARTESIAN_POINT('Ctrl Pts',(-6.72941756715414,-20.9054810194554,
-11.8502334328646));
#53810=CARTESIAN_POINT('Ctrl Pts',(-6.72902256625366,-18.9767970133252,
-11.426261407818));
#53811=CARTESIAN_POINT('Ctrl Pts',(-6.72736650672518,-17.1431698816911,
-10.6891596966517));
#53812=CARTESIAN_POINT('Ctrl Pts',(-6.72416283555794,-15.4573996370106,
-9.66126047143717));
#53813=CARTESIAN_POINT('Ctrl Pts',(-6.71993196287863,-14.1564693360957,
-8.53486457539566));
#53814=CARTESIAN_POINT('Ctrl Pts',(-6.71707743903688,-13.4537908800506,
-7.74007194970102));
#53815=CARTESIAN_POINT('Ctrl Pts',(-6.71588870767409,-13.2016810518248,
-7.42369098479773));
#53816=CARTESIAN_POINT('Ctrl Pts',(-7.02718530998673,-24.31001596234,-11.3520775656941));
#53817=CARTESIAN_POINT('Ctrl Pts',(-7.02756400531626,-23.8309256023114,
-11.4283612752642));
#53818=CARTESIAN_POINT('Ctrl Pts',(-7.02824891920641,-22.715203036292,-11.5344334835993));
#53819=CARTESIAN_POINT('Ctrl Pts',(-7.02897724317147,-20.9601356719232,
-11.4446336096401));
#53820=CARTESIAN_POINT('Ctrl Pts',(-7.02876731759399,-19.0974432641274,
-11.0353407112804));
#53821=CARTESIAN_POINT('Ctrl Pts',(-7.02790277820779,-17.3268270760829,
-10.3242162170371));
#53822=CARTESIAN_POINT('Ctrl Pts',(-7.02622942251418,-15.6982394083911,
-9.33267672447058));
#53823=CARTESIAN_POINT('Ctrl Pts',(-7.02397939018392,-14.4407075914223,
-8.24600021840375));
#53824=CARTESIAN_POINT('Ctrl Pts',(-7.02249270527262,-13.7610270857261,
-7.4788788442118));
#53825=CARTESIAN_POINT('Ctrl Pts',(-7.02184974022686,-13.5171506741341,
-7.17356208348521));
#53826=CARTESIAN_POINT('Ctrl Pts',(-6.99838062461256,-24.2298260420536,
-10.8539091165241));
#53827=CARTESIAN_POINT('Ctrl Pts',(-6.99835912903231,-23.7718326954283,
-10.9268138766316));
#53828=CARTESIAN_POINT('Ctrl Pts',(-6.9982153209083,-22.7049180611933,-11.0282120131631));
#53829=CARTESIAN_POINT('Ctrl Pts',(-6.99814245032493,-21.0278292767672,
-10.9423805653543));
#53830=CARTESIAN_POINT('Ctrl Pts',(-6.99816421389256,-19.2468670671633,
-10.5510771500295));
#53831=CARTESIAN_POINT('Ctrl Pts',(-6.99828068869748,-17.5546312925736,
-9.87141112190437));
#53832=CARTESIAN_POINT('Ctrl Pts',(-6.99850456716759,-15.9978548244506,
-8.92372022371394));
#53833=CARTESIAN_POINT('Ctrl Pts',(-6.99873523316308,-14.7957513523325,
-7.88504846905375));
#53834=CARTESIAN_POINT('Ctrl Pts',(-6.99894167868191,-14.1458853061617,
-7.15167096124464));
#53835=CARTESIAN_POINT('Ctrl Pts',(-6.99898903069594,-13.9127708169516,
-6.85988336420863));
#53836=CARTESIAN_POINT('',(-7.0000030891977,-24.125943062142,-10.9277695894192));
#53837=CARTESIAN_POINT('Origin',(-5.99998370364475,-24.1259473086388,-10.9277595202031));
#53838=CARTESIAN_POINT('Ctrl Pts',(-7.00001101651448,-24.1259401091717,
-10.9277661762291));
#53839=CARTESIAN_POINT('Ctrl Pts',(-7.00001786894841,-23.9375949534064,
-10.9560764261617));
#53840=CARTESIAN_POINT('Ctrl Pts',(-7.00001802524214,-23.7511662537831,
-10.9791079086878));
#53841=CARTESIAN_POINT('Ctrl Pts',(-7.0000155683377,-23.5669990799827,-10.9972403661653));
#53842=CARTESIAN_POINT('Ctrl Pts',(-7.0000130640501,-23.3792801108786,-11.0157225210181));
#53843=CARTESIAN_POINT('Ctrl Pts',(-7.00000784335894,-23.1939106487979,
-11.0291149206812));
#53844=CARTESIAN_POINT('Ctrl Pts',(-7.00000354816807,-23.0112023806734,
-11.0378133705975));
#53845=CARTESIAN_POINT('Ctrl Pts',(-7.00000225617042,-22.9562435535322,
-11.0404298729061));
#53846=CARTESIAN_POINT('Ctrl Pts',(-7.00000104339694,-22.9015251573104,
-11.0426216150342));
#53847=CARTESIAN_POINT('Ctrl Pts',(-6.99999999753982,-22.847054769903,-11.0443992490626));
#53848=CARTESIAN_POINT('Ctrl Pts',(-6.99999887667118,-22.7886776292046,
-11.0463043794779));
#53849=CARTESIAN_POINT('Ctrl Pts',(-6.99999794691794,-22.7305853442371,
-11.0477338778685));
#53850=CARTESIAN_POINT('Ctrl Pts',(-6.9999971808834,-22.6727849338843,-11.0487021572659));
#53851=CARTESIAN_POINT('Ctrl Pts',(-6.99999462212509,-22.4797162504666,
-11.0519364669757));
#53852=CARTESIAN_POINT('Ctrl Pts',(-6.99999387748843,-22.2899078168075,
-11.050026312357));
#53853=CARTESIAN_POINT('Ctrl Pts',(-6.99999403435033,-22.1035889084951,
-11.0434957480642));
#53854=CARTESIAN_POINT('Ctrl Pts',(-6.99999406717179,-22.0646039374335,
-11.0421293067177));
#53855=CARTESIAN_POINT('Ctrl Pts',(-6.99999414003531,-22.0257715713113,
-11.0405605114676));
#53856=CARTESIAN_POINT('Ctrl Pts',(-6.99999424548476,-21.9870936476159,
-11.0387940517674));
#53857=CARTESIAN_POINT('Ctrl Pts',(-6.99999432422052,-21.9582140730811,
-11.0374750925343));
#53858=CARTESIAN_POINT('Ctrl Pts',(-6.99999441863043,-21.9301065451492,
-11.0360814515155));
#53859=CARTESIAN_POINT('Ctrl Pts',(-6.99999453138995,-21.901184306029,-11.0345337140022));
#53860=CARTESIAN_POINT('Ctrl Pts',(-6.99999463682153,-21.8741416446345,
-11.033086559744));
#53861=CARTESIAN_POINT('Ctrl Pts',(-6.99999475847225,-21.8463866802539,
-11.0315045683461));
#53862=CARTESIAN_POINT('Ctrl Pts',(-6.99999490350815,-21.8166248342906,
-11.0296819413284));
#53863=CARTESIAN_POINT('Ctrl Pts',(-6.99999520366054,-21.7550325699726,
-11.0259100071154));
#53864=CARTESIAN_POINT('Ctrl Pts',(-6.99999556265647,-21.6935868982399,
-11.0216269195953));
#53865=CARTESIAN_POINT('Ctrl Pts',(-6.99999595370132,-21.6322955714664,
-11.0168388713854));
#53866=CARTESIAN_POINT('Ctrl Pts',(-6.99999673579101,-21.5097129179193,
-11.0072627749656));
#53867=CARTESIAN_POINT('Ctrl Pts',(-6.99999764537228,-21.3877476442089,
-10.995666835787));
#53868=CARTESIAN_POINT('Ctrl Pts',(-6.99999847632133,-21.2664591437397,
-10.9821001893882));
#53869=CARTESIAN_POINT('Ctrl Pts',(-6.99999902465859,-21.1864217398015,
-10.9731476575841));
#53870=CARTESIAN_POINT('Ctrl Pts',(-6.99999953897947,-21.1066789849853,
-10.9633369557869));
#53871=CARTESIAN_POINT('Ctrl Pts',(-6.99999996276647,-21.0272472797666,
-10.9526820994163));
#53872=CARTESIAN_POINT('Ctrl Pts',(-7.00000126736821,-20.7827217472362,
-10.9198817910146));
#53873=CARTESIAN_POINT('Ctrl Pts',(-7.00000171385074,-20.5411477461523,
-10.8790828146912));
#53874=CARTESIAN_POINT('Ctrl Pts',(-7.00000170643174,-20.303018854281,-10.8307712657362));
#53875=CARTESIAN_POINT('Ctrl Pts',(-7.00000169893342,-20.0623438256886,
-10.7819431569977));
#53876=CARTESIAN_POINT('Ctrl Pts',(-7.00000122940917,-19.8251879290421,
-10.7254409706034));
#53877=CARTESIAN_POINT('Ctrl Pts',(-7.00000072342062,-19.5920096956152,
-10.6617510391509));
#53878=CARTESIAN_POINT('Ctrl Pts',(-7.00000046988425,-19.4751707606954,
-10.6298378384775));
#53879=CARTESIAN_POINT('Ctrl Pts',(-7.00000020716486,-19.3593297160924,
-10.5961197500517));
#53880=CARTESIAN_POINT('Ctrl Pts',(-6.9999999876648,-19.2445395631775,-10.5606565087878));
#53881=CARTESIAN_POINT('Ctrl Pts',(-6.99999993928972,-19.2192412461647,
-10.552840853028));
#53882=CARTESIAN_POINT('Ctrl Pts',(-6.9999998930078,-19.1939939597544,-10.5449404304622));
#53883=CARTESIAN_POINT('Ctrl Pts',(-6.99999984878645,-19.1687981731766,
-10.5369559936987));
#53884=CARTESIAN_POINT('Ctrl Pts',(-6.99999965374685,-19.0576713989215,
-10.501740395288));
#53885=CARTESIAN_POINT('Ctrl Pts',(-6.99999949863733,-18.9475466272878,
-10.4648905924172));
#53886=CARTESIAN_POINT('Ctrl Pts',(-6.99999938184507,-18.8384626319797,
-10.4264703291383));
#53887=CARTESIAN_POINT('Ctrl Pts',(-6.99999932344894,-18.7839206343257,
-10.4072601974988));
#53888=CARTESIAN_POINT('Ctrl Pts',(-6.99999927466345,-18.7296388307531,
-10.3876574507573));
#53889=CARTESIAN_POINT('Ctrl Pts',(-6.99999923547097,-18.6756218024774,
-10.3676699084702));
#53890=CARTESIAN_POINT('Ctrl Pts',(-6.99999921587473,-18.6486132883395,
-10.3576761373267));
#53891=CARTESIAN_POINT('Ctrl Pts',(-6.99999919867877,-18.6216709680258,
-10.3475861672968));
#53892=CARTESIAN_POINT('Ctrl Pts',(-6.99999918389284,-18.5947954063783,
-10.3374009714111));
#53893=CARTESIAN_POINT('Ctrl Pts',(-6.99999917282753,-18.574682595247,-10.3297786964287));
#53894=CARTESIAN_POINT('Ctrl Pts',(-6.99999916268429,-18.5536617939582,
-10.3217399904519));
#53895=CARTESIAN_POINT('Ctrl Pts',(-6.99999915445564,-18.5338561124317,
-10.3140994170821));
#53896=CARTESIAN_POINT('Ctrl Pts',(-6.99999915168883,-18.5271966314625,
-10.3115303435119));
#53897=CARTESIAN_POINT('Ctrl Pts',(-6.99999914912845,-18.5206743677,-10.3090067028305));
#53898=CARTESIAN_POINT('Ctrl Pts',(-6.999999146783,-18.514369557807,-10.3065606767057));
#53899=CARTESIAN_POINT('Ctrl Pts',(-6.99999907528804,-18.3221834138003,
-10.2319997720873));
#53900=CARTESIAN_POINT('Ctrl Pts',(-6.99999912491154,-18.129618500928,-10.1510712869352));
#53901=CARTESIAN_POINT('Ctrl Pts',(-6.99999933315392,-17.9371558589848,
-10.0634928398734));
#53902=CARTESIAN_POINT('Ctrl Pts',(-6.99999947285248,-17.8080430745273,
-10.0047411930891));
#53903=CARTESIAN_POINT('Ctrl Pts',(-6.99999968442919,-17.6789773237612,
-9.94299703195445));
#53904=CARTESIAN_POINT('Ctrl Pts',(-6.99999998816754,-17.5501167549105,
-9.87817779024853));
#53905=CARTESIAN_POINT('Ctrl Pts',(-7.0000004290411,-17.3630767616226,-9.78409322549982));
#53906=CARTESIAN_POINT('Ctrl Pts',(-7.00000106781896,-17.1764668647133,
-9.68352906351492));
#53907=CARTESIAN_POINT('Ctrl Pts',(-7.00000153332838,-16.9908087713364,
-9.57627873816244));
#53908=CARTESIAN_POINT('Ctrl Pts',(-7.00000199136873,-16.8081295564687,
-9.47074924104577));
#53909=CARTESIAN_POINT('Ctrl Pts',(-7.00000228134209,-16.6263718162228,
-9.35874636734403));
#53910=CARTESIAN_POINT('Ctrl Pts',(-7.00000202664203,-16.4460799745243,
-9.24008933015733));
#53911=CARTESIAN_POINT('Ctrl Pts',(-7.00000181210222,-16.2942159408053,
-9.14014173337999));
#53912=CARTESIAN_POINT('Ctrl Pts',(-7.00000121063474,-16.1433927337385,
-9.03547319345289));
#53913=CARTESIAN_POINT('Ctrl Pts',(-6.9999999866241,-15.9939628611808,-8.92598513115652));
#53914=CARTESIAN_POINT('Ctrl Pts',(-6.99999852879712,-15.8159881827653,
-8.79558213780594));
#53915=CARTESIAN_POINT('Ctrl Pts',(-6.99999617282013,-15.6399894215366,
-8.65834119823577));
#53916=CARTESIAN_POINT('Ctrl Pts',(-6.99999449839202,-15.4665325624122,
-8.51418171570541));
#53917=CARTESIAN_POINT('Ctrl Pts',(-6.99999284818661,-15.2955849730465,
-8.37210767984897));
#53918=CARTESIAN_POINT('Ctrl Pts',(-6.99999186150246,-15.1271062546936,
-8.22331377023279));
#53919=CARTESIAN_POINT('Ctrl Pts',(-6.99999320063255,-14.9616802774441,
-8.06775049235327));
#53920=CARTESIAN_POINT('Ctrl Pts',(-6.99999413393081,-14.8463876882616,
-7.9593316491543));
#53921=CARTESIAN_POINT('Ctrl Pts',(-6.99999620010739,-14.7325787767775,
-7.84762528725475));
#53922=CARTESIAN_POINT('Ctrl Pts',(-6.99999999965516,-14.6204636757736,
-7.73262300683288));
#53923=CARTESIAN_POINT('Ctrl Pts',(-7.00000506889282,-14.4708832189494,
-7.57919056564272));
#53924=CARTESIAN_POINT('Ctrl Pts',(-7.000013298643,-14.3243160482873,-7.4198896663707));
#53925=CARTESIAN_POINT('Ctrl Pts',(-7.0000165774608,-14.1813332730425,-7.25480434059693));
#53926=CARTESIAN_POINT('Ctrl Pts',(-7.00001838122332,-14.1026747488295,
-7.16398663145419));
#53927=CARTESIAN_POINT('Ctrl Pts',(-7.00001867169897,-14.0251016864707,
-7.07141891103329));
#53928=CARTESIAN_POINT('Ctrl Pts',(-7.00001598753963,-13.9487143147424,
-6.9771195452243));
#53929=CARTESIAN_POINT('Origin',(-5.9999949808,-24.1259380084106,-10.9277770011797));
#53930=CARTESIAN_POINT('Origin',(-6.,-24.1259427055448,-10.9277790621884));
#53931=CARTESIAN_POINT('Ctrl Pts',(-7.11139092859113,-15.2184460959384,
-5.12052280876705));
#53932=CARTESIAN_POINT('Ctrl Pts',(-7.11195855208738,-15.223719151167,-5.10426519075832));
#53933=CARTESIAN_POINT('Ctrl Pts',(-7.1136372886512,-15.2578366320999,-5.00059119811903));
#53934=CARTESIAN_POINT('Ctrl Pts',(-7.09280491237501,-15.3302302392258,
-4.7990182300767));
#53935=CARTESIAN_POINT('Ctrl Pts',(-7.00309038524378,-15.4434708112035,
-4.52630930653596));
#53936=CARTESIAN_POINT('Ctrl Pts',(-6.84623752314838,-15.5669468302129,
-4.27377175622976));
#53937=CARTESIAN_POINT('Ctrl Pts',(-6.63334306727782,-15.6888399309992,
-4.07033663875181));
#53938=CARTESIAN_POINT('Ctrl Pts',(-6.41901059637953,-15.7837928943819,
-3.95186938726383));
#53939=CARTESIAN_POINT('Ctrl Pts',(-6.28055126152101,-15.8346590679381,
-3.90855896005759));
#53940=CARTESIAN_POINT('Ctrl Pts',(-6.2306744828422,-15.8517787323193,-3.89680690069701));
#53941=CARTESIAN_POINT('Ctrl Pts',(-6.81161777639602,-14.6714606846117,
-4.93192660160615));
#53942=CARTESIAN_POINT('Ctrl Pts',(-6.81212328893671,-14.6760579235687,
-4.91772778087989));
#53943=CARTESIAN_POINT('Ctrl Pts',(-6.81362107184503,-14.7058456581685,
-4.82713697317831));
#53944=CARTESIAN_POINT('Ctrl Pts',(-6.79504003367809,-14.7695536197022,
-4.65054863615196));
#53945=CARTESIAN_POINT('Ctrl Pts',(-6.71482257063571,-14.8700027075903,
-4.41160379131102));
#53946=CARTESIAN_POINT('Ctrl Pts',(-6.57482808057142,-14.9798985601858,
-4.1910730559742));
#53947=CARTESIAN_POINT('Ctrl Pts',(-6.38564964768888,-15.0883124121041,
-4.01451732905237));
#53948=CARTESIAN_POINT('Ctrl Pts',(-6.19637626652847,-15.1724027362906,
-3.91259797704156));
#53949=CARTESIAN_POINT('Ctrl Pts',(-6.074854837314,-15.2171825715151,-3.87564777537514));
#53950=CARTESIAN_POINT('Ctrl Pts',(-6.03118272070632,-15.2322159785286,
-3.86565437501437));
#53951=CARTESIAN_POINT('Ctrl Pts',(-7.05013766657753,-14.0913326111332,
-4.75158252095379));
#53952=CARTESIAN_POINT('Ctrl Pts',(-7.05080210660599,-14.0972996850573,
-4.73318902546363));
#53953=CARTESIAN_POINT('Ctrl Pts',(-7.05275988231677,-14.1358643779999,
-4.61601626193555));
#53954=CARTESIAN_POINT('Ctrl Pts',(-7.02844934901559,-14.2172150025108,
-4.38943660681483));
#53955=CARTESIAN_POINT('Ctrl Pts',(-6.92428438305125,-14.3441879473141,
-4.08336733342954));
#53956=CARTESIAN_POINT('Ctrl Pts',(-6.74149011609023,-14.4833416388626,
-3.79856184173989));
#53957=CARTESIAN_POINT('Ctrl Pts',(-6.49116329395665,-14.6222984391297,
-3.56690077099674));
#53958=CARTESIAN_POINT('Ctrl Pts',(-6.23599489810763,-14.7324402085332,
-3.43022373396813));
#53959=CARTESIAN_POINT('Ctrl Pts',(-6.06915862423839,-14.7925192353585,
-3.37975541404639));
#53960=CARTESIAN_POINT('Ctrl Pts',(-6.00878489668786,-14.8128876803479,
-3.366032318725));
#53961=CARTESIAN_POINT('Ctrl Pts',(-7.66625772563486,-13.8781838194697,
-4.7040112511534));
#53962=CARTESIAN_POINT('Ctrl Pts',(-7.66719405941554,-13.8866359010153,
-4.67801897499989));
#53963=CARTESIAN_POINT('Ctrl Pts',(-7.66993998357738,-13.9411223884602,
-4.5126554880603));
#53964=CARTESIAN_POINT('Ctrl Pts',(-7.63581514365367,-14.0544598371705,
-4.19506349567618));
#53965=CARTESIAN_POINT('Ctrl Pts',(-7.49054162946217,-14.2292531573274,
-3.76657173189326));
#53966=CARTESIAN_POINT('Ctrl Pts',(-7.23439272786235,-14.4206227014939,
-3.36486723673259));
#53967=CARTESIAN_POINT('Ctrl Pts',(-6.87963590267719,-14.6133863806732,
-3.03354935884729));
#53968=CARTESIAN_POINT('Ctrl Pts',(-6.5124326609995,-14.7687834107463,-2.83442303682432));
#53969=CARTESIAN_POINT('Ctrl Pts',(-6.26884892595884,-14.8551443456087,
-2.75974286449289));
#53970=CARTESIAN_POINT('Ctrl Pts',(-6.18022691312438,-14.8846412572503,
-2.73933575737199));
#53971=CARTESIAN_POINT('',(-6.26386060036066,-15.8144217559011,-3.90573753028149));
#53972=CARTESIAN_POINT('',(-6.24994602117306,-14.8593867195859,-2.765467751532));
#53973=CARTESIAN_POINT('Ctrl Pts',(-6.26385652429609,-15.8144219194311,
-3.90575243311533));
#53974=CARTESIAN_POINT('Ctrl Pts',(-6.25434889993882,-15.7850152629862,
-3.90347479234289));
#53975=CARTESIAN_POINT('Ctrl Pts',(-6.24501694829635,-15.7549827955045,
-3.89975684459112));
#53976=CARTESIAN_POINT('Ctrl Pts',(-6.23596391386494,-15.7244969352914,
-3.89444911839014));
#53977=CARTESIAN_POINT('Ctrl Pts',(-6.22713722592631,-15.6947732910614,
-3.88927409744056));
#53978=CARTESIAN_POINT('Ctrl Pts',(-6.21857597188545,-15.6646189504095,
-3.88258712079457));
#53979=CARTESIAN_POINT('Ctrl Pts',(-6.21038173197456,-15.6342338906057,
-3.87427759589834));
#53980=CARTESIAN_POINT('Ctrl Pts',(-6.20231383173428,-15.6043173109158,
-3.86609618814901));
#53981=CARTESIAN_POINT('Ctrl Pts',(-6.1946020366201,-15.5741775227862,-3.85634126058895));
#53982=CARTESIAN_POINT('Ctrl Pts',(-6.18734459441452,-15.5440393360241,
-3.84494433544094));
#53983=CARTESIAN_POINT('Ctrl Pts',(-6.18021471889425,-15.5144308990662,
-3.83374773816641));
#53984=CARTESIAN_POINT('Ctrl Pts',(-6.1735236967773,-15.4848246440614,-3.82096592640214));
#53985=CARTESIAN_POINT('Ctrl Pts',(-6.16736111007851,-15.4554586832164,
-3.80657778903749));
#53986=CARTESIAN_POINT('Ctrl Pts',(-6.16656426144443,-15.4516615397551,
-3.8047173417665));
#53987=CARTESIAN_POINT('Ctrl Pts',(-6.16577623898295,-15.447868440501,-3.80283010325966));
#53988=CARTESIAN_POINT('Ctrl Pts',(-6.16499722734954,-15.4440799220539,
-3.80091608773727));
#53989=CARTESIAN_POINT('Ctrl Pts',(-6.15906489963985,-15.4152296045508,
-3.78634048086142));
#53990=CARTESIAN_POINT('Ctrl Pts',(-6.15365615351787,-15.3866443021748,
-3.77020801988018));
#53991=CARTESIAN_POINT('Ctrl Pts',(-6.14884557554313,-15.3585670169028,
-3.75255266407344));
#53992=CARTESIAN_POINT('Ctrl Pts',(-6.14409662647095,-15.3308494331651,
-3.73512349318845));
#53993=CARTESIAN_POINT('Ctrl Pts',(-6.13993089002222,-15.3036277392733,
-3.71621021877419));
#53994=CARTESIAN_POINT('Ctrl Pts',(-6.13640685600528,-15.2771366455292,
-3.69589448367759));
#53995=CARTESIAN_POINT('Ctrl Pts',(-6.1329035160769,-15.2508011147102,-3.67569804811645));
#53996=CARTESIAN_POINT('Ctrl Pts',(-6.13003458396478,-15.2251884341616,
-3.65411578637488));
#53997=CARTESIAN_POINT('Ctrl Pts',(-6.12784062593483,-15.2005180877307,
-3.63127496816577));
#53998=CARTESIAN_POINT('Ctrl Pts',(-6.12565411250769,-15.1759314534436,
-3.6085116540916));
#53999=CARTESIAN_POINT('Ctrl Pts',(-6.12413813899947,-15.1522815144872,
-3.58449873898918));
#54000=CARTESIAN_POINT('Ctrl Pts',(-6.1233133216665,-15.1297627974945,-3.55940429861102));
#54001=CARTESIAN_POINT('Ctrl Pts',(-6.1224892469612,-15.107264355321,-3.53433245211507));
#54002=CARTESIAN_POINT('Ctrl Pts',(-6.1223551290373,-15.0858957220768,-3.50818164249182));
#54003=CARTESIAN_POINT('Ctrl Pts',(-6.12291059718962,-15.0658178438706,
-3.48115374423421));
#54004=CARTESIAN_POINT('Ctrl Pts',(-6.12346877188963,-15.0456421351504,
-3.45399415112549));
#54005=CARTESIAN_POINT('Ctrl Pts',(-6.12472322579646,-15.0267702666732,
-3.4259496505214));
#54006=CARTESIAN_POINT('Ctrl Pts',(-6.12665239297863,-15.0093237705288,
-3.39724939775243));
#54007=CARTESIAN_POINT('Ctrl Pts',(-6.12858902383243,-14.9918097763886,
-3.36843810781452));
#54008=CARTESIAN_POINT('Ctrl Pts',(-6.13120544722315,-14.975732443847,-3.3389668257281));
#54009=CARTESIAN_POINT('Ctrl Pts',(-6.13446002689163,-14.9611673003063,
-3.30907972141196));
#54010=CARTESIAN_POINT('Ctrl Pts',(-6.13775200151227,-14.9464348040192,
-3.27884921581207));
#54011=CARTESIAN_POINT('Ctrl Pts',(-6.1416966582409,-14.9332494960981,-3.24819414394665));
#54012=CARTESIAN_POINT('Ctrl Pts',(-6.14623348971912,-14.9216388079144,
-3.21736676232502));
#54013=CARTESIAN_POINT('Ctrl Pts',(-6.14953766811315,-14.9131827334006,
-3.19491515291709));
#54014=CARTESIAN_POINT('Ctrl Pts',(-6.15315556109662,-14.9055607658247,
-3.17237216667401));
#54015=CARTESIAN_POINT('Ctrl Pts',(-6.15705925816722,-14.8987671910623,
-3.14983127721761));
#54016=CARTESIAN_POINT('Ctrl Pts',(-6.16251488973931,-14.8892727963152,
-3.11832914322578));
#54017=CARTESIAN_POINT('Ctrl Pts',(-6.16852868281514,-14.8813980812299,
-3.08683240633574));
#54018=CARTESIAN_POINT('Ctrl Pts',(-6.17501497441148,-14.8750872662013,
-3.0555762596843));
#54019=CARTESIAN_POINT('Ctrl Pts',(-6.18164965391719,-14.8686320776684,
-3.02360506126752));
#54020=CARTESIAN_POINT('Ctrl Pts',(-6.18877834589665,-14.8638126550383,
-2.99188622572886));
#54021=CARTESIAN_POINT('Ctrl Pts',(-6.19630368712461,-14.8605266126875,
-2.96063793694244));
#54022=CARTESIAN_POINT('Ctrl Pts',(-6.2039405004092,-14.8571918945508,-2.92892677067158));
#54023=CARTESIAN_POINT('Ctrl Pts',(-6.21198544673472,-14.8554356045965,
-2.89770057631721));
#54024=CARTESIAN_POINT('Ctrl Pts',(-6.22033644639755,-14.8551167953603,
-2.86714542587604));
#54025=CARTESIAN_POINT('Ctrl Pts',(-6.22888773877028,-14.8547903397142,
-2.83585743216696));
#54026=CARTESIAN_POINT('Ctrl Pts',(-6.23775961330328,-14.8559703733874,
-2.8052732725674));
#54027=CARTESIAN_POINT('Ctrl Pts',(-6.24684741590646,-14.8584816777926,
-2.77554433674993));
#54028=CARTESIAN_POINT('Ctrl Pts',(-6.24787754516983,-14.8587663415634,
-2.77217447407888));
#54029=CARTESIAN_POINT('Ctrl Pts',(-6.24891045694085,-14.8590680933294,
-2.76881554859793));
#54030=CARTESIAN_POINT('Ctrl Pts',(-6.24994600541046,-14.8593866659903,
-2.76546774155524));
#54031=CARTESIAN_POINT('',(-7.00000000902828,-14.5427410186974,-3.16613136210122));
#54032=CARTESIAN_POINT('Ctrl Pts',(-7.00000002511356,-14.542739937087,-3.16613069231016));
#54033=CARTESIAN_POINT('Ctrl Pts',(-6.96011600416233,-14.5636692275086,
-3.13137525098935));
#54034=CARTESIAN_POINT('Ctrl Pts',(-6.91914513183867,-14.584253870872,-3.09860123268627));
#54035=CARTESIAN_POINT('Ctrl Pts',(-6.8771519201577,-14.604510166625,-3.06774662680443));
#54036=CARTESIAN_POINT('Ctrl Pts',(-6.87107538686914,-14.6074413083624,
-3.0632818804266));
#54037=CARTESIAN_POINT('Ctrl Pts',(-6.86497736856078,-14.6103655792405,
-3.05885736617627));
#54038=CARTESIAN_POINT('Ctrl Pts',(-6.85885798311168,-14.6132830322912,
-3.05447294022931));
#54039=CARTESIAN_POINT('Ctrl Pts',(-6.81631977316428,-14.6335633743967,
-3.02399510336446));
#54040=CARTESIAN_POINT('Ctrl Pts',(-6.77275254603296,-14.6535142578584,
-2.99545177547727));
#54041=CARTESIAN_POINT('Ctrl Pts',(-6.72820659561677,-14.673148951286,-2.96879836373911));
#54042=CARTESIAN_POINT('Ctrl Pts',(-6.70154365414986,-14.6849012806603,
-2.95284498637419));
#54043=CARTESIAN_POINT('Ctrl Pts',(-6.6745292329114,-14.6965403430539,-2.93756929117119));
#54044=CARTESIAN_POINT('Ctrl Pts',(-6.64716751507883,-14.708068749641,-2.92296767350332));
#54045=CARTESIAN_POINT('Ctrl Pts',(-6.60219121491642,-14.7270187687235,
-2.89896601019018));
#54046=CARTESIAN_POINT('Ctrl Pts',(-6.55628914166064,-14.7456653224943,
-2.87678981055785));
#54047=CARTESIAN_POINT('Ctrl Pts',(-6.50944454425378,-14.7640218520635,
-2.85644737493458));
#54048=CARTESIAN_POINT('Ctrl Pts',(-6.48523668037748,-14.7735079485112,
-2.84593502260923));
#54049=CARTESIAN_POINT('Ctrl Pts',(-6.46077662967747,-14.7829165125535,
-2.8359130621748));
#54050=CARTESIAN_POINT('Ctrl Pts',(-6.43605934025051,-14.7922487267942,
-2.82638732690259));
#54051=CARTESIAN_POINT('Ctrl Pts',(-6.38889531125482,-14.8100558906559,
-2.80821089797369));
#54052=CARTESIAN_POINT('Ctrl Pts',(-6.34079553367693,-14.8275856751904,
-2.79183826000356));
#54053=CARTESIAN_POINT('Ctrl Pts',(-6.29174550793962,-14.8448349818748,
-2.77732265229406));
#54054=CARTESIAN_POINT('Ctrl Pts',(-6.27788844248412,-14.8497080633502,
-2.77322186492171));
#54055=CARTESIAN_POINT('Ctrl Pts',(-6.26395544574025,-14.8545586992195,
-2.76926958738593));
#54056=CARTESIAN_POINT('Ctrl Pts',(-6.24994600541046,-14.8593866659903,
-2.76546774155524));
#54057=CARTESIAN_POINT('',(-7.00001088476076,-14.7967989998614,-4.92966193866457));
#54058=CARTESIAN_POINT('Ctrl Pts',(-7.,-14.796798999896,-4.92966193873101));
#54059=CARTESIAN_POINT('Ctrl Pts',(-7.,-14.7449205055658,-4.79939605137961));
#54060=CARTESIAN_POINT('Ctrl Pts',(-7.,-14.7001933080234,-4.67547153146728));
#54061=CARTESIAN_POINT('Ctrl Pts',(-7.,-14.6626174072688,-4.55788837899402));
#54062=CARTESIAN_POINT('Ctrl Pts',(-7.,-14.6500921070173,-4.51869399483627));
#54063=CARTESIAN_POINT('Ctrl Pts',(-7.,-14.6389128416482,-4.48210949886636));
#54064=CARTESIAN_POINT('Ctrl Pts',(-7.,-14.6274252721102,-4.44241901566712));
#54065=CARTESIAN_POINT('Ctrl Pts',(-7.,-14.5814749939582,-4.28365708287018));
#54066=CARTESIAN_POINT('Ctrl Pts',(-7.,-14.5473536100588,-4.12819986609514));
#54067=CARTESIAN_POINT('Ctrl Pts',(-7.,-14.5258257394674,-3.98126610507176));
#54068=CARTESIAN_POINT('Ctrl Pts',(-7.,-14.4827699982847,-3.68739858302502));
#54069=CARTESIAN_POINT('Ctrl Pts',(-7.,-14.4884084168554,-3.41568714349165));
#54070=CARTESIAN_POINT('Ctrl Pts',(-7.,-14.5427409951797,-3.16613178647166));
#54071=CARTESIAN_POINT('Ctrl Pts',(-7.00001663766714,-14.7967989999222,
-4.92966193871151));
#54072=CARTESIAN_POINT('Ctrl Pts',(-7.00001663809637,-14.7975367734645,
-4.92865411678288));
#54073=CARTESIAN_POINT('Ctrl Pts',(-7.00001534769258,-14.7982733606461,
-4.9276484327044));
#54074=CARTESIAN_POINT('Ctrl Pts',(-7.000012781729,-14.7990087562765,-4.92664488855557));
#54075=CARTESIAN_POINT('Ctrl Pts',(-6.99994577229626,-14.8182134107743,
-4.90043760929783));
#54076=CARTESIAN_POINT('Ctrl Pts',(-6.99901241540824,-14.83660348244,-4.87569190868736));
#54077=CARTESIAN_POINT('Ctrl Pts',(-6.99748340315736,-14.8541002168799,
-4.85241809457354));
#54078=CARTESIAN_POINT('Ctrl Pts',(-6.99586198477726,-14.8726543695993,
-4.82773772333545));
#54079=CARTESIAN_POINT('Ctrl Pts',(-6.99357070413138,-14.8902040910381,
-4.80471221012978));
#54080=CARTESIAN_POINT('Ctrl Pts',(-6.99088477554742,-14.9066808349925,
-4.78332681937195));
#54081=CARTESIAN_POINT('Ctrl Pts',(-6.98885340324955,-14.9191422241106,
-4.76715301243458));
#54082=CARTESIAN_POINT('Ctrl Pts',(-6.98659528081006,-14.9309904422388,
-4.75191671818498));
#54083=CARTESIAN_POINT('Ctrl Pts',(-6.98421315519464,-14.9422037188569,
-4.73760410263847));
#54084=CARTESIAN_POINT('Ctrl Pts',(-6.98193649879244,-14.9529205248208,
-4.72392518175988));
#54085=CARTESIAN_POINT('Ctrl Pts',(-6.97954644605706,-14.9630574726601,
-4.71108984384714));
#54086=CARTESIAN_POINT('Ctrl Pts',(-6.97712173274568,-14.9726001913429,
-4.69908246542887));
#54087=CARTESIAN_POINT('Ctrl Pts',(-6.97495841148752,-14.9811141736312,
-4.68836952181397));
#54088=CARTESIAN_POINT('Ctrl Pts',(-6.97276741258127,-14.9891552339856,
-4.67831550295479));
#54089=CARTESIAN_POINT('Ctrl Pts',(-6.97059882000231,-14.9967157329114,
-4.66890728451756));
#54090=CARTESIAN_POINT('Ctrl Pts',(-6.96829921293241,-15.0047329957899,
-4.65893067303073));
#54091=CARTESIAN_POINT('Ctrl Pts',(-6.96602484765305,-15.0122098870659,
-4.64968020175899));
#54092=CARTESIAN_POINT('Ctrl Pts',(-6.96382697423633,-15.0191395327482,
-4.64114030304257));
#54093=CARTESIAN_POINT('Ctrl Pts',(-6.96272803752797,-15.0226043555894,
-4.63687035368436));
#54094=CARTESIAN_POINT('Ctrl Pts',(-6.96164809842778,-15.0259323699146,
-4.63277808260133));
#54095=CARTESIAN_POINT('Ctrl Pts',(-6.96059277771306,-15.0291229292358,
-4.62886157934885));
#54096=CARTESIAN_POINT('Ctrl Pts',(-6.9600651173557,-15.0307182088964,-4.6269033277226));
#54097=CARTESIAN_POINT('Ctrl Pts',(-6.95954360389157,-15.0322791249762,
-4.62498902010119));
#54098=CARTESIAN_POINT('Ctrl Pts',(-6.95902889420468,-15.033805600673,-4.62311842999734));
#54099=CARTESIAN_POINT('Ctrl Pts',(-6.95877153936123,-15.0345688385214,
-4.62218313494541));
#54100=CARTESIAN_POINT('Ctrl Pts',(-6.95851588499231,-15.0353234662854,
-4.62125876941255));
#54101=CARTESIAN_POINT('Ctrl Pts',(-6.95826201026872,-15.0360694750285,
-4.62034530544564));
#54102=CARTESIAN_POINT('Ctrl Pts',(-6.95813507290692,-15.0364424794,-4.61988857346219));
#54103=CARTESIAN_POINT('Ctrl Pts',(-6.95807521070884,-15.0366179364207,
-4.61967379541748));
#54104=CARTESIAN_POINT('Ctrl Pts',(-6.95798268246544,-15.0368889292216,
-4.61934206723523));
#54105=CARTESIAN_POINT('Ctrl Pts',(-6.95789015422205,-15.0371599220225,
-4.61901033905299));
#54106=CARTESIAN_POINT('Ctrl Pts',(-6.95776511469508,-15.0375264468331,
-4.61856161381191));
#54107=CARTESIAN_POINT('Ctrl Pts',(-6.95750580230632,-15.038281635463,-4.61763759073908));
#54108=CARTESIAN_POINT('Ctrl Pts',(-6.94614005914319,-15.0713817894802,
-4.57713737024271));
#54109=CARTESIAN_POINT('Ctrl Pts',(-6.9327462899655,-15.1039951502087,-4.53816352059833));
#54110=CARTESIAN_POINT('Ctrl Pts',(-6.91760941176288,-15.1359960352447,
-4.50084476430815));
#54111=CARTESIAN_POINT('Ctrl Pts',(-6.91219238734351,-15.1474481704446,
-4.48748952609994));
#54112=CARTESIAN_POINT('Ctrl Pts',(-6.90655172950781,-15.1588220949498,
-4.47434605023249));
#54113=CARTESIAN_POINT('Ctrl Pts',(-6.90069928966027,-15.1701127885821,
-4.46141953274621));
#54114=CARTESIAN_POINT('Ctrl Pts',(-6.89902619990268,-15.1733405609923,
-4.4577241126187));
#54115=CARTESIAN_POINT('Ctrl Pts',(-6.89733579847696,-15.1765615335403,
-4.45404642133306));
#54116=CARTESIAN_POINT('Ctrl Pts',(-6.89562842115357,-15.1797756007415,
-4.45038651876726));
#54117=CARTESIAN_POINT('Ctrl Pts',(-6.88344418924519,-15.2027119134196,
-4.42426862378707));
#54118=CARTESIAN_POINT('Ctrl Pts',(-6.87039641764602,-15.2252960975963,
-4.3990569651195));
#54119=CARTESIAN_POINT('Ctrl Pts',(-6.85660014356463,-15.2474931839915,
-4.37477093617939));
#54120=CARTESIAN_POINT('Ctrl Pts',(-6.84970200652394,-15.258591727189,-4.36262792170933));
#54121=CARTESIAN_POINT('Ctrl Pts',(-6.8426166363207,-15.2695934999198,-4.35071638136407));
#54122=CARTESIAN_POINT('Ctrl Pts',(-6.83535729734611,-15.2804947496512,
-4.33903818947538));
#54123=CARTESIAN_POINT('Ctrl Pts',(-6.83172762785882,-15.285945374517,-4.33319909353104));
#54124=CARTESIAN_POINT('Ctrl Pts',(-6.8280544601488,-15.2913708688442,-4.32741833799953));
#54125=CARTESIAN_POINT('Ctrl Pts',(-6.82433940590007,-15.2967707803477,
-4.32169615217796));
#54126=CARTESIAN_POINT('Ctrl Pts',(-6.82173742230159,-15.3005528196464,
-4.31768839545131));
#54127=CARTESIAN_POINT('Ctrl Pts',(-6.8193564466768,-15.3039769310697,-4.31407383849168));
#54128=CARTESIAN_POINT('Ctrl Pts',(-6.81669076362756,-15.3077687266043,
-4.31008576083222));
#54129=CARTESIAN_POINT('Ctrl Pts',(-6.81555044377055,-15.3093907723097,
-4.30837975000409));
#54130=CARTESIAN_POINT('Ctrl Pts',(-6.81435755445571,-15.3110800798102,
-4.30660574250561));
#54131=CARTESIAN_POINT('Ctrl Pts',(-6.8130701686411,-15.3128933243765,-4.30470553027457));
#54132=CARTESIAN_POINT('Ctrl Pts',(-6.79825969502292,-15.3337534352373,
-4.28284491724214));
#54133=CARTESIAN_POINT('Ctrl Pts',(-6.78272730742013,-15.354374326057,-4.26171751977155));
#54134=CARTESIAN_POINT('Ctrl Pts',(-6.76652828469596,-15.3747298948658,
-4.24136254811858));
#54135=CARTESIAN_POINT('Ctrl Pts',(-6.7355636332618,-15.4136398404618,-4.20245374399387));
#54136=CARTESIAN_POINT('Ctrl Pts',(-6.70216661465935,-15.4515790298085,
-4.16636672048905));
#54137=CARTESIAN_POINT('Ctrl Pts',(-6.66680173141148,-15.4883912322177,
-4.13326346432175));
#54138=CARTESIAN_POINT('Ctrl Pts',(-6.63958886664646,-15.5167177921796,
-4.10779089519013));
#54139=CARTESIAN_POINT('Ctrl Pts',(-6.61120949516485,-15.5443775351441,
-4.08408532659129));
#54140=CARTESIAN_POINT('Ctrl Pts',(-6.58185638319706,-15.5713077873573,
-4.06222104642336));
#54141=CARTESIAN_POINT('Ctrl Pts',(-6.54207699837613,-15.6078037087195,
-4.03259053857168));
#54142=CARTESIAN_POINT('Ctrl Pts',(-6.50051151132605,-15.6429592491191,
-4.0063409416901));
#54143=CARTESIAN_POINT('Ctrl Pts',(-6.45769611140315,-15.6766488500718,
-3.98352821426703));
#54144=CARTESIAN_POINT('Ctrl Pts',(-6.42609327516521,-15.7015157658018,
-3.96668971946865));
#54145=CARTESIAN_POINT('Ctrl Pts',(-6.39380826821476,-15.7255844436343,
-3.95172398635191));
#54146=CARTESIAN_POINT('Ctrl Pts',(-6.36104005522242,-15.7488112379618,
-3.93865360293187));
#54147=CARTESIAN_POINT('Ctrl Pts',(-6.32903948906336,-15.7714939081676,
-3.92588941376309));
#54148=CARTESIAN_POINT('Ctrl Pts',(-6.29657817025406,-15.7933737950221,
-3.91493248274305));
#54149=CARTESIAN_POINT('Ctrl Pts',(-6.26385652444153,-15.8144219193375,
-3.90575243315613));
#54150=CARTESIAN_POINT('Ctrl Pts',(-6.22266927200468,-14.5714076497178,
-3.97375074908438));
#54151=CARTESIAN_POINT('Ctrl Pts',(-6.22400481395816,-14.9771466562601,
-3.92718887782356));
#54152=CARTESIAN_POINT('Ctrl Pts',(-6.22726440271229,-16.0460349078152,
-3.85976027256915));
#54153=CARTESIAN_POINT('Ctrl Pts',(-6.23205292877977,-17.7794285729011,
-3.98191084033141));
#54154=CARTESIAN_POINT('Ctrl Pts',(-6.23570674183347,-19.7179592036766,
-4.44990468744485));
#54155=CARTESIAN_POINT('Ctrl Pts',(-6.23759590828025,-21.5545920913375,
-5.23225281484869));
#54156=CARTESIAN_POINT('Ctrl Pts',(-6.23804310410169,-23.2351578294011,
-6.30682863397947));
#54157=CARTESIAN_POINT('Ctrl Pts',(-6.2364962539807,-24.5993870470491,-7.54006269483624));
#54158=CARTESIAN_POINT('Ctrl Pts',(-6.23490846670046,-25.3447857086981,
-8.44425797847651));
#54159=CARTESIAN_POINT('Ctrl Pts',(-6.23413317444848,-25.6421043947626,
-8.85534264102317));
#54160=CARTESIAN_POINT('Ctrl Pts',(-6.71589077441495,-14.5843362145528,
-4.08566013088855));
#54161=CARTESIAN_POINT('Ctrl Pts',(-6.71707950162014,-14.9863211817523,
-4.04021329081558));
#54162=CARTESIAN_POINT('Ctrl Pts',(-6.7199340298597,-16.0451951223557,-3.97507849086041));
#54163=CARTESIAN_POINT('Ctrl Pts',(-6.72416488025816,-17.7615742587119,
-4.09849304259662));
#54164=CARTESIAN_POINT('Ctrl Pts',(-6.72736853924326,-19.6804278393728,
-4.5636779526249));
#54165=CARTESIAN_POINT('Ctrl Pts',(-6.72902459162388,-21.4982069937746,
-5.33903826408915));
#54166=CARTESIAN_POINT('Ctrl Pts',(-6.72941958809745,-23.1617854706901,
-6.40302993263691));
#54167=CARTESIAN_POINT('Ctrl Pts',(-6.72805205550861,-24.5127345552137,
-7.62318907122469));
#54168=CARTESIAN_POINT('Ctrl Pts',(-6.72668378134466,-25.2513986694556,
-8.51793692454479));
#54169=CARTESIAN_POINT('Ctrl Pts',(-6.72599063608826,-25.5460990905114,
-8.924725493994));
#54170=CARTESIAN_POINT('Ctrl Pts',(-7.02184867179209,-14.6305390362147,
-4.48559661493872));
#54171=CARTESIAN_POINT('Ctrl Pts',(-7.02249163003048,-15.0188785470189,
-4.44215144359658));
#54172=CARTESIAN_POINT('Ctrl Pts',(-7.02397829161063,-16.041923997109,-4.38032116097713));
#54173=CARTESIAN_POINT('Ctrl Pts',(-7.02622832902972,-17.6995302278369,
-4.50113419981309));
#54174=CARTESIAN_POINT('Ctrl Pts',(-7.02790167456001,-19.5522397357699,
-4.95159520695056));
#54175=CARTESIAN_POINT('Ctrl Pts',(-7.02876621306822,-21.3070950890534,
-5.70076885107868));
#54176=CARTESIAN_POINT('Ctrl Pts',(-7.02897613242694,-22.9136310478051,
-6.72847731338896));
#54177=CARTESIAN_POINT('Ctrl Pts',(-7.02824783070861,-24.2181462496305,
-7.9059965921817));
#54178=CARTESIAN_POINT('Ctrl Pts',(-7.02756288622409,-24.9320744273322,
-8.76993223223512));
#54179=CARTESIAN_POINT('Ctrl Pts',(-7.02718420231269,-25.2168998853482,
-9.16263757723443));
#54180=CARTESIAN_POINT('Ctrl Pts',(-6.99898915412836,-14.6884801947993,
-4.9871430090862));
#54181=CARTESIAN_POINT('Ctrl Pts',(-6.99894179669343,-15.0596433779913,
-4.94565457308912));
#54182=CARTESIAN_POINT('Ctrl Pts',(-6.99873531344683,-16.0377464552832,
-4.88660278316425));
#54183=CARTESIAN_POINT('Ctrl Pts',(-6.998504682319,-17.6222149766872,-5.00216659369601));
#54184=CARTESIAN_POINT('Ctrl Pts',(-6.99828080313596,-19.3931412309868,
-5.43285519773799));
#54185=CARTESIAN_POINT('Ctrl Pts',(-6.99816433582362,-21.0703293317465,
-6.14885025581044));
#54186=CARTESIAN_POINT('Ctrl Pts',(-6.998142566822,-22.6063533391169,-7.13148755499935));
#54187=CARTESIAN_POINT('Ctrl Pts',(-6.99821545410715,-23.8529237850754,
-8.25667423059523));
#54188=CARTESIAN_POINT('Ctrl Pts',(-6.99835921778234,-24.5356449630949,
-9.08279282694947));
#54189=CARTESIAN_POINT('Ctrl Pts',(-6.99838071861337,-24.8079420244304,
-9.45819132371699));
#54190=CARTESIAN_POINT('',(-7.00000355772207,-24.7867164860314,-9.33251602987223));
#54191=CARTESIAN_POINT('Ctrl Pts',(-7.00001601661514,-14.7967989997676,
-4.92966193854915));
#54192=CARTESIAN_POINT('Ctrl Pts',(-7.00002088999496,-15.0161849076412,
-4.90663942338753));
#54193=CARTESIAN_POINT('Ctrl Pts',(-7.00001598309289,-15.2342923928345,
-4.89043249278858));
#54194=CARTESIAN_POINT('Ctrl Pts',(-7.00000988157662,-15.4506295864929,
-4.88069445257409));
#54195=CARTESIAN_POINT('Ctrl Pts',(-7.00000652467729,-15.5696528173402,
-4.87533683011053));
#54196=CARTESIAN_POINT('Ctrl Pts',(-7.00000279094495,-15.6881411279891,
-4.87193736278651));
#54197=CARTESIAN_POINT('Ctrl Pts',(-6.99999999965555,-15.8060192824143,
-4.87043886254274));
#54198=CARTESIAN_POINT('Ctrl Pts',(-6.99999455422801,-16.0359835948731,
-4.86751549154191));
#54199=CARTESIAN_POINT('Ctrl Pts',(-6.99999266081081,-16.2636228788866,
-4.87182624541992));
#54200=CARTESIAN_POINT('Ctrl Pts',(-6.99999257345303,-16.4885261114551,
-4.88291895400832));
#54201=CARTESIAN_POINT('Ctrl Pts',(-6.99999248483031,-16.7166859233864,
-4.89417228405802));
#54202=CARTESIAN_POINT('Ctrl Pts',(-6.99999425319372,-16.9420299260002,
-4.91240537065293));
#54203=CARTESIAN_POINT('Ctrl Pts',(-6.99999619757822,-17.1641819043159,
-4.93715669708171));
#54204=CARTESIAN_POINT('Ctrl Pts',(-6.99999754424684,-17.3180429828072,
-4.95429931182364));
#54205=CARTESIAN_POINT('Ctrl Pts',(-6.99999897835409,-17.4703740013657,
-4.97456885757716));
#54206=CARTESIAN_POINT('Ctrl Pts',(-6.99999998662334,-17.6210642719037,
-4.99781499900363));
#54207=CARTESIAN_POINT('Ctrl Pts',(-7.00000143709259,-17.8378432762666,
-5.03125627809693));
#54208=CARTESIAN_POINT('Ctrl Pts',(-7.00000201442373,-18.051224743139,-5.07085612413644));
#54209=CARTESIAN_POINT('Ctrl Pts',(-7.00000210876075,-18.260914284654,-5.11608683430385));
#54210=CARTESIAN_POINT('Ctrl Pts',(-7.00000220461189,-18.4739693834249,
-5.16204350602229));
#54211=CARTESIAN_POINT('Ctrl Pts',(-7.00000180217035,-18.6832131501843,
-5.21381323096648));
#54212=CARTESIAN_POINT('Ctrl Pts',(-7.00000129011946,-18.8883856688076,
-5.27086615566158));
#54213=CARTESIAN_POINT('Ctrl Pts',(-7.00000086167035,-19.0600599782347,
-5.31860413496579));
#54214=CARTESIAN_POINT('Ctrl Pts',(-7.00000035619256,-19.2288848433898,
-5.37004141745854));
#54215=CARTESIAN_POINT('Ctrl Pts',(-6.99999998816687,-19.3947330689617,
-5.42488007160696));
#54216=CARTESIAN_POINT('Ctrl Pts',(-6.9999997037335,-19.5229109953601,-5.46726282819648));
#54217=CARTESIAN_POINT('Ctrl Pts',(-6.99999950019772,-19.6493114378435,
-5.51167745875434));
#54218=CARTESIAN_POINT('Ctrl Pts',(-6.99999936067303,-19.7738903396788,
-5.55798426808907));
#54219=CARTESIAN_POINT('Ctrl Pts',(-6.99999924478735,-19.8773624232099,
-5.59644553217921));
#54220=CARTESIAN_POINT('Ctrl Pts',(-6.99999917321298,-19.9795780416209,
-5.63621220749404));
#54221=CARTESIAN_POINT('Ctrl Pts',(-6.99999913936349,-20.0805155867661,
-5.67720662381942));
#54222=CARTESIAN_POINT('Ctrl Pts',(-6.99999912243875,-20.1309843593387,
-5.69770383198211));
#54223=CARTESIAN_POINT('Ctrl Pts',(-6.99999911498657,-20.1811336135949,
-5.71850797539744));
#54224=CARTESIAN_POINT('Ctrl Pts',(-6.9999991163999,-20.2309610063002,-5.73960958184171));
#54225=CARTESIAN_POINT('Ctrl Pts',(-6.99999911710657,-20.2558747026529,
-5.75016038506384));
#54226=CARTESIAN_POINT('Ctrl Pts',(-6.99999912003181,-20.2807079336179,
-5.76078555404321));
#54227=CARTESIAN_POINT('Ctrl Pts',(-6.99999912511196,-20.3054604155709,
-5.77148391108337));
#54228=CARTESIAN_POINT('Ctrl Pts',(-6.99999912765204,-20.3178366565475,
-5.77683308960345));
#54229=CARTESIAN_POINT('Ctrl Pts',(-6.99999913073096,-20.330192710271,-5.78220056513874));
#54230=CARTESIAN_POINT('Ctrl Pts',(-6.99999913434146,-20.3425285425323,
-5.78758619130768));
#54231=CARTESIAN_POINT('Ctrl Pts',(-6.99999913749777,-20.3533125294659,
-5.79229430673962));
#54232=CARTESIAN_POINT('Ctrl Pts',(-6.99999914056829,-20.3627039949546,
-5.79641054026109));
#54233=CARTESIAN_POINT('Ctrl Pts',(-6.99999914483357,-20.3743145101157,
-5.80152322606212));
#54234=CARTESIAN_POINT('Ctrl Pts',(-6.99999914544735,-20.3759852951245,
-5.802258955586));
#54235=CARTESIAN_POINT('Ctrl Pts',(-6.99999914608783,-20.3777019974094,
-5.80301539887061));
#54236=CARTESIAN_POINT('Ctrl Pts',(-6.99999914676092,-20.3794753410883,
-5.80379737558169));
#54237=CARTESIAN_POINT('Ctrl Pts',(-6.99999923697264,-20.6171481358953,
-5.90860198430455));
#54238=CARTESIAN_POINT('Ctrl Pts',(-6.99999952144547,-20.8492773499208,
-6.02101208188487));
#54239=CARTESIAN_POINT('Ctrl Pts',(-6.99999999018442,-21.0754641488202,
-6.14041758832291));
#54240=CARTESIAN_POINT('Ctrl Pts',(-7.00000044364504,-21.2942784891113,
-6.25593112512301));
#54241=CARTESIAN_POINT('Ctrl Pts',(-7.00000106797113,-21.5075320214405,
-6.37799078394024));
#54242=CARTESIAN_POINT('Ctrl Pts',(-7.00000142593302,-21.7149314703275,
-6.50595747362906));
#54243=CARTESIAN_POINT('Ctrl Pts',(-7.00000178765839,-21.9245114365704,
-6.63526955545526));
#54244=CARTESIAN_POINT('Ctrl Pts',(-7.0000018762758,-22.1281136184752,-6.77061353997294));
#54245=CARTESIAN_POINT('Ctrl Pts',(-7.0000013155977,-22.325477297402,-6.91136295359017));
#54246=CARTESIAN_POINT('Ctrl Pts',(-7.0000010387387,-22.4229341272705,-6.98086404787235));
#54247=CARTESIAN_POINT('Ctrl Pts',(-7.00000060481352,-22.5188704490222,
-7.05168366000249));
#54248=CARTESIAN_POINT('Ctrl Pts',(-6.999999976358,-22.6132585283086,-7.12374926523835));
#54249=CARTESIAN_POINT('Ctrl Pts',(-6.99999887928019,-22.7780292468715,
-7.24955224426024));
#54250=CARTESIAN_POINT('Ctrl Pts',(-6.99999719586383,-22.9380810757636,
-7.3791511577127));
#54251=CARTESIAN_POINT('Ctrl Pts',(-6.99999590263445,-23.0933375024812,
-7.51215861203649));
#54252=CARTESIAN_POINT('Ctrl Pts',(-6.99999568171304,-23.1198598429666,
-7.53488017703224));
#54253=CARTESIAN_POINT('Ctrl Pts',(-6.99999546002068,-23.1476959266424,
-7.55895202597045));
#54254=CARTESIAN_POINT('Ctrl Pts',(-6.99999525388502,-23.175812124434,-7.58352663462908));
#54255=CARTESIAN_POINT('Ctrl Pts',(-6.9999951202971,-23.1940330588923,-7.59945241296604));
#54256=CARTESIAN_POINT('Ctrl Pts',(-6.9999949932363,-23.2123722665019,-7.61558857541806));
#54257=CARTESIAN_POINT('Ctrl Pts',(-6.99999487630671,-23.2305561250311,
-7.63169548141941));
#54258=CARTESIAN_POINT('Ctrl Pts',(-6.99999457894647,-23.2767989705564,
-7.67265648894783));
#54259=CARTESIAN_POINT('Ctrl Pts',(-6.99999434327551,-23.3225495659397,
-7.71387576700431));
#54260=CARTESIAN_POINT('Ctrl Pts',(-6.99999419420459,-23.3678081332012,
-7.75534001206123));
#54261=CARTESIAN_POINT('Ctrl Pts',(-6.99999365475073,-23.5315886342942,
-7.9053897207413));
#54262=CARTESIAN_POINT('Ctrl Pts',(-6.99999426200425,-23.6889263430828,
-8.05864816970276));
#54263=CARTESIAN_POINT('Ctrl Pts',(-6.99999708872154,-23.8398710235771,
-8.21453737949556));
#54264=CARTESIAN_POINT('Ctrl Pts',(-6.99999738650744,-23.8557725776303,
-8.23095982437877));
#54265=CARTESIAN_POINT('Ctrl Pts',(-6.99999770877207,-23.8716032104523,
-8.24741150351764));
#54266=CARTESIAN_POINT('Ctrl Pts',(-6.99999805666162,-23.8873630000909,
-8.26389176796206));
#54267=CARTESIAN_POINT('Ctrl Pts',(-6.99999863110494,-23.9133859316887,
-8.29110436433449));
#54268=CARTESIAN_POINT('Ctrl Pts',(-6.99999927542365,-23.9392157050888,
-8.31839489775144));
#54269=CARTESIAN_POINT('Ctrl Pts',(-6.99999999465528,-23.9648526940703,
-8.3457604773189));
#54270=CARTESIAN_POINT('Ctrl Pts',(-7.00000393348073,-24.105252005446,-8.49562630319423));
#54271=CARTESIAN_POINT('Ctrl Pts',(-7.00001006470838,-24.2398674196823,
-8.64773911793527));
#54272=CARTESIAN_POINT('Ctrl Pts',(-7.00001375740975,-24.368761885244,-8.80154981297568));
#54273=CARTESIAN_POINT('Ctrl Pts',(-7.00001750459986,-24.4995582908587,
-8.95763010679384));
#54274=CARTESIAN_POINT('Ctrl Pts',(-7.00001874206956,-24.6244637358377,
-9.11545880287537));
#54275=CARTESIAN_POINT('Ctrl Pts',(-7.00001328594145,-24.7435693586713,
-9.27450916479436));
#54276=CARTESIAN_POINT('Ctrl Pts',(-7.00001262322841,-24.7580361834604,
-9.29382776339437));
#54277=CARTESIAN_POINT('Ctrl Pts',(-7.00001186253236,-24.7724174727017,
-9.31316444096061));
#54278=CARTESIAN_POINT('Ctrl Pts',(-7.00001099698694,-24.786713413932,-9.33251829944506));
#54279=CARTESIAN_POINT('',(-6.271594443024,-25.5608538793679,-8.76071211955051));
#54280=CARTESIAN_POINT('Origin',(-5.99998362344702,-24.7867137519324,-9.33252812839853));
#54281=CARTESIAN_POINT('Ctrl Pts',(-6.26386060036066,-15.8144217559011,
-3.90573753028149));
#54282=CARTESIAN_POINT('Ctrl Pts',(-6.26455152101633,-16.0555043624403,
-3.90327937002865));
#54283=CARTESIAN_POINT('Ctrl Pts',(-6.26520985795224,-16.2942797838742,
-3.90810432648021));
#54284=CARTESIAN_POINT('Ctrl Pts',(-6.26583561154063,-16.5303211757527,
-3.9197834877742));
#54285=CARTESIAN_POINT('Ctrl Pts',(-6.26647066563248,-16.769870823628,-3.93163623509615));
#54286=CARTESIAN_POINT('Ctrl Pts',(-6.26707216061391,-17.006604611909,-3.95054842272576));
#54287=CARTESIAN_POINT('Ctrl Pts',(-6.26764009687402,-17.2401298953749,
-3.97608001918924));
#54288=CARTESIAN_POINT('Ctrl Pts',(-6.26812468476161,-17.4393838112797,
-3.99786468635311));
#54289=CARTESIAN_POINT('Ctrl Pts',(-6.26858484108239,-17.6363028076252,
-4.02446858056822));
#54290=CARTESIAN_POINT('Ctrl Pts',(-6.26902056607808,-17.8306725457858,
-4.05562321047439));
#54291=CARTESIAN_POINT('Ctrl Pts',(-6.26953467319349,-18.0600072555133,
-4.0923822145962));
#54292=CARTESIAN_POINT('Ctrl Pts',(-6.27001476853342,-18.2857921847647,
-4.13547499922886));
#54293=CARTESIAN_POINT('Ctrl Pts',(-6.27046085249489,-18.5077369937188,
-4.18435768233148));
#54294=CARTESIAN_POINT('Ctrl Pts',(-6.2706208341698,-18.5873343461017,-4.20188876211064));
#54295=CARTESIAN_POINT('Ctrl Pts',(-6.27077644131375,-18.666438221103,-4.22016475889813));
#54296=CARTESIAN_POINT('Ctrl Pts',(-6.27092767394504,-18.7450366707039,
-4.2391613241562));
#54297=CARTESIAN_POINT('Ctrl Pts',(-6.27136815415621,-18.9739625406082,
-4.29449072631342));
#54298=CARTESIAN_POINT('Ctrl Pts',(-6.2717715237205,-19.1985969459198,-4.35593088266701));
#54299=CARTESIAN_POINT('Ctrl Pts',(-6.2721377826379,-19.4186799866693,-4.42289859637978));
#54300=CARTESIAN_POINT('Ctrl Pts',(-6.27250404155531,-19.6387630274189,
-4.48986631009256));
#54301=CARTESIAN_POINT('Ctrl Pts',(-6.27283318982583,-19.8542949102162,
-4.56236164112509));
#54302=CARTESIAN_POINT('Ctrl Pts',(-6.27312522744947,-20.0650658262731,
-4.63982808853314));
#54303=CARTESIAN_POINT('Ctrl Pts',(-6.27334042054069,-20.2203761058236,
-4.69691061124459));
#54304=CARTESIAN_POINT('Ctrl Pts',(-6.27353526296335,-20.3728239547611,
-4.75658573046659));
#54305=CARTESIAN_POINT('Ctrl Pts',(-6.27370997638795,-20.5226551266523,
-4.81874475214896));
#54306=CARTESIAN_POINT('Ctrl Pts',(-6.27388468981255,-20.6724862985435,
-4.88090377383133));
#54307=CARTESIAN_POINT('Ctrl Pts',(-6.27403927423909,-20.8197011255933,
-4.9455469677457));
#54308=CARTESIAN_POINT('Ctrl Pts',(-6.2741739513381,-20.9645377629538,-5.01262254869206));
#54309=CARTESIAN_POINT('Ctrl Pts',(-6.27427013657007,-21.0679788503139,
-5.06052735478846));
#54310=CARTESIAN_POINT('Ctrl Pts',(-6.27435616768303,-21.1702067690755,
-5.10967398530267));
#54311=CARTESIAN_POINT('Ctrl Pts',(-6.27443212542871,-21.2713096271537,
-5.1600492269349));
#54312=CARTESIAN_POINT('Ctrl Pts',(-6.27457884449751,-21.466598692925,-5.25735343834247));
#54313=CARTESIAN_POINT('Ctrl Pts',(-6.27469165431798,-21.6616526261861,
-5.36122068036853));
#54314=CARTESIAN_POINT('Ctrl Pts',(-6.27477055489012,-21.8559696046935,
-5.47186403281939));
#54315=CARTESIAN_POINT('Ctrl Pts',(-6.27484862803197,-22.0482487810896,
-5.58134706845722));
#54316=CARTESIAN_POINT('Ctrl Pts',(-6.2748934994088,-22.2398064589334,-5.69746491395644));
#54317=CARTESIAN_POINT('Ctrl Pts',(-6.27490516902061,-22.430109432408,-5.82040617935769));
#54318=CARTESIAN_POINT('Ctrl Pts',(-6.27491664504186,-22.6172554148452,
-5.94130793656888));
#54319=CARTESIAN_POINT('Ctrl Pts',(-6.27489601174817,-22.8031880010741,
-6.06880865090116));
#54320=CARTESIAN_POINT('Ctrl Pts',(-6.27484326913954,-22.9873536900837,
-6.20306945318438));
#54321=CARTESIAN_POINT('Ctrl Pts',(-6.27479056659583,-23.1713794811427,
-6.33722826681168));
#54322=CARTESIAN_POINT('Ctrl Pts',(-6.2747058035011,-23.353641205317,-6.4781370005255));
#54323=CARTESIAN_POINT('Ctrl Pts',(-6.27458897985536,-23.5335384516302,
-6.62593686197285));
#54324=CARTESIAN_POINT('Ctrl Pts',(-6.27454781366932,-23.5969304427347,
-6.67801841238085));
#54325=CARTESIAN_POINT('Ctrl Pts',(-6.2745026665428,-23.6600283853014,-6.73095545421918));
#54326=CARTESIAN_POINT('Ctrl Pts',(-6.27445353846372,-23.7228045291254,
-6.78475355165375));
#54327=CARTESIAN_POINT('Ctrl Pts',(-6.27431624089265,-23.8982441601719,
-6.93510235917805));
#54328=CARTESIAN_POINT('Ctrl Pts',(-6.27414785100046,-24.0711731898611,
-7.09217873860768));
#54329=CARTESIAN_POINT('Ctrl Pts',(-6.273948368523,-24.241035364564,-7.25599605961389));
#54330=CARTESIAN_POINT('Ctrl Pts',(-6.2737507271022,-24.4093298532675,-7.4183014835715));
#54331=CARTESIAN_POINT('Ctrl Pts',(-6.27352256436492,-24.5746138826622,
-7.58722407975246));
#54332=CARTESIAN_POINT('Ctrl Pts',(-6.27326388005427,-24.736307790633,-7.76274419335866));
#54333=CARTESIAN_POINT('Ctrl Pts',(-6.27300884371265,-24.8957214893191,
-7.93578912037485));
#54334=CARTESIAN_POINT('Ctrl Pts',(-6.27272414055906,-25.0516456202578,
-8.11524684955891));
#54335=CARTESIAN_POINT('Ctrl Pts',(-6.27240977034733,-25.2034865494107,
-8.3010657208509));
#54336=CARTESIAN_POINT('Ctrl Pts',(-6.27215746715882,-25.3253490832686,
-8.45019783312509));
#54337=CARTESIAN_POINT('Ctrl Pts',(-6.2718860550044,-25.4445808669205,-8.60342664882594));
#54338=CARTESIAN_POINT('Ctrl Pts',(-6.27159553375681,-25.5608567073965,
-8.76070944735595));
#54339=CARTESIAN_POINT('Origin',(-5.999994993365,-24.786719601394,-9.33250915082771));
#54340=CARTESIAN_POINT('',(-5.98852246669785,-25.7188096068216,-9.69456809148799));
#54341=CARTESIAN_POINT('Origin',(-5.999994993365,-24.786719601394,-9.33250915082771));
#54342=CARTESIAN_POINT('Origin',(-6.,-24.7867243682986,-9.33251101023518));
#54343=CARTESIAN_POINT('Ctrl Pts',(-5.98841833130012,-25.7189877482677,
-9.69410640815296));
#54344=CARTESIAN_POINT('Ctrl Pts',(-5.98810627248473,-25.6713270177476,
-9.81679904172914));
#54345=CARTESIAN_POINT('Ctrl Pts',(-5.98726405054396,-25.5029619479273,
-10.2439466060386));
#54346=CARTESIAN_POINT('Ctrl Pts',(-5.98726405054303,-25.276881441752,-10.7897532301295));
#54347=CARTESIAN_POINT('Ctrl Pts',(-5.98810627250475,-25.0938945838116,
-11.2108442545143));
#54348=CARTESIAN_POINT('Ctrl Pts',(-5.988418331338,-25.0408390143962,-11.3313022777533));
#54349=CARTESIAN_POINT('Ctrl Pts',(-6.5801963721225,-25.7253769306717,-9.69658812258632));
#54350=CARTESIAN_POINT('Ctrl Pts',(-6.57988216475446,-25.6778801589542,
-9.81936871691908));
#54351=CARTESIAN_POINT('Ctrl Pts',(-6.57903377348696,-25.5099484810557,
-10.2467760959601));
#54352=CARTESIAN_POINT('Ctrl Pts',(-6.57903377348612,-25.283822418215,-10.7926927035727));
#54353=CARTESIAN_POINT('Ctrl Pts',(-6.57988216477348,-25.1003453891382,
-11.2136609903448));
#54354=CARTESIAN_POINT('Ctrl Pts',(-6.58019637215976,-25.0471116856881,
-11.3340652748482));
#54355=CARTESIAN_POINT('Ctrl Pts',(-7.00079676976986,-25.3372908820653,
-9.54584601778628));
#54356=CARTESIAN_POINT('Ctrl Pts',(-7.00061248512561,-25.2904141391689,
-9.66739289158177));
#54357=CARTESIAN_POINT('Ctrl Pts',(-7.00011448465087,-25.1245686184425,
-10.0904742413177));
#54358=CARTESIAN_POINT('Ctrl Pts',(-7.00011448465083,-24.900795602742,-10.6307100906301));
#54359=CARTESIAN_POINT('Ctrl Pts',(-7.00061248513681,-24.7189024024401,
-11.0471442768304));
#54360=CARTESIAN_POINT('Ctrl Pts',(-7.00079676979122,-24.6661026445716,
-11.1662377625412));
#54361=CARTESIAN_POINT('Ctrl Pts',(-6.99999917319453,-24.7856430606156,
-9.33157252365516));
#54362=CARTESIAN_POINT('Ctrl Pts',(-6.99999957777276,-24.7394735072572,
-9.45129807097163));
#54363=CARTESIAN_POINT('Ctrl Pts',(-7.00000004362276,-24.5761256640229,
-9.8680415723771));
#54364=CARTESIAN_POINT('Ctrl Pts',(-7.00000004362357,-24.355704222059,-10.4001860069027));
#54365=CARTESIAN_POINT('Ctrl Pts',(-6.999999577773,-24.1765264326202,-10.810372532843));
#54366=CARTESIAN_POINT('Ctrl Pts',(-6.99999917319377,-24.1245144885734,
-10.9276780876708));
#54367=CARTESIAN_POINT('Origin',(-5.98852353414726,11.4730434399881,4.75229019692621));
#54368=CARTESIAN_POINT('Origin',(-7.0002100696521,11.4504616060432,4.74293652827744));
#54369=CARTESIAN_POINT('Ctrl Pts',(-6.05508738338166,-25.8431978089075,
-9.37216207432707));
#54370=CARTESIAN_POINT('Ctrl Pts',(-4.03672492225411,-26.0304387093361,
-8.81555276746131));
#54371=CARTESIAN_POINT('Ctrl Pts',(7.59697247682684E-7,-26.2482635689839,
-8.27058109728118));
#54372=CARTESIAN_POINT('Ctrl Pts',(4.03672644164874,-26.0304386273479,-8.81555297258393));
#54373=CARTESIAN_POINT('Ctrl Pts',(6.05508966247359,-25.8431975974789,-9.37216270283815));
#54374=CARTESIAN_POINT('Ctrl Pts',(-6.05508738338166,-25.5527881519605,
-10.1400064040411));
#54375=CARTESIAN_POINT('Ctrl Pts',(-4.03672492225411,-25.6069167071504,
-9.95059902476454));
#54376=CARTESIAN_POINT('Ctrl Pts',(7.59697247682684E-7,-25.7964943223401,
-9.81341146699688));
#54377=CARTESIAN_POINT('Ctrl Pts',(4.03672644164874,-25.6069166358008,-9.95059907640347));
#54378=CARTESIAN_POINT('Ctrl Pts',(6.05508966247359,-25.5527880908442,-10.1400066179177));
#54379=CARTESIAN_POINT('Ctrl Pts',(-6.05508738338166,-25.2383576100257,
-10.8990909622833));
#54380=CARTESIAN_POINT('Ctrl Pts',(-4.03672492225411,-25.1425761077887,
-11.0715861668952));
#54381=CARTESIAN_POINT('Ctrl Pts',(7.59697247682684E-7,-25.1794674505639,
-11.3029246861743));
#54382=CARTESIAN_POINT('Ctrl Pts',(4.03672644164874,-25.1425760939039,-11.0715860798213));
#54383=CARTESIAN_POINT('Ctrl Pts',(6.05508966247359,-25.2383577181847,-10.8990907675073));
#54384=CARTESIAN_POINT('Ctrl Pts',(-6.05508738338166,-24.900747869581,-11.6473837381431));
#54385=CARTESIAN_POINT('Ctrl Pts',(-4.03672492225411,-24.6394316467689,
-12.1736501920162));
#54386=CARTESIAN_POINT('Ctrl Pts',(7.59697247682684E-7,-24.4078877465999,
-12.7132770985331));
#54387=CARTESIAN_POINT('Ctrl Pts',(4.03672644164874,-24.6394317339223,-12.1736499889053));
#54388=CARTESIAN_POINT('Ctrl Pts',(6.05508966247359,-24.9007481646544,-11.647383143894));
#54389=CARTESIAN_POINT('Ctrl Pts',(-5.98852262888631,-25.7188097476013,
-9.69456765092976));
#54390=CARTESIAN_POINT('Ctrl Pts',(-5.9390643825995,-25.724559801551,-9.67819736170012));
#54391=CARTESIAN_POINT('Ctrl Pts',(-5.88263516414606,-25.7310811669272,
-9.65968542650558));
#54392=CARTESIAN_POINT('Ctrl Pts',(-5.8191641443799,-25.7383219151964,-9.63921749653948));
#54393=CARTESIAN_POINT('Ctrl Pts',(-5.75804505445195,-25.7452943562608,
-9.61950800933027));
#54394=CARTESIAN_POINT('Ctrl Pts',(-5.69039610157012,-25.7529339130711,
-9.59798498846537));
#54395=CARTESIAN_POINT('Ctrl Pts',(-5.61614355003017,-25.761179079695,-9.57485600815482));
#54396=CARTESIAN_POINT('Ctrl Pts',(-5.54046210244506,-25.7695829140783,
-9.55128193999465));
#54397=CARTESIAN_POINT('Ctrl Pts',(-5.45792023964537,-25.7786161404993,
-9.52603926689531));
#54398=CARTESIAN_POINT('Ctrl Pts',(-5.36843221659716,-25.7881950956482,
-9.49939300492048));
#54399=CARTESIAN_POINT('Ctrl Pts',(-5.32368820507305,-25.7929845732227,
-9.48606987393307));
#54400=CARTESIAN_POINT('Ctrl Pts',(-5.27720755484741,-25.79791017272,-9.47239656836499));
#54401=CARTESIAN_POINT('Ctrl Pts',(-5.22897913301206,-25.8029594239223,
-9.4584106464505));
#54402=CARTESIAN_POINT('Ctrl Pts',(-5.20486492209439,-25.8054840495234,
-9.45141768549325));
#54403=CARTESIAN_POINT('Ctrl Pts',(-5.18031376829501,-25.8080395842763,
-9.44434656901355));
#54404=CARTESIAN_POINT('Ctrl Pts',(-5.15532426463177,-25.8106243048844,
-9.43720234551523));
#54405=CARTESIAN_POINT('Ctrl Pts',(-5.13033476096853,-25.8132090254925,
-9.4300581220169));
#54406=CARTESIAN_POINT('Ctrl Pts',(-5.10370559224123,-25.8159456101558,
-9.42250242119417));
#54407=CARTESIAN_POINT('Ctrl Pts',(-5.07903930494025,-25.818464270517,-9.41555542182804));
#54408=CARTESIAN_POINT('Ctrl Pts',(-5.06413128986708,-25.8199865193325,
-9.41135673679693));
#54409=CARTESIAN_POINT('Ctrl Pts',(-5.04933271582664,-25.8214915258363,
-9.40720810707613));
#54410=CARTESIAN_POINT('Ctrl Pts',(-5.0346439037231,-25.8229794943833,-9.40310875488214));
#54411=CARTESIAN_POINT('Ctrl Pts',(-4.91716822316177,-25.8348797158908,
-9.37032365385047));
#54412=CARTESIAN_POINT('Ctrl Pts',(-4.80671568615821,-25.8456906475692,
-9.34068705338644));
#54413=CARTESIAN_POINT('Ctrl Pts',(-4.70342528861786,-25.8555215872748,
-9.31382718463705));
#54414=CARTESIAN_POINT('Ctrl Pts',(-4.60047417080891,-25.865320235125,-9.28705554295689));
#54415=CARTESIAN_POINT('Ctrl Pts',(-4.50463790934284,-25.8741455223677,
-9.26304224523494));
#54416=CARTESIAN_POINT('Ctrl Pts',(-4.41602611056628,-25.8820979118167,
-9.24146192010301));
#54417=CARTESIAN_POINT('Ctrl Pts',(-4.38394681488766,-25.8849768405374,
-9.23364939806524));
#54418=CARTESIAN_POINT('Ctrl Pts',(-4.35281410508567,-25.8877412796611,
-9.22615615817267));
#54419=CARTESIAN_POINT('Ctrl Pts',(-4.3226323863034,-25.8903956683114,-9.21896821569922));
#54420=CARTESIAN_POINT('Ctrl Pts',(-4.28802313193754,-25.8934394449979,
-9.21072583125368));
#54421=CARTESIAN_POINT('Ctrl Pts',(-4.25466435763063,-25.8963385236158,
-9.20288485679624));
#54422=CARTESIAN_POINT('Ctrl Pts',(-4.22256207443942,-25.8990992696321,
-9.1954255081038));
#54423=CARTESIAN_POINT('Ctrl Pts',(-4.20651093284382,-25.9004796426402,
-9.19169583375758));
#54424=CARTESIAN_POINT('Ctrl Pts',(-4.19077391402756,-25.901825434645,-9.18806156664566));
#54425=CARTESIAN_POINT('Ctrl Pts',(-4.17535169773152,-25.9031373973644,
-9.18452039028601));
#54426=CARTESIAN_POINT('Ctrl Pts',(-4.1676405895835,-25.9037933787241,-9.18274980210618));
#54427=CARTESIAN_POINT('Ctrl Pts',(-4.16000818206553,-25.9044409028845,
-9.18100248665958));
#54428=CARTESIAN_POINT('Ctrl Pts',(-4.15245455838758,-25.9050800628873,
-9.17927815906634));
#54429=CARTESIAN_POINT('Ctrl Pts',(-4.14867774654861,-25.9053996428886,
-9.17841599526972));
#54430=CARTESIAN_POINT('Ctrl Pts',(-4.14492063066965,-25.9057171318577,
-9.17755957843908));
#54431=CARTESIAN_POINT('Ctrl Pts',(-4.14118322091831,-25.9060325412745,
-9.17670887350226));
#54432=CARTESIAN_POINT('Ctrl Pts',(-4.13931451604264,-25.9061902459829,
-9.17628352103385));
#54433=CARTESIAN_POINT('Ctrl Pts',(-4.13745073769887,-25.9063474308037,
-9.17585959653905));
#54434=CARTESIAN_POINT('Ctrl Pts',(-4.13559188714296,-25.9065040971616,
-9.17543709566931));
#54435=CARTESIAN_POINT('Ctrl Pts',(-4.13373303658705,-25.9066607635196,
-9.17501459479957));
#54436=CARTESIAN_POINT('Ctrl Pts',(-4.13363444556609,-25.9066691641448,
-9.17499191745734));
#54437=CARTESIAN_POINT('Ctrl Pts',(-4.1300301200903,-25.9069725422699,-9.17417385959775));
#54438=CARTESIAN_POINT('Ctrl Pts',(-4.08661760549322,-25.9106265983135,
-9.16432071259167));
#54439=CARTESIAN_POINT('Ctrl Pts',(-4.04433457952546,-25.9141332066327,
-9.15487888299753));
#54440=CARTESIAN_POINT('Ctrl Pts',(-4.00318800195899,-25.9174995886589,
-9.14582562332909));
#54441=CARTESIAN_POINT('Ctrl Pts',(-3.90004608897409,-25.9259380810574,
-9.12313186418366));
#54442=CARTESIAN_POINT('Ctrl Pts',(-3.80404668550376,-25.9334963251751,
-9.10287652665312));
#54443=CARTESIAN_POINT('Ctrl Pts',(-3.71528285380719,-25.9402828195675,
-9.08473148518902));
#54444=CARTESIAN_POINT('Ctrl Pts',(-3.627035643983,-25.9470298153109,-9.06669205121298));
#54445=CARTESIAN_POINT('Ctrl Pts',(-3.54593976008338,-25.9530141365386,
-9.05073831598289));
#54446=CARTESIAN_POINT('Ctrl Pts',(-3.47206598411144,-25.9583296823689,
-9.03659310550064));
#54447=CARTESIAN_POINT('Ctrl Pts',(-3.41362152278194,-25.9625350205777,
-9.02540227091624));
#54448=CARTESIAN_POINT('Ctrl Pts',(-3.35969695816188,-25.9663215400282,
-9.0153442568734));
#54449=CARTESIAN_POINT('Ctrl Pts',(-3.31031961185454,-25.9697293685188,
-9.00630267440747));
#54450=CARTESIAN_POINT('Ctrl Pts',(-3.27705079779092,-25.9720254500398,
-9.00021075678946));
#54451=CARTESIAN_POINT('Ctrl Pts',(-3.24584610897252,-25.9741495022497,
-8.994580642952));
#54452=CARTESIAN_POINT('Ctrl Pts',(-3.21671236822705,-25.9761122277145,
-8.98938162097428));
#54453=CARTESIAN_POINT('Ctrl Pts',(-3.20214549785432,-25.9770935904469,
-8.98678210998543));
#54454=CARTESIAN_POINT('Ctrl Pts',(-3.1880963645055,-25.9780346232269,-8.98429037258426));
#54455=CARTESIAN_POINT('Ctrl Pts',(-3.17456569417812,-25.9789365146577,
-8.98190301543562));
#54456=CARTESIAN_POINT('Ctrl Pts',(-3.16780035901443,-25.9793874603731,
-8.9807093368613));
#54457=CARTESIAN_POINT('Ctrl Pts',(-3.16116463960638,-25.9798286208403,
-8.97954175338216));
#54458=CARTESIAN_POINT('Ctrl Pts',(-3.15465862374933,-25.9802601405916,
-8.97839985366472));
#54459=CARTESIAN_POINT('Ctrl Pts',(-3.1514056158208,-25.9804759004673,-8.97782890380599));
#54460=CARTESIAN_POINT('Ctrl Pts',(-3.14818503378004,-25.9806892501687,
-8.97726437488937));
#54461=CARTESIAN_POINT('Ctrl Pts',(-3.14499688817315,-25.980900207222,-8.97670621709465));
#54462=CARTESIAN_POINT('Ctrl Pts',(-3.14180874256627,-25.9811111642753,
-8.97614805929993));
#54463=CARTESIAN_POINT('Ctrl Pts',(-3.13695795646078,-25.9814316329932,
-8.97530023435297));
#54464=CARTESIAN_POINT('Ctrl Pts',(-3.13552977107617,-25.9815259178094,
-8.97505080774237));
#54465=CARTESIAN_POINT('Ctrl Pts',(-3.11970257976371,-25.9825707848406,
-8.97228665490416));
#54466=CARTESIAN_POINT('Ctrl Pts',(-3.09679456800648,-25.9840828600508,
-8.96828669945725));
#54467=CARTESIAN_POINT('Ctrl Pts',(-3.06678982289584,-25.9860344425227,
-8.96312842074186));
#54468=CARTESIAN_POINT('Ctrl Pts',(-3.03690025826695,-25.9879785333725,
-8.95798994332873));
#54469=CARTESIAN_POINT('Ctrl Pts',(-2.99996826007926,-25.9903587923726,
-8.95170200207538));
#54470=CARTESIAN_POINT('Ctrl Pts',(-2.95596929739872,-25.9931304079546,
-8.94438903715539));
#54471=CARTESIAN_POINT('Ctrl Pts',(-2.9382186804789,-25.9942485680986,-8.94143874853641));
#54472=CARTESIAN_POINT('Ctrl Pts',(-2.91931776614415,-25.9954302236241,
-8.93832217564728));
#54473=CARTESIAN_POINT('Ctrl Pts',(-2.8992645887638,-25.9966716041366,-8.93504972133033));
#54474=CARTESIAN_POINT('Ctrl Pts',(-2.8497154996617,-25.9997389122471,-8.92696386403911));
#54475=CARTESIAN_POINT('Ctrl Pts',(-2.79313189633374,-26.0031721325053,
-8.91792294670148));
#54476=CARTESIAN_POINT('Ctrl Pts',(-2.72948003412134,-26.006901810286,-8.9081174418846));
#54477=CARTESIAN_POINT('Ctrl Pts',(-2.66624669988098,-26.0106069644404,
-8.89837641087733));
#54478=CARTESIAN_POINT('Ctrl Pts',(-2.5960375787483,-26.0146047328404,-8.88788080115353));
#54479=CARTESIAN_POINT('Ctrl Pts',(-2.51881565324327,-26.0188086392253,
-8.87686505424636));
#54480=CARTESIAN_POINT('Ctrl Pts',(-2.46592221941314,-26.0216881199264,
-8.8693197790371));
#54481=CARTESIAN_POINT('Ctrl Pts',(-2.40973856258863,-26.0246639339917,
-8.86153146052812));
#54482=CARTESIAN_POINT('Ctrl Pts',(-2.35025240331417,-26.0277030808939,
-8.8535885713598));
#54483=CARTESIAN_POINT('Ctrl Pts',(-2.31847580468596,-26.029326546797,-8.84934560116087));
#54484=CARTESIAN_POINT('Ctrl Pts',(-2.2857568244182,-26.0309680115456,-8.84505870662713));
#54485=CARTESIAN_POINT('Ctrl Pts',(-2.2520936107303,-26.0326219258945,-8.84074265221651));
#54486=CARTESIAN_POINT('Ctrl Pts',(-2.23526200388636,-26.033448883069,-8.8385846250112));
#54487=CARTESIAN_POINT('Ctrl Pts',(-2.21819433868372,-26.0342789518604,
-8.83641930756526));
#54488=CARTESIAN_POINT('Ctrl Pts',(-2.20089038788782,-26.0351113981157,
-8.83424864635563));
#54489=CARTESIAN_POINT('Ctrl Pts',(-2.19223841248987,-26.0355276212433,
-8.83316331575081));
#54490=CARTESIAN_POINT('Ctrl Pts',(-2.18352736569337,-26.0359444386846,
-8.83207664918696));
#54491=CARTESIAN_POINT('Ctrl Pts',(-2.17475721935004,-26.0363617573365,
-8.83098889277727));
#54492=CARTESIAN_POINT('Ctrl Pts',(-2.16817960959255,-26.0366747463254,
-8.83017307547));
#54493=CARTESIAN_POINT('Ctrl Pts',(-2.16156875633996,-26.0369880172407,
-8.82935664512291));
#54494=CARTESIAN_POINT('Ctrl Pts',(-2.15492464778689,-26.0373015303008,
-8.8285397067524));
#54495=CARTESIAN_POINT('Ctrl Pts',(-2.15270994493586,-26.0374060346541,
-8.82826739396223));
#54496=CARTESIAN_POINT('Ctrl Pts',(-2.14918581021123,-26.0375720050318,
-8.82783494548843));
#54497=CARTESIAN_POINT('Ctrl Pts',(-2.14826945370358,-26.037615122561,-8.82772260303836));
#54498=CARTESIAN_POINT('Ctrl Pts',(-2.01266622350348,-26.0439956918975,
-8.81109806990979));
#54499=CARTESIAN_POINT('Ctrl Pts',(-1.87302045106776,-26.0499592140147,
-8.79562775335127));
#54500=CARTESIAN_POINT('Ctrl Pts',(-1.72934561672299,-26.0553981437514,
-8.78158323778946));
#54501=CARTESIAN_POINT('Ctrl Pts',(-1.55031236599416,-26.0621755955974,
-8.76408236307183));
#54502=CARTESIAN_POINT('Ctrl Pts',(-1.36502204175769,-26.0681392785514,
-8.74879507273714));
#54503=CARTESIAN_POINT('Ctrl Pts',(-1.17351855624395,-26.0730598440868,
-8.73625149146255));
#54504=CARTESIAN_POINT('Ctrl Pts',(-0.994986214400786,-26.0776471239783,
-8.72455752707311));
#54505=CARTESIAN_POINT('Ctrl Pts',(-0.811053940501206,-26.0813276621787,
-8.71524850658676));
#54506=CARTESIAN_POINT('Ctrl Pts',(-0.621782179047148,-26.0838950606796,
-8.70877900139082));
#54507=CARTESIAN_POINT('Ctrl Pts',(-0.437432969141425,-26.0863956866659,
-8.70247775411448));
#54508=CARTESIAN_POINT('Ctrl Pts',(-0.24801674368234,-26.0878397285108,
-8.69887053619326));
#54509=CARTESIAN_POINT('Ctrl Pts',(-0.0536790750609311,-26.0880417664438,
-8.69839184997735));
#54510=CARTESIAN_POINT('Ctrl Pts',(0.0580605512452798,-26.0881579335424,
-8.69811661656912));
#54511=CARTESIAN_POINT('Ctrl Pts',(0.171426389472391,-26.0878632658087,
-8.69887602550745));
#54512=CARTESIAN_POINT('Ctrl Pts',(0.286383677659182,-26.0871206111961,
-8.700755502493));
#54513=CARTESIAN_POINT('Ctrl Pts',(0.308582461111033,-26.0869772011593,
-8.70111843818209));
#54514=CARTESIAN_POINT('Ctrl Pts',(0.330840572337808,-26.0868170817409,
-8.70152314662147));
#54515=CARTESIAN_POINT('Ctrl Pts',(0.353157737064551,-26.0866399792483,
-8.70197025192061));
#54516=CARTESIAN_POINT('Ctrl Pts',(0.484497400390817,-26.0855977060906,
-8.70460152969178));
#54517=CARTESIAN_POINT('Ctrl Pts',(0.617882879397884,-26.0839671724966,
-8.70870081522193));
#54518=CARTESIAN_POINT('Ctrl Pts',(0.753271868137669,-26.0817077353392,
-8.71440618982747));
#54519=CARTESIAN_POINT('Ctrl Pts',(0.832468974465638,-26.0803860555892,
-8.71774360421753));
#54520=CARTESIAN_POINT('Ctrl Pts',(0.912351579049761,-26.0788492375685,
-8.72163053479288));
#54521=CARTESIAN_POINT('Ctrl Pts',(0.992910103713763,-26.0770891929669,
-8.7260955784618));
#54522=CARTESIAN_POINT('Ctrl Pts',(1.03318936604576,-26.0762091706661,-8.72832810029627));
#54523=CARTESIAN_POINT('Ctrl Pts',(1.0736376083974,-26.0752733456166,-8.73070515169355));
#54524=CARTESIAN_POINT('Ctrl Pts',(1.11425355911735,-26.0742807242355,-8.73323033517445));
#54525=CARTESIAN_POINT('Ctrl Pts',(1.13456153447733,-26.0737844135449,-8.7344929269149));
#54526=CARTESIAN_POINT('Ctrl Pts',(1.15491143693055,-26.0732739040251,-8.73579255176232));
#54527=CARTESIAN_POINT('Ctrl Pts',(1.17530310417698,-26.0727490719265,-8.73712966381612));
#54528=CARTESIAN_POINT('Ctrl Pts',(1.1854989378002,-26.0724866558773,-8.73779821984302));
#54529=CARTESIAN_POINT('Ctrl Pts',(1.19570521262178,-26.0722206591995,-8.73847614767697));
#54530=CARTESIAN_POINT('Ctrl Pts',(1.20592190804525,-26.0719510664548,-8.73916350431498));
#54531=CARTESIAN_POINT('Ctrl Pts',(1.20990015194453,-26.071846090663,-8.73943115175267));
#54532=CARTESIAN_POINT('Ctrl Pts',(1.21387997583525,-26.0717405696339,-8.73970022879072));
#54533=CARTESIAN_POINT('Ctrl Pts',(1.21786137849269,-26.0716345024541,-8.73997073880825));
#54534=CARTESIAN_POINT('Ctrl Pts',(1.2189923796168,-26.0716043718419,-8.74004758286554));
#54535=CARTESIAN_POINT('Ctrl Pts',(1.22012350814158,-26.0715741971573,-8.74012454255906));
#54536=CARTESIAN_POINT('Ctrl Pts',(1.22125476403901,-26.071543978378,-8.74020161795894));
#54537=CARTESIAN_POINT('Ctrl Pts',(1.2238115417489,-26.0714756802134,-8.74037581785909));
#54538=CARTESIAN_POINT('Ctrl Pts',(1.22636897009813,-26.0714071567992,-8.7405506088244));
#54539=CARTESIAN_POINT('Ctrl Pts',(1.22892704876324,-26.0713384078877,-8.74072599163071));
#54540=CARTESIAN_POINT('Ctrl Pts',(1.23148512742836,-26.0712696589762,-8.74090137443703));
#54541=CARTESIAN_POINT('Ctrl Pts',(1.23542074353098,-26.071163456459,-8.74117233826181));
#54542=CARTESIAN_POINT('Ctrl Pts',(1.23660323538091,-26.0711314843902,-8.74125391641842));
#54543=CARTESIAN_POINT('Ctrl Pts',(1.30395073383312,-26.0693105510324,-8.74590010892824));
#54544=CARTESIAN_POINT('Ctrl Pts',(1.37844760563595,-26.067146299812,-8.75143637844141));
#54545=CARTESIAN_POINT('Ctrl Pts',(1.46006216964867,-26.064542777595,-8.75811811399493));
#54546=CARTESIAN_POINT('Ctrl Pts',(1.54172917708157,-26.0619375824215,-8.76480414305991));
#54547=CARTESIAN_POINT('Ctrl Pts',(1.63052324890772,-26.0588924819595,-8.77263715624206));
#54548=CARTESIAN_POINT('Ctrl Pts',(1.72639942053101,-26.0552949733739,-8.7819207900803));
#54549=CARTESIAN_POINT('Ctrl Pts',(1.81110726429991,-26.0521165277804,-8.79012300123937));
#54550=CARTESIAN_POINT('Ctrl Pts',(1.90134329068553,-26.0485066029823,-8.79945826899446));
#54551=CARTESIAN_POINT('Ctrl Pts',(1.99706565552955,-26.0443777045615,-8.81016651175319));
#54552=CARTESIAN_POINT('Ctrl Pts',(2.10635221589194,-26.0396637267232,-8.82239215014537));
#54553=CARTESIAN_POINT('Ctrl Pts',(2.22279080382339,-26.0342733681395,-8.83640677412009));
#54554=CARTESIAN_POINT('Ctrl Pts',(2.34629930883073,-26.0280648257203,-8.85260839878758));
#54555=CARTESIAN_POINT('Ctrl Pts',(2.462528553975,-26.0222221981314,-8.86785514317251));
#54556=CARTESIAN_POINT('Ctrl Pts',(2.58501896755301,-26.0156547777424,-8.88503916917858));
#54557=CARTESIAN_POINT('Ctrl Pts',(2.71368124103882,-26.0082351007993,-8.90452762382412));
#54558=CARTESIAN_POINT('Ctrl Pts',(2.74250184117935,-26.0065730786963,-8.90889307566542));
#54559=CARTESIAN_POINT('Ctrl Pts',(2.77163203637594,-26.0048682608314,-8.913374290048));
#54560=CARTESIAN_POINT('Ctrl Pts',(2.80107067532219,-26.0031191765166,-8.91797557208791));
#54561=CARTESIAN_POINT('Ctrl Pts',(2.82649121064435,-26.0016088261337,-8.92194882142312));
#54562=CARTESIAN_POINT('Ctrl Pts',(2.85493636831501,-25.9998980382213,-8.92645224024806));
#54563=CARTESIAN_POINT('Ctrl Pts',(2.88361403628995,-25.9981472674012,-8.93106468954868));
#54564=CARTESIAN_POINT('Ctrl Pts',(2.89878519010301,-25.9972210688893,-8.93350478258051));
#54565=CARTESIAN_POINT('Ctrl Pts',(2.9140215577521,-25.9962839629684,-8.93597460837235));
#54566=CARTESIAN_POINT('Ctrl Pts',(2.92891080622877,-25.9953617172812,-8.93840622669497));
#54567=CARTESIAN_POINT('Ctrl Pts',(3.02425371736574,-25.9894561412721,-8.95397703068931));
#54568=CARTESIAN_POINT('Ctrl Pts',(3.11262114766818,-25.9837161646081,-8.96915081969007));
#54569=CARTESIAN_POINT('Ctrl Pts',(3.19406215928281,-25.9782486650069,-8.98363485151774));
#54570=CARTESIAN_POINT('Ctrl Pts',(3.25118405732209,-25.9744138163409,-8.99379380427207));
#54571=CARTESIAN_POINT('Ctrl Pts',(3.30489854065411,-25.9707125845228,-9.00361447197882));
#54572=CARTESIAN_POINT('Ctrl Pts',(3.35522197544709,-25.9671762224164,-9.01301002420905));
#54573=CARTESIAN_POINT('Ctrl Pts',(3.427773408449,-25.962077839536,-9.02655561744909));
#54574=CARTESIAN_POINT('Ctrl Pts',(3.49327684430623,-25.9573229291771,-9.03921551278359));
#54575=CARTESIAN_POINT('Ctrl Pts',(3.55177751951473,-25.9529893719757,-9.05077090283914));
#54576=CARTESIAN_POINT('Ctrl Pts',(3.61056551398029,-25.9486345310124,-9.06238304584795));
#54577=CARTESIAN_POINT('Ctrl Pts',(3.66228194477024,-25.9447051257599,-9.07287986166669));
#54578=CARTESIAN_POINT('Ctrl Pts',(3.70696567207482,-25.9412618732795,-9.08208825809521));
#54579=CARTESIAN_POINT('Ctrl Pts',(3.75187527224184,-25.9378012154182,-9.09134320227131));
#54580=CARTESIAN_POINT('Ctrl Pts',(3.78968101170105,-25.9348315888708,-9.09929670080249));
#54581=CARTESIAN_POINT('Ctrl Pts',(3.82041316876645,-25.9323970499494,-9.10582170121249));
#54582=CARTESIAN_POINT('Ctrl Pts',(3.8268804092965,-25.9318847283199,-9.10719481495197));
#54583=CARTESIAN_POINT('Ctrl Pts',(3.83303436389836,-25.9313960424363,-9.10850483834948));
#54584=CARTESIAN_POINT('Ctrl Pts',(3.83887525621521,-25.9309313071267,-9.10975085836551));
#54585=CARTESIAN_POINT('Ctrl Pts',(3.8511418551453,-25.9299553052862,-9.11236765507504));
#54586=CARTESIAN_POINT('Ctrl Pts',(3.86202771366167,-25.9290849785934,-9.11470204665891));
#54587=CARTESIAN_POINT('Ctrl Pts',(3.87153458996032,-25.9283227689994,-9.11674693379315));
#54588=CARTESIAN_POINT('Ctrl Pts',(3.87628802810965,-25.9279416642024,-9.11776937736027));
#54589=CARTESIAN_POINT('Ctrl Pts',(3.8806967207052,-25.9275875891028,-9.11871944496946));
#54590=CARTESIAN_POINT('Ctrl Pts',(3.88476083919448,-25.927260777662,-9.1195964528732));
#54591=CARTESIAN_POINT('Ctrl Pts',(3.88679289843912,-25.9270973719416,-9.12003495682507));
#54592=CARTESIAN_POINT('Ctrl Pts',(3.88873881415724,-25.9269407821652,-9.1204551958613));
#54593=CARTESIAN_POINT('Ctrl Pts',(3.89059860635588,-25.926791035726,-9.12085709015195));
#54594=CARTESIAN_POINT('Ctrl Pts',(3.8915285024552,-25.9267161625064,-9.12105803729728));
#54595=CARTESIAN_POINT('Ctrl Pts',(3.89243686767465,-25.926643000123,-9.12125439825693));
#54596=CARTESIAN_POINT('Ctrl Pts',(3.89332370434875,-25.9265715517621,-9.12144616374056));
#54597=CARTESIAN_POINT('Ctrl Pts',(3.89376712268579,-25.9265358275816,-9.12154204648237));
#54598=CARTESIAN_POINT('Ctrl Pts',(3.89420515887107,-25.9265005318859,-9.12163678041626));
#54599=CARTESIAN_POINT('Ctrl Pts',(3.89463512416906,-25.9264658820949,-9.12172978186106));
#54600=CARTESIAN_POINT('Ctrl Pts',(3.89506508946705,-25.9264312323039,-9.12182278330586));
#54601=CARTESIAN_POINT('Ctrl Pts',(3.89549238058995,-25.926396819668,-9.12191514342382));
#54602=CARTESIAN_POINT('Ctrl Pts',(3.89721720697796,-25.9262577386616,-9.12228846130778));
#54603=CARTESIAN_POINT('Ctrl Pts',(3.9060039205876,-25.9255492238917,-9.12419023957051));
#54604=CARTESIAN_POINT('Ctrl Pts',(3.91477185382022,-25.9248400577957,-9.12609425770661));
#54605=CARTESIAN_POINT('Ctrl Pts',(3.92352101537451,-25.9241302699203,-9.12800043834213));
#54606=CARTESIAN_POINT('Ctrl Pts',(4.08352595055138,-25.9111496474579,-9.16286072834021));
#54607=CARTESIAN_POINT('Ctrl Pts',(4.2372515957779,-25.8979630799124,-9.19844051498696));
#54608=CARTESIAN_POINT('Ctrl Pts',(4.38475854301892,-25.8847426375439,-9.23428876981734));
#54609=CARTESIAN_POINT('Ctrl Pts',(4.40472993871036,-25.8829526833031,-9.23914236956607));
#54610=CARTESIAN_POINT('Ctrl Pts',(4.42458735601385,-25.8811620725191,-9.2440009577067));
#54611=CARTESIAN_POINT('Ctrl Pts',(4.44433096147399,-25.879371199339,-9.24886347726735));
#54612=CARTESIAN_POINT('Ctrl Pts',(4.59308062293749,-25.8658786394415,-9.28549802914619));
#54613=CARTESIAN_POINT('Ctrl Pts',(4.73536929234841,-25.8523732550644,-9.32235201322874));
#54614=CARTESIAN_POINT('Ctrl Pts',(4.87127285544964,-25.8390137277172,-9.35900010657507));
#54615=CARTESIAN_POINT('Ctrl Pts',(4.89543477021471,-25.836638574677,-9.36551566869522));
#54616=CARTESIAN_POINT('Ctrl Pts',(4.9193948852595,-25.8342679688519,-9.37202483785233));
#54617=CARTESIAN_POINT('Ctrl Pts',(4.9431536540866,-25.8319027217208,-9.37852537158515));
#54618=CARTESIAN_POINT('Ctrl Pts',(5.07994861810915,-25.8182844278368,-9.41595324861781));
#54619=CARTESIAN_POINT('Ctrl Pts',(5.21006827342324,-25.8048459299023,-9.45309118221072));
#54620=CARTESIAN_POINT('Ctrl Pts',(5.33360072841922,-25.7917314277818,-9.489540727972));
#54621=CARTESIAN_POINT('Ctrl Pts',(5.36979447838387,-25.787889012356,-9.50022007329588));
#54622=CARTESIAN_POINT('Ctrl Pts',(5.40542280302128,-25.7840742393724,-9.51084062080672));
#54623=CARTESIAN_POINT('Ctrl Pts',(5.44048800084055,-25.7802903253814,-9.52139307544913));
#54624=CARTESIAN_POINT('Ctrl Pts',(5.56340174988859,-25.7670266028409,-9.55838250777583));
#54625=CARTESIAN_POINT('Ctrl Pts',(5.6793960161412,-25.7541441947357,-9.59453182277264));
#54626=CARTESIAN_POINT('Ctrl Pts',(5.78856808116882,-25.7417693278559,-9.62947415865375));
#54627=CARTESIAN_POINT('Ctrl Pts',(5.84238474412072,-25.735669103959,-9.64669907706479));
#54628=CARTESIAN_POINT('Ctrl Pts',(5.89454365554831,-25.7296917865968,-9.66363139276406));
#54629=CARTESIAN_POINT('Ctrl Pts',(5.94505661807474,-25.7238501735518,-9.68023115871441));
#54630=CARTESIAN_POINT('Ctrl Pts',(5.9596842864737,-25.722158544824,-9.68503815992117));
#54631=CARTESIAN_POINT('Ctrl Pts',(5.97417392860902,-25.720478286976,-9.68981729094707));
#54632=CARTESIAN_POINT('Ctrl Pts',(5.98852581858797,-25.7188097024617,-9.6945676349031));
#54633=CARTESIAN_POINT('Ctrl Pts',(-6.39567215644055,-25.5334667653534,
-8.78352118705417));
#54634=CARTESIAN_POINT('Ctrl Pts',(-6.35564925718895,-25.5378748085094,
-8.77012419398008));
#54635=CARTESIAN_POINT('Ctrl Pts',(-5.98525024729305,-25.578353672155,-8.64740198386364));
#54636=CARTESIAN_POINT('Ctrl Pts',(-5.25616848901603,-25.6522246220423,
-8.42856426610991));
#54637=CARTESIAN_POINT('Ctrl Pts',(-4.17576488242819,-25.743621550053,-8.16491332440422));
#54638=CARTESIAN_POINT('Ctrl Pts',(-3.01937236728622,-25.8195370899232,
-7.95089144637005));
#54639=CARTESIAN_POINT('Ctrl Pts',(-1.83578745054832,-25.8725333118012,
-7.80507997421356));
#54640=CARTESIAN_POINT('Ctrl Pts',(-0.697920992822499,-25.8989854873888,
-7.73463084102237));
#54641=CARTESIAN_POINT('Ctrl Pts',(0.331415178953193,-25.9017875496813,
-7.72744135310422));
#54642=CARTESIAN_POINT('Ctrl Pts',(1.24581749154929,-25.8874717448211,-7.76509324630723));
#54643=CARTESIAN_POINT('Ctrl Pts',(2.07031043576891,-25.8615908861053,-7.83520428425946));
#54644=CARTESIAN_POINT('Ctrl Pts',(2.81707948213384,-25.8276633033017,-7.9287568097775));
#54645=CARTESIAN_POINT('Ctrl Pts',(3.49019584722931,-25.7886676982261,-8.037881035032));
#54646=CARTESIAN_POINT('Ctrl Pts',(4.09498188336493,-25.7470110244898,-8.15592462114486));
#54647=CARTESIAN_POINT('Ctrl Pts',(4.65006137406161,-25.7034067880011,-8.28093045992463));
#54648=CARTESIAN_POINT('Ctrl Pts',(5.1805088354666,-25.6570334421092,-8.41545276582232));
#54649=CARTESIAN_POINT('Ctrl Pts',(5.70542717861576,-25.6067226998712,-8.56333529062248));
#54650=CARTESIAN_POINT('Ctrl Pts',(6.10978535963893,-25.5646819644592,-8.68891077621009));
#54651=CARTESIAN_POINT('Ctrl Pts',(6.34031713688981,-25.5395629979994,-8.76499255552385));
#54652=CARTESIAN_POINT('Ctrl Pts',(6.39541677264867,-25.5334956821542,-8.783436799282));
#54653=CARTESIAN_POINT('Ctrl Pts',(-6.33018760766523,-25.7767195002423,
-9.0673579311918));
#54654=CARTESIAN_POINT('Ctrl Pts',(-6.29063887077213,-25.7811601733469,
-9.05404229513906));
#54655=CARTESIAN_POINT('Ctrl Pts',(-5.9246008136023,-25.8219416068059,-8.9320552503747));
#54656=CARTESIAN_POINT('Ctrl Pts',(-5.20363827098165,-25.8964098971313,
-8.7143622180441));
#54657=CARTESIAN_POINT('Ctrl Pts',(-4.13466637401218,-25.9886138348841,
-8.45189574262935));
#54658=CARTESIAN_POINT('Ctrl Pts',(-2.99013371586683,-26.0652394577625,
-8.23872385364562));
#54659=CARTESIAN_POINT('Ctrl Pts',(-1.8183506761573,-26.1187440570414,-8.09343083226769));
#54660=CARTESIAN_POINT('Ctrl Pts',(-0.69152385866634,-26.1454448732183,
-8.02320443539093));
#54661=CARTESIAN_POINT('Ctrl Pts',(0.328416326756525,-26.1482718798261,
-8.01603491323138));
#54662=CARTESIAN_POINT('Ctrl Pts',(1.23411374808423,-26.1338238284116,-8.05357264195744));
#54663=CARTESIAN_POINT('Ctrl Pts',(2.05053453836073,-26.1076962181796,-8.12344815886598));
#54664=CARTESIAN_POINT('Ctrl Pts',(2.78984559872145,-26.073444587786,-8.21666390189123));
#54665=CARTESIAN_POINT('Ctrl Pts',(3.45612791104389,-26.0340809624483,-8.32536882872224));
#54666=CARTESIAN_POINT('Ctrl Pts',(4.05467909015723,-25.9920396096016,-8.44292969175125));
#54667=CARTESIAN_POINT('Ctrl Pts',(4.60394317824861,-25.9480439491093,-8.56739151877058));
#54668=CARTESIAN_POINT('Ctrl Pts',(5.12872579717185,-25.9012684884609,-8.70128826221729));
#54669=CARTESIAN_POINT('Ctrl Pts',(5.64789551119545,-25.8505397548962,-8.84842891857438));
#54670=CARTESIAN_POINT('Ctrl Pts',(6.04766431563905,-25.8081682551775,-8.97331340642041));
#54671=CARTESIAN_POINT('Ctrl Pts',(6.27548853167199,-25.7828608658207,-9.0489418703681));
#54672=CARTESIAN_POINT('Ctrl Pts',(6.32993492696099,-25.7767485946731,-9.06727395103012));
#54673=CARTESIAN_POINT('Ctrl Pts',(-6.21932807443185,-25.8366561953098,
-9.42526544364698));
#54674=CARTESIAN_POINT('Ctrl Pts',(-6.18048319064934,-25.8411258831892,
-9.41216291856682));
#54675=CARTESIAN_POINT('Ctrl Pts',(-5.82094596423115,-25.8821753788867,
-9.2921233703167));
#54676=CARTESIAN_POINT('Ctrl Pts',(-5.11256521731997,-25.9571564779671,
-9.07782999761601));
#54677=CARTESIAN_POINT('Ctrl Pts',(-4.06220012752473,-26.050033738679,-8.81943609738017));
#54678=CARTESIAN_POINT('Ctrl Pts',(-2.93773661016636,-26.1272380042585,
-8.60958393773643));
#54679=CARTESIAN_POINT('Ctrl Pts',(-1.78661031458413,-26.181144206621,-8.46656055933674));
#54680=CARTESIAN_POINT('Ctrl Pts',(-0.679624998528299,-26.2080305784431,
-8.39742173764442));
#54681=CARTESIAN_POINT('Ctrl Pts',(0.322797658933812,-26.2108747126336,
-8.39036078365421));
#54682=CARTESIAN_POINT('Ctrl Pts',(1.21266000783635,-26.1963305309027,-8.42732124814706));
#54683=CARTESIAN_POINT('Ctrl Pts',(2.01470259288328,-26.1700129285436,-8.49610835129674));
#54684=CARTESIAN_POINT('Ctrl Pts',(2.74098505369467,-26.1355047474246,-8.58786922908991));
#54685=CARTESIAN_POINT('Ctrl Pts',(3.39555710167175,-26.0958440060889,-8.69487932361028));
#54686=CARTESIAN_POINT('Ctrl Pts',(3.98362867447789,-26.0534876192753,-8.81061117452099));
#54687=CARTESIAN_POINT('Ctrl Pts',(4.52330902351571,-26.0091675072182,-8.93313965918623));
#54688=CARTESIAN_POINT('Ctrl Pts',(5.03895227535259,-25.9620546978064,-9.06495615570801));
#54689=CARTESIAN_POINT('Ctrl Pts',(5.54907007362038,-25.9109702775198,-9.20980289930939));
#54690=CARTESIAN_POINT('Ctrl Pts',(5.94182116576813,-25.8683117841367,-9.33272190788584));
#54691=CARTESIAN_POINT('Ctrl Pts',(6.16560261524064,-25.842837696862,-9.40714417382229));
#54692=CARTESIAN_POINT('Ctrl Pts',(6.21907959820766,-25.8366854345371,-9.42518270291576));
#54693=CARTESIAN_POINT('Ctrl Pts',(-6.09477939300047,-25.6963156654864,
-9.75500591347859));
#54694=CARTESIAN_POINT('Ctrl Pts',(-6.05666692574697,-25.7008024726199,
-9.74218730560947));
#54695=CARTESIAN_POINT('Ctrl Pts',(-5.70391276856241,-25.742009023419,-9.62475061279524));
#54696=CARTESIAN_POINT('Ctrl Pts',(-5.0089808343114,-25.8172720694164,-9.41513947846463));
#54697=CARTESIAN_POINT('Ctrl Pts',(-3.97907981782402,-25.9104968519052,
-9.16254124191398));
#54698=CARTESIAN_POINT('Ctrl Pts',(-2.87715857377971,-25.9879832334434,
-8.95752879977658));
#54699=CARTESIAN_POINT('Ctrl Pts',(-1.74963945844121,-26.0420697001683,
-8.81787687582311));
#54700=CARTESIAN_POINT('Ctrl Pts',(-0.665625857011165,-26.0690256208802,
-8.75037927471988));
#54701=CARTESIAN_POINT('Ctrl Pts',(0.316165362970241,-26.0718741826498,
-8.7434844242914));
#54702=CARTESIAN_POINT('Ctrl Pts',(1.18758896401743,-26.0572974010932,-8.77956970368741));
#54703=CARTESIAN_POINT('Ctrl Pts',(1.97305721072115,-26.0309007595064,-8.84672692345386));
#54704=CARTESIAN_POINT('Ctrl Pts',(2.68446448312301,-25.9962767107602,-8.93633110958157));
#54705=CARTESIAN_POINT('Ctrl Pts',(3.32579714718034,-25.9564745219278,-9.04085572994667));
#54706=CARTESIAN_POINT('Ctrl Pts',(3.90213960567823,-25.9139626268742,-9.15393553592159));
#54707=CARTESIAN_POINT('Ctrl Pts',(4.43120697430674,-25.8694776070166,-9.27369442375866));
#54708=CARTESIAN_POINT('Ctrl Pts',(4.9368483277969,-25.8221884699618,-9.40257105750336));
#54709=CARTESIAN_POINT('Ctrl Pts',(5.43719781099545,-25.7709121598798,-9.54422799064497));
#54710=CARTESIAN_POINT('Ctrl Pts',(5.82250829244966,-25.7280923401021,-9.66446919527306));
#54711=CARTESIAN_POINT('Ctrl Pts',(6.04206701108776,-25.7025208518976,-9.73727734754774));
#54712=CARTESIAN_POINT('Ctrl Pts',(6.09453542110669,-25.6963449753506,-9.75492488947298));
#54713=CARTESIAN_POINT('',(6.2715945487114,-25.5608537657928,-8.76071457496679));
#54714=CARTESIAN_POINT('Origin',(5.999999949026,-24.7867247244533,-9.33250966433407));
#54715=CARTESIAN_POINT('Ctrl Pts',(-6.27159387328033,-25.5608571664718,
-8.76070928018898));
#54716=CARTESIAN_POINT('Ctrl Pts',(-6.13239662748639,-25.5759656514786,
-8.7150479758369));
#54717=CARTESIAN_POINT('Ctrl Pts',(-5.98564488114135,-25.5914802309821,
-8.66855401201454));
#54718=CARTESIAN_POINT('Ctrl Pts',(-5.8313285777228,-25.6072278292077,-8.62173958399663));
#54719=CARTESIAN_POINT('Ctrl Pts',(-5.67907400717005,-25.6227650326784,
-8.57555061707842));
#54720=CARTESIAN_POINT('Ctrl Pts',(-5.5194553658102,-25.638529254758,-8.5290498308945));
#54721=CARTESIAN_POINT('Ctrl Pts',(-5.3524722987654,-25.6543232435974,-8.48276837708628));
#54722=CARTESIAN_POINT('Ctrl Pts',(-5.32566767468479,-25.6568585421822,
-8.47533913894142));
#54723=CARTESIAN_POINT('Ctrl Pts',(-5.29867331186681,-25.6593945386632,
-8.46791563305459));
#54724=CARTESIAN_POINT('Ctrl Pts',(-5.27148923944926,-25.6619303363728,
-8.46050014861381));
#54725=CARTESIAN_POINT('Ctrl Pts',(-5.14595591345888,-25.6736403964273,
-8.42625618356754));
#54726=CARTESIAN_POINT('Ctrl Pts',(-5.01637663597878,-25.6853468539278,
-8.39218216515349));
#54727=CARTESIAN_POINT('Ctrl Pts',(-4.88275737867318,-25.6969639530219,
-8.35851823953318));
#54728=CARTESIAN_POINT('Ctrl Pts',(-4.71106404924362,-25.7118912805792,
-8.31526196354444));
#54729=CARTESIAN_POINT('Ctrl Pts',(-4.53269546289204,-25.7266725141005,
-8.2726803045729));
#54730=CARTESIAN_POINT('Ctrl Pts',(-4.34764543288302,-25.7411116027605,
-8.23131616579629));
#54731=CARTESIAN_POINT('Ctrl Pts',(-4.29584179776617,-25.7451537381783,
-8.21973652567409));
#54732=CARTESIAN_POINT('Ctrl Pts',(-4.24351464845383,-25.749168908436,-8.20825255408196));
#54733=CARTESIAN_POINT('Ctrl Pts',(-4.1906640978516,-25.7531524513767,-8.19687675629923));
#54734=CARTESIAN_POINT('Ctrl Pts',(-4.1433877342813,-25.7567158470692,-8.18670077240217));
#54735=CARTESIAN_POINT('Ctrl Pts',(-4.09569255336367,-25.7602539316812,
-8.17661135076348));
#54736=CARTESIAN_POINT('Ctrl Pts',(-4.04757898367837,-25.763763442795,-8.16661761563247));
#54737=CARTESIAN_POINT('Ctrl Pts',(-3.90056246621801,-25.7744871555712,
-8.13608061442903));
#54738=CARTESIAN_POINT('Ctrl Pts',(-3.74963596581336,-25.7849451013877,
-8.10643536982598));
#54739=CARTESIAN_POINT('Ctrl Pts',(-3.59479965807767,-25.7950405862901,
-8.07795017483715));
#54740=CARTESIAN_POINT('Ctrl Pts',(-3.51738150420983,-25.8000883287413,
-8.06370757734273));
#54741=CARTESIAN_POINT('Ctrl Pts',(-3.43898588989754,-25.8050453466729,
-8.04975523678017));
#54742=CARTESIAN_POINT('Ctrl Pts',(-3.35961278777928,-25.8098988466742,
-8.03612821016658));
#54743=CARTESIAN_POINT('Ctrl Pts',(-3.31992623672015,-25.8123255966748,
-8.02931469685979));
#54744=CARTESIAN_POINT('Ctrl Pts',(-3.27999531131834,-25.8147264547301,
-8.02258252194119));
#54745=CARTESIAN_POINT('Ctrl Pts',(-3.23982000760281,-25.8170997783463,
-8.01593617415272));
#54746=CARTESIAN_POINT('Ctrl Pts',(-3.21973235574504,-25.8182864401545,
-8.01261300025848));
#54747=CARTESIAN_POINT('Ctrl Pts',(-3.19958360915905,-25.8194662175381,
-8.00931128379531));
#54748=CARTESIAN_POINT('Ctrl Pts',(-3.17937376685695,-25.8206389011645,
-8.00603159108714));
#54749=CARTESIAN_POINT('Ctrl Pts',(-3.16169015484261,-25.8216649993376,
-8.00316185996749));
#54750=CARTESIAN_POINT('Ctrl Pts',(-3.1439597664119,-25.8226856663045,-8.00030899082377));
#54751=CARTESIAN_POINT('Ctrl Pts',(-3.12618260080978,-25.8237007603499,
-7.99747336560969));
#54752=CARTESIAN_POINT('Ctrl Pts',(-3.12364300572377,-25.8238457737849,
-7.99706827629339));
#54753=CARTESIAN_POINT('Ctrl Pts',(-3.119862030777,-25.8240613385894,-7.99646617212091));
#54754=CARTESIAN_POINT('Ctrl Pts',(-3.11856095164579,-25.8241354590471,
-7.99625915455978));
#54755=CARTESIAN_POINT('Ctrl Pts',(-3.09161417078269,-25.8256705753082,
-7.99197159301134));
#54756=CARTESIAN_POINT('Ctrl Pts',(-3.06344233361257,-25.8272571050421,
-7.98754642079284));
#54757=CARTESIAN_POINT('Ctrl Pts',(-3.03404546696661,-25.8288893695084,
-7.98299952580576));
#54758=CARTESIAN_POINT('Ctrl Pts',(-2.96197962651402,-25.8328908337468,
-7.97185290216591));
#54759=CARTESIAN_POINT('Ctrl Pts',(-2.88255169635183,-25.8371684006697,
-7.95997137232352));
#54760=CARTESIAN_POINT('Ctrl Pts',(-2.79576131083062,-25.841626199276,-7.94762271516167));
#54761=CARTESIAN_POINT('Ctrl Pts',(-2.70930117926136,-25.8460670351093,
-7.93532104699295));
#54762=CARTESIAN_POINT('Ctrl Pts',(-2.61553427012774,-25.8506867792073,
-7.92255580484241));
#54763=CARTESIAN_POINT('Ctrl Pts',(-2.51446131570232,-25.8553724137153,
-7.9096401288769));
#54764=CARTESIAN_POINT('Ctrl Pts',(-2.50259867559497,-25.855922353075,-7.90812425337299));
#54765=CARTESIAN_POINT('Ctrl Pts',(-2.4906353982387,-25.8564731788712,-7.90660636062048));
#54766=CARTESIAN_POINT('Ctrl Pts',(-2.47857148836738,-25.8570246913402,
-7.90508700081806));
#54767=CARTESIAN_POINT('Ctrl Pts',(-2.3768856639869,-25.861673350081,-7.89228042685596));
#54768=CARTESIAN_POINT('Ctrl Pts',(-2.26804985194134,-25.8663725618713,
-7.8793660063024));
#54769=CARTESIAN_POINT('Ctrl Pts',(-2.1520628455556,-25.8709939026914,-7.86670051264183));
#54770=CARTESIAN_POINT('Ctrl Pts',(-2.11969740242275,-25.8722834587216,
-7.86316628645914));
#54771=CARTESIAN_POINT('Ctrl Pts',(-2.08677517449752,-25.873566836411,-7.85965172837312));
#54772=CARTESIAN_POINT('Ctrl Pts',(-2.05329625573017,-25.8748409749134,
-7.85616525556634));
#54773=CARTESIAN_POINT('Ctrl Pts',(-1.9765681295929,-25.8777610889233,-7.84817483845787));
#54774=CARTESIAN_POINT('Ctrl Pts',(-1.89691552648792,-25.8806329588327,
-7.840331393524));
#54775=CARTESIAN_POINT('Ctrl Pts',(-1.81433840119601,-25.883417618283,-7.83274216281742));
#54776=CARTESIAN_POINT('Ctrl Pts',(-1.81240188497499,-25.8834829213337,
-7.83256418776299));
#54777=CARTESIAN_POINT('Ctrl Pts',(-1.81046376043746,-25.8835481761546,
-7.83238635274822));
#54778=CARTESIAN_POINT('Ctrl Pts',(-1.80852402756431,-25.8836133822471,
-7.83220865924));
#54779=CARTESIAN_POINT('Ctrl Pts',(-1.76910661538462,-25.8849384386295,
-7.8285977402562));
#54780=CARTESIAN_POINT('Ctrl Pts',(-1.72902503616309,-25.8862433884901,
-7.82504522437304));
#54781=CARTESIAN_POINT('Ctrl Pts',(-1.68827931318858,-25.8875239411659,
-7.82156332394353));
#54782=CARTESIAN_POINT('Ctrl Pts',(-1.66690390214362,-25.8881957255352,
-7.8197367014795));
#54783=CARTESIAN_POINT('Ctrl Pts',(-1.6453457107572,-25.8888607906522,-7.81792951673663));
#54784=CARTESIAN_POINT('Ctrl Pts',(-1.62360473988849,-25.8895184934827,
-7.81614356885966));
#54785=CARTESIAN_POINT('Ctrl Pts',(-1.61273425445413,-25.889847344898,-7.81525059492118));
#54786=CARTESIAN_POINT('Ctrl Pts',(-1.60181807411424,-25.8901743553977,
-7.81436293047768));
#54787=CARTESIAN_POINT('Ctrl Pts',(-1.59085619897136,-25.8904994435564,
-7.81348080339152));
#54788=CARTESIAN_POINT('Ctrl Pts',(-1.58537526139992,-25.8906619876357,
-7.81303973984844));
#54789=CARTESIAN_POINT('Ctrl Pts',(-1.57988290012557,-25.8908240511081,
-7.81260006066224));
#54790=CARTESIAN_POINT('Ctrl Pts',(-1.57437911516126,-25.8909856237326,
-7.8121617945058));
#54791=CARTESIAN_POINT('Ctrl Pts',(-1.56887533019695,-25.891147196357,-7.81172352834936));
#54792=CARTESIAN_POINT('Ctrl Pts',(-1.56205960297571,-25.8913460657113,
-7.81118421489639));
#54793=CARTESIAN_POINT('Ctrl Pts',(-1.5578334892067,-25.891468858754,-7.8108512638946));
#54794=CARTESIAN_POINT('Ctrl Pts',(-1.3321001972036,-25.8980277162027,-7.79306704656922));
#54795=CARTESIAN_POINT('Ctrl Pts',(-1.11005352541792,-25.9030588998715,
-7.77943809159168));
#54796=CARTESIAN_POINT('Ctrl Pts',(-0.891696532275825,-25.9066954304679,
-7.76958901908101));
#54797=CARTESIAN_POINT('Ctrl Pts',(-0.848420448729468,-25.9074161529858,
-7.76763703541109));
#54798=CARTESIAN_POINT('Ctrl Pts',(-0.805289186957621,-25.9080820818315,
-7.76583364729354));
#54799=CARTESIAN_POINT('Ctrl Pts',(-0.762302618692336,-25.9086942325735,
-7.76417611600142));
#54800=CARTESIAN_POINT('Ctrl Pts',(-0.724715197699748,-25.9092294966938,
-7.76272677196211));
#54801=CARTESIAN_POINT('Ctrl Pts',(-0.687238390643442,-25.9097236225523,
-7.76138892166378));
#54802=CARTESIAN_POINT('Ctrl Pts',(-0.649872395352755,-25.9101771897174,
-7.76016066762126));
#54803=CARTESIAN_POINT('Ctrl Pts',(-0.558062488216829,-25.9112916243521,
-7.75714279298135));
#54804=CARTESIAN_POINT('Ctrl Pts',(-0.466921605523578,-25.9121612251801,
-7.75478648506841));
#54805=CARTESIAN_POINT('Ctrl Pts',(-0.376448981809044,-25.912796745889,
-7.75306363614118));
#54806=CARTESIAN_POINT('Ctrl Pts',(-0.312801804844112,-25.9132438325033,
-7.75185161789683));
#54807=CARTESIAN_POINT('Ctrl Pts',(-0.249485514272613,-25.9135750126004,
-7.75095306738243));
#54808=CARTESIAN_POINT('Ctrl Pts',(-0.186500110414278,-25.9137938241859,
-7.75035834249019));
#54809=CARTESIAN_POINT('Ctrl Pts',(-0.155007408485111,-25.9139032299786,
-7.75006098004408));
#54810=CARTESIAN_POINT('Ctrl Pts',(-0.123597428111178,-25.913984541275,
-7.74983957593512));
#54811=CARTESIAN_POINT('Ctrl Pts',(-0.0922701689136151,-25.9140381882415,
-7.74969293845181));
#54812=CARTESIAN_POINT('Ctrl Pts',(-0.0647192814703127,-25.9140853682876,
-7.7495639775117));
#54813=CARTESIAN_POINT('Ctrl Pts',(-0.038338168266232,-25.9141107437916,
-7.74949397649207));
#54814=CARTESIAN_POINT('Ctrl Pts',(-0.0102093428318921,-25.9141157543342,
-7.74947894130717));
#54815=CARTESIAN_POINT('Ctrl Pts',(-0.00635375371269017,-25.9141164411241,
-7.74947688044987));
#54816=CARTESIAN_POINT('Ctrl Pts',(-0.00246532864027055,-25.9141167170767,
-7.74947592678315));
#54817=CARTESIAN_POINT('Ctrl Pts',(0.00146344560313601,-25.914116558326,
-7.74947614275909));
#54818=CARTESIAN_POINT('Ctrl Pts',(0.123999816235535,-25.9141116069754,
-7.74948287893321));
#54819=CARTESIAN_POINT('Ctrl Pts',(0.246532789979175,-25.913695197672,-7.75063931458382));
#54820=CARTESIAN_POINT('Ctrl Pts',(0.369067470035637,-25.9128590922614,
-7.75293722185313));
#54821=CARTESIAN_POINT('Ctrl Pts',(0.644882197451568,-25.9109770929301,
-7.75810960788148));
#54822=CARTESIAN_POINT('Ctrl Pts',(0.920705383094992,-25.906969775555,-7.76906208263353));
#54823=CARTESIAN_POINT('Ctrl Pts',(1.19652643911715,-25.9008589498774,-7.78581258443593));
#54824=CARTESIAN_POINT('Ctrl Pts',(1.22212487704151,-25.9002918155403,-7.78736716727589));
#54825=CARTESIAN_POINT('Ctrl Pts',(1.24772329840508,-25.8997065511409,-7.78897172567729));
#54826=CARTESIAN_POINT('Ctrl Pts',(1.27332169550984,-25.8991031670055,-7.79062629563441));
#54827=CARTESIAN_POINT('Ctrl Pts',(1.37083378686459,-25.8968046930544,-7.79692905655149));
#54828=CARTESIAN_POINT('Ctrl Pts',(1.46834552751268,-25.8942433061664,-7.8039574668929));
#54829=CARTESIAN_POINT('Ctrl Pts',(1.56585687063046,-25.891418310992,-7.81170938496717));
#54830=CARTESIAN_POINT('Ctrl Pts',(1.74018381696231,-25.8863678956618,-7.82556795939445));
#54831=CARTESIAN_POINT('Ctrl Pts',(1.91451114826134,-25.8804759883749,-7.84173976099296));
#54832=CARTESIAN_POINT('Ctrl Pts',(2.08883802674337,-25.8737418647172,-7.86022512769866));
#54833=CARTESIAN_POINT('Ctrl Pts',(2.17524324653938,-25.8704040923677,-7.86938741057279));
#54834=CARTESIAN_POINT('Ctrl Pts',(2.26164833787882,-25.866859375497,-7.87911818625325));
#54835=CARTESIAN_POINT('Ctrl Pts',(2.34805359177775,-25.8631079380462,-7.88941699555171));
#54836=CARTESIAN_POINT('Ctrl Pts',(2.47841969237041,-25.8574478624142,-7.90495558317692));
#54837=CARTESIAN_POINT('Ctrl Pts',(2.60878583208703,-25.8513174296,-7.92178731761465));
#54838=CARTESIAN_POINT('Ctrl Pts',(2.73915198362067,-25.8447165664372,-7.93991205113027));
#54839=CARTESIAN_POINT('Ctrl Pts',(2.77255027453888,-25.8430255021109,-7.94455539693475));
#54840=CARTESIAN_POINT('Ctrl Pts',(2.80594857215923,-25.8413035482865,-7.94928360557479));
#54841=CARTESIAN_POINT('Ctrl Pts',(2.83934685804493,-25.839550699752,-7.95409669970059));
#54842=CARTESIAN_POINT('Ctrl Pts',(2.87113163810415,-25.8378825331479,-7.9586772682578));
#54843=CARTESIAN_POINT('Ctrl Pts',(2.90291640750873,-25.8361863848123,-7.96333471870051));
#54844=CARTESIAN_POINT('Ctrl Pts',(2.93470118226646,-25.8344622612576,-7.9680690215513));
#54845=CARTESIAN_POINT('Ctrl Pts',(2.98358847357107,-25.8318104340509,-7.97535072306892));
#54846=CARTESIAN_POINT('Ctrl Pts',(3.03247576140606,-25.8290924419971,-7.98281424467595));
#54847=CARTESIAN_POINT('Ctrl Pts',(3.08136305166704,-25.8263083279687,-7.99045953951483));
#54848=CARTESIAN_POINT('Ctrl Pts',(3.09765881508736,-25.8253802899592,-7.99300797112779));
#54849=CARTESIAN_POINT('Ctrl Pts',(3.11203760519597,-25.8245558042673,-7.99527206014206));
#54850=CARTESIAN_POINT('Ctrl Pts',(3.13025034275539,-25.8235021734813,-7.99816542476062));
#54851=CARTESIAN_POINT('Ctrl Pts',(3.25877662888247,-25.8160667590396,-8.01858373955937));
#54852=CARTESIAN_POINT('Ctrl Pts',(3.38588318060853,-25.8082995024302,-8.04008654538536));
#54853=CARTESIAN_POINT('Ctrl Pts',(3.51155623329027,-25.8002302720259,-8.06258873711801));
#54854=CARTESIAN_POINT('Ctrl Pts',(3.7138153469081,-25.7872435946569,-8.09880392611186));
#54855=CARTESIAN_POINT('Ctrl Pts',(3.91236064810576,-25.7734753352644,-8.1376067494722));
#54856=CARTESIAN_POINT('Ctrl Pts',(4.10715837540643,-25.7590471476669,-8.1786507566697));
#54857=CARTESIAN_POINT('Ctrl Pts',(4.29250871330393,-25.7453187049201,-8.21770419280647));
#54858=CARTESIAN_POINT('Ctrl Pts',(4.47446644684118,-25.7309927563673,-8.25878685121989));
#54859=CARTESIAN_POINT('Ctrl Pts',(4.65302175618465,-25.7161700471708,-8.30161450758188));
#54860=CARTESIAN_POINT('Ctrl Pts',(4.83066123692135,-25.7014233651795,-8.34422249647499));
#54861=CARTESIAN_POINT('Ctrl Pts',(5.00493325561088,-25.6861850570542,-8.38855772601219));
#54862=CARTESIAN_POINT('Ctrl Pts',(5.17584377090514,-25.6705512675105,-8.43435749453037));
#54863=CARTESIAN_POINT('Ctrl Pts',(5.35321544765739,-25.6543264526676,-8.48188869366663));
#54864=CARTESIAN_POINT('Ctrl Pts',(5.52696673857987,-25.637675856963,-8.53099734398442));
#54865=CARTESIAN_POINT('Ctrl Pts',(5.69711918676562,-25.6207045183267,-8.58141278880069));
#54866=CARTESIAN_POINT('Ctrl Pts',(5.87745056215045,-25.6027179135436,-8.63484420634003));
#54867=CARTESIAN_POINT('Ctrl Pts',(6.05373965417498,-25.5843713774276,-8.6897436347901));
#54868=CARTESIAN_POINT('Ctrl Pts',(6.22602530087962,-25.5657888055731,-8.74582073094045));
#54869=CARTESIAN_POINT('Ctrl Pts',(6.24124677966927,-25.56414703083,-8.7507751560244));
#54870=CARTESIAN_POINT('Ctrl Pts',(6.25643701466447,-25.5625034022857,-8.75573878175259));
#54871=CARTESIAN_POINT('Ctrl Pts',(6.27159604017614,-25.5608580130601,-8.76071143363601));
#54872=CARTESIAN_POINT('Origin',(5.999999999061,-24.7867247845918,-9.33250979146072));
#54873=CARTESIAN_POINT('Origin',(5.99996968604069,-24.7866936472161,-9.33251391760964));
#54874=CARTESIAN_POINT('Ctrl Pts',(6.2381662493015,-15.8434653591368,-3.89871982521923));
#54875=CARTESIAN_POINT('Ctrl Pts',(6.28270685588528,-15.8280466725275,-3.90962901102358));
#54876=CARTESIAN_POINT('Ctrl Pts',(6.4154468492204,-15.7792172453928,-3.95133964265943));
#54877=CARTESIAN_POINT('Ctrl Pts',(6.62496348493694,-15.6869699783287,-4.06531809963326));
#54878=CARTESIAN_POINT('Ctrl Pts',(6.83862806647333,-15.5655783391514,-4.26654921887387));
#54879=CARTESIAN_POINT('Ctrl Pts',(6.99712296257017,-15.442135225343,-4.51768655011421));
#54880=CARTESIAN_POINT('Ctrl Pts',(7.08874537959131,-15.3284821169024,-4.79018566349332));
#54881=CARTESIAN_POINT('Ctrl Pts',(7.11061770868682,-15.2560930725951,-4.99096328383844));
#54882=CARTESIAN_POINT('Ctrl Pts',(7.10961146250444,-15.222090971502,-5.09378162079904));
#54883=CARTESIAN_POINT('Ctrl Pts',(7.10920395886533,-15.2171853595682,-5.10881479487898));
#54884=CARTESIAN_POINT('Ctrl Pts',(6.03906557358641,-15.2264275198782,-3.86392206373007));
#54885=CARTESIAN_POINT('Ctrl Pts',(6.07822367443455,-15.2128353613506,-3.87323986549437));
#54886=CARTESIAN_POINT('Ctrl Pts',(6.19515881189246,-15.1696984985832,-3.90896870950711));
#54887=CARTESIAN_POINT('Ctrl Pts',(6.38078979300515,-15.0877569698194,-4.00735611687519));
#54888=CARTESIAN_POINT('Ctrl Pts',(6.57124098797509,-14.9794788173172,-4.18254724403121));
#54889=CARTESIAN_POINT('Ctrl Pts',(6.71312520739851,-14.8692976146181,-4.40251563354182));
#54890=CARTESIAN_POINT('Ctrl Pts',(6.7952965756176,-14.7681803773293,-4.64199449680407));
#54891=CARTESIAN_POINT('Ctrl Pts',(6.81486950788481,-14.7042676737426,-4.81843665892518));
#54892=CARTESIAN_POINT('Ctrl Pts',(6.81396801300512,-14.6744725826796,-4.90857742684284));
#54893=CARTESIAN_POINT('Ctrl Pts',(6.81360381237917,-14.6701794058539,-4.9217513094863));
#54894=CARTESIAN_POINT('Ctrl Pts',(6.02069930843359,-14.8094597286314,-3.36567359206999));
#54895=CARTESIAN_POINT('Ctrl Pts',(6.07475684431375,-14.7910755618093,-3.3784527664935));
#54896=CARTESIAN_POINT('Ctrl Pts',(6.23519938320304,-14.7332353813749,-3.42721134903272));
#54897=CARTESIAN_POINT('Ctrl Pts',(6.48547730175931,-14.6258688961522,-3.55919023320549));
#54898=CARTESIAN_POINT('Ctrl Pts',(6.73750978253762,-14.4870496263752,-3.78912848623333));
#54899=CARTESIAN_POINT('Ctrl Pts',(6.92276415304904,-14.3475283510534,-4.07325817936266));
#54900=CARTESIAN_POINT('Ctrl Pts',(7.02943302213632,-14.219745403388,-4.37999050482277));
#54901=CARTESIAN_POINT('Ctrl Pts',(7.05501806254693,-14.1381849340581,-4.60629545051647));
#54902=CARTESIAN_POINT('Ctrl Pts',(7.0538438996794,-14.0996506859718,-4.72280681189381));
#54903=CARTESIAN_POINT('Ctrl Pts',(7.05336593073427,-14.0940854822575,-4.73985802582531));
#54904=CARTESIAN_POINT('Ctrl Pts',(6.19651102201121,-14.8792022748334,-2.74314825562037));
#54905=CARTESIAN_POINT('Ctrl Pts',(6.27563796232849,-14.8526593570817,-2.76209401164177));
#54906=CARTESIAN_POINT('Ctrl Pts',(6.50937290672894,-14.7696970350242,-2.83405688006437));
#54907=CARTESIAN_POINT('Ctrl Pts',(6.8689582011957,-14.6184250149389,-3.02602829313312));
#54908=CARTESIAN_POINT('Ctrl Pts',(7.22557715812671,-14.4261278195948,-3.35437471770514));
#54909=CARTESIAN_POINT('Ctrl Pts',(7.48475247284693,-14.2345643866072,-3.75448887950438));
#54910=CARTESIAN_POINT('Ctrl Pts',(7.63324425106608,-14.0589978633,-4.18314620121717));
#54911=CARTESIAN_POINT('Ctrl Pts',(7.66907320432673,-13.9456327396364,-4.49970129815192));
#54912=CARTESIAN_POINT('Ctrl Pts',(7.66743397918277,-13.891339277167,-4.66374917088238));
#54913=CARTESIAN_POINT('Ctrl Pts',(7.6667623725601,-13.8834801583075,-4.68778504726345));
#54914=CARTESIAN_POINT('',(6.999999953679,-14.796797858554,-4.9296888417313));
#54915=CARTESIAN_POINT('',(6.99999996004463,-14.5427407425438,-3.16613273045081));
#54916=CARTESIAN_POINT('Ctrl Pts',(7.,-14.796797858554,-4.9296888417313));
#54917=CARTESIAN_POINT('Ctrl Pts',(7.,-14.754906007383,-4.82443917935157));
#54918=CARTESIAN_POINT('Ctrl Pts',(7.,-14.7198932163359,-4.72994340387162));
#54919=CARTESIAN_POINT('Ctrl Pts',(7.,-14.692006860887,-4.64804677830323));
#54920=CARTESIAN_POINT('Ctrl Pts',(7.,-14.6780636831625,-4.60709846551903));
#54921=CARTESIAN_POINT('Ctrl Pts',(7.,-14.6658488264905,-4.56931600454163));
#54922=CARTESIAN_POINT('Ctrl Pts',(7.,-14.655164565243,-4.53496157999509));
#54923=CARTESIAN_POINT('Ctrl Pts',(7.,-14.6498224346192,-4.51778436772182));
#54924=CARTESIAN_POINT('Ctrl Pts',(7.,-14.6448613847077,-4.50146376159314));
#54925=CARTESIAN_POINT('Ctrl Pts',(7.,-14.6402500967837,-4.48603013365108));
#54926=CARTESIAN_POINT('Ctrl Pts',(7.,-14.6379444528216,-4.47831331968006));
#54927=CARTESIAN_POINT('Ctrl Pts',(7.,-14.6357262493564,-4.47081825025569));
#54928=CARTESIAN_POINT('Ctrl Pts',(7.,-14.6335913344904,-4.46354849404081));
#54929=CARTESIAN_POINT('Ctrl Pts',(7.,-14.6325238770573,-4.45991361593337));
#54930=CARTESIAN_POINT('Ctrl Pts',(7.,-14.6314772417741,-4.4563350661283));
#54931=CARTESIAN_POINT('Ctrl Pts',(7.,-14.6304509145204,-4.45281327894708));
#54932=CARTESIAN_POINT('Ctrl Pts',(7.,-14.6294245872668,-4.44929149176586));
#54933=CARTESIAN_POINT('Ctrl Pts',(7.,-14.6289298517031,-4.44759316899773));
#54934=CARTESIAN_POINT('Ctrl Pts',(7.,-14.6274323416498,-4.4424186347167));
#54935=CARTESIAN_POINT('Ctrl Pts',(7.,-14.6034721807969,-4.35962608622025));
#54936=CARTESIAN_POINT('Ctrl Pts',(7.,-14.5830070402295,-4.27937186692289));
#54937=CARTESIAN_POINT('Ctrl Pts',(7.,-14.5661203115116,-4.20227971847956));
#54938=CARTESIAN_POINT('Ctrl Pts',(7.,-14.5492335827938,-4.12518757003624));
#54939=CARTESIAN_POINT('Ctrl Pts',(7.,-14.5361411909217,-4.05283234742234));
#54940=CARTESIAN_POINT('Ctrl Pts',(7.,-14.525657599663,-3.98131352903846));
#54941=CARTESIAN_POINT('Ctrl Pts',(7.,-14.5046904171456,-3.83827589227071));
#54942=CARTESIAN_POINT('Ctrl Pts',(7.,-14.4945119231233,-3.69577454270348));
#54943=CARTESIAN_POINT('Ctrl Pts',(7.,-14.4973995817608,-3.55814511608832));
#54944=CARTESIAN_POINT('Ctrl Pts',(7.,-14.5002872403983,-3.42051568947317));
#54945=CARTESIAN_POINT('Ctrl Pts',(7.,-14.5162103430636,-3.28798606398169));
#54946=CARTESIAN_POINT('Ctrl Pts',(7.,-14.5427407867182,-3.16613306625888));
#54947=CARTESIAN_POINT('',(6.24994468128209,-14.8593881421341,-2.7654624279623));
#54948=CARTESIAN_POINT('Ctrl Pts',(6.24994466999289,-14.8593881037488,-2.76546242081725));
#54949=CARTESIAN_POINT('Ctrl Pts',(6.29949253242022,-14.8423128454431,-2.77890846415222));
#54950=CARTESIAN_POINT('Ctrl Pts',(6.34809291873447,-14.8249522944953,-2.79423376364713));
#54951=CARTESIAN_POINT('Ctrl Pts',(6.39576306624784,-14.8073119088175,-2.81137470270461));
#54952=CARTESIAN_POINT('Ctrl Pts',(6.40561146986023,-14.8036674972288,-2.81491593122894));
#54953=CARTESIAN_POINT('Ctrl Pts',(6.4154201217803,-14.8000111072706,-2.81853482140992));
#54954=CARTESIAN_POINT('Ctrl Pts',(6.42518909072932,-14.7963427361861,-2.82223106921286));
#54955=CARTESIAN_POINT('Ctrl Pts',(6.47313505804959,-14.778338420577,-2.84037220337882));
#54956=CARTESIAN_POINT('Ctrl Pts',(6.52012706823349,-14.7600460751789,-2.86037304645751));
#54957=CARTESIAN_POINT('Ctrl Pts',(6.56619556493753,-14.7414556825689,-2.88220221975805));
#54958=CARTESIAN_POINT('Ctrl Pts',(6.59344693697557,-14.7304587162775,-2.89511505532804));
#54959=CARTESIAN_POINT('Ctrl Pts',(6.62037471767466,-14.7193573113327,-2.90866855706025));
#54960=CARTESIAN_POINT('Ctrl Pts',(6.64698065073811,-14.7081484355682,-2.92286341778547));
#54961=CARTESIAN_POINT('Ctrl Pts',(6.69272061293139,-14.6888785399223,-2.94726671126749));
#54962=CARTESIAN_POINT('Ctrl Pts',(6.73750177898171,-14.6692956536967,-2.9735559602869));
#54963=CARTESIAN_POINT('Ctrl Pts',(6.78129414167393,-14.6493873062218,-3.00175771322334));
#54964=CARTESIAN_POINT('Ctrl Pts',(6.80384852332261,-14.6391339095257,-3.01628246274099));
#54965=CARTESIAN_POINT('Ctrl Pts',(6.82614003401257,-14.6287941458886,-3.03131510454672));
#54966=CARTESIAN_POINT('Ctrl Pts',(6.84816042293265,-14.6183662324647,-3.04686275341766));
#54967=CARTESIAN_POINT('Ctrl Pts',(6.89066022810777,-14.5982401442968,-3.07687003668339));
#54968=CARTESIAN_POINT('Ctrl Pts',(6.93215285126177,-14.5777855466898,-3.10879426210764));
#54969=CARTESIAN_POINT('Ctrl Pts',(6.97258071543327,-14.5569859365848,-3.14269338952529));
#54970=CARTESIAN_POINT('Ctrl Pts',(6.98177604604753,-14.5522550586252,-3.15040375688028));
#54971=CARTESIAN_POINT('Ctrl Pts',(6.99091610578742,-14.5475063422576,-3.15821639324445));
#54972=CARTESIAN_POINT('Ctrl Pts',(6.99999987588419,-14.5427396158966,-3.1661321485828));
#54973=CARTESIAN_POINT('',(6.26386081962776,-15.8144408557884,-3.90572621562457));
#54974=CARTESIAN_POINT('Ctrl Pts',(6.26385680272581,-15.8144410175731,-3.90574090061969));
#54975=CARTESIAN_POINT('Ctrl Pts',(6.25434739267814,-15.785035322926,-3.90346327992607));
#54976=CARTESIAN_POINT('Ctrl Pts',(6.24501465448848,-15.7550032667797,-3.89974567582242));
#54977=CARTESIAN_POINT('Ctrl Pts',(6.23596151625569,-15.724517427388,-3.89443848692829));
#54978=CARTESIAN_POINT('Ctrl Pts',(6.22713568305973,-15.6947970225525,-3.88926455025411));
#54979=CARTESIAN_POINT('Ctrl Pts',(6.21857587660778,-15.6646456440639,-3.88257916996334));
#54980=CARTESIAN_POINT('Ctrl Pts',(6.21038339038277,-15.6342633509603,-3.87427169593729));
#54981=CARTESIAN_POINT('Ctrl Pts',(6.20231719059348,-15.6043493981626,-3.86609228087353));
#54982=CARTESIAN_POINT('Ctrl Pts',(6.1946073963697,-15.5742120457398,-3.85633977680809));
#54983=CARTESIAN_POINT('Ctrl Pts',(6.18735199987957,-15.5440761704759,-3.8449456613132));
#54984=CARTESIAN_POINT('Ctrl Pts',(6.18022409990826,-15.5144698622994,-3.83375177058379));
#54985=CARTESIAN_POINT('Ctrl Pts',(6.17353510231177,-15.4848656159052,-3.82097302339114));
#54986=CARTESIAN_POINT('Ctrl Pts',(6.16737434330549,-15.4555016018223,-3.80658826970777));
#54987=CARTESIAN_POINT('Ctrl Pts',(6.16657568470721,-15.451694956845,-3.80472348207339));
#54988=CARTESIAN_POINT('Ctrl Pts',(6.16578589435225,-15.4478923758297,-3.8028317707424));
#54989=CARTESIAN_POINT('Ctrl Pts',(6.16500515775714,-15.444094399648,-3.80091314997598));
#54990=CARTESIAN_POINT('Ctrl Pts',(6.15907432331299,-15.4152432248763,-3.78633842375209));
#54991=CARTESIAN_POINT('Ctrl Pts',(6.15366693892629,-15.3866570736564,-3.77020678733933));
#54992=CARTESIAN_POINT('Ctrl Pts',(6.14885762209861,-15.3585789395669,-3.75255219896567));
#54993=CARTESIAN_POINT('Ctrl Pts',(6.1441072471592,-15.3308449246739,-3.73511398119362));
#54994=CARTESIAN_POINT('Ctrl Pts',(6.13994064449411,-15.3036073583595,-3.71618992922669));
#54995=CARTESIAN_POINT('Ctrl Pts',(6.1364164212586,-15.2771013424223,-3.695861834686));
#54996=CARTESIAN_POINT('Ctrl Pts',(6.1329126344815,-15.2507490310199,-3.67565161981157));
#54997=CARTESIAN_POINT('Ctrl Pts',(6.13004401913192,-15.225120618436,-3.65405381053664));
#54998=CARTESIAN_POINT('Ctrl Pts',(6.1278512193941,-15.2004359938299,-3.63119595624287));
#54999=CARTESIAN_POINT('Ctrl Pts',(6.12566730832878,-15.1758514301367,-3.60843075791641));
#55000=CARTESIAN_POINT('Ctrl Pts',(6.12415388155219,-15.1522037620878,-3.58441614318941));
#55001=CARTESIAN_POINT('Ctrl Pts',(6.12333154166847,-15.1296874723247,-3.55932021761716));
#55002=CARTESIAN_POINT('Ctrl Pts',(6.12302921506252,-15.1214095405384,-3.55009390359353));
#55003=CARTESIAN_POINT('Ctrl Pts',(6.1228200957212,-15.1132842492035,-3.54072181573136));
#55004=CARTESIAN_POINT('Ctrl Pts',(6.12270449763779,-15.1053201949041,-3.53121353501667));
#55005=CARTESIAN_POINT('Ctrl Pts',(6.12239025057169,-15.0836703489532,-3.50536579403046));
#55006=CARTESIAN_POINT('Ctrl Pts',(6.12276865950795,-15.0632149366601,-3.47850974789018));
#55007=CARTESIAN_POINT('Ctrl Pts',(6.12383157496324,-15.044100649971,-3.45085760590152));
#55008=CARTESIAN_POINT('Ctrl Pts',(6.12490061466795,-15.0248762316071,-3.42304613928017));
#55009=CARTESIAN_POINT('Ctrl Pts',(6.12666199158116,-15.0070088394718,-3.39443016446765));
#55010=CARTESIAN_POINT('Ctrl Pts',(6.12908657998587,-14.9906035321586,-3.36524562850755));
#55011=CARTESIAN_POINT('Ctrl Pts',(6.13152236548042,-14.9741224628318,-3.33592631426071));
#55012=CARTESIAN_POINT('Ctrl Pts',(6.13462731787943,-14.9591171667997,-3.30603402985629));
#55013=CARTESIAN_POINT('Ctrl Pts',(6.1383529517025,-14.945645493166,-3.27581569596834));
#55014=CARTESIAN_POINT('Ctrl Pts',(6.14212000873812,-14.9320240356226,-3.24526138153937));
#55015=CARTESIAN_POINT('Ctrl Pts',(6.14652137385283,-14.9199704463401,-3.2143745768921));
#55016=CARTESIAN_POINT('Ctrl Pts',(6.15149089059401,-14.9094939790091,-3.18340537369647));
#55017=CARTESIAN_POINT('Ctrl Pts',(6.15328515498051,-14.9057114075424,-3.17222381595833));
#55018=CARTESIAN_POINT('Ctrl Pts',(6.15515335276949,-14.902133962306,-3.16103140626657));
#55019=CARTESIAN_POINT('Ctrl Pts',(6.15709197107948,-14.8987605391209,-3.14983943667008));
#55020=CARTESIAN_POINT('Ctrl Pts',(6.1625485231329,-14.8892654987031,-3.11833784382476));
#55021=CARTESIAN_POINT('Ctrl Pts',(6.1685631653214,-14.8813901398998,-3.08684159759775));
#55022=CARTESIAN_POINT('Ctrl Pts',(6.17504972278387,-14.8750788685375,-3.05558574897629));
#55023=CARTESIAN_POINT('Ctrl Pts',(6.18168467070373,-14.8686232166698,-3.02361487243744));
#55024=CARTESIAN_POINT('Ctrl Pts',(6.18881302060891,-14.8638035249704,-2.99189615705139));
#55025=CARTESIAN_POINT('Ctrl Pts',(6.19633675700028,-14.8605176411598,-2.96064760775454));
#55026=CARTESIAN_POINT('Ctrl Pts',(6.20397194257905,-14.8571830835174,-2.92893617336372));
#55027=CARTESIAN_POINT('Ctrl Pts',(6.21201396047443,-14.8554273949708,-2.89770931890753));
#55028=CARTESIAN_POINT('Ctrl Pts',(6.22035994366165,-14.8551099062963,-2.86715290245178));
#55029=CARTESIAN_POINT('Ctrl Pts',(6.22890611290103,-14.8547848023651,-2.83586356235581));
#55030=CARTESIAN_POINT('Ctrl Pts',(6.23777067522327,-14.8559669469053,-2.80527742314284));
#55031=CARTESIAN_POINT('Ctrl Pts',(6.2468480287175,-14.8584814517712,-2.77554561910762));
#55032=CARTESIAN_POINT('Ctrl Pts',(6.24787754648693,-14.8587666370339,-2.77217355470682));
#55033=CARTESIAN_POINT('Ctrl Pts',(6.24890980941479,-14.8590689433739,-2.76881242822435));
#55034=CARTESIAN_POINT('Ctrl Pts',(6.24994466999289,-14.8593881037488,-2.76546242081725));
#55035=CARTESIAN_POINT('Ctrl Pts',(6.26385680289834,-15.8144410175599,-3.90574090066702));
#55036=CARTESIAN_POINT('Ctrl Pts',(6.29464231014065,-15.7946386727068,-3.91437791970859));
#55037=CARTESIAN_POINT('Ctrl Pts',(6.32519901986354,-15.7740985767096,-3.92458862745004));
#55038=CARTESIAN_POINT('Ctrl Pts',(6.35535969010304,-15.7528444265997,-3.93639986371284));
#55039=CARTESIAN_POINT('Ctrl Pts',(6.39985352172865,-15.7214897329266,-3.95382411700011));
#55040=CARTESIAN_POINT('Ctrl Pts',(6.44348728197708,-15.6885800104884,-3.97473232893006));
#55041=CARTESIAN_POINT('Ctrl Pts',(6.48575810107706,-15.6542249774097,-3.9990727963858));
#55042=CARTESIAN_POINT('Ctrl Pts',(6.51303557488992,-15.6320555817108,-4.01477976582129));
#55043=CARTESIAN_POINT('Ctrl Pts',(6.53974464965851,-15.6092847175838,-4.03191581203157));
#55044=CARTESIAN_POINT('Ctrl Pts',(6.56573941608896,-15.5859462401836,-4.05046724920638));
#55045=CARTESIAN_POINT('Ctrl Pts',(6.56926098315705,-15.5827845263189,-4.05298045240809));
#55046=CARTESIAN_POINT('Ctrl Pts',(6.57276942762224,-15.5796124004499,-4.05551963423667));
#55047=CARTESIAN_POINT('Ctrl Pts',(6.57626437337287,-15.5764299517938,-4.05808476273979));
#55048=CARTESIAN_POINT('Ctrl Pts',(6.61460947149103,-15.5415134424451,-4.08622829089611));
#55049=CARTESIAN_POINT('Ctrl Pts',(6.65133308425788,-15.5053526401255,-4.11749543403956));
#55050=CARTESIAN_POINT('Ctrl Pts',(6.68600408697268,-15.4680864724447,-4.15172691181702));
#55051=CARTESIAN_POINT('Ctrl Pts',(6.7111562078007,-15.4410516860551,-4.17656017874796));
#55052=CARTESIAN_POINT('Ctrl Pts',(6.73522739077866,-15.4134355611798,-4.20295334288734));
#55053=CARTESIAN_POINT('Ctrl Pts',(6.75803716642575,-15.3852981854079,-4.23084617397227));
#55054=CARTESIAN_POINT('Ctrl Pts',(6.75931380622222,-15.3837233652854,-4.23240730717894));
#55055=CARTESIAN_POINT('Ctrl Pts',(6.76058649060395,-15.3821469139671,-4.23397313859397));
#55056=CARTESIAN_POINT('Ctrl Pts',(6.76185518645526,-15.3805688425827,-4.23554365783243));
#55057=CARTESIAN_POINT('Ctrl Pts',(6.7700468794139,-15.3703795791482,-4.24568415870487));
#55058=CARTESIAN_POINT('Ctrl Pts',(6.77807230818569,-15.3601227655933,-4.25602009707487));
#55059=CARTESIAN_POINT('Ctrl Pts',(6.78592456218493,-15.3498016129747,-4.26654660476092));
#55060=CARTESIAN_POINT('Ctrl Pts',(6.79045875165238,-15.3438417877449,-4.27262500980026));
#55061=CARTESIAN_POINT('Ctrl Pts',(6.79493519828708,-15.3378605072598,-4.27876696178125));
#55062=CARTESIAN_POINT('Ctrl Pts',(6.79935253216999,-15.3318584131363,-4.28497151510868));
#55063=CARTESIAN_POINT('Ctrl Pts',(6.80156119911144,-15.3288573660746,-4.28807379177239));
#55064=CARTESIAN_POINT('Ctrl Pts',(6.8037550875957,-15.3258511156132,-4.29119171892957));
#55065=CARTESIAN_POINT('Ctrl Pts',(6.80593402451752,-15.3228397423737,-4.2943251791777));
#55066=CARTESIAN_POINT('Ctrl Pts',(6.80759005980613,-15.3205510389688,-4.29670667113113));
#55067=CARTESIAN_POINT('Ctrl Pts',(6.80965642237721,-15.3176739784075,-4.29970838286095));
#55068=CARTESIAN_POINT('Ctrl Pts',(6.81117695486563,-15.3155432926217,-4.30193722155344));
#55069=CARTESIAN_POINT('Ctrl Pts',(6.81165707079494,-15.3148705176603,-4.30264098879832));
#55070=CARTESIAN_POINT('Ctrl Pts',(6.81208312885854,-15.3142721780336,-4.30326741588872));
#55071=CARTESIAN_POINT('Ctrl Pts',(6.81242580594044,-15.3137903355188,-4.3037720420517));
#55072=CARTESIAN_POINT('Ctrl Pts',(6.82705299909326,-15.2932228569605,-4.32531204208564));
#55073=CARTESIAN_POINT('Ctrl Pts',(6.84166190719415,-15.2714248648976,-4.34856896054824));
#55074=CARTESIAN_POINT('Ctrl Pts',(6.85595717412585,-15.2484182524569,-4.373666513424));
#55075=CARTESIAN_POINT('Ctrl Pts',(6.86936271662908,-15.2268435506759,-4.3972020174066));
#55076=CARTESIAN_POINT('Ctrl Pts',(6.88249251343736,-15.2042058902949,-4.42235627841688));
#55077=CARTESIAN_POINT('Ctrl Pts',(6.89505966326525,-15.1805403619258,-4.44921795667627));
#55078=CARTESIAN_POINT('Ctrl Pts',(6.89589374366113,-15.1789696833279,-4.45100076340202));
#55079=CARTESIAN_POINT('Ctrl Pts',(6.89672532848846,-15.1773944839582,-4.45279108572735));
#55080=CARTESIAN_POINT('Ctrl Pts',(6.89755432638955,-15.1758147771217,-4.45458894715883));
#55081=CARTESIAN_POINT('Ctrl Pts',(6.90969329051585,-15.1526832292701,-4.48091491902407));
#55082=CARTESIAN_POINT('Ctrl Pts',(6.92128063254415,-15.1285834265236,-4.50885955213998));
#55083=CARTESIAN_POINT('Ctrl Pts',(6.93203465924816,-15.103570623826,-4.53846268874816));
#55084=CARTESIAN_POINT('Ctrl Pts',(6.93454271509536,-15.0977371339354,-4.54536673705574));
#55085=CARTESIAN_POINT('Ctrl Pts',(6.93700528186122,-15.0918540797584,-4.55236087968532));
#55086=CARTESIAN_POINT('Ctrl Pts',(6.93941847433871,-15.0859223430359,-4.55944540688696));
#55087=CARTESIAN_POINT('Ctrl Pts',(6.94912526570966,-15.062062608941,-4.58794210913917));
#55088=CARTESIAN_POINT('Ctrl Pts',(6.95803613112938,-15.0374135620583,-4.61790307748903));
#55089=CARTESIAN_POINT('Ctrl Pts',(6.96587583092441,-15.0120452933159,-4.64933257084334));
#55090=CARTESIAN_POINT('Ctrl Pts',(6.9693799351623,-15.0007064588793,-4.66338058591238));
#55091=CARTESIAN_POINT('Ctrl Pts',(6.97266954009498,-14.9892242191139,-4.67772166388442));
#55092=CARTESIAN_POINT('Ctrl Pts',(6.97571741922449,-14.9776062938991,-4.69235455327343));
#55093=CARTESIAN_POINT('Ctrl Pts',(6.98225036636205,-14.9527039640981,-4.72371927896829));
#55094=CARTESIAN_POINT('Ctrl Pts',(6.98767463465472,-14.9271766313242,-4.75642696399957));
#55095=CARTESIAN_POINT('Ctrl Pts',(6.99173368562324,-14.901120484089,-4.79041861766872));
#55096=CARTESIAN_POINT('Ctrl Pts',(6.99559723923891,-14.8763192872967,-4.82277312059423));
#55097=CARTESIAN_POINT('Ctrl Pts',(6.99822422923869,-14.851038940224,-4.85629082491783));
#55098=CARTESIAN_POINT('Ctrl Pts',(6.99936263918771,-14.8253844806674,-4.89089220479161));
#55099=CARTESIAN_POINT('Ctrl Pts',(6.99968896476072,-14.8180306216972,-4.90081070130889));
#55100=CARTESIAN_POINT('Ctrl Pts',(6.99989275741611,-14.8106461698658,-4.91081805718665));
#55101=CARTESIAN_POINT('Ctrl Pts',(6.99996751968053,-14.8032339673454,-4.92091194510101));
#55102=CARTESIAN_POINT('Ctrl Pts',(6.99998913554391,-14.8010908921153,-4.9238303706439));
#55103=CARTESIAN_POINT('Ctrl Pts',(6.99999996330327,-14.7989454981677,-4.92675602852862));
#55104=CARTESIAN_POINT('Ctrl Pts',(6.99999987085796,-14.7967978585547,-4.92968884172919));
#55105=CARTESIAN_POINT('Ctrl Pts',(6.99990204847876,-14.6847053727042,-4.95612542422809));
#55106=CARTESIAN_POINT('Ctrl Pts',(6.99990204847876,-15.0109966856309,-4.91843511379028));
#55107=CARTESIAN_POINT('Ctrl Pts',(6.99990204847876,-15.8988773644907,-4.8561641130756));
#55108=CARTESIAN_POINT('Ctrl Pts',(6.99990204847876,-17.3517264997127,-4.93000583026503));
#55109=CARTESIAN_POINT('Ctrl Pts',(6.99990204847876,-19.0057036593414,-5.27370352517816));
#55110=CARTESIAN_POINT('Ctrl Pts',(6.99990204847876,-20.5902612526977,-5.86661657541822));
#55111=CARTESIAN_POINT('Ctrl Pts',(6.99990204847876,-22.0651320115504,-6.69609676488873));
#55112=CARTESIAN_POINT('Ctrl Pts',(6.99990204847876,-23.3944663504207,-7.73957935185531));
#55113=CARTESIAN_POINT('Ctrl Pts',(6.99990204847876,-24.2870419231056,-8.69530609464369));
#55114=CARTESIAN_POINT('Ctrl Pts',(6.99990204847876,-24.7366373563668,-9.28612088063576));
#55115=CARTESIAN_POINT('Ctrl Pts',(6.99990204847876,-24.8428462632706,-9.43308828770487));
#55116=CARTESIAN_POINT('Ctrl Pts',(7.00659078506582,-14.6298576689916,-4.48143047120262));
#55117=CARTESIAN_POINT('Ctrl Pts',(7.00659078506582,-14.9704072356705,-4.44209164486882));
#55118=CARTESIAN_POINT('Ctrl Pts',(7.00659078506582,-15.8968485520861,-4.37713026806021));
#55119=CARTESIAN_POINT('Ctrl Pts',(7.00659078506582,-17.4127173390504,-4.45416586533225));
#55120=CARTESIAN_POINT('Ctrl Pts',(7.00659078506582,-19.1390748339291,-4.81286872482972));
#55121=CARTESIAN_POINT('Ctrl Pts',(7.00659078506582,-20.792516687395,-5.43161542968116));
#55122=CARTESIAN_POINT('Ctrl Pts',(7.00659078506582,-22.3315011340853,-6.29709341005203));
#55123=CARTESIAN_POINT('Ctrl Pts',(7.00659078506582,-23.7189804924501,-7.38626117312299));
#55124=CARTESIAN_POINT('Ctrl Pts',(7.00659078506582,-24.6502122945406,-8.38339439103266));
#55125=CARTESIAN_POINT('Ctrl Pts',(7.00659078506582,-25.1193210874972,-8.99983838783685));
#55126=CARTESIAN_POINT('Ctrl Pts',(7.00659078506582,-25.2301483657287,-9.15319520571074));
#55127=CARTESIAN_POINT('Ctrl Pts',(6.71769910521849,-14.5861379424571,-4.10304574168264));
#55128=CARTESIAN_POINT('Ctrl Pts',(6.71769910521849,-14.9380529248673,-4.06239286463224));
#55129=CARTESIAN_POINT('Ctrl Pts',(6.71769910521849,-15.8952313627117,-3.99528695853561));
#55130=CARTESIAN_POINT('Ctrl Pts',(6.71769910521849,-17.4613338286547,-4.07486843383928));
#55131=CARTESIAN_POINT('Ctrl Pts',(6.71769910521849,-19.2453865094556,-4.44553208016281));
#55132=CARTESIAN_POINT('Ctrl Pts',(6.71769910521849,-20.9537367877186,-5.0848710840269));
#55133=CARTESIAN_POINT('Ctrl Pts',(6.71769910521849,-22.5438269819634,-5.97904331169807));
#55134=CARTESIAN_POINT('Ctrl Pts',(6.71769910521849,-23.9776543946596,-7.10462724665685));
#55135=CARTESIAN_POINT('Ctrl Pts',(6.71769910521849,-24.9396995155246,-8.13476603538479));
#55136=CARTESIAN_POINT('Ctrl Pts',(6.71769910521849,-25.424362628746,-8.77163936672992));
#55137=CARTESIAN_POINT('Ctrl Pts',(6.71769910521849,-25.5388712631324,-8.93008925640513));
#55138=CARTESIAN_POINT('Ctrl Pts',(6.25532321980198,-14.5721230213941,-3.98174964636385));
#55139=CARTESIAN_POINT('Ctrl Pts',(6.25532321980198,-14.9276813340999,-3.94067553344174));
#55140=CARTESIAN_POINT('Ctrl Pts',(6.25532321980198,-15.8947129518397,-3.87288217087801));
#55141=CARTESIAN_POINT('Ctrl Pts',(6.25532321980198,-17.4769184701448,-3.95327976015244));
#55142=CARTESIAN_POINT('Ctrl Pts',(6.25532321980198,-19.2794660854095,-4.32777759064623));
#55143=CARTESIAN_POINT('Ctrl Pts',(6.25532321980198,-21.0054179659765,-4.97371772100629));
#55144=CARTESIAN_POINT('Ctrl Pts',(6.25532321980198,-22.6118907653904,-5.87708825897841));
#55145=CARTESIAN_POINT('Ctrl Pts',(6.25532321980198,-24.0605756434636,-7.01434586655842));
#55146=CARTESIAN_POINT('Ctrl Pts',(6.25532321980198,-25.0324983702633,-8.05506501583201));
#55147=CARTESIAN_POINT('Ctrl Pts',(6.25532321980198,-25.5221476210515,-8.69848723331493));
#55148=CARTESIAN_POINT('Ctrl Pts',(6.25532321980198,-25.6378363615289,-8.85856977270761));
#55149=CARTESIAN_POINT('Ctrl Pts',(7.0000000000004,-14.796797858554,-4.92968884173129));
#55150=CARTESIAN_POINT('Ctrl Pts',(7.0000000000004,-14.9621718211134,-4.91233286861492));
#55151=CARTESIAN_POINT('Ctrl Pts',(6.99999999998289,-15.1274388227087,-4.89876704773387));
#55152=CARTESIAN_POINT('Ctrl Pts',(6.9999999993942,-15.2926819700917,-4.88893416787038));
#55153=CARTESIAN_POINT('Ctrl Pts',(6.99999999894932,-15.4175591375174,-4.88150328674497));
#55154=CARTESIAN_POINT('Ctrl Pts',(6.99999999821322,-15.5424229437211,-4.87620540119634));
#55155=CARTESIAN_POINT('Ctrl Pts',(6.99999999796755,-15.6673108058121,-4.87303547957403));
#55156=CARTESIAN_POINT('Ctrl Pts',(6.99999999764153,-15.8330446050339,-4.86882880051888));
#55157=CARTESIAN_POINT('Ctrl Pts',(6.99999999919545,-15.9988211310191,-4.86836780068467));
#55158=CARTESIAN_POINT('Ctrl Pts',(6.99999999987699,-16.1647597219873,-4.87168759212841));
#55159=CARTESIAN_POINT('Ctrl Pts',(6.99999999995264,-16.1831793000345,-4.87205609687008));
#55160=CARTESIAN_POINT('Ctrl Pts',(7.00000000000042,-16.2016008696669,-4.87247123934923));
#55161=CARTESIAN_POINT('Ctrl Pts',(7.00000000000042,-16.2200245895141,-4.87293310700196));
#55162=CARTESIAN_POINT('Ctrl Pts',(7.00000000000042,-16.4234357726081,-4.87803245970895));
#55163=CARTESIAN_POINT('Ctrl Pts',(6.99999999555751,-16.6270899052425,-4.8887471286057));
#55164=CARTESIAN_POINT('Ctrl Pts',(6.99999999493389,-16.8304432106282,-4.90512255000003));
#55165=CARTESIAN_POINT('Ctrl Pts',(6.99999999440532,-17.0028030857336,-4.91900216499311));
#55166=CARTESIAN_POINT('Ctrl Pts',(6.99999999611259,-17.1749465731231,-4.93694763771438));
#55167=CARTESIAN_POINT('Ctrl Pts',(6.99999999794676,-17.3465425019982,-4.95895729935852));
#55168=CARTESIAN_POINT('Ctrl Pts',(6.99999999900155,-17.4452234773389,-4.9716145628041));
#55169=CARTESIAN_POINT('Ctrl Pts',(7.00000000000042,-17.5437233863106,-4.9856154106428));
#55170=CARTESIAN_POINT('Ctrl Pts',(7.00000000000042,-17.6419802648722,-5.00094556168401));
#55171=CARTESIAN_POINT('Ctrl Pts',(7.00000000000042,-17.9008409010356,-5.04133329543972));
#55172=CARTESIAN_POINT('Ctrl Pts',(6.99999999747738,-18.158010911339,-5.09103787417142));
#55173=CARTESIAN_POINT('Ctrl Pts',(6.99999999839647,-18.4130245932067,-5.14984752267489));
#55174=CARTESIAN_POINT('Ctrl Pts',(6.99999999910283,-18.6090113775211,-5.19504475998561));
#55175=CARTESIAN_POINT('Ctrl Pts',(6.99999999994416,-18.8037248579095,-5.2456209122658));
#55176=CARTESIAN_POINT('Ctrl Pts',(6.99999999999558,-18.9969550950569,-5.30150070689851));
#55177=CARTESIAN_POINT('Ctrl Pts',(6.99999999999892,-19.0094781659271,-5.30512222410372));
#55178=CARTESIAN_POINT('Ctrl Pts',(7.00000000000042,-19.0219950067074,-5.30876602405832));
#55179=CARTESIAN_POINT('Ctrl Pts',(7.00000000000042,-19.0345055606664,-5.3124320838912));
#55180=CARTESIAN_POINT('Ctrl Pts',(7.00000000000042,-19.37829694462,-5.41317580696964));
#55181=CARTESIAN_POINT('Ctrl Pts',(7.00000000000848,-19.717337955919,-5.53070296422703));
#55182=CARTESIAN_POINT('Ctrl Pts',(6.99999999997893,-20.0498647476411,-5.66455067298009));
#55183=CARTESIAN_POINT('Ctrl Pts',(6.99999999996922,-20.159096338497,-5.70851825250593));
#55184=CARTESIAN_POINT('Ctrl Pts',(7.00000000000042,-20.2676248241435,-5.75424653186144));
#55185=CARTESIAN_POINT('Ctrl Pts',(7.00000000000042,-20.3753872113398,-5.80171797264263));
#55186=CARTESIAN_POINT('Ctrl Pts',(7.00000000000042,-20.4431561669975,-5.83157152404412));
#55187=CARTESIAN_POINT('Ctrl Pts',(6.99999999997258,-20.5106234743014,-5.86211220561406));
#55188=CARTESIAN_POINT('Ctrl Pts',(6.99999999993318,-20.5777739523651,-5.89333485504115));
#55189=CARTESIAN_POINT('Ctrl Pts',(6.99999999971921,-20.9424626713701,-6.06290249404886));
#55190=CARTESIAN_POINT('Ctrl Pts',(7.00000000000042,-21.2978034884988,-6.25258824524381));
#55191=CARTESIAN_POINT('Ctrl Pts',(7.00000000000042,-21.6416259231186,-6.46100648199057));
#55192=CARTESIAN_POINT('Ctrl Pts',(7.00000000000042,-21.7794446663838,-6.54454942907526));
#55193=CARTESIAN_POINT('Ctrl Pts',(6.99999999962401,-21.9154122185717,-6.63110373594479));
#55194=CARTESIAN_POINT('Ctrl Pts',(6.9999999991279,-22.0494161776191,-6.72060846296995));
#55195=CARTESIAN_POINT('Ctrl Pts',(6.99999999825563,-22.2850230329977,-6.87797640512509));
#55196=CARTESIAN_POINT('Ctrl Pts',(6.99999999886891,-22.51456232569,-7.04446337791262));
#55197=CARTESIAN_POINT('Ctrl Pts',(6.99999999982076,-22.7374335824926,-7.21972686077438));
#55198=CARTESIAN_POINT('Ctrl Pts',(6.99999999992681,-22.7622653187281,-7.23925426256033));
#55199=CARTESIAN_POINT('Ctrl Pts',(7.00000000000042,-22.7870142347845,-7.25889064419841));
#55200=CARTESIAN_POINT('Ctrl Pts',(7.00000000000042,-22.8116794661682,-7.27863555348144));
#55201=CARTESIAN_POINT('Ctrl Pts',(7.00000000000042,-22.9843713301579,-7.41687813208722));
#55202=CARTESIAN_POINT('Ctrl Pts',(6.99999999634688,-23.1529951472481,-7.56040930321861));
#55203=CARTESIAN_POINT('Ctrl Pts',(6.99999999542238,-23.3170682079529,-7.70885139832025));
#55204=CARTESIAN_POINT('Ctrl Pts',(6.9999999953121,-23.3366383426619,-7.7265571190836));
#55205=CARTESIAN_POINT('Ctrl Pts',(6.9999999952367,-23.3561437763943,-7.74433266391942));
#55206=CARTESIAN_POINT('Ctrl Pts',(6.99999999520118,-23.3755837254306,-7.76217735716987));
#55207=CARTESIAN_POINT('Ctrl Pts',(6.9999999948931,-23.5442002619243,-7.91695710299456));
#55208=CARTESIAN_POINT('Ctrl Pts',(7.00000000000042,-23.7078863139086,-8.07694208893929));
#55209=CARTESIAN_POINT('Ctrl Pts',(7.00000000000042,-23.8662409010678,-8.24158764729914));
#55210=CARTESIAN_POINT('Ctrl Pts',(7.00000000000042,-23.9842449793353,-8.36427968738245));
#55211=CARTESIAN_POINT('Ctrl Pts',(6.99999999741473,-24.0992427801723,-8.48959370330393));
#55212=CARTESIAN_POINT('Ctrl Pts',(6.99999999745776,-24.2113303506499,-8.61757573537637));
#55213=CARTESIAN_POINT('Ctrl Pts',(6.99999999749883,-24.3183213987655,-8.73973853802289));
#55214=CARTESIAN_POINT('Ctrl Pts',(6.99999999865173,-24.4226608384595,-8.86433273762792));
#55215=CARTESIAN_POINT('Ctrl Pts',(6.99999999924105,-24.5244006140281,-8.99142942662163));
#55216=CARTESIAN_POINT('Ctrl Pts',(6.99999999975917,-24.6138492002674,-9.10317155581979));
#55217=CARTESIAN_POINT('Ctrl Pts',(6.99999999990904,-24.7012880004826,-9.21684861925867));
#55218=CARTESIAN_POINT('Ctrl Pts',(6.99999999989438,-24.7867157006584,-9.33251047983016));
#55219=CARTESIAN_POINT('Ctrl Pts',(6.26386081962776,-15.8144408557884,-3.90572621562457));
#55220=CARTESIAN_POINT('Ctrl Pts',(6.2646071586712,-16.0736409969805,-3.9030665414647));
#55221=CARTESIAN_POINT('Ctrl Pts',(6.26531568823028,-16.3306820728263,-3.90881653564373));
#55222=CARTESIAN_POINT('Ctrl Pts',(6.26598639114327,-16.5850710475842,-3.92256329479193));
#55223=CARTESIAN_POINT('Ctrl Pts',(6.26666474239918,-16.8423609402882,-3.93646681474453));
#55224=CARTESIAN_POINT('Ctrl Pts',(6.26730439940407,-17.0969379570018,-3.95855050562228));
#55225=CARTESIAN_POINT('Ctrl Pts',(6.26790534774945,-17.3483447734508,-3.98839371483313));
#55226=CARTESIAN_POINT('Ctrl Pts',(6.26800177179145,-17.3886837836389,-3.99318215111106));
#55227=CARTESIAN_POINT('Ctrl Pts',(6.26809719927749,-17.4289412844092,-3.9981703715966));
#55228=CARTESIAN_POINT('Ctrl Pts',(6.26819163015533,-17.4691155095948,-4.00335665446775));
#55229=CARTESIAN_POINT('Ctrl Pts',(6.26876871904396,-17.7146294717142,-4.03505122606151));
#55230=CARTESIAN_POINT('Ctrl Pts',(6.26930858726239,-17.9570293256807,-4.07414120498853));
#55231=CARTESIAN_POINT('Ctrl Pts',(6.26981122436712,-18.1959065670098,-4.12010977122704));
#55232=CARTESIAN_POINT('Ctrl Pts',(6.2701791280684,-18.3707520378482,-4.15375632358596));
#55233=CARTESIAN_POINT('Ctrl Pts',(6.27052708539201,-18.5437113313115,-4.19108847665381));
#55234=CARTESIAN_POINT('Ctrl Pts',(6.27085509303089,-18.7146405947199,-4.23191026973416));
#55235=CARTESIAN_POINT('Ctrl Pts',(6.2712113775946,-18.9003053501125,-4.27625123321704));
#55236=CARTESIAN_POINT('Ctrl Pts',(6.27154412351328,-19.0835747569271,-4.32470934801864));
#55237=CARTESIAN_POINT('Ctrl Pts',(6.27185332670676,-19.2642821898755,-4.37704086000345));
#55238=CARTESIAN_POINT('Ctrl Pts',(6.27227096822154,-19.5083641645074,-4.44772516209511));
#55239=CARTESIAN_POINT('Ctrl Pts',(6.27264565837955,-19.7477704004717,-4.52547486619641));
#55240=CARTESIAN_POINT('Ctrl Pts',(6.27297738924788,-19.9821807614481,-4.6096809486922));
#55241=CARTESIAN_POINT('Ctrl Pts',(6.27330912011622,-20.2165911224246,-4.69388703118799));
#55242=CARTESIAN_POINT('Ctrl Pts',(6.27359789171407,-20.4460057935968,-4.78454955708087));
#55243=CARTESIAN_POINT('Ctrl Pts',(6.27384369825113,-20.6701561128595,-4.88108731395748));
#55244=CARTESIAN_POINT('Ctrl Pts',(6.27395596446719,-20.7725313729845,-4.92517860949804));
#55245=CARTESIAN_POINT('Ctrl Pts',(6.27405926829797,-20.8738091877889,-4.97049584617027));
#55246=CARTESIAN_POINT('Ctrl Pts',(6.27415361636911,-20.9739673872759,-5.01698553344749));
#55247=CARTESIAN_POINT('Ctrl Pts',(6.27415652052491,-20.9770503863449,-5.01841654621858));
#55248=CARTESIAN_POINT('Ctrl Pts',(6.27415941613443,-20.9801323246383,-5.0198486698902));
#55249=CARTESIAN_POINT('Ctrl Pts',(6.27416230320351,-20.9832132015518,-5.02128190292619));
#55250=CARTESIAN_POINT('Ctrl Pts',(6.27420631261963,-21.0301769528704,-5.04312957869283));
#55251=CARTESIAN_POINT('Ctrl Pts',(6.27424833750549,-21.0768940659048,-5.06523502894291));
#55252=CARTESIAN_POINT('Ctrl Pts',(6.27428839847348,-21.1233628572361,-5.08759201950987));
#55253=CARTESIAN_POINT('Ctrl Pts',(6.27431785036691,-21.1575256335968,-5.10402835983542));
#55254=CARTESIAN_POINT('Ctrl Pts',(6.27434670151799,-21.1921531263297,-5.12089368240502));
#55255=CARTESIAN_POINT('Ctrl Pts',(6.27437398777163,-21.2260042193405,-5.13758066042605));
#55256=CARTESIAN_POINT('Ctrl Pts',(6.27438625154805,-21.2412185555358,-5.14508060418307));
#55257=CARTESIAN_POINT('Ctrl Pts',(6.27439819920825,-21.2562763691942,-5.15254387739071));
#55258=CARTESIAN_POINT('Ctrl Pts',(6.2744097432151,-21.2710665000488,-5.15991228247023));
#55259=CARTESIAN_POINT('Ctrl Pts',(6.27456064730716,-21.4644041598464,-5.25623260637502));
#55260=CARTESIAN_POINT('Ctrl Pts',(6.2746773653161,-21.6577057048019,-5.3590789236825));
#55261=CARTESIAN_POINT('Ctrl Pts',(6.27475989550217,-21.850472368102,-5.46870175362177));
#55262=CARTESIAN_POINT('Ctrl Pts',(6.27484107219999,-22.0400776740309,-5.57652677819603));
#55263=CARTESIAN_POINT('Ctrl Pts',(6.27488917324043,-22.2291655493083,-5.69090793688106));
#55264=CARTESIAN_POINT('Ctrl Pts',(6.27490419794014,-22.4172131850419,-5.8120683919335));
#55265=CARTESIAN_POINT('Ctrl Pts',(6.27490863190822,-22.4727082850861,-5.84782428723265));
#55266=CARTESIAN_POINT('Ctrl Pts',(6.27491018522934,-22.528112462999,-5.88417049254058));
#55267=CARTESIAN_POINT('Ctrl Pts',(6.27490885790158,-22.5834114504708,-5.92111247066758));
#55268=CARTESIAN_POINT('Ctrl Pts',(6.27490450920186,-22.7645865146092,-6.04214479987562));
#55269=CARTESIAN_POINT('Ctrl Pts',(6.2748692394911,-22.9446359710181,-6.16957378427421));
#55270=CARTESIAN_POINT('Ctrl Pts',(6.27480304923703,-23.1230252934947,-6.30354372742591));
#55271=CARTESIAN_POINT('Ctrl Pts',(6.27475277065118,-23.2585310864459,-6.40530824520284));
#55272=CARTESIAN_POINT('Ctrl Pts',(6.27468465083775,-23.3930780744229,-6.51084651979255));
#55273=CARTESIAN_POINT('Ctrl Pts',(6.27459869032304,-23.5264136418796,-6.62021342797622));
#55274=CARTESIAN_POINT('Ctrl Pts',(6.27448994615905,-23.6950895143096,-6.75856779961703));
#55275=CARTESIAN_POINT('Ctrl Pts',(6.27435264959262,-23.8618281643152,-6.90305003869651));
#55276=CARTESIAN_POINT('Ctrl Pts',(6.2741868031039,-24.0260801485733,-7.05375344142317));
#55277=CARTESIAN_POINT('Ctrl Pts',(6.27401315348193,-24.1980602440996,-7.21154749008647));
#55278=CARTESIAN_POINT('Ctrl Pts',(6.27380820415679,-24.3673135015332,-7.37616273233735));
#55279=CARTESIAN_POINT('Ctrl Pts',(6.27357195890655,-24.5332705410363,-7.54763129887915));
#55280=CARTESIAN_POINT('Ctrl Pts',(6.27333930669852,-24.6967035482112,-7.71649200855313));
#55281=CARTESIAN_POINT('Ctrl Pts',(6.27307630327827,-24.8569398563571,-7.8919992254237));
#55282=CARTESIAN_POINT('Ctrl Pts',(6.27278295324511,-25.0133970264588,-8.0741513007398));
#55283=CARTESIAN_POINT('Ctrl Pts',(6.27261682273637,-25.1020021272812,-8.17730798565161));
#55284=CARTESIAN_POINT('Ctrl Pts',(6.2724409594699,-25.1893944759236,-8.2825952175158));
#55285=CARTESIAN_POINT('Ctrl Pts',(6.27225536443483,-25.2754626136126,-8.39000786636834));
#55286=CARTESIAN_POINT('Ctrl Pts',(6.27204648913939,-25.3723267763896,-8.51089390598911));
#55287=CARTESIAN_POINT('Ctrl Pts',(6.27182528752588,-25.4675139092961,-8.63447218014262));
#55288=CARTESIAN_POINT('Ctrl Pts',(6.27159176118745,-25.5608443099078,-8.76072156011458));
#55289=CARTESIAN_POINT('Ctrl Pts',(-6.390310997303,-15.4600784053605,-3.94962015010527));
#55290=CARTESIAN_POINT('Ctrl Pts',(-4.260207331535,-16.2181814867602,-3.32898635579781));
#55291=CARTESIAN_POINT('Ctrl Pts',(0.0001535201438716,-16.9763032808813,
-2.70680215368588));
#55292=CARTESIAN_POINT('Ctrl Pts',(4.260514371823,-16.2181268476495,-3.32903119765556));
#55293=CARTESIAN_POINT('Ctrl Pts',(6.390771557735,-15.4599144861734,-3.94975434528492));
#55294=CARTESIAN_POINT('Ctrl Pts',(-6.390310997303,-16.2401890659177,-3.91822923290135));
#55295=CARTESIAN_POINT('Ctrl Pts',(-4.260207331535,-16.958959273677,-3.34433191874026));
#55296=CARTESIAN_POINT('Ctrl Pts',(0.0001535201438716,-17.677737083364,
-2.76848699945107));
#55297=CARTESIAN_POINT('Ctrl Pts',(4.260514371823,-16.9589074701588,-3.34437342085115));
#55298=CARTESIAN_POINT('Ctrl Pts',(6.390771557735,-16.2400336513955,-3.91835332258528));
#55299=CARTESIAN_POINT('Ctrl Pts',(-6.390310997303,-18.1257601336346,-4.02650683733696));
#55300=CARTESIAN_POINT('Ctrl Pts',(-4.260207331535,-18.7394139170257,-3.53811573879116));
#55301=CARTESIAN_POINT('Ctrl Pts',(0.0001535201438716,-19.3530458146751,
-3.05103811570896));
#55302=CARTESIAN_POINT('Ctrl Pts',(4.260514371823,-18.7393696915499,-3.53815084329452));
#55303=CARTESIAN_POINT('Ctrl Pts',(6.390771557735,-18.1256274476752,-4.02661243864776));
#55304=CARTESIAN_POINT('Ctrl Pts',(-6.390310997303,-21.0044951210519,-4.89945800150725));
#55305=CARTESIAN_POINT('Ctrl Pts',(-4.260207331535,-21.4424839510746,-4.44478850539219));
#55306=CARTESIAN_POINT('Ctrl Pts',(0.0001535201438716,-21.8807678511962,
-3.98943347064956));
#55307=CARTESIAN_POINT('Ctrl Pts',(4.260514371823,-21.4424523632204,-4.44482132359356));
#55308=CARTESIAN_POINT('Ctrl Pts',(6.390771557735,-21.0044004178749,-4.89955631142534));
#55309=CARTESIAN_POINT('Ctrl Pts',(-6.390310997303,-23.7052287527357,-6.63374442412537));
#55310=CARTESIAN_POINT('Ctrl Pts',(-4.260207331535,-23.9981322521798,-6.09525912369956));
#55311=CARTESIAN_POINT('Ctrl Pts',(0.0001535201438716,-24.2900551830466,
-5.55782158681654));
#55312=CARTESIAN_POINT('Ctrl Pts',(4.260514371823,-23.9981112128033,-6.09529785772377));
#55313=CARTESIAN_POINT('Ctrl Pts',(6.390771557735,-23.7051654203099,-6.63386085694714));
#55314=CARTESIAN_POINT('Ctrl Pts',(-6.390310997303,-25.1149831379802,-8.18394766638624));
#55315=CARTESIAN_POINT('Ctrl Pts',(-4.260207331535,-25.3660571924324,-7.53598855301376));
#55316=CARTESIAN_POINT('Ctrl Pts',(0.0001535201438716,-25.6190353418683,
-6.88615733883246));
#55317=CARTESIAN_POINT('Ctrl Pts',(4.260514371823,-25.366038959873,-7.53603538743866));
#55318=CARTESIAN_POINT('Ctrl Pts',(6.390771557735,-25.1149288500562,-8.18408776992176));
#55319=CARTESIAN_POINT('Ctrl Pts',(-6.390310997303,-25.6807362935916,-8.9842586986279));
#55320=CARTESIAN_POINT('Ctrl Pts',(-4.260207331535,-25.9287981973013,-8.27687157370651));
#55321=CARTESIAN_POINT('Ctrl Pts',(0.0001535201438716,-26.1774653804787,
-7.56887552599929));
#55322=CARTESIAN_POINT('Ctrl Pts',(4.260514371823,-25.9287802754393,-8.27692260016797));
#55323=CARTESIAN_POINT('Ctrl Pts',(6.390771557735,-25.680682656946,-8.98441165186304));
#55324=CARTESIAN_POINT('Ctrl Pts',(-6.26386107908002,-15.8144217366209,
-3.90573578027562));
#55325=CARTESIAN_POINT('Ctrl Pts',(-6.12401716319831,-15.8609391874445,
-3.86696795218159));
#55326=CARTESIAN_POINT('Ctrl Pts',(-5.98376053165562,-15.9057297542361,
-3.82937120018312));
#55327=CARTESIAN_POINT('Ctrl Pts',(-5.84314866563788,-15.9488113053792,
-3.79297601711986));
#55328=CARTESIAN_POINT('Ctrl Pts',(-5.52871437968464,-16.0451496668211,
-3.71158961835612));
#55329=CARTESIAN_POINT('Ctrl Pts',(-5.21250664998199,-16.1329423990905,
-3.63621373671984));
#55330=CARTESIAN_POINT('Ctrl Pts',(-4.89516718476226,-16.2124037512588,
-3.56716941662384));
#55331=CARTESIAN_POINT('Ctrl Pts',(-4.65229613832461,-16.273218316945,-3.51432737171561));
#55332=CARTESIAN_POINT('Ctrl Pts',(-4.40876127626954,-16.3291527723426,
-3.46519332271945));
#55333=CARTESIAN_POINT('Ctrl Pts',(-4.16483356053705,-16.3803011892008,
-3.4198993433696));
#55334=CARTESIAN_POINT('Ctrl Pts',(-3.84173002158442,-16.448051729352,-3.35990351642046));
#55335=CARTESIAN_POINT('Ctrl Pts',(-3.51793901645062,-16.507405349351,-3.30664570419035));
#55336=CARTESIAN_POINT('Ctrl Pts',(-3.19411251218769,-16.5586055111643,
-3.26031478599686));
#55337=CARTESIAN_POINT('Ctrl Pts',(-3.17358297433124,-16.5618514334293,
-3.25737755780072));
#55338=CARTESIAN_POINT('Ctrl Pts',(-3.15305327848952,-16.5650645834705,
-3.25446816200489));
#55339=CARTESIAN_POINT('Ctrl Pts',(-3.13252358460693,-16.5682450223921,
-3.25158664359035));
#55340=CARTESIAN_POINT('Ctrl Pts',(-2.82078843643712,-16.6165387088018,
-3.20783194490625));
#55341=CARTESIAN_POINT('Ctrl Pts',(-2.50902475984557,-16.6572953705827,
-3.17050248577678));
#55342=CARTESIAN_POINT('Ctrl Pts',(-2.19780052300139,-16.6907193045148,
-3.1397510112421));
#55343=CARTESIAN_POINT('Ctrl Pts',(-1.86506876129886,-16.726453039564,-3.10687441910832));
#55344=CARTESIAN_POINT('Ctrl Pts',(-1.53295439181552,-16.7538058312664,
-3.08151509558727));
#55345=CARTESIAN_POINT('Ctrl Pts',(-1.20216613281015,-16.7730740139961,
-3.06357945409478));
#55346=CARTESIAN_POINT('Ctrl Pts',(-0.869774260649804,-16.7924356060608,
-3.04555686323255));
#55347=CARTESIAN_POINT('Ctrl Pts',(-0.538721361552426,-16.8036339974548,
-3.03503012321186));
#55348=CARTESIAN_POINT('Ctrl Pts',(-0.209675401395077,-16.8069665914283,
-3.03189242033579));
#55349=CARTESIAN_POINT('Ctrl Pts',(-0.139707438544078,-16.8076752304622,
-3.03122522272557));
#55350=CARTESIAN_POINT('Ctrl Pts',(-0.0698300377265377,-16.8080282039476,
-3.03089207963549));
#55351=CARTESIAN_POINT('Ctrl Pts',(-4.93267029250509E-5,-16.8080283533074,
-3.03089189447942));
#55352=CARTESIAN_POINT('Ctrl Pts',(0.000256727375841293,-16.8080283539625,
-3.03089189366733));
#55353=CARTESIAN_POINT('Ctrl Pts',(0.000562783265965696,-16.8080283478307,
-3.03089189926015));
#55354=CARTESIAN_POINT('Ctrl Pts',(0.000868840966959984,-16.8080283349116,
-3.03089191125823));
#55355=CARTESIAN_POINT('Ctrl Pts',(0.330223347700769,-16.8080144324858,
-3.03090482262456));
#55356=CARTESIAN_POINT('Ctrl Pts',(0.661679104087344,-16.8001415993432,
-3.03833569807948));
#55357=CARTESIAN_POINT('Ctrl Pts',(0.994608533444343,-16.7841147967613,
-3.05329056982103));
#55358=CARTESIAN_POINT('Ctrl Pts',(1.32345073774953,-16.7682847480354,-3.06806184731997));
#55359=CARTESIAN_POINT('Ctrl Pts',(1.65373070732275,-16.7444997130104,-3.09017351227283));
#55360=CARTESIAN_POINT('Ctrl Pts',(1.98479404869071,-16.7124651864611,-3.11972239231826));
#55361=CARTESIAN_POINT('Ctrl Pts',(2.05630999150204,-16.7055451228889,-3.12610550923702));
#55362=CARTESIAN_POINT('Ctrl Pts',(2.12786230171351,-16.6982400651354,-3.13283565777945));
#55363=CARTESIAN_POINT('Ctrl Pts',(2.1994440690604,-16.6905469802818,-3.13991378115135));
#55364=CARTESIAN_POINT('Ctrl Pts',(2.50988585026661,-16.657182968,-3.17061077716883));
#55365=CARTESIAN_POINT('Ctrl Pts',(2.82088461213451,-16.6165211571424,-3.20785426138439));
#55366=CARTESIAN_POINT('Ctrl Pts',(3.1319039030523,-16.5683497168773,-3.25150005214996));
#55367=CARTESIAN_POINT('Ctrl Pts',(3.45498851193197,-16.5183095701993,-3.29683898658431));
#55368=CARTESIAN_POINT('Ctrl Pts',(3.77809569404769,-16.4601659132149,-3.34908678857731));
#55369=CARTESIAN_POINT('Ctrl Pts',(4.10058014142998,-16.3936746989229,-3.40805934070719));
#55370=CARTESIAN_POINT('Ctrl Pts',(4.12247803430224,-16.3891596982792,-3.41206379623807));
#55371=CARTESIAN_POINT('Ctrl Pts',(4.14437303812036,-16.3846062051229,-3.41609925003709));
#55372=CARTESIAN_POINT('Ctrl Pts',(4.16626494305972,-16.3800141418853,-3.42016564051079));
#55373=CARTESIAN_POINT('Ctrl Pts',(4.48426643316004,-16.3133098986396,-3.47923396889741));
#55374=CARTESIAN_POINT('Ctrl Pts',(4.80161746509365,-16.2384676068073,-3.54483250854387));
#55375=CARTESIAN_POINT('Ctrl Pts',(5.11771182738074,-16.1552757166658,-3.61666694204498));
#55376=CARTESIAN_POINT('Ctrl Pts',(5.36077908835196,-16.0913036017398,-3.67190550709942));
#55377=CARTESIAN_POINT('Ctrl Pts',(5.60310246923606,-16.0223941423869,-3.73083088379307));
#55378=CARTESIAN_POINT('Ctrl Pts',(5.84438925839552,-15.9484491529106,-3.79329715013008));
#55379=CARTESIAN_POINT('Ctrl Pts',(5.98458157661485,-15.9054856755834,-3.82959126601931));
#55380=CARTESIAN_POINT('Ctrl Pts',(6.12442366940432,-15.8608222503357,-3.86708052801428));
#55381=CARTESIAN_POINT('Ctrl Pts',(6.26385845645402,-15.8144409512224,-3.90573485384998));
#55382=CARTESIAN_POINT('Ctrl Pts',(-6.3837685640945,-15.7767343726346,-3.93925153079634));
#55383=CARTESIAN_POINT('Ctrl Pts',(-6.20607782972262,-15.8406682009394,
-3.88901212835295));
#55384=CARTESIAN_POINT('Ctrl Pts',(-5.4836198762884,-16.0875649593149,-3.69326716669371));
#55385=CARTESIAN_POINT('Ctrl Pts',(-4.1035174816222,-16.4626408119468,-3.38487949324654));
#55386=CARTESIAN_POINT('Ctrl Pts',(-2.14467957257126,-16.7896566974073,
-3.10376395696803));
#55387=CARTESIAN_POINT('Ctrl Pts',(0.000847861998201127,-16.9109161991796,
-2.996367192768));
#55388=CARTESIAN_POINT('Ctrl Pts',(2.14629737698611,-16.7894735254493,-3.10392477724487));
#55389=CARTESIAN_POINT('Ctrl Pts',(4.10495670713201,-16.4623223834777,-3.38514788225707));
#55390=CARTESIAN_POINT('Ctrl Pts',(5.48449760235313,-16.0872874995829,-3.6934902959204));
#55391=CARTESIAN_POINT('Ctrl Pts',(6.20649253218868,-15.8405191837971,-3.88912925735201));
#55392=CARTESIAN_POINT('Ctrl Pts',(6.38378443801723,-15.7767286639177,-3.93925601899087));
#55393=CARTESIAN_POINT('Ctrl Pts',(-6.17892139218255,-15.1602625279266,
-3.89269138696012));
#55394=CARTESIAN_POINT('Ctrl Pts',(-6.00683890361596,-15.2221601613956,
-3.84473793976352));
#55395=CARTESIAN_POINT('Ctrl Pts',(-5.30721149445514,-15.461200315072,-3.65787934807116));
#55396=CARTESIAN_POINT('Ctrl Pts',(-3.97097810938147,-15.8243579582481,
-3.36339135340124));
#55397=CARTESIAN_POINT('Ctrl Pts',(-2.07510068658041,-16.1409487021963,
-3.09490132827578));
#55398=CARTESIAN_POINT('Ctrl Pts',(0.000820296697672055,-16.2583236281581,
-2.9923308284817));
#55399=CARTESIAN_POINT('Ctrl Pts',(2.07666620641412,-16.1407713880041,-3.09505492534853));
#55400=CARTESIAN_POINT('Ctrl Pts',(3.9723713467328,-15.8240496584546,-3.36364767993662));
#55401=CARTESIAN_POINT('Ctrl Pts',(5.30806143406014,-15.4609316732643,-3.6580923832534));
#55402=CARTESIAN_POINT('Ctrl Pts',(6.00724051639534,-15.2220158906671,-3.84484973879705));
#55403=CARTESIAN_POINT('Ctrl Pts',(6.17893676471506,-15.1602570013782,-3.89269567046585));
#55404=CARTESIAN_POINT('Ctrl Pts',(-6.17564082336744,-14.7487479575801,
-3.38940352206825));
#55405=CARTESIAN_POINT('Ctrl Pts',(-6.00404507762524,-14.809901241264,-3.34205562192575));
#55406=CARTESIAN_POINT('Ctrl Pts',(-5.30627654165239,-15.0461285322073,
-3.15749986835487));
#55407=CARTESIAN_POINT('Ctrl Pts',(-3.97251250102238,-15.4054450914358,
-2.86622749566697));
#55408=CARTESIAN_POINT('Ctrl Pts',(-2.07720323431513,-15.7192792537822,
-2.600083132903));
#55409=CARTESIAN_POINT('Ctrl Pts',(0.000821374932474116,-15.8358083161971,
-2.49822962199973));
#55410=CARTESIAN_POINT('Ctrl Pts',(2.07876949073072,-15.7191033001096,-2.60023557233471));
#55411=CARTESIAN_POINT('Ctrl Pts',(3.97390417607718,-15.4051397524895,-2.86648131292695));
#55412=CARTESIAN_POINT('Ctrl Pts',(5.30712443090202,-15.0458629393537,-3.15771038243398));
#55413=CARTESIAN_POINT('Ctrl Pts',(6.00444555828538,-14.8097587041699,-3.34216601186277));
#55414=CARTESIAN_POINT('Ctrl Pts',(6.17565615402447,-14.7487424970808,-3.38940775256534));
#55415=CARTESIAN_POINT('Ctrl Pts',(-6.37449173036292,-14.8207095476402,
-2.77587757352679));
#55416=CARTESIAN_POINT('Ctrl Pts',(-6.19797218928426,-14.8829064861205,
-2.72705638613095));
#55417=CARTESIAN_POINT('Ctrl Pts',(-5.47999872535319,-15.1232382790275,
-2.53670636090267));
#55418=CARTESIAN_POINT('Ctrl Pts',(-4.10596568664865,-15.489339540839,-2.23586437891013));
#55419=CARTESIAN_POINT('Ctrl Pts',(-2.14896198146769,-15.8098992465146,
-1.96027369700207));
#55420=CARTESIAN_POINT('Ctrl Pts',(0.000850125320108021,-15.9291719775344,
-1.85457369962847));
#55421=CARTESIAN_POINT('Ctrl Pts',(2.15058105504337,-15.809719266933,-1.96043178241714));
#55422=CARTESIAN_POINT('Ctrl Pts',(4.10740092124632,-15.4890280381271,-2.23612686966137));
#55423=CARTESIAN_POINT('Ctrl Pts',(5.48087148341781,-15.1229679377722,-2.53692358082765));
#55424=CARTESIAN_POINT('Ctrl Pts',(6.19838416728458,-14.8827615143263,-2.72717021488259));
#55425=CARTESIAN_POINT('Ctrl Pts',(6.37450750336995,-14.8207039930432,-2.77588193753119));
#55426=CARTESIAN_POINT('Ctrl Pts',(-6.24994605269825,-14.8593868267772,
-2.76546777148552));
#55427=CARTESIAN_POINT('Ctrl Pts',(-6.11224128919459,-14.9068450911447,
-2.72809069871833));
#55428=CARTESIAN_POINT('Ctrl Pts',(-5.97365547012716,-14.9527218912298,
-2.69169109149479));
#55429=CARTESIAN_POINT('Ctrl Pts',(-5.83421266230798,-14.9970062068934,
-2.65632554963629));
#55430=CARTESIAN_POINT('Ctrl Pts',(-5.52516534036188,-15.0951536077819,
-2.57794484164944));
#55431=CARTESIAN_POINT('Ctrl Pts',(-5.21190774264299,-15.1854811987466,
-2.50464131142876));
#55432=CARTESIAN_POINT('Ctrl Pts',(-4.89477543421764,-15.2678455319869,
-2.43707517713196));
#55433=CARTESIAN_POINT('Ctrl Pts',(-4.66466389456281,-15.3276091796224,
-2.38804911835932));
#55434=CARTESIAN_POINT('Ctrl Pts',(-4.43251153326942,-15.3831813833709,
-2.34203415873297));
#55435=CARTESIAN_POINT('Ctrl Pts',(-4.1984578515508,-15.4345020292727,-2.2992338678819));
#55436=CARTESIAN_POINT('Ctrl Pts',(-4.18854879210617,-15.4366747758291,
-2.29742184500246));
#55437=CARTESIAN_POINT('Ctrl Pts',(-4.1786363290934,-15.4388399004789,-2.29561557911493));
#55438=CARTESIAN_POINT('Ctrl Pts',(-4.16872047032422,-15.4409973987708,
-2.29381508614649));
#55439=CARTESIAN_POINT('Ctrl Pts',(-4.06152918762868,-15.4643201401194,
-2.274351602926));
#55440=CARTESIAN_POINT('Ctrl Pts',(-3.95394109213383,-15.4867517351017,
-2.25556268317071));
#55441=CARTESIAN_POINT('Ctrl Pts',(-3.84597072661888,-15.5082870367113,
-2.23746575262707));
#55442=CARTESIAN_POINT('Ctrl Pts',(-3.78699157947931,-15.5200507620286,
-2.22758024817205));
#55443=CARTESIAN_POINT('Ctrl Pts',(-3.72789835363644,-15.5315470317432,
-2.2179012300442));
#55444=CARTESIAN_POINT('Ctrl Pts',(-3.66869348220133,-15.5427749527341,
-2.20843132159147));
#55445=CARTESIAN_POINT('Ctrl Pts',(-3.63909104648377,-15.5483889132295,
-2.2036963673651));
#55446=CARTESIAN_POINT('Ctrl Pts',(-3.60946069920004,-15.5539357857702,
-2.19901369043729));
#55447=CARTESIAN_POINT('Ctrl Pts',(-3.57980274610709,-15.5594154544918,
-2.19438361195204));
#55448=CARTESIAN_POINT('Ctrl Pts',(-3.56497376956061,-15.5621552888526,
-2.19206857270941));
#55449=CARTESIAN_POINT('Ctrl Pts',(-3.55013789155253,-15.5648783222099,
-2.18976668307023));
#55450=CARTESIAN_POINT('Ctrl Pts',(-3.53529515056274,-15.5675845398395,
-2.18747798241135));
#55451=CARTESIAN_POINT('Ctrl Pts',(-3.52787378006785,-15.5689376486542,
-2.18633363208192));
#55452=CARTESIAN_POINT('Ctrl Pts',(-3.52045069382698,-15.5702865535341,
-2.18519257899711));
#55453=CARTESIAN_POINT('Ctrl Pts',(-3.5130258966674,-15.5716312526235,-2.18405482802872));
#55454=CARTESIAN_POINT('Ctrl Pts',(-3.50560109950782,-15.572975951713,-2.18291707706032));
#55455=CARTESIAN_POINT('Ctrl Pts',(-3.49969582841781,-15.5740427847343,
-2.18201427674118));
#55456=CARTESIAN_POINT('Ctrl Pts',(-3.49074637726386,-15.5756527306545,
-2.1806514863284));
#55457=CARTESIAN_POINT('Ctrl Pts',(-3.18937218028059,-15.6298679166515,
-2.13475930151785));
#55458=CARTESIAN_POINT('Ctrl Pts',(-2.8863104354888,-15.6769573631538,-2.09449088189289));
#55459=CARTESIAN_POINT('Ctrl Pts',(-2.58189061930374,-15.7169297571031,
-2.06012185686861));
#55460=CARTESIAN_POINT('Ctrl Pts',(-2.45625178067274,-15.733426991797,-2.04593722052317));
#55461=CARTESIAN_POINT('Ctrl Pts',(-2.33038134326096,-15.7487114909266,
-2.03275775631289));
#55462=CARTESIAN_POINT('Ctrl Pts',(-2.20430144629838,-15.7627819152971,
-2.02060420803763));
#55463=CARTESIAN_POINT('Ctrl Pts',(-1.90245288183243,-15.7964679945211,
-1.99150733225939));
#55464=CARTESIAN_POINT('Ctrl Pts',(-1.59940460449395,-15.8231979990122,
-1.96828846747673));
#55465=CARTESIAN_POINT('Ctrl Pts',(-1.29555337158924,-15.842976677377,-1.95105143023668));
#55466=CARTESIAN_POINT('Ctrl Pts',(-0.993107503021079,-15.8626638759445,
-1.93389411726555));
#55467=CARTESIAN_POINT('Ctrl Pts',(-0.689865522197483,-15.875463913011,
-1.92266330219558));
#55468=CARTESIAN_POINT('Ctrl Pts',(-0.386210791332723,-15.881342888697,
-1.91749439950967));
#55469=CARTESIAN_POINT('Ctrl Pts',(-0.257555172826256,-15.883833754724,
-1.91530438465247));
#55470=CARTESIAN_POINT('Ctrl Pts',(-0.128825412042817,-15.8850817198573,
-1.91420298318698));
#55471=CARTESIAN_POINT('Ctrl Pts',(-5.06157679712277E-5,-15.8850820917059,
-1.91420238091613));
#55472=CARTESIAN_POINT('Ctrl Pts',(0.000256975117818086,-15.8850820925941,
-1.91420237947755));
#55473=CARTESIAN_POINT('Ctrl Pts',(0.000564565725845489,-15.885082086369,
-1.91420238427594));
#55474=CARTESIAN_POINT('Ctrl Pts',(0.000872156055743548,-15.8850820730305,
-1.91420239531148));
#55475=CARTESIAN_POINT('Ctrl Pts',(0.297675497334216,-15.8850692023486,
-1.91421304384406));
#55476=CARTESIAN_POINT('Ctrl Pts',(0.594220548053702,-15.8784364142884,
-1.9200281299929));
#55477=CARTESIAN_POINT('Ctrl Pts',(0.890169967705006,-15.8652261227378,
-1.93155600891819));
#55478=CARTESIAN_POINT('Ctrl Pts',(1.17953867129292,-15.8523095745503,-1.94282755452101));
#55479=CARTESIAN_POINT('Ctrl Pts',(1.46833837285049,-15.8331045734909,-1.95956096628514));
#55480=CARTESIAN_POINT('Ctrl Pts',(1.75624190641963,-15.8076155284317,-1.9817012282312));
#55481=CARTESIAN_POINT('Ctrl Pts',(1.90640216753209,-15.7943213475158,-1.99324880277364));
#55482=CARTESIAN_POINT('Ctrl Pts',(2.05632258772584,-15.7793184671638,-2.00625435834685));
#55483=CARTESIAN_POINT('Ctrl Pts',(2.20595339365679,-15.762605219908,-2.02070306900956));
#55484=CARTESIAN_POINT('Ctrl Pts',(2.34662518566424,-15.7468926637462,-2.03428667573061));
#55485=CARTESIAN_POINT('Ctrl Pts',(2.48704100784772,-15.7296684005041,-2.04914582503358));
#55486=CARTESIAN_POINT('Ctrl Pts',(2.62716943519071,-15.7109343642876,-2.06524908302113));
#55487=CARTESIAN_POINT('Ctrl Pts',(2.77176006676714,-15.6916037674924,-2.08186512793797));
#55488=CARTESIAN_POINT('Ctrl Pts',(2.91604212779795,-15.6706654399321,-2.09981011040458));
#55489=CARTESIAN_POINT('Ctrl Pts',(3.05997654759935,-15.6481199360848,-2.11905354500426));
#55490=CARTESIAN_POINT('Ctrl Pts',(3.13194375750006,-15.6368471841611,-2.12867526230409));
#55491=CARTESIAN_POINT('Ctrl Pts',(3.20382405485216,-15.6251726137908,-2.13862158957259));
#55492=CARTESIAN_POINT('Ctrl Pts',(3.27561263489304,-15.613096202853,-2.14888818338128));
#55493=CARTESIAN_POINT('Ctrl Pts',(3.31150692491348,-15.6070579973841,-2.15402148028563));
#55494=CARTESIAN_POINT('Ctrl Pts',(3.34737828542149,-15.6009193302214,-2.15923484362356));
#55495=CARTESIAN_POINT('Ctrl Pts',(3.38322611752088,-15.5946801907778,-2.16452771501257));
#55496=CARTESIAN_POINT('Ctrl Pts',(3.40115003357058,-15.591560621056,-2.16717415070707));
#55497=CARTESIAN_POINT('Ctrl Pts',(3.41906806750332,-15.5884159331665,-2.16984046340098));
#55498=CARTESIAN_POINT('Ctrl Pts',(3.43698014470371,-15.5852461253899,-2.17252658147989));
#55499=CARTESIAN_POINT('Ctrl Pts',(3.44593618330391,-15.5836612215015,-2.17386964051935));
#55500=CARTESIAN_POINT('Ctrl Pts',(3.45489073272004,-15.5820700376354,-2.17521765090421));
#55501=CARTESIAN_POINT('Ctrl Pts',(3.46384378364179,-15.5804725735521,-2.17657060356384));
#55502=CARTESIAN_POINT('Ctrl Pts',(3.47279683456355,-15.5788751094689,-2.17792355622348));
#55503=CARTESIAN_POINT('Ctrl Pts',(3.48327010629409,-15.5769976228693,-2.1795131641832));
#55504=CARTESIAN_POINT('Ctrl Pts',(3.49069843161647,-15.5756613403914,-2.18064427925889));
#55505=CARTESIAN_POINT('Ctrl Pts',(3.71882625272019,-15.5346233948462,-2.21538142477097));
#55506=CARTESIAN_POINT('Ctrl Pts',(3.94535648705172,-15.4896112321074,-2.25326998516031));
#55507=CARTESIAN_POINT('Ctrl Pts',(4.17013179886758,-15.4406820257936,-2.29412672109735));
#55508=CARTESIAN_POINT('Ctrl Pts',(4.49398044986303,-15.3701864836853,-2.35299172148549));
#55509=CARTESIAN_POINT('Ctrl Pts',(4.8141865358934,-15.2915616281918,-2.41801658538009));
#55510=CARTESIAN_POINT('Ctrl Pts',(5.13041264068862,-15.2049672772219,-2.48860252594909));
#55511=CARTESIAN_POINT('Ctrl Pts',(5.36770661560993,-15.1399874497005,-2.54156974831684));
#55512=CARTESIAN_POINT('Ctrl Pts',(5.60275959993477,-15.0705192344865,-2.5976691992491));
#55513=CARTESIAN_POINT('Ctrl Pts',(5.8354275471442,-14.9966156188503,-2.65666031041631));
#55514=CARTESIAN_POINT('Ctrl Pts',(5.97445995846876,-14.9524539798677,-2.69191087471044));
#55515=CARTESIAN_POINT('Ctrl Pts',(6.11264069900418,-14.9067083356646,-2.72819417249631));
#55516=CARTESIAN_POINT('Ctrl Pts',(6.24994470386048,-14.8593882189047,-2.76546244225239));
#55517=CARTESIAN_POINT('Ctrl Pts',(7.10495696060184,-15.2147787467643,5.08680107463094));
#55518=CARTESIAN_POINT('Ctrl Pts',(7.10596084475798,-15.2419087055295,5.00460205443588));
#55519=CARTESIAN_POINT('Ctrl Pts',(7.09052318662475,-15.3082820625518,4.81707696377181));
#55520=CARTESIAN_POINT('Ctrl Pts',(7.0043168782856,-15.4227062459899,4.53822716637853));
#55521=CARTESIAN_POINT('Ctrl Pts',(6.84418516995453,-15.5500445504962,4.27661325180109));
#55522=CARTESIAN_POINT('Ctrl Pts',(6.63017629479599,-15.673047448177,4.07076452833132));
#55523=CARTESIAN_POINT('Ctrl Pts',(6.42344282838547,-15.7648481127942,3.95589962337636));
#55524=CARTESIAN_POINT('Ctrl Pts',(6.29350100205884,-15.8132040931925,3.9133231394474));
#55525=CARTESIAN_POINT('Ctrl Pts',(6.25215637714488,-15.8277458920358,3.90246971967927));
#55526=CARTESIAN_POINT('Ctrl Pts',(6.81722694411318,-14.6678650098582,4.90248406328812));
#55527=CARTESIAN_POINT('Ctrl Pts',(6.81812715945108,-14.691775308277,4.83000073281271));
#55528=CARTESIAN_POINT('Ctrl Pts',(6.80424853975033,-14.7506252433578,4.66430263806235));
#55529=CARTESIAN_POINT('Ctrl Pts',(6.72648871389155,-14.8529185526735,4.41778502112603));
#55530=CARTESIAN_POINT('Ctrl Pts',(6.58227945968176,-14.9671735461734,4.18722534021326));
#55531=CARTESIAN_POINT('Ctrl Pts',(6.39031761580399,-15.0775057042662,4.00683702016848));
#55532=CARTESIAN_POINT('Ctrl Pts',(6.20591548437909,-15.159553132176,3.90697891677903));
#55533=CARTESIAN_POINT('Ctrl Pts',(6.09061389420951,-15.2025631711381,3.87022200760893));
#55534=CARTESIAN_POINT('Ctrl Pts',(6.05399099367591,-15.2154743878466,3.86087547311471));
#55535=CARTESIAN_POINT('Ctrl Pts',(7.05919742644666,-14.099365919639,4.71767508414311));
#55536=CARTESIAN_POINT('Ctrl Pts',(7.06038809058804,-14.1302863226927,4.62399558055472));
#55537=CARTESIAN_POINT('Ctrl Pts',(7.04218600841309,-14.205534883539,4.41132787330049));
#55538=CARTESIAN_POINT('Ctrl Pts',(6.94133832169349,-14.3347911618672,4.09585993930461));
#55539=CARTESIAN_POINT('Ctrl Pts',(6.75329582486237,-14.4793527715302,3.79837680263864));
#55540=CARTESIAN_POINT('Ctrl Pts',(6.49963210608973,-14.6206396718045,3.56192024772834));
#55541=CARTESIAN_POINT('Ctrl Pts',(6.25142152215052,-14.7279766140739,3.42816698756074));
#55542=CARTESIAN_POINT('Ctrl Pts',(6.09355729230462,-14.7855072753609,3.37811577971091));
#55543=CARTESIAN_POINT('Ctrl Pts',(6.04313356608242,-14.8029143472445,3.36532862725582));
#55544=CARTESIAN_POINT('Ctrl Pts',(7.66738224158263,-13.8935052574552,4.65727912036421));
#55545=CARTESIAN_POINT('Ctrl Pts',(7.66906120809273,-13.9369286846848,4.52581419290841));
#55546=CARTESIAN_POINT('Ctrl Pts',(7.64357464066956,-14.0414170913453,4.22911839576172));
#55547=CARTESIAN_POINT('Ctrl Pts',(7.50370581709582,-14.2185108259714,3.79000846918474));
#55548=CARTESIAN_POINT('Ctrl Pts',(7.24169365276974,-14.416290207258,3.37284545922798));
#55549=CARTESIAN_POINT('Ctrl Pts',(6.88427276433928,-14.6112405403477,3.03667830773213));
#55550=CARTESIAN_POINT('Ctrl Pts',(6.52923106880879,-14.7618210155054,2.84303151425121));
#55551=CARTESIAN_POINT('Ctrl Pts',(6.30036209622375,-14.8439269044745,2.76955534331772));
#55552=CARTESIAN_POINT('Ctrl Pts',(6.22694060282119,-14.8689183013122,2.75070496021726));
#55553=CARTESIAN_POINT('',(6.2638598901157,-15.8144313886664,3.90573722905719));
#55554=CARTESIAN_POINT('',(6.24994591741779,-14.8593874699437,2.76546569721984));
#55555=CARTESIAN_POINT('Ctrl Pts',(6.26385676107766,-15.8144315143033,3.90574866939898));
#55556=CARTESIAN_POINT('Ctrl Pts',(6.25434379880635,-15.7850266167952,3.90346982270102));
#55557=CARTESIAN_POINT('Ctrl Pts',(6.24500788984914,-15.7549953789465,3.89975105195181));
#55558=CARTESIAN_POINT('Ctrl Pts',(6.23595188136702,-15.7245103682235,3.8944427648052));
#55559=CARTESIAN_POINT('Ctrl Pts',(6.22712248221697,-15.6947881867238,3.88926730741544));
#55560=CARTESIAN_POINT('Ctrl Pts',(6.2185594413941,-15.664634965679,3.88258020830732));
#55561=CARTESIAN_POINT('Ctrl Pts',(6.21036401048873,-15.6342507943812,3.87427078583523));
#55562=CARTESIAN_POINT('Ctrl Pts',(6.20229493636841,-15.6043350848697,3.86608947766504));
#55563=CARTESIAN_POINT('Ctrl Pts',(6.19458254627921,-15.5741959424333,3.85633486755289));
#55564=CARTESIAN_POINT('Ctrl Pts',(6.18732480245288,-15.5440582729263,3.84493840162574));
#55565=CARTESIAN_POINT('Ctrl Pts',(6.18019462696393,-15.5144503289763,3.83374224976934));
#55566=CARTESIAN_POINT('Ctrl Pts',(6.17350358986061,-15.4848444425667,3.82096101904608));
#55567=CARTESIAN_POINT('Ctrl Pts',(6.16734101033035,-15.4554788128665,3.80657352922948));
#55568=CARTESIAN_POINT('Ctrl Pts',(6.16654374976043,-15.4516797448697,3.80471220179757));
#55569=CARTESIAN_POINT('Ctrl Pts',(6.16575532487597,-15.4478847246442,3.80282405647154));
#55570=CARTESIAN_POINT('Ctrl Pts',(6.16497592004,-15.4440942898146,3.80090910734589));
#55571=CARTESIAN_POINT('Ctrl Pts',(6.15904357729299,-15.4152438676313,3.78633371079701));
#55572=CARTESIAN_POINT('Ctrl Pts',(6.15363479800696,-15.3866584553602,3.77020145346772));
#55573=CARTESIAN_POINT('Ctrl Pts',(6.14882417024651,-15.3585810547484,3.75254629327471));
#55574=CARTESIAN_POINT('Ctrl Pts',(6.14407517199114,-15.3308633569425,3.73511731536792));
#55575=CARTESIAN_POINT('Ctrl Pts',(6.13990937017329,-15.3036415436826,3.71620422607133));
#55576=CARTESIAN_POINT('Ctrl Pts',(6.13638525666128,-15.2771503252054,3.69588866707889));
#55577=CARTESIAN_POINT('Ctrl Pts',(6.13288183768904,-15.2508146702685,3.67569240649792));
#55578=CARTESIAN_POINT('Ctrl Pts',(6.13001281258441,-15.2252018603058,3.65411031081203));
#55579=CARTESIAN_POINT('Ctrl Pts',(6.12781875017019,-15.2005313792643,3.6312696488277));
#55580=CARTESIAN_POINT('Ctrl Pts',(6.12563213271504,-15.1759446108464,3.60850649046963));
#55581=CARTESIAN_POINT('Ctrl Pts',(6.1241160438716,-15.1522945325966,3.5844937213183));
#55582=CARTESIAN_POINT('Ctrl Pts',(6.1232911028458,-15.1297756714056,3.55939941650749));
#55583=CARTESIAN_POINT('Ctrl Pts',(6.1224669045622,-15.1072770852501,3.53432770555339));
#55584=CARTESIAN_POINT('Ctrl Pts',(6.12233265472249,-15.0859083031204,3.50817702111357));
#55585=CARTESIAN_POINT('Ctrl Pts',(6.12288798583855,-15.0658302715291,3.48114923737607));
#55586=CARTESIAN_POINT('Ctrl Pts',(6.12344602286289,-15.0456544076528,3.45398975796753));
#55587=CARTESIAN_POINT('Ctrl Pts',(6.1247003340058,-15.0267823796104,3.42594536020585));
#55588=CARTESIAN_POINT('Ctrl Pts',(6.12662935671012,-15.009335720049,3.39724519948053));
#55589=CARTESIAN_POINT('Ctrl Pts',(6.12856584253839,-14.9918215617575,3.36843400177455));
#55590=CARTESIAN_POINT('Ctrl Pts',(6.13118211919576,-14.9757440612021,3.33896280103151));
#55591=CARTESIAN_POINT('Ctrl Pts',(6.13443655377272,-14.9611787464408,3.30907576756275));
#55592=CARTESIAN_POINT('Ctrl Pts',(6.13772838224608,-14.9464460742299,3.27884532801018));
#55593=CARTESIAN_POINT('Ctrl Pts',(6.14167289476094,-14.9332605876828,3.2481903112989));
#55594=CARTESIAN_POINT('Ctrl Pts',(6.14620958715487,-14.9216497189146,3.21736297478641));
#55595=CARTESIAN_POINT('Ctrl Pts',(6.14951384885931,-14.9131930404153,3.1949101438155));
#55596=CARTESIAN_POINT('Ctrl Pts',(6.15313186295512,-14.9055705611463,3.17236592052286));
#55597=CARTESIAN_POINT('Ctrl Pts',(6.15703571528297,-14.8987765659417,3.14982379446668));
#55598=CARTESIAN_POINT('Ctrl Pts',(6.16249126701368,-14.8892821001721,3.11832164620606));
#55599=CARTESIAN_POINT('Ctrl Pts',(6.16850504640394,-14.8814072953678,3.0868249131614));
#55600=CARTESIAN_POINT('Ctrl Pts',(6.17499163073684,-14.8750962878681,3.05556885520286));
#55601=CARTESIAN_POINT('Ctrl Pts',(6.18162661140325,-14.8686409007804,3.02359773918563));
#55602=CARTESIAN_POINT('Ctrl Pts',(6.18875592528047,-14.8638211729704,2.99187907491926));
#55603=CARTESIAN_POINT('Ctrl Pts',(6.19628251443661,-14.8605346123414,2.96063113067753));
#55604=CARTESIAN_POINT('Ctrl Pts',(6.20392059387846,-14.8571993683613,2.92892031511933));
#55605=CARTESIAN_POINT('Ctrl Pts',(6.21196745122266,-14.855442332926,2.8976946499334));
#55606=CARTESIAN_POINT('Ctrl Pts',(6.2203213744668,-14.8551224309158,2.86714030820995));
#55607=CARTESIAN_POINT('Ctrl Pts',(6.22887565822237,-14.8547948563751,2.83585315109482));
#55608=CARTESIAN_POINT('Ctrl Pts',(6.23775158600005,-14.8559734060631,2.80527012090917));
#55609=CARTESIAN_POINT('Ctrl Pts',(6.24684494550031,-14.8584827088845,2.77554272822559));
#55610=CARTESIAN_POINT('Ctrl Pts',(6.24787581205197,-14.8587671754061,2.7721726893764));
#55611=CARTESIAN_POINT('Ctrl Pts',(6.24890948106048,-14.8590687268172,2.76881359532572));
#55612=CARTESIAN_POINT('Ctrl Pts',(6.24994580734849,-14.8593870957008,2.76546562756306));
#55613=CARTESIAN_POINT('',(7.000000212767,-14.5427408801051,3.16613451323743));
#55614=CARTESIAN_POINT('Ctrl Pts',(7.00000061650467,-14.5427408381467,3.16613402467205));
#55615=CARTESIAN_POINT('Ctrl Pts',(6.9274660400329,-14.5808036624884,3.10292449647818));
#55616=CARTESIAN_POINT('Ctrl Pts',(6.77485267168808,-14.6548676519438,2.98919830046988));
#55617=CARTESIAN_POINT('Ctrl Pts',(6.523266472515,-14.7608743894712,2.85474660862042));
#55618=CARTESIAN_POINT('Ctrl Pts',(6.343316019062,-14.8272098476568,2.79080490252102));
#55619=CARTESIAN_POINT('Ctrl Pts',(6.249945936522,-14.8593875349017,2.76546570931229));
#55620=CARTESIAN_POINT('',(7.,-14.7967973072037,4.92969292433389));
#55621=CARTESIAN_POINT('Ctrl Pts',(7.,-14.7967973072037,4.92969292433389));
#55622=CARTESIAN_POINT('Ctrl Pts',(7.,-14.7447744258633,4.79864067714473));
#55623=CARTESIAN_POINT('Ctrl Pts',(7.,-14.7000166221108,4.67450080516981));
#55624=CARTESIAN_POINT('Ctrl Pts',(7.,-14.6625238959461,4.55727330840913));
#55625=CARTESIAN_POINT('Ctrl Pts',(7.,-14.6500263205578,4.51819747615557));
#55626=CARTESIAN_POINT('Ctrl Pts',(7.,-14.6389585887663,4.48203729950645));
#55627=CARTESIAN_POINT('Ctrl Pts',(7.,-14.6274528623107,4.44234993671987));
#55628=CARTESIAN_POINT('Ctrl Pts',(7.,-14.5814299564882,4.28360048557353));
#55629=CARTESIAN_POINT('Ctrl Pts',(7.,-14.5472852583712,4.12817676488021));
#55630=CARTESIAN_POINT('Ctrl Pts',(7.,-14.5257751444716,3.98124543293447));
#55631=CARTESIAN_POINT('Ctrl Pts',(7.,-14.4827549166725,3.687382769043));
#55632=CARTESIAN_POINT('Ctrl Pts',(7.,-14.4884099871871,3.41567923317487));
#55633=CARTESIAN_POINT('Ctrl Pts',(7.,-14.5427403560153,3.1661348253301));
#55634=CARTESIAN_POINT('Ctrl Pts',(6.99999343558281,-14.7967973069948,4.92969292493306));
#55635=CARTESIAN_POINT('Ctrl Pts',(6.99998714159524,-14.8239179309797,4.89270461052958));
#55636=CARTESIAN_POINT('Ctrl Pts',(6.9982547064127,-14.850757358501,4.85673485006274));
#55637=CARTESIAN_POINT('Ctrl Pts',(6.99505575114715,-14.8771900729887,4.82190106750212));
#55638=CARTESIAN_POINT('Ctrl Pts',(6.99209903435036,-14.9016211901575,4.78970504678811));
#55639=CARTESIAN_POINT('Ctrl Pts',(6.98788864163826,-14.9257052987112,4.75847903979292));
#55640=CARTESIAN_POINT('Ctrl Pts',(6.98260450667771,-14.9493619608291,4.72829169721352));
#55641=CARTESIAN_POINT('Ctrl Pts',(6.97647442545662,-14.9768058587017,4.69327161100413));
#55642=CARTESIAN_POINT('Ctrl Pts',(6.96890071874895,-15.0036742903436,4.65964911936404));
#55643=CARTESIAN_POINT('Ctrl Pts',(6.96018164214258,-15.029873005234,4.62746011075656));
#55644=CARTESIAN_POINT('Ctrl Pts',(6.95290685067125,-15.0517319928595,4.60060310102263));
#55645=CARTESIAN_POINT('Ctrl Pts',(6.94483369969458,-15.0731252847008,4.57474347357701));
#55646=CARTESIAN_POINT('Ctrl Pts',(6.93611472286893,-15.0940101584121,4.54988840293343));
#55647=CARTESIAN_POINT('Ctrl Pts',(6.92641726606428,-15.1172388198407,4.5222439924983));
#55648=CARTESIAN_POINT('Ctrl Pts',(6.9159209747684,-15.1398384368918,4.49584242419178));
#55649=CARTESIAN_POINT('Ctrl Pts',(6.90481356637586,-15.1617639785878,4.47067684408087));
#55650=CARTESIAN_POINT('Ctrl Pts',(6.89164887893216,-15.187750499769,4.44085017481732));
#55651=CARTESIAN_POINT('Ctrl Pts',(6.87762735375645,-15.2127898786367,4.41275936110785));
#55652=CARTESIAN_POINT('Ctrl Pts',(6.86305650501248,-15.2368326817435,4.38633881455129));
#55653=CARTESIAN_POINT('Ctrl Pts',(6.85386413204496,-15.2520006666169,4.36967077261212));
#55654=CARTESIAN_POINT('Ctrl Pts',(6.84445212298921,-15.2667724597872,4.35366711183038));
#55655=CARTESIAN_POINT('Ctrl Pts',(6.83488868064054,-15.2811396624472,4.33830772432577));
#55656=CARTESIAN_POINT('Ctrl Pts',(6.82863658643842,-15.2905322118218,4.32826653475569));
#55657=CARTESIAN_POINT('Ctrl Pts',(6.82231963531967,-15.2997519048661,4.31850064377616));
#55658=CARTESIAN_POINT('Ctrl Pts',(6.81595546454256,-15.3087970230533,4.30900383629424));
#55659=CARTESIAN_POINT('Ctrl Pts',(6.812773379154,-15.3133195821468,4.30425543255328));
#55660=CARTESIAN_POINT('Ctrl Pts',(6.80957948092657,-15.3177984978365,4.29957430535766));
#55661=CARTESIAN_POINT('Ctrl Pts',(6.80637586700466,-15.3222336059642,4.29495962197931));
#55662=CARTESIAN_POINT('Ctrl Pts',(6.8047740600437,-15.324451160028,4.29265228029014));
#55663=CARTESIAN_POINT('Ctrl Pts',(6.80316982367116,-15.3266577622202,4.29036154989132));
#55664=CARTESIAN_POINT('Ctrl Pts',(6.80156341558733,-15.3288533933844,4.28808732631316));
#55665=CARTESIAN_POINT('Ctrl Pts',(6.80017844998843,-15.3307463579809,4.28612660322439));
#55666=CARTESIAN_POINT('Ctrl Pts',(6.79918126657756,-15.3321039244195,4.28472268101543));
#55667=CARTESIAN_POINT('Ctrl Pts',(6.79756509623338,-15.3342897856083,4.2824669077432));
#55668=CARTESIAN_POINT('Ctrl Pts',(6.79730668636575,-15.334639283483,4.28210623160855));
#55669=CARTESIAN_POINT('Ctrl Pts',(6.79703237237366,-15.3350099512053,4.28172384280776));
#55670=CARTESIAN_POINT('Ctrl Pts',(6.7967379311547,-15.3354073554815,4.28131407143311));
#55671=CARTESIAN_POINT('Ctrl Pts',(6.78772434840391,-15.3475728951486,4.26876994392498));
#55672=CARTESIAN_POINT('Ctrl Pts',(6.77846784471264,-15.3596525050359,4.25648444123868));
#55673=CARTESIAN_POINT('Ctrl Pts',(6.76897945880369,-15.3716409411952,4.2444655704202));
#55674=CARTESIAN_POINT('Ctrl Pts',(6.73811526233739,-15.4106373998654,4.20537011268854));
#55675=CARTESIAN_POINT('Ctrl Pts',(6.7048017087282,-15.4486674809531,4.16909532298495));
#55676=CARTESIAN_POINT('Ctrl Pts',(6.66950284278148,-15.4855742727397,4.13580485241239));
#55677=CARTESIAN_POINT('Ctrl Pts',(6.64224200441824,-15.5140768905552,4.11009507072465));
#55678=CARTESIAN_POINT('Ctrl Pts',(6.61379575867552,-15.5419100335608,4.0861655014366));
#55679=CARTESIAN_POINT('Ctrl Pts',(6.58435873894976,-15.5690100258892,4.0640921555984));
#55680=CARTESIAN_POINT('Ctrl Pts',(6.54460852115848,-15.6056044436405,4.03428545938306));
#55681=CARTESIAN_POINT('Ctrl Pts',(6.50305392191834,-15.6408613873316,4.00786272879156));
#55682=CARTESIAN_POINT('Ctrl Pts',(6.46023258511493,-15.6746538066925,3.98488306639121));
#55683=CARTESIAN_POINT('Ctrl Pts',(6.42831606070949,-15.6998407031736,3.96775536766484));
#55684=CARTESIAN_POINT('Ctrl Pts',(6.39569462096411,-15.7242144403282,3.95254071434452));
#55685=CARTESIAN_POINT('Ctrl Pts',(6.36257366505378,-15.7477295054672,3.93926371625084));
#55686=CARTESIAN_POINT('Ctrl Pts',(6.33007871080959,-15.7708001247999,3.92623765967438));
#55687=CARTESIAN_POINT('Ctrl Pts',(6.2971030388051,-15.7930443446869,3.91507635689925));
#55688=CARTESIAN_POINT('Ctrl Pts',(6.26385676124029,-15.8144315141987,3.90574866944461));
#55689=CARTESIAN_POINT('Ctrl Pts',(6.99927539745615,-24.8232831402285,9.44704209109788));
#55690=CARTESIAN_POINT('Ctrl Pts',(6.99927539745615,-24.8010531575336,9.4162903362361));
#55691=CARTESIAN_POINT('Ctrl Pts',(6.99927539745615,-24.4365976663568,8.91758027915424));
#55692=CARTESIAN_POINT('Ctrl Pts',(6.99927539745615,-23.6477703264689,8.00909386847417));
#55693=CARTESIAN_POINT('Ctrl Pts',(6.99927539745615,-22.3080761741899,6.88883533571338));
#55694=CARTESIAN_POINT('Ctrl Pts',(6.99927539745615,-20.8057449101191,5.99308684816581));
#55695=CARTESIAN_POINT('Ctrl Pts',(6.99927539745615,-19.1796205257273,5.34745368361758));
#55696=CARTESIAN_POINT('Ctrl Pts',(6.99927539745615,-17.4733157461454,4.96741765649446));
#55697=CARTESIAN_POINT('Ctrl Pts',(6.99927539745615,-15.9617928931792,4.87762288481046));
#55698=CARTESIAN_POINT('Ctrl Pts',(6.99927539745615,-15.0339583706354,4.94001221664358));
#55699=CARTESIAN_POINT('Ctrl Pts',(6.99927539745615,-14.6874883923254,4.98003222191423));
#55700=CARTESIAN_POINT('Ctrl Pts',(7.01782517045299,-25.2179999147367,9.16177341463118));
#55701=CARTESIAN_POINT('Ctrl Pts',(7.01782517045299,-25.19478265848,9.12965654467665));
#55702=CARTESIAN_POINT('Ctrl Pts',(7.01782517045299,-24.8141504925113,8.60881700089838));
#55703=CARTESIAN_POINT('Ctrl Pts',(7.01782517045299,-23.9905674344651,7.66026544206334));
#55704=CARTESIAN_POINT('Ctrl Pts',(7.01782517045299,-22.5908623958162,6.48980066752073));
#55705=CARTESIAN_POINT('Ctrl Pts',(7.01782517045299,-21.0220249302349,5.55445248829491));
#55706=CARTESIAN_POINT('Ctrl Pts',(7.01782517045299,-19.3234985875938,4.88000520626589));
#55707=CARTESIAN_POINT('Ctrl Pts',(7.01782517045299,-17.5410927392784,4.48306759693387));
#55708=CARTESIAN_POINT('Ctrl Pts',(7.01782517045299,-15.962488194199,4.38928801747339));
#55709=CARTESIAN_POINT('Ctrl Pts',(7.01782517045299,-14.9935216292188,4.45442837118926));
#55710=CARTESIAN_POINT('Ctrl Pts',(7.01782517045299,-14.6315898189319,4.4962370680108));
#55711=CARTESIAN_POINT('Ctrl Pts',(6.7281872031432,-25.5366594111987,8.93147265552196));
#55712=CARTESIAN_POINT('Ctrl Pts',(6.7281872031432,-25.5126451173818,8.89825371210526));
#55713=CARTESIAN_POINT('Ctrl Pts',(6.7281872031432,-25.1189533315064,8.35954877332631));
#55714=CARTESIAN_POINT('Ctrl Pts',(6.7281872031432,-24.2673115732516,7.37865214896281));
#55715=CARTESIAN_POINT('Ctrl Pts',(6.7281872031432,-22.819159039915,6.16765528467975));
#55716=CARTESIAN_POINT('Ctrl Pts',(6.7281872031432,-21.1966303353074,5.20033780841415));
#55717=CARTESIAN_POINT('Ctrl Pts',(6.7281872031432,-19.4396530398759,4.50262855029769));
#55718=CARTESIAN_POINT('Ctrl Pts',(6.7281872031432,-17.5958099033305,4.09204609479212));
#55719=CARTESIAN_POINT('Ctrl Pts',(6.7281872031432,-15.9630495188911,3.99504953312507));
#55720=CARTESIAN_POINT('Ctrl Pts',(6.7281872031432,-14.9608765720764,4.06241081917415));
#55721=CARTESIAN_POINT('Ctrl Pts',(6.7281872031432,-14.5864622429053,4.10566354772994));
#55722=CARTESIAN_POINT('Ctrl Pts',(6.25506922963065,-25.6378135708472,8.85836678542715));
#55723=CARTESIAN_POINT('Ctrl Pts',(6.25506922963065,-25.6135462682048,8.82479800364957));
#55724=CARTESIAN_POINT('Ctrl Pts',(6.25506922963065,-25.2157088821168,8.28042193616291));
#55725=CARTESIAN_POINT('Ctrl Pts',(6.25506922963065,-24.3551602678926,7.28925780695488));
#55726=CARTESIAN_POINT('Ctrl Pts',(6.25506922963065,-22.8916287307343,6.06539457741163));
#55727=CARTESIAN_POINT('Ctrl Pts',(6.25506922963065,-21.2520564663921,5.08792887894081));
#55728=CARTESIAN_POINT('Ctrl Pts',(6.25506922963065,-19.4765247042674,4.38283542023071));
#55729=CARTESIAN_POINT('Ctrl Pts',(6.25506922963065,-17.6131791291381,3.96792159232686));
#55730=CARTESIAN_POINT('Ctrl Pts',(6.25506922963065,-15.9632277038415,3.8699038430408));
#55731=CARTESIAN_POINT('Ctrl Pts',(6.25506922963065,-14.9505138389429,3.93797013410656));
#55732=CARTESIAN_POINT('Ctrl Pts',(6.25506922963065,-14.5721371024931,3.9816812510631));
#55733=CARTESIAN_POINT('',(7.00000000000001,-24.7867247203242,9.3325097692458));
#55734=CARTESIAN_POINT('Ctrl Pts',(7.00000000000006,-24.7867247293774,9.3325097625576));
#55735=CARTESIAN_POINT('Ctrl Pts',(7.00000000000006,-24.6891841466124,9.20047771820845));
#55736=CARTESIAN_POINT('Ctrl Pts',(7.00000000006096,-24.5890317764085,9.07102172536068));
#55737=CARTESIAN_POINT('Ctrl Pts',(6.99999999867112,-24.4862334316389,8.94403929589311));
#55738=CARTESIAN_POINT('Ctrl Pts',(6.99999999727842,-24.3832240272285,8.81679615341495));
#55739=CARTESIAN_POINT('Ctrl Pts',(6.99999999421911,-24.2775574615185,8.69203640523486));
#55740=CARTESIAN_POINT('Ctrl Pts',(6.99999999313353,-24.1691581090645,8.56968917785705));
#55741=CARTESIAN_POINT('Ctrl Pts',(6.99999999205177,-24.0611403059592,8.44777259424111));
#55742=CARTESIAN_POINT('Ctrl Pts',(6.99999999470455,-23.9504086005632,8.3282512584488));
#55743=CARTESIAN_POINT('Ctrl Pts',(6.99999999802626,-23.8368520340605,8.21109188955697));
#55744=CARTESIAN_POINT('Ctrl Pts',(6.99999999906758,-23.8012536060717,8.17436403237392));
#55745=CARTESIAN_POINT('Ctrl Pts',(7.00000000000006,-23.7653773200082,8.13786858660161));
#55746=CARTESIAN_POINT('Ctrl Pts',(7.00000000000006,-23.7292190979857,8.10160535508103));
#55747=CARTESIAN_POINT('Ctrl Pts',(7.00000000000006,-23.7003753309043,8.07267782089671));
#55748=CARTESIAN_POINT('Ctrl Pts',(6.99999999938504,-23.6713554071327,8.04389419508844));
#55749=CARTESIAN_POINT('Ctrl Pts',(6.99999999847359,-23.6421621123814,8.01525903994437));
#55750=CARTESIAN_POINT('Ctrl Pts',(6.99999999415761,-23.5039224403086,7.8796623390377));
#55751=CARTESIAN_POINT('Ctrl Pts',(6.999999985704,-23.3617919491904,7.74739742263809));
#55752=CARTESIAN_POINT('Ctrl Pts',(6.99999998494287,-23.2160995784014,7.61883386487858));
#55753=CARTESIAN_POINT('Ctrl Pts',(6.99999998418013,-23.0700992502754,7.48999855582098));
#55754=CARTESIAN_POINT('Ctrl Pts',(6.99999998976671,-22.9205222589565,7.36488057062783));
#55755=CARTESIAN_POINT('Ctrl Pts',(6.9999999946827,-22.767738442797,7.24381675242766));
#55756=CARTESIAN_POINT('Ctrl Pts',(6.99999999757257,-22.6779242372364,7.17264919733506));
#55757=CARTESIAN_POINT('Ctrl Pts',(7.00000000000006,-22.5870025612902,7.10288195460848));
#55758=CARTESIAN_POINT('Ctrl Pts',(7.00000000000006,-22.4950541460765,7.03457718217675));
#55759=CARTESIAN_POINT('Ctrl Pts',(7.00000000000006,-22.4318690559121,6.98763952485299));
#55760=CARTESIAN_POINT('Ctrl Pts',(6.99999999889743,-22.3681959174977,6.94139789754036));
#55761=CARTESIAN_POINT('Ctrl Pts',(6.99999999756665,-22.304043965429,6.89585784795075));
#55762=CARTESIAN_POINT('Ctrl Pts',(6.99999999341031,-22.1036825049342,6.7536256858332));
#55763=CARTESIAN_POINT('Ctrl Pts',(6.99999998911108,-21.898652821419,6.61823403059507));
#55764=CARTESIAN_POINT('Ctrl Pts',(6.99999999137297,-21.6892902101513,6.48986655377202));
#55765=CARTESIAN_POINT('Ctrl Pts',(6.99999999340036,-21.5016335197964,6.37480772973475));
#55766=CARTESIAN_POINT('Ctrl Pts',(7.00000000000006,-21.3104950496311,6.26539244936196));
#55767=CARTESIAN_POINT('Ctrl Pts',(7.00000000000006,-21.1160970528281,6.16178294553015));
#55768=CARTESIAN_POINT('Ctrl Pts',(7.00000000000006,-21.0125348880333,6.10658677742867));
#55769=CARTESIAN_POINT('Ctrl Pts',(6.99999999798932,-20.9080532399373,6.05302326345818));
#55770=CARTESIAN_POINT('Ctrl Pts',(6.99999999626512,-20.8027183557833,6.00113756742284));
#55771=CARTESIAN_POINT('Ctrl Pts',(6.99999999250276,-20.5728669132141,5.88791769559971));
#55772=CARTESIAN_POINT('Ctrl Pts',(6.99999999167287,-20.3389511481081,5.78268995354166));
#55773=CARTESIAN_POINT('Ctrl Pts',(6.99999999476618,-20.1017155246842,5.68575103531911));
#55774=CARTESIAN_POINT('Ctrl Pts',(6.99999999683554,-19.943009495447,5.62090077983214));
#55775=CARTESIAN_POINT('Ctrl Pts',(7.00000000000006,-19.7828182918934,5.55975913888656));
#55776=CARTESIAN_POINT('Ctrl Pts',(7.00000000000006,-19.621370056996,5.50240303026548));
#55777=CARTESIAN_POINT('Ctrl Pts',(7.00000000000006,-19.4741199931052,5.45009096464057));
#55778=CARTESIAN_POINT('Ctrl Pts',(6.99999999705142,-19.325822246007,5.40094132587375));
#55779=CARTESIAN_POINT('Ctrl Pts',(6.99999999409848,-19.1765613925645,5.35498619481664));
#55780=CARTESIAN_POINT('Ctrl Pts',(6.99999998947438,-18.9428301888559,5.28302393645594));
#55781=CARTESIAN_POINT('Ctrl Pts',(6.99999998692793,-18.7067374602874,5.21889241441373));
#55782=CARTESIAN_POINT('Ctrl Pts',(6.99999999182273,-18.4686229513191,5.16272268300951));
#55783=CARTESIAN_POINT('Ctrl Pts',(6.99999999470013,-18.3286474621975,5.12970333588448));
#55784=CARTESIAN_POINT('Ctrl Pts',(7.00000000000006,-18.1879731692716,5.09943628849387));
#55785=CARTESIAN_POINT('Ctrl Pts',(7.00000000000006,-18.0466687179138,5.07195657342431));
#55786=CARTESIAN_POINT('Ctrl Pts',(7.00000000000006,-17.8556422214223,5.03480732834476));
#55787=CARTESIAN_POINT('Ctrl Pts',(6.99999998960242,-17.6634649798387,5.00268525153448));
#55788=CARTESIAN_POINT('Ctrl Pts',(6.99999998461919,-17.4706096574179,4.97570566154593));
#55789=CARTESIAN_POINT('Ctrl Pts',(6.99999997943812,-17.2700973511263,4.94765489404053));
#55790=CARTESIAN_POINT('Ctrl Pts',(6.99999998080614,-17.0688524595463,4.92516342212063));
#55791=CARTESIAN_POINT('Ctrl Pts',(6.99999998755749,-16.8674108909919,4.9082236915833));
#55792=CARTESIAN_POINT('Ctrl Pts',(6.99999999250501,-16.7197904556305,4.89580991614076));
#55793=CARTESIAN_POINT('Ctrl Pts',(7.00000000000006,-16.5720645451366,4.88637647464254));
#55794=CARTESIAN_POINT('Ctrl Pts',(7.00000000000006,-16.4244437708488,4.87990262774485));
#55795=CARTESIAN_POINT('Ctrl Pts',(7.00000000000006,-16.2585064874591,4.87262551805303));
#55796=CARTESIAN_POINT('Ctrl Pts',(6.99999999328001,-16.0927163640638,4.86916233119042));
#55797=CARTESIAN_POINT('Ctrl Pts',(6.9999999927155,-15.9269559837606,4.86945767505926));
#55798=CARTESIAN_POINT('Ctrl Pts',(6.9999999924927,-15.8615333271543,4.86957424200051));
#55799=CARTESIAN_POINT('Ctrl Pts',(6.99999999280525,-15.7961152191328,4.87027685618125));
#55800=CARTESIAN_POINT('Ctrl Pts',(6.9999999934186,-15.730694189542,4.87156433035057));
#55801=CARTESIAN_POINT('Ctrl Pts',(6.99999999496721,-15.5655165568815,4.87481499663831));
#55802=CARTESIAN_POINT('Ctrl Pts',(6.99999999795174,-15.4003202163135,4.8817904164755));
#55803=CARTESIAN_POINT('Ctrl Pts',(6.99999999909501,-15.2350196079666,4.89250633197123));
#55804=CARTESIAN_POINT('Ctrl Pts',(7.0000000001046,-15.0890457501804,4.90196935537002));
#55805=CARTESIAN_POINT('Ctrl Pts',(6.9999999999995,-14.9429903418779,4.91435004126209));
#55806=CARTESIAN_POINT('Ctrl Pts',(6.9999999999995,-14.7967973072039,4.92969292433615));
#55807=CARTESIAN_POINT('',(6.27159471697182,-25.5608579993274,8.76071062883475));
#55808=CARTESIAN_POINT('Origin',(5.999999877384,-24.7867246592848,9.33250977407517));
#55809=CARTESIAN_POINT('Ctrl Pts',(6.27159470456809,-25.5608577604391,8.76071047658128));
#55810=CARTESIAN_POINT('Ctrl Pts',(6.27193966902721,-25.4228903795494,8.57412214168591));
#55811=CARTESIAN_POINT('Ctrl Pts',(6.27225782571643,-25.2809102066271,8.39339828302729));
#55812=CARTESIAN_POINT('Ctrl Pts',(6.27254917034726,-25.1354917711551,8.21861676875514));
#55813=CARTESIAN_POINT('Ctrl Pts',(6.27284515826659,-24.987755737636,8.04104968403698));
#55814=CARTESIAN_POINT('Ctrl Pts',(6.27311347269038,-24.8364709624808,7.86961580871584));
#55815=CARTESIAN_POINT('Ctrl Pts',(6.2733541100562,-24.6822005684409,7.70435943122668));
#55816=CARTESIAN_POINT('Ctrl Pts',(6.27354178927972,-24.5618811506001,7.57547176449234));
#55817=CARTESIAN_POINT('Ctrl Pts',(6.27371263301604,-24.4397448251206,7.45034099904443));
#55818=CARTESIAN_POINT('Ctrl Pts',(6.27386663993444,-24.3160426977393,7.32897316278893));
#55819=CARTESIAN_POINT('Ctrl Pts',(6.27406868999589,-24.1537511416417,7.16974409031388));
#55820=CARTESIAN_POINT('Ctrl Pts',(6.27424176008809,-23.9887664762674,7.01699206659435));
#55821=CARTESIAN_POINT('Ctrl Pts',(6.27438584795811,-23.8216766750998,6.87061872315646));
#55822=CARTESIAN_POINT('Ctrl Pts',(6.27447252017228,-23.7211682629063,6.78257174342696));
#55823=CARTESIAN_POINT('Ctrl Pts',(6.2745487057562,-23.6198972280055,6.69683229111827));
#55824=CARTESIAN_POINT('Ctrl Pts',(6.2746144043585,-23.5179834667241,6.61337488456931));
#55825=CARTESIAN_POINT('Ctrl Pts',(6.27472591341892,-23.3450070659173,6.47172412392615));
#55826=CARTESIAN_POINT('Ctrl Pts',(6.27480721189808,-23.1701816572621,6.33664862667355));
#55827=CARTESIAN_POINT('Ctrl Pts',(6.27485829873449,-22.9940551698525,6.2080049654047));
#55828=CARTESIAN_POINT('Ctrl Pts',(6.27487121299898,-22.9495320753769,6.17548507604218));
#55829=CARTESIAN_POINT('Ctrl Pts',(6.27488219665249,-22.9049256033793,6.14337608661024));
#55830=CARTESIAN_POINT('Ctrl Pts',(6.27489124968589,-22.8602441341368,6.1116754534218));
#55831=CARTESIAN_POINT('Ctrl Pts',(6.27492812707301,-22.6782348822084,5.98254343001002));
#55832=CARTESIAN_POINT('Ctrl Pts',(6.27493296908659,-22.4949851869132,5.8601886507752));
#55833=CARTESIAN_POINT('Ctrl Pts',(6.27490577566025,-22.311038116279,5.74438505749212));
#55834=CARTESIAN_POINT('Ctrl Pts',(6.27488257629484,-22.1541084505275,5.64559022958816));
#55835=CARTESIAN_POINT('Ctrl Pts',(6.27483606089023,-21.9966702918831,5.55156316095694));
#55836=CARTESIAN_POINT('Ctrl Pts',(6.27476622991235,-21.8390323265443,5.46215438396946));
#55837=CARTESIAN_POINT('Ctrl Pts',(6.27472435194508,-21.7444960941419,5.40853551809573));
#55838=CARTESIAN_POINT('Ctrl Pts',(6.27467408870909,-21.6498875057298,5.35657744466591));
#55839=CARTESIAN_POINT('Ctrl Pts',(6.27461544171774,-21.5552687891301,5.30624659367549));
#55840=CARTESIAN_POINT('Ctrl Pts',(6.27458611822207,-21.5079594308303,5.28108116818028));
#55841=CARTESIAN_POINT('Ctrl Pts',(6.27455469615558,-21.4606475361946,5.25632255645321));
#55842=CARTESIAN_POINT('Ctrl Pts',(6.27452117896326,-21.4133405353867,5.23196644753487));
#55843=CARTESIAN_POINT('Ctrl Pts',(6.2745044203671,-21.3896870349827,5.2197883930757));
#55844=CARTESIAN_POINT('Ctrl Pts',(6.27448713781172,-21.3660347577391,5.20771096486579));
#55845=CARTESIAN_POINT('Ctrl Pts',(6.27446933129768,-21.3423846215274,5.19573362252721));
#55846=CARTESIAN_POINT('Ctrl Pts',(6.2744539194677,-21.3219150406985,5.18536703626652));
#55847=CARTESIAN_POINT('Ctrl Pts',(6.27443872981217,-21.3022173582447,5.17546074478448));
#55848=CARTESIAN_POINT('Ctrl Pts',(6.27442216608405,-21.2812921796582,5.16501365511446));
#55849=CARTESIAN_POINT('Ctrl Pts',(6.27441959241852,-21.2780408336758,5.16339039044863));
#55850=CARTESIAN_POINT('Ctrl Pts',(6.27441698557903,-21.2747598068533,5.16175416025187));
#55851=CARTESIAN_POINT('Ctrl Pts',(6.27441433957761,-21.2714415474909,5.16010131199954));
#55852=CARTESIAN_POINT('Ctrl Pts',(6.2744027961717,-21.2569653592138,5.15289062112795));
#55853=CARTESIAN_POINT('Ctrl Pts',(6.27439106289382,-21.2424654770366,5.14570487885345));
#55854=CARTESIAN_POINT('Ctrl Pts',(6.27437913974498,-21.2279419562817,5.13854426366239));
#55855=CARTESIAN_POINT('Ctrl Pts',(6.27420010632505,-21.0098623512413,5.03102321838198));
#55856=CARTESIAN_POINT('Ctrl Pts',(6.27397826279242,-20.7864492528495,4.92916545629279));
#55857=CARTESIAN_POINT('Ctrl Pts',(6.27371361342478,-20.557965514843,4.83351364503586));
#55858=CARTESIAN_POINT('Ctrl Pts',(6.27345238602023,-20.3324361119388,4.73909862859882));
#55859=CARTESIAN_POINT('Ctrl Pts',(6.27314945258748,-20.1019663004246,4.65073011011745));
#55860=CARTESIAN_POINT('Ctrl Pts',(6.27280481907884,-19.8668531444355,4.56895455785876));
#55861=CARTESIAN_POINT('Ctrl Pts',(6.27260797682087,-19.7325649706386,4.52224730522605));
#55862=CARTESIAN_POINT('Ctrl Pts',(6.27239753085122,-19.5967628237501,4.47769131674242));
#55863=CARTESIAN_POINT('Ctrl Pts',(6.27217348257728,-19.459508772695,4.43539209668543));
#55864=CARTESIAN_POINT('Ctrl Pts',(6.271770135294,-19.2124144852199,4.35924209921435));
#55865=CARTESIAN_POINT('Ctrl Pts',(6.27132270318547,-18.9606112060094,4.29040494719483));
#55866=CARTESIAN_POINT('Ctrl Pts',(6.27083119645392,-18.7045321058939,4.22947048310928));
#55867=CARTESIAN_POINT('Ctrl Pts',(6.27036732592469,-18.46285169733,4.17196221254298));
#55868=CARTESIAN_POINT('Ctrl Pts',(6.26986419915261,-18.2173631494559,4.12149308400121));
#55869=CARTESIAN_POINT('Ctrl Pts',(6.26932182605469,-17.9684785610763,4.07857896905072));
#55870=CARTESIAN_POINT('Ctrl Pts',(6.26905885374381,-17.8478056228359,4.05777184564955));
#55871=CARTESIAN_POINT('Ctrl Pts',(6.26878665527169,-17.7263350402975,4.03874108335308));
#55872=CARTESIAN_POINT('Ctrl Pts',(6.26850523199004,-17.6041178805849,4.02154717118703));
#55873=CARTESIAN_POINT('Ctrl Pts',(6.26791730977991,-17.3487936507139,3.98562731842176));
#55874=CARTESIAN_POINT('Ctrl Pts',(6.26728912705079,-17.090207808471,3.95772398693753));
#55875=CARTESIAN_POINT('Ctrl Pts',(6.26662069841196,-16.8288453305975,3.93824738933384));
#55876=CARTESIAN_POINT('Ctrl Pts',(6.26595958210327,-16.5703420490729,3.91898385757345));
#55877=CARTESIAN_POINT('Ctrl Pts',(6.26525909558954,-16.3091225019333,3.90796371089906));
#55878=CARTESIAN_POINT('Ctrl Pts',(6.2645192563654,-16.0457065940275,3.90559011833706));
#55879=CARTESIAN_POINT('Ctrl Pts',(6.26430324577284,-15.9687971460041,3.90489710136923));
#55880=CARTESIAN_POINT('Ctrl Pts',(6.26408388053192,-15.8917008014357,3.90494121137407));
#55881=CARTESIAN_POINT('Ctrl Pts',(6.26386116113799,-15.8144313373356,3.90573258303281));
#55882=CARTESIAN_POINT('Ctrl Pts',(6.99999999998952,-24.1259274559597,10.9278021978186));
#55883=CARTESIAN_POINT('Ctrl Pts',(6.99999999998952,-24.1259309536957,10.9277942568591));
#55884=CARTESIAN_POINT('Ctrl Pts',(6.99999999998951,-24.2426238189736,10.6628645501556));
#55885=CARTESIAN_POINT('Ctrl Pts',(6.99999999998952,-24.4687760835905,10.1334756387629));
#55886=CARTESIAN_POINT('Ctrl Pts',(6.99999999998952,-24.6831198888034,9.59921869200081));
#55887=CARTESIAN_POINT('Ctrl Pts',(6.99999999998952,-24.7867214499183,9.3325057406461));
#55888=CARTESIAN_POINT('Ctrl Pts',(7.00000270572098,-24.6668575634642,11.1660644378209));
#55889=CARTESIAN_POINT('Ctrl Pts',(7.00000270572098,-24.6668611143903,11.166056376103));
#55890=CARTESIAN_POINT('Ctrl Pts',(7.00000270572098,-24.7853285323176,10.8970978743295));
#55891=CARTESIAN_POINT('Ctrl Pts',(7.00000270572098,-25.0149163654532,10.3596666804281));
#55892=CARTESIAN_POINT('Ctrl Pts',(7.00000270572098,-25.2325164806272,9.81729343793396));
#55893=CARTESIAN_POINT('Ctrl Pts',(7.00000270572098,-25.3376935135448,9.54652457474008));
#55894=CARTESIAN_POINT('Ctrl Pts',(6.57967197783012,-25.0472372157093,11.3336093881579));
#55895=CARTESIAN_POINT('Ctrl Pts',(6.57967197783012,-25.0472408040386,11.3336012415232));
#55896=CARTESIAN_POINT('Ctrl Pts',(6.57967197783013,-25.1669560795239,11.0618097089269));
#55897=CARTESIAN_POINT('Ctrl Pts',(6.57967197783013,-25.3989597892029,10.5187232176258));
#55898=CARTESIAN_POINT('Ctrl Pts',(6.57967197783013,-25.6188497270954,9.97064263198274));
#55899=CARTESIAN_POINT('Ctrl Pts',(6.57967197783013,-25.725134624792,9.69702166956874));
#55900=CARTESIAN_POINT('Ctrl Pts',(5.98852435812812,-25.041028565088,11.3308746781035));
#55901=CARTESIAN_POINT('Ctrl Pts',(5.98852435812812,-25.0410321528068,11.3308665328549));
#55902=CARTESIAN_POINT('Ctrl Pts',(5.98852435812812,-25.1607270604577,11.0591212416852));
#55903=CARTESIAN_POINT('Ctrl Pts',(5.98852435812812,-25.3926913375983,10.5161270575494));
#55904=CARTESIAN_POINT('Ctrl Pts',(5.98852435812812,-25.612543900438,9.96813962856901));
#55905=CARTESIAN_POINT('Ctrl Pts',(5.98852435812812,-25.7188107152924,9.69456521882008));
#55906=CARTESIAN_POINT('',(6.99999999994034,-24.1259366382796,10.9277762174568));
#55907=CARTESIAN_POINT('',(5.98852583803503,-25.0410393004634,11.3308502321861));
#55908=CARTESIAN_POINT('Origin',(5.999999999061,-24.1259421376201,10.9277802195584));
#55909=CARTESIAN_POINT('',(5.98852581355429,-25.7188095579012,9.69456736137508));
#55910=CARTESIAN_POINT('Origin',(5.98846824183665,11.4751154476891,-4.75314848428435));
#55911=CARTESIAN_POINT('Origin',(6.,-24.7867247762541,9.33250981979305));
#55912=CARTESIAN_POINT('Origin',(6.99999997875368,11.466399700858,-4.74964867790657));
#55913=CARTESIAN_POINT('Origin',(5.999999877384,-24.7867246592848,9.33250977407517));
#55914=CARTESIAN_POINT('Origin',(5.99999764419348,-24.7867226422921,9.33250908124204));
#55915=CARTESIAN_POINT('Ctrl Pts',(-6.09469640311948,-25.6962418117966,
9.7551784065007));
#55916=CARTESIAN_POINT('Ctrl Pts',(-6.05660168697869,-25.7007415434035,
9.74233001812424));
#55917=CARTESIAN_POINT('Ctrl Pts',(-5.71257762314107,-25.7410984324824,
9.6273925641447));
#55918=CARTESIAN_POINT('Ctrl Pts',(-5.02644182509294,-25.8164780718308,
9.41768044975332));
#55919=CARTESIAN_POINT('Ctrl Pts',(-3.98600488143526,-25.9134384022202,
9.15524677412187));
#55920=CARTESIAN_POINT('Ctrl Pts',(-2.8123888149195,-25.9986878426019,8.92978553974035));
#55921=CARTESIAN_POINT('Ctrl Pts',(-1.5205631427427,-26.0604307224869,8.77036250541219));
#55922=CARTESIAN_POINT('Ctrl Pts',(-0.189421525835868,-26.0860723981169,
8.70665832164758));
#55923=CARTESIAN_POINT('Ctrl Pts',(1.08612112080106,-26.0718380483953,8.74173357669442));
#55924=CARTESIAN_POINT('Ctrl Pts',(2.24134091421009,-26.0285585011884,8.85233532810853));
#55925=CARTESIAN_POINT('Ctrl Pts',(3.27311180245308,-25.9668527571587,9.01365179906474));
#55926=CARTESIAN_POINT('Ctrl Pts',(4.20014655779273,-25.8939006521098,9.20794869621394));
#55927=CARTESIAN_POINT('Ctrl Pts',(5.05723014173037,-25.8125878936172,9.4287012924232));
#55928=CARTESIAN_POINT('Ctrl Pts',(5.68071122126434,-25.7446165392363,9.61762164998467));
#55929=CARTESIAN_POINT('Ctrl Pts',(6.02262167191654,-25.7047562746841,9.73086139421362));
#55930=CARTESIAN_POINT('Ctrl Pts',(6.09456166924508,-25.6962600629342,9.75512415601962));
#55931=CARTESIAN_POINT('Ctrl Pts',(-6.21867431498588,-25.8360125710361,
9.42697393428334));
#55932=CARTESIAN_POINT('Ctrl Pts',(-6.17985088714009,-25.8404824786046,
9.41383765250037));
#55933=CARTESIAN_POINT('Ctrl Pts',(-5.82924224916864,-25.8805416875889,
9.29631173738694));
#55934=CARTESIAN_POINT('Ctrl Pts',(-5.12989137233682,-25.9548390426123,
9.08164968448808));
#55935=CARTESIAN_POINT('Ctrl Pts',(-4.06887094891187,-26.0493410505566,
8.81251246578824));
#55936=CARTESIAN_POINT('Ctrl Pts',(-2.87132776045126,-26.1315203199728,
8.5808712554897));
#55937=CARTESIAN_POINT('Ctrl Pts',(-1.55248691671686,-26.1902927337396,
8.41678346782181));
#55938=CARTESIAN_POINT('Ctrl Pts',(-0.19335884440114,-26.2142179075024,
8.35106522395349));
#55939=CARTESIAN_POINT('Ctrl Pts',(1.108874349186,-26.2009903666146,8.38726562889104));
#55940=CARTESIAN_POINT('Ctrl Pts',(2.28838573698317,-26.1600181790614,8.50117758368943));
#55941=CARTESIAN_POINT('Ctrl Pts',(3.34148469930592,-26.100892207404,8.66706320406161));
#55942=CARTESIAN_POINT('Ctrl Pts',(4.2872641912706,-26.0303266009707,8.86657455129211));
#55943=CARTESIAN_POINT('Ctrl Pts',(5.16125575357753,-25.9509728497055,9.09291528453062));
#55944=CARTESIAN_POINT('Ctrl Pts',(5.79676396111412,-25.8840139145535,9.2863126503946));
#55945=CARTESIAN_POINT('Ctrl Pts',(6.14522058517763,-25.844468417588,9.40211094159923));
#55946=CARTESIAN_POINT('Ctrl Pts',(6.21853693462757,-25.8360280913984,9.42691729984634));
#55947=CARTESIAN_POINT('Ctrl Pts',(-6.32919761543151,-25.7772858661747,
9.07051004505295));
#55948=CARTESIAN_POINT('Ctrl Pts',(-6.28967065067404,-25.7817133140807,
9.05716267819206));
#55949=CARTESIAN_POINT('Ctrl Pts',(-5.93271715893866,-25.8213579419598,
8.9377585934402));
#55950=CARTESIAN_POINT('Ctrl Pts',(-5.22084676055086,-25.8942953190302,
8.71984047487983));
#55951=CARTESIAN_POINT('Ctrl Pts',(-4.14083391245333,-25.9858860937408,
8.4469072451494));
#55952=CARTESIAN_POINT('Ctrl Pts',(-2.9218247883032,-26.064533180692,8.21226132360347));
#55953=CARTESIAN_POINT('Ctrl Pts',(-1.57942699571631,-26.1199617139831,
8.04629578965705));
#55954=CARTESIAN_POINT('Ctrl Pts',(-0.19662764179811,-26.1419937501351,
7.98000626123406));
#55955=CARTESIAN_POINT('Ctrl Pts',(1.1279836696488,-26.1298735851424,8.01650033217842));
#55956=CARTESIAN_POINT('Ctrl Pts',(2.32846860320679,-26.0914804388835,8.13163211550858));
#55957=CARTESIAN_POINT('Ctrl Pts',(3.40040463577914,-26.0352882674276,8.2995525215612));
#55958=CARTESIAN_POINT('Ctrl Pts',(4.36313923323556,-25.9674885931878,8.50172441513352));
#55959=CARTESIAN_POINT('Ctrl Pts',(5.25277086508226,-25.8904646791243,8.73128493448436));
#55960=CARTESIAN_POINT('Ctrl Pts',(5.89966040962877,-25.8247715602233,8.92760803942481));
#55961=CARTESIAN_POINT('Ctrl Pts',(6.25441184426259,-25.7856590242105,9.0452475831158));
#55962=CARTESIAN_POINT('Ctrl Pts',(6.32905697510172,-25.7772984101985,9.07045271479765));
#55963=CARTESIAN_POINT('Ctrl Pts',(-6.39488356510505,-25.5363210851819,
8.78685862229896));
#55964=CARTESIAN_POINT('Ctrl Pts',(-6.35487788300617,-25.5407054580702,
8.77343701897817));
#55965=CARTESIAN_POINT('Ctrl Pts',(-5.99361978169661,-25.5799359843783,
8.6533993304153));
#55966=CARTESIAN_POINT('Ctrl Pts',(-5.27347862179922,-25.6516209548836,
8.43484619237215));
#55967=CARTESIAN_POINT('Ctrl Pts',(-4.18145578460061,-25.7406725883865,
8.16210729422091));
#55968=CARTESIAN_POINT('Ctrl Pts',(-2.94953678778058,-25.8163266294645,
7.92849078581892));
#55969=CARTESIAN_POINT('Ctrl Pts',(-1.59373038385119,-25.8689857738098,
7.76397286656282));
#55970=CARTESIAN_POINT('Ctrl Pts',(-0.198299206200063,-25.8894847637204,
7.69871982059602));
#55971=CARTESIAN_POINT('Ctrl Pts',(1.13802038687766,-25.878258581833,7.73459107892983));
#55972=CARTESIAN_POINT('Ctrl Pts',(2.35020389933381,-25.841985032254,7.84850202252168));
#55973=CARTESIAN_POINT('Ctrl Pts',(3.43313687205662,-25.7882490837982,8.01534045536797));
#55974=CARTESIAN_POINT('Ctrl Pts',(4.40622315056078,-25.7228108459456,8.21685902817043));
#55975=CARTESIAN_POINT('Ctrl Pts',(5.3057872814089,-25.6478273726657,8.44635273790059));
#55976=CARTESIAN_POINT('Ctrl Pts',(5.96018217347372,-25.5832948665882,8.64321714159226));
#55977=CARTESIAN_POINT('Ctrl Pts',(6.31919070575898,-25.5446108926227,8.76145682819641));
#55978=CARTESIAN_POINT('Ctrl Pts',(6.39473997492991,-25.5363312511989,8.78680248516681));
#55979=CARTESIAN_POINT('',(-5.98852245733359,-25.7188096065167,9.69456809190346));
#55980=CARTESIAN_POINT('Ctrl Pts',(-5.98852261948844,-25.7188097472697,
9.69456765143706));
#55981=CARTESIAN_POINT('Ctrl Pts',(-5.87205076808918,-25.7323508459181,
9.65601640935633));
#55982=CARTESIAN_POINT('Ctrl Pts',(-5.74888355778406,-25.746373594707,9.61637880011002));
#55983=CARTESIAN_POINT('Ctrl Pts',(-5.61901871697422,-25.7607490246833,
9.5760400312444));
#55984=CARTESIAN_POINT('Ctrl Pts',(-5.51146429426311,-25.7726547958118,
9.54263135056406));
#55985=CARTESIAN_POINT('Ctrl Pts',(-5.39931579746942,-25.7848021023116,
9.50874244458172));
#55986=CARTESIAN_POINT('Ctrl Pts',(-5.28257497451045,-25.7971025206909,
9.47461444800713));
#55987=CARTESIAN_POINT('Ctrl Pts',(-5.21037293139857,-25.8047101023029,
9.45350691237782));
#55988=CARTESIAN_POINT('Ctrl Pts',(-5.13641382824573,-25.8123749355037,
9.43231101177835));
#55989=CARTESIAN_POINT('Ctrl Pts',(-5.06069778882864,-25.8200705226206,
9.41109484794326));
#55990=CARTESIAN_POINT('Ctrl Pts',(-5.00129388444668,-25.8261081855091,
9.39444945843907));
#55991=CARTESIAN_POINT('Ctrl Pts',(-4.94080854949479,-25.8321647187785,
9.377791649925));
#55992=CARTESIAN_POINT('Ctrl Pts',(-4.87924165198486,-25.8382274288517,
9.36115618324037));
#55993=CARTESIAN_POINT('Ctrl Pts',(-4.8092217112253,-25.8451225399803,9.34223669177861));
#55994=CARTESIAN_POINT('Ctrl Pts',(-4.73780290849893,-25.8520255508772,
9.32334635625624));
#55995=CARTESIAN_POINT('Ctrl Pts',(-4.66498524299772,-25.8589160889116,
9.30453992876295));
#55996=CARTESIAN_POINT('Ctrl Pts',(-4.62857641024712,-25.8623613579288,
9.2951367150163));
#55997=CARTESIAN_POINT('Ctrl Pts',(-4.59181786184596,-25.8658035036575,
9.28575447631326));
#55998=CARTESIAN_POINT('Ctrl Pts',(-4.55470959785817,-25.8692398176418,
9.27640039284914));
#55999=CARTESIAN_POINT('Ctrl Pts',(-4.53615546586427,-25.8709579746339,
9.27172335111707));
#56000=CARTESIAN_POINT('Ctrl Pts',(-4.51751390497513,-25.8726746733591,
9.26705334806893));
#56001=CARTESIAN_POINT('Ctrl Pts',(-4.49878491520425,-25.8743895701679,
9.26239128860525));
#56002=CARTESIAN_POINT('Ctrl Pts',(-4.4894204203188,-25.8752470185724,9.26006025887341));
#56003=CARTESIAN_POINT('Ctrl Pts',(-4.48003406821296,-25.8761040164758,
9.25773121502947));
#56004=CARTESIAN_POINT('Ctrl Pts',(-4.47062585888851,-25.8769605203525,
9.25540427130754));
#56005=CARTESIAN_POINT('Ctrl Pts',(-4.46121764956405,-25.8778170242292,
9.25307732758562));
#56006=CARTESIAN_POINT('Ctrl Pts',(-4.45054315232633,-25.8787856647035,
9.25044668891445));
#56007=CARTESIAN_POINT('Ctrl Pts',(-4.44233565926112,-25.8795285061608,
9.24842985504751));
#56008=CARTESIAN_POINT('Ctrl Pts',(-4.30838925356762,-25.8916516895023,
9.21551509712931));
#56009=CARTESIAN_POINT('Ctrl Pts',(-4.17012435788879,-25.9037024484591,
9.18295084365975));
#56010=CARTESIAN_POINT('Ctrl Pts',(-4.02753309951194,-25.9155531876057,
9.15106007112726));
#56011=CARTESIAN_POINT('Ctrl Pts',(-3.8905339033088,-25.9269391712625,9.12041997261784));
#56012=CARTESIAN_POINT('Ctrl Pts',(-3.74954081454694,-25.9381402957922,
9.09040173486523));
#56013=CARTESIAN_POINT('Ctrl Pts',(-3.60456156897667,-25.9490391261433,
9.06130964661601));
#56014=CARTESIAN_POINT('Ctrl Pts',(-3.45662342664788,-25.960160391876,9.03162381486039));
#56015=CARTESIAN_POINT('Ctrl Pts',(-3.30453072157153,-25.9709665875444,
9.00290331842774));
#56016=CARTESIAN_POINT('Ctrl Pts',(-3.14828345387676,-25.9813235521379,
8.97548872364016));
#56017=CARTESIAN_POINT('Ctrl Pts',(-3.07015982002938,-25.9865020344347,
8.96178142624636));
#56018=CARTESIAN_POINT('Ctrl Pts',(-2.99099754541688,-25.9915680760911,
8.94840082530653));
#56019=CARTESIAN_POINT('Ctrl Pts',(-2.91079662918044,-25.9965041492459,
8.93539060519317));
#56020=CARTESIAN_POINT('Ctrl Pts',(-2.89466050088125,-25.997497268944,8.9327729969313));
#56021=CARTESIAN_POINT('Ctrl Pts',(-2.87848233137155,-25.998485127942,8.93017037799633));
#56022=CARTESIAN_POINT('Ctrl Pts',(-2.86226211536348,-25.9994675784444,
8.92758311470445));
#56023=CARTESIAN_POINT('Ctrl Pts',(-2.83817290394011,-26.0009266501271,
8.92374067928837));
#56024=CARTESIAN_POINT('Ctrl Pts',(-2.8139909532798,-26.0023737929314,8.91993211216811));
#56025=CARTESIAN_POINT('Ctrl Pts',(-2.78971627344246,-26.003808543257,8.91615858572895));
#56026=CARTESIAN_POINT('Ctrl Pts',(-2.76940638392122,-26.0050089554065,
8.91300139042923));
#56027=CARTESIAN_POINT('Ctrl Pts',(-2.74903157928846,-26.006200691413,8.90986872755713));
#56028=CARTESIAN_POINT('Ctrl Pts',(-2.72859185955307,-26.0073834764163,
8.90676129069268));
#56029=CARTESIAN_POINT('Ctrl Pts',(-2.71837199968538,-26.007974868918,8.90520757226045));
#56030=CARTESIAN_POINT('Ctrl Pts',(-2.70813591104199,-26.0085640236571,
8.90366016032589));
#56031=CARTESIAN_POINT('Ctrl Pts',(-2.69788359362411,-26.0091509061281,
8.90211914177612));
#56032=CARTESIAN_POINT('Ctrl Pts',(-2.68763127620623,-26.0097377885991,
8.90057812322635));
#56033=CARTESIAN_POINT('Ctrl Pts',(-2.67595577371932,-26.0104020578559,
8.89883444796471));
#56034=CARTESIAN_POINT('Ctrl Pts',(-2.66707795504813,-26.0109047021626,
8.8975153532073));
#56035=CARTESIAN_POINT('Ctrl Pts',(-2.48139215827501,-26.0214178599607,
8.8699255622776));
#56036=CARTESIAN_POINT('Ctrl Pts',(-2.29080876604695,-26.0311760156796,
8.84445328322325));
#56037=CARTESIAN_POINT('Ctrl Pts',(-2.09532194105447,-26.0399856650684,
8.82157126467362));
#56038=CARTESIAN_POINT('Ctrl Pts',(-1.9917234742176,-26.0446543488535,8.80944491273167));
#56039=CARTESIAN_POINT('Ctrl Pts',(-1.88674823703957,-26.0490562995372,
8.79804672030007));
#56040=CARTESIAN_POINT('Ctrl Pts',(-1.780397909139,-26.0531602706882,8.78745187647168));
#56041=CARTESIAN_POINT('Ctrl Pts',(-1.69972470653747,-26.0562733828212,
8.77941504198727));
#56042=CARTESIAN_POINT('Ctrl Pts',(-1.61826034686804,-26.0592154388561,
8.77183925424756));
#56043=CARTESIAN_POINT('Ctrl Pts',(-1.53600337413081,-26.0619732073235,
8.76475545687387));
#56044=CARTESIAN_POINT('Ctrl Pts',(-1.46173164277354,-26.0644632605304,
8.75835933168204));
#56045=CARTESIAN_POINT('Ctrl Pts',(-1.38681370638488,-26.0668030643981,
8.75236433646886));
#56046=CARTESIAN_POINT('Ctrl Pts',(-1.3112508292327,-26.0689820755537,8.7467928800968));
#56047=CARTESIAN_POINT('Ctrl Pts',(-1.231625923349,-26.071278223672,8.74092191930256));
#56048=CARTESIAN_POINT('Ctrl Pts',(-1.15128415269192,-26.0733958218917,
8.73552129254775));
#56049=CARTESIAN_POINT('Ctrl Pts',(-1.07022551571206,-26.0753224370171,
8.73061668494928));
#56050=CARTESIAN_POINT('Ctrl Pts',(-1.02969619722213,-26.0762857445798,
8.72816438115004));
#56051=CARTESIAN_POINT('Ctrl Pts',(-0.98898766215019,-26.0772013021562,
8.72583608075884));
#56052=CARTESIAN_POINT('Ctrl Pts',(-0.948099910399618,-26.0780675402656,
8.72363495437701));
#56053=CARTESIAN_POINT('Ctrl Pts',(-0.927656034524333,-26.0785006593203,
8.7225343911861));
#56054=CARTESIAN_POINT('Ctrl Pts',(-0.907167354479833,-26.0789214482325,
8.72146562140689));
#56055=CARTESIAN_POINT('Ctrl Pts',(-0.886633870263706,-26.0793297099792,
8.72042903833157));
#56056=CARTESIAN_POINT('Ctrl Pts',(-0.876367128155643,-26.0795338408526,
8.71991074679392));
#56057=CARTESIAN_POINT('Ctrl Pts',(-0.866089185004711,-26.079734839917,
8.71940050192643));
#56058=CARTESIAN_POINT('Ctrl Pts',(-0.855800040811281,-26.079932682501,
8.7188983526701));
#56059=CARTESIAN_POINT('Ctrl Pts',(-0.845510896617851,-26.0801305250849,
8.71839620341376));
#56060=CARTESIAN_POINT('Ctrl Pts',(-0.833523570718007,-26.0803565416018,
8.71782265449286));
#56061=CARTESIAN_POINT('Ctrl Pts',(-0.824899005104173,-26.0805167160892,
8.71741624059158));
#56062=CARTESIAN_POINT('Ctrl Pts',(-0.603175520651301,-26.0846345403429,
8.70696800350271));
#56063=CARTESIAN_POINT('Ctrl Pts',(-0.379356108570173,-26.0871465246656,
8.70066472775404));
#56064=CARTESIAN_POINT('Ctrl Pts',(-0.153436083497702,-26.0879151272826,
8.69871721344072));
#56065=CARTESIAN_POINT('Ctrl Pts',(-0.0981464446286718,-26.0881032281873,
8.69824059627036));
#56066=CARTESIAN_POINT('Ctrl Pts',(-0.0427310278451865,-26.0881867999571,
8.69802505275581));
#56067=CARTESIAN_POINT('Ctrl Pts',(0.0128096108926353,-26.0881656968573,
8.69807222268358));
#56068=CARTESIAN_POINT('Ctrl Pts',(0.154052750421511,-26.0881120304222,
8.69819217860849));
#56069=CARTESIAN_POINT('Ctrl Pts',(0.296108408152308,-26.0873798254852,
8.7000158483331));
#56070=CARTESIAN_POINT('Ctrl Pts',(0.438976598234224,-26.0859626567222,
8.70358283824473));
#56071=CARTESIAN_POINT('Ctrl Pts',(0.510410693275183,-26.0852540723408,
8.70536633320055));
#56072=CARTESIAN_POINT('Ctrl Pts',(0.582047920928446,-26.0843742507233,
8.70758565970145));
#56073=CARTESIAN_POINT('Ctrl Pts',(0.653888281158019,-26.0833228711942,
8.71024444189027));
#56074=CARTESIAN_POINT('Ctrl Pts',(0.689808461272805,-26.0827971814297,
8.71157383298468));
#56075=CARTESIAN_POINT('Ctrl Pts',(0.725779424517649,-26.0822286026698,
8.71301308815532));
#56076=CARTESIAN_POINT('Ctrl Pts',(0.761801170818189,-26.0816171119166,
8.71456262061539));
#56077=CARTESIAN_POINT('Ctrl Pts',(0.779812043968459,-26.0813113665399,
8.71533738684542));
#56078=CARTESIAN_POINT('Ctrl Pts',(0.797835612882008,-26.0809948932044,
8.71613972241004));
#56079=CARTESIAN_POINT('Ctrl Pts',(0.815871877547348,-26.080667690937,8.71696967412839));
#56080=CARTESIAN_POINT('Ctrl Pts',(0.833908142212687,-26.0803404886696,
8.71779962584674));
#56081=CARTESIAN_POINT('Ctrl Pts',(0.853574764293333,-26.0799713301349,
8.71873647825257));
#56082=CARTESIAN_POINT('Ctrl Pts',(0.870018758785876,-26.079653897058,8.71954242311313));
#56083=CARTESIAN_POINT('Ctrl Pts',(0.954872427155101,-26.078015891095,8.72370122880682));
#56084=CARTESIAN_POINT('Ctrl Pts',(1.0391059101382,-26.076156590501,8.72843204864025));
#56085=CARTESIAN_POINT('Ctrl Pts',(1.12271338003659,-26.0740881719382,8.73370882155194));
#56086=CARTESIAN_POINT('Ctrl Pts',(1.3402282305506,-26.0687069332157,8.74743697852737));
#56087=CARTESIAN_POINT('Ctrl Pts',(1.5535046430587,-26.0619120284224,8.76485717734693));
#56088=CARTESIAN_POINT('Ctrl Pts',(1.76254242009392,-26.0539162720016,8.78549732054007));
#56089=CARTESIAN_POINT('Ctrl Pts',(1.93919399353098,-26.0471592973887,8.80293968824389));
#56090=CARTESIAN_POINT('Ctrl Pts',(2.11281902545704,-26.0395442787905,8.82268239493087));
#56091=CARTESIAN_POINT('Ctrl Pts',(2.28342873011419,-26.0311868724098,8.84446388766023));
#56092=CARTESIAN_POINT('Ctrl Pts',(2.31456109991648,-26.0296618368524,8.84843851201034));
#56093=CARTESIAN_POINT('Ctrl Pts',(2.34559309142218,-26.0281120514085,8.85248107847408));
#56094=CARTESIAN_POINT('Ctrl Pts',(2.37652480038782,-26.0265381896921,8.85659000339911));
#56095=CARTESIAN_POINT('Ctrl Pts',(2.47723059023904,-26.0214140955968,8.86996761956882));
#56096=CARTESIAN_POINT('Ctrl Pts',(2.57774644974939,-26.0159915621639,8.88416101575656));
#56097=CARTESIAN_POINT('Ctrl Pts',(2.67730193160887,-26.0103253466226,8.89903408455566));
#56098=CARTESIAN_POINT('Ctrl Pts',(2.77899779894568,-26.0045373107131,8.91422691576128));
#56099=CARTESIAN_POINT('Ctrl Pts',(2.87969140145513,-25.9984950673453,8.93012887625942));
#56100=CARTESIAN_POINT('Ctrl Pts',(2.97857178122217,-25.9922749026816,8.94654430623396));
#56101=CARTESIAN_POINT('Ctrl Pts',(3.01268321850991,-25.990129090162,8.95220724878584));
#56102=CARTESIAN_POINT('Ctrl Pts',(3.04657896412302,-25.987962252216,8.95793087169091));
#56103=CARTESIAN_POINT('Ctrl Pts',(3.08022604339517,-25.9857779723932,8.96370583404467));
#56104=CARTESIAN_POINT('Ctrl Pts',(3.158836884694,-25.9806747634902,8.97719807940202));
#56105=CARTESIAN_POINT('Ctrl Pts',(3.23630489543888,-25.975463261375,8.99100506538785));
#56106=CARTESIAN_POINT('Ctrl Pts',(3.31262859492041,-25.970160982455,9.00508184636205));
#56107=CARTESIAN_POINT('Ctrl Pts',(3.45637318408933,-25.9601749111536,9.03159341631611));
#56108=CARTESIAN_POINT('Ctrl Pts',(3.59605850748064,-25.9498675873679,9.05906057616685));
#56109=CARTESIAN_POINT('Ctrl Pts',(3.73168881455355,-25.9393524808365,9.08719458139868));
#56110=CARTESIAN_POINT('Ctrl Pts',(3.83551160795134,-25.9313033378646,9.10873070467139));
#56111=CARTESIAN_POINT('Ctrl Pts',(3.93695723417314,-25.9231322695015,9.13065783474855));
#56112=CARTESIAN_POINT('Ctrl Pts',(4.03602569256835,-25.9148863293522,9.15285338040713));
#56113=CARTESIAN_POINT('Ctrl Pts',(4.06079280716715,-25.9128248443149,9.15840226682177));
#56114=CARTESIAN_POINT('Ctrl Pts',(4.08642489231271,-25.9106752273038,9.16419233880571));
#56115=CARTESIAN_POINT('Ctrl Pts',(4.1143843731552,-25.9083070134603,9.17057701734529));
#56116=CARTESIAN_POINT('Ctrl Pts',(4.14234385399768,-25.9059387996168,9.17696169588488));
#56117=CARTESIAN_POINT('Ctrl Pts',(4.17012474473776,-25.9035635175156,9.18337091410878));
#56118=CARTESIAN_POINT('Ctrl Pts',(4.19772704539506,-25.9011821865988,9.18980197274797));
#56119=CARTESIAN_POINT('Ctrl Pts',(4.20554193317243,-25.9005079734559,9.19162276305741));
#56120=CARTESIAN_POINT('Ctrl Pts',(4.21334250587241,-25.8998332751815,9.19344530470966));
#56121=CARTESIAN_POINT('Ctrl Pts',(4.22112876290821,-25.8991581142587,9.19526953801704));
#56122=CARTESIAN_POINT('Ctrl Pts',(4.26834485877105,-25.8950639182024,9.2063317434286));
#56123=CARTESIAN_POINT('Ctrl Pts',(4.31503452262567,-25.8909527255516,9.2174561272442));
#56124=CARTESIAN_POINT('Ctrl Pts',(4.36119776862006,-25.8868296951047,9.22862951527465));
#56125=CARTESIAN_POINT('Ctrl Pts',(4.51915676195424,-25.8727217240369,9.26686203310144));
#56126=CARTESIAN_POINT('Ctrl Pts',(4.6709530903513,-25.8584777221685,9.30566322163177));
#56127=CARTESIAN_POINT('Ctrl Pts',(4.81658449855443,-25.8442847881759,9.3445420794192));
#56128=CARTESIAN_POINT('Ctrl Pts',(4.86926930130758,-25.8391502369337,9.35860721124118));
#56129=CARTESIAN_POINT('Ctrl Pts',(4.92114738772172,-25.8340221297987,9.37268292895603));
#56130=CARTESIAN_POINT('Ctrl Pts',(4.97221904074658,-25.8289085328382,9.38674739646932));
#56131=CARTESIAN_POINT('Ctrl Pts',(5.00451866423531,-25.8256745028683,9.39564229174571));
#56132=CARTESIAN_POINT('Ctrl Pts',(5.03649568642666,-25.8224465977366,9.40453183293909));
#56133=CARTESIAN_POINT('Ctrl Pts',(5.06815007165425,-25.8192265494893,9.41341124437178));
#56134=CARTESIAN_POINT('Ctrl Pts',(5.21038871658686,-25.8047572967769,9.45331078564873));
#56135=CARTESIAN_POINT('Ctrl Pts',(5.34611257561003,-25.7904491258196,9.49300242145934));
#56136=CARTESIAN_POINT('Ctrl Pts',(5.47532119496024,-25.7764528364258,9.53208334850019));
#56137=CARTESIAN_POINT('Ctrl Pts',(5.60704624399722,-25.7621839593494,9.57192540436887));
#56138=CARTESIAN_POINT('Ctrl Pts',(5.73199999778889,-25.7482390388816,9.61113271254057));
#56139=CARTESIAN_POINT('Ctrl Pts',(5.8501840030794,-25.7347477749795,9.6493230303475));
#56140=CARTESIAN_POINT('Ctrl Pts',(5.86232336330077,-25.7333620095205,9.65324577796201));
#56141=CARTESIAN_POINT('Ctrl Pts',(5.87439129930585,-25.7319810062009,9.65715783398083));
#56142=CARTESIAN_POINT('Ctrl Pts',(5.8863878126649,-25.7306048893156,9.66105881025516));
#56143=CARTESIAN_POINT('Ctrl Pts',(5.92102951904501,-25.7266311483079,9.67232345612738));
#56144=CARTESIAN_POINT('Ctrl Pts',(5.9550756602132,-25.7226981692095,9.68349569974831));
#56145=CARTESIAN_POINT('Ctrl Pts',(5.9885258216116,-25.718808932825,9.6945670296885));
#56146=CARTESIAN_POINT('',(-6.27159361730913,-25.5608563036422,8.76070973783771));
#56147=CARTESIAN_POINT('Origin',(-5.9999949808,-24.7867195890602,9.33250914740362));
#56148=CARTESIAN_POINT('Ctrl Pts',(-6.27159386306998,-25.5608571679688,
8.76070927462923));
#56149=CARTESIAN_POINT('Ctrl Pts',(-6.19708063904679,-25.5689447885619,
8.73626652820671));
#56150=CARTESIAN_POINT('Ctrl Pts',(-6.11543892371899,-25.5777035217229,
8.70997409263041));
#56151=CARTESIAN_POINT('Ctrl Pts',(-6.02658468462762,-25.5870520421337,
8.68208172051963));
#56152=CARTESIAN_POINT('Ctrl Pts',(-5.93855991912608,-25.5963132920793,
8.65444972975093));
#56153=CARTESIAN_POINT('Ctrl Pts',(-5.84345650869302,-25.6061534766376,
8.62524745406809));
#56154=CARTESIAN_POINT('Ctrl Pts',(-5.74118377300316,-25.6164754174791,
8.59476439199516));
#56155=CARTESIAN_POINT('Ctrl Pts',(-5.6404952783399,-25.6266374677882,8.56475352338832));
#56156=CARTESIAN_POINT('Ctrl Pts',(-5.53285768058784,-25.637266563283,8.53350119440277));
#56157=CARTESIAN_POINT('Ctrl Pts',(-5.41817809549367,-25.6482508438218,
8.50132997441968));
#56158=CARTESIAN_POINT('Ctrl Pts',(-5.37925184358973,-25.6519792918353,
8.49040994002917));
#56159=CARTESIAN_POINT('Ctrl Pts',(-5.3395141985331,-25.655748491532,8.47938443645545));
#56160=CARTESIAN_POINT('Ctrl Pts',(-5.29896141203056,-25.6595535226999,
8.46826733717323));
#56161=CARTESIAN_POINT('Ctrl Pts',(-5.21821293618428,-25.6671300789331,
8.4461310328575));
#56162=CARTESIAN_POINT('Ctrl Pts',(-5.13423254664718,-25.6748489226137,
8.42363083556044));
#56163=CARTESIAN_POINT('Ctrl Pts',(-5.04699089785595,-25.6826701550035,
8.40088618117009));
#56164=CARTESIAN_POINT('Ctrl Pts',(-4.92201106411443,-25.6938746237093,
8.36830285470159));
#56165=CARTESIAN_POINT('Ctrl Pts',(-4.79033815562892,-25.705289985841,8.33521556942507));
#56166=CARTESIAN_POINT('Ctrl Pts',(-4.65188625538751,-25.7167847988647,
8.30201758529982));
#56167=CARTESIAN_POINT('Ctrl Pts',(-4.51343435514609,-25.7282796118884,
8.26881960117456));
#56168=CARTESIAN_POINT('Ctrl Pts',(-4.36820326559321,-25.7398539743359,
8.23551064667246));
#56169=CARTESIAN_POINT('Ctrl Pts',(-4.21611007769853,-25.7513585178058,
8.20253712861326));
#56170=CARTESIAN_POINT('Ctrl Pts',(-4.07082689961474,-25.7623479425188,
8.1710400079167));
#56171=CARTESIAN_POINT('Ctrl Pts',(-3.91928181453819,-25.7732734603624,
8.13984920306125));
#56172=CARTESIAN_POINT('Ctrl Pts',(-3.761419633208,-25.7839929667704,8.10939932611515));
#56173=CARTESIAN_POINT('Ctrl Pts',(-3.73054600125373,-25.7860894162986,
8.10344414238486));
#56174=CARTESIAN_POINT('Ctrl Pts',(-3.69943078308636,-25.788177940232,8.09751744688045));
#56175=CARTESIAN_POINT('Ctrl Pts',(-3.66807362121464,-25.7902574078211,
8.09162271016127));
#56176=CARTESIAN_POINT('Ctrl Pts',(-3.58017497496326,-25.7960864553211,
8.0750989131498));
#56177=CARTESIAN_POINT('Ctrl Pts',(-3.49037512908124,-25.801844445895,8.05882589710281));
#56178=CARTESIAN_POINT('Ctrl Pts',(-3.39866710983025,-25.807505523488,8.04288325215432));
#56179=CARTESIAN_POINT('Ctrl Pts',(-3.35281310020476,-25.8103360622845,
8.03491192968008));
#56180=CARTESIAN_POINT('Ctrl Pts',(-3.30648203828449,-25.8131423273748,
8.02702323602364));
#56181=CARTESIAN_POINT('Ctrl Pts',(-3.25967322258879,-25.815920977859,8.01922760763646));
#56182=CARTESIAN_POINT('Ctrl Pts',(-3.23626881474094,-25.8173103031012,
8.01532979344288));
#56183=CARTESIAN_POINT('Ctrl Pts',(-3.21274496785339,-25.8186927217834,
8.01145524786678));
#56184=CARTESIAN_POINT('Ctrl Pts',(-3.18910159820844,-25.8200678035715,
8.00760529749764));
#56185=CARTESIAN_POINT('Ctrl Pts',(-3.17727991338596,-25.8207553444655,
8.00568032231307));
#56186=CARTESIAN_POINT('Ctrl Pts',(-3.16542834783943,-25.8214410509499,
8.00376149607821));
#56187=CARTESIAN_POINT('Ctrl Pts',(-3.15354689173673,-25.8221248687264,
8.00184898647939));
#56188=CARTESIAN_POINT('Ctrl Pts',(-3.14166543563402,-25.8228086865028,
7.99993647688058));
#56189=CARTESIAN_POINT('Ctrl Pts',(-3.12814004787691,-25.8235825258922,
7.99777350945494));
#56190=CARTESIAN_POINT('Ctrl Pts',(-3.11781284205206,-25.8241706010689,
7.99613057617227));
#56191=CARTESIAN_POINT('Ctrl Pts',(-3.0766201969457,-25.8265162860935,7.98957732558404));
#56192=CARTESIAN_POINT('Ctrl Pts',(-3.03568681538845,-25.8288017557171,
7.98319650478659));
#56193=CARTESIAN_POINT('Ctrl Pts',(-2.99501443262273,-25.831028571739,7.97698351883132));
#56194=CARTESIAN_POINT('Ctrl Pts',(-2.79739857890957,-25.8418480546241,
7.94679633922273));
#56195=CARTESIAN_POINT('Ctrl Pts',(-2.60594810869286,-25.8512836540238,
7.92056972156591));
#56196=CARTESIAN_POINT('Ctrl Pts',(-2.42085607247106,-25.8595191508833,
7.89776586357605));
#56197=CARTESIAN_POINT('Ctrl Pts',(-2.23092812240802,-25.8679698172016,
7.87436620743766));
#56198=CARTESIAN_POINT('Ctrl Pts',(-2.04769488441589,-25.8751569357714,
7.85457014091518));
#56199=CARTESIAN_POINT('Ctrl Pts',(-1.87131612638337,-25.8812684573676,
7.83781972802053));
#56200=CARTESIAN_POINT('Ctrl Pts',(-1.78117029277795,-25.8843920092909,
7.82925872016184));
#56201=CARTESIAN_POINT('Ctrl Pts',(-1.69281421002091,-25.8872344221247,
7.82149368573478));
#56202=CARTESIAN_POINT('Ctrl Pts',(-1.60626489564927,-25.8898196497827,
7.81445284170412));
#56203=CARTESIAN_POINT('Ctrl Pts',(-1.43907111686404,-25.8948137272552,
7.80085151709666));
#56204=CARTESIAN_POINT('Ctrl Pts',(-1.27862185686045,-25.8988490684406,
7.78995019290348));
#56205=CARTESIAN_POINT('Ctrl Pts',(-1.12501667405839,-25.9020959959412,
7.78123961020363));
#56206=CARTESIAN_POINT('Ctrl Pts',(-0.969939764400389,-25.9053740330067,
7.77244556939216));
#56207=CARTESIAN_POINT('Ctrl Pts',(-0.821838316641244,-25.9078484881115,
7.76588428017098));
#56208=CARTESIAN_POINT('Ctrl Pts',(-0.680782402076676,-25.9096791063164,
7.76107122809345));
#56209=CARTESIAN_POINT('Ctrl Pts',(-0.538388127957247,-25.9115270936998,
7.75621250905998));
#56210=CARTESIAN_POINT('Ctrl Pts',(-0.403173335643225,-25.9127189872834,
7.75313518406329));
#56211=CARTESIAN_POINT('Ctrl Pts',(-0.275183173989101,-25.9134031475166,
7.75138353240064));
#56212=CARTESIAN_POINT('Ctrl Pts',(-0.236228034117317,-25.9136113788153,
7.75085039895786));
#56213=CARTESIAN_POINT('Ctrl Pts',(-0.1979419845857,-25.9137724639869,7.75044037647808));
#56214=CARTESIAN_POINT('Ctrl Pts',(-0.160325891522733,-25.9138902918349,
7.75014142876869));
#56215=CARTESIAN_POINT('Ctrl Pts',(-0.154008553609919,-25.9139100801296,
7.75009122276523));
#56216=CARTESIAN_POINT('Ctrl Pts',(-0.147710111200664,-25.9139286480524,
7.75004415046106));
#56217=CARTESIAN_POINT('Ctrl Pts',(-0.141430567613903,-25.913946013496,
7.75000015435446));
#56218=CARTESIAN_POINT('Ctrl Pts',(-0.103047981675466,-25.9140521566614,
7.74973123602959));
#56219=CARTESIAN_POINT('Ctrl Pts',(-0.0662560356263134,-25.914112617826,
7.74957970423149));
#56220=CARTESIAN_POINT('Ctrl Pts',(-0.0289815746365708,-25.9141334372774,
7.74952611540055));
#56221=CARTESIAN_POINT('Ctrl Pts',(-0.0185593623277894,-25.9141392585485,
7.74951113157091));
#56222=CARTESIAN_POINT('Ctrl Pts',(-0.00809942559603181,-25.9141418866517,
7.7495041020777));
#56223=CARTESIAN_POINT('Ctrl Pts',(0.00244355485639335,-25.9141412348339,
7.74950529306156));
#56224=CARTESIAN_POINT('Ctrl Pts',(0.127127988062576,-25.9141335262425,
7.74951937799214));
#56225=CARTESIAN_POINT('Ctrl Pts',(0.258986421343677,-25.9136690002263,
7.75068426010729));
#56226=CARTESIAN_POINT('Ctrl Pts',(0.397985636277575,-25.9126040409567,
7.75344426793973));
#56227=CARTESIAN_POINT('Ctrl Pts',(0.535666715031177,-25.9115491807465,
7.75617810248635));
#56228=CARTESIAN_POINT('Ctrl Pts',(0.680354109440456,-25.9099051999983,
7.7604770911692));
#56229=CARTESIAN_POINT('Ctrl Pts',(0.831993583507304,-25.9075172201685,
7.76681628057526));
#56230=CARTESIAN_POINT('Ctrl Pts',(0.942261577046938,-25.9057807478808,
7.77142596219527));
#56231=CARTESIAN_POINT('Ctrl Pts',(1.05620525649912,-25.9036505489341,7.77711535741795));
#56232=CARTESIAN_POINT('Ctrl Pts',(1.17379482852109,-25.9010619875873,7.78408109758496));
#56233=CARTESIAN_POINT('Ctrl Pts',(1.33435500102349,-25.8975274917197,7.79359231889132));
#56234=CARTESIAN_POINT('Ctrl Pts',(1.50171435131308,-25.8931388014668,7.80548239116508));
#56235=CARTESIAN_POINT('Ctrl Pts',(1.67576186882429,-25.8877241846894,7.82026642896838));
#56236=CARTESIAN_POINT('Ctrl Pts',(1.84377414670226,-25.8824973241652,7.83453781820211));
#56237=CARTESIAN_POINT('Ctrl Pts',(2.01801902803007,-25.8763143723798,7.85150627903865));
#56238=CARTESIAN_POINT('Ctrl Pts',(2.19835996516099,-25.8690099414244,7.87166085380236));
#56239=CARTESIAN_POINT('Ctrl Pts',(2.26108100385463,-25.8664695226827,7.87867044288246));
#56240=CARTESIAN_POINT('Ctrl Pts',(2.32453906477803,-25.863793357096,7.88606563249174));
#56241=CARTESIAN_POINT('Ctrl Pts',(2.38872722789465,-25.860974186408,7.89386765098496));
#56242=CARTESIAN_POINT('Ctrl Pts',(2.47499317077123,-25.8571853504963,7.90435320547007));
#56243=CARTESIAN_POINT('Ctrl Pts',(2.56257788935075,-25.8531382212515,7.91557357215087));
#56244=CARTESIAN_POINT('Ctrl Pts',(2.65146471499337,-25.8488156602481,7.92757932298422));
#56245=CARTESIAN_POINT('Ctrl Pts',(2.72897727348801,-25.8450462291744,7.93804877621325));
#56246=CARTESIAN_POINT('Ctrl Pts',(2.80748002606418,-25.8410673718969,7.94911553139678));
#56247=CARTESIAN_POINT('Ctrl Pts',(2.88696068428701,-25.8368674907817,7.96081345907223));
#56248=CARTESIAN_POINT('Ctrl Pts',(2.92670101339843,-25.8347675502241,7.96666242290996));
#56249=CARTESIAN_POINT('Ctrl Pts',(2.96668581773295,-25.8326123476695,7.97266918466076));
#56250=CARTESIAN_POINT('Ctrl Pts',(3.00691344022713,-25.8304004283776,7.97883801999785));
#56251=CARTESIAN_POINT('Ctrl Pts',(3.02702725147422,-25.8292944687317,7.98192243766639));
#56252=CARTESIAN_POINT('Ctrl Pts',(3.04720176720655,-25.8281743295397,7.98504737402185));
#56253=CARTESIAN_POINT('Ctrl Pts',(3.06743677570191,-25.8270398270069,7.98821336459234));
#56254=CARTESIAN_POINT('Ctrl Pts',(3.07755427994959,-25.8264725757405,7.98979635987758));
#56255=CARTESIAN_POINT('Ctrl Pts',(3.0876869073839,-25.8259017336162,7.99138961873463));
#56256=CARTESIAN_POINT('Ctrl Pts',(3.0978346310618,-25.8253272776051,7.99299320821095));
#56257=CARTESIAN_POINT('Ctrl Pts',(3.10798235473969,-25.824752821594,7.99459679768727));
#56258=CARTESIAN_POINT('Ctrl Pts',(3.11649244049615,-25.8242692120269,7.99594695329885));
#56259=CARTESIAN_POINT('Ctrl Pts',(3.12832306372715,-25.8235930448162,7.99783503561468));
#56260=CARTESIAN_POINT('Ctrl Pts',(3.2439668548878,-25.8169835418194,8.01629095232871));
#56261=CARTESIAN_POINT('Ctrl Pts',(3.35681912047297,-25.8101925839103,8.03535399059616));
#56262=CARTESIAN_POINT('Ctrl Pts',(3.4668879598088,-25.8032672596649,8.05487798524582));
#56263=CARTESIAN_POINT('Ctrl Pts',(3.63912660834516,-25.7924303280147,8.08542965157373));
#56264=CARTESIAN_POINT('Ctrl Pts',(3.80454906828157,-25.7812653381788,8.11710708630667));
#56265=CARTESIAN_POINT('Ctrl Pts',(3.96321157962074,-25.7699424992933,8.1493898816964));
#56266=CARTESIAN_POINT('Ctrl Pts',(4.12187409095991,-25.7586196604077,8.18167267708613));
#56267=CARTESIAN_POINT('Ctrl Pts',(4.27377692490459,-25.7471388839885,8.21456112151753));
#56268=CARTESIAN_POINT('Ctrl Pts',(4.41898858671655,-25.7356525460951,8.24759161726221));
#56269=CARTESIAN_POINT('Ctrl Pts',(4.5635182889215,-25.7242201516549,8.28046699141669));
#56270=CARTESIAN_POINT('Ctrl Pts',(4.70142003179067,-25.7127823131508,8.31348335264749));
#56271=CARTESIAN_POINT('Ctrl Pts',(4.83277463773686,-25.7014759066788,8.34623482767659));
#56272=CARTESIAN_POINT('Ctrl Pts',(4.90532346773847,-25.6952312336797,8.36432388650382));
#56273=CARTESIAN_POINT('Ctrl Pts',(4.97587516450272,-25.6890263399827,8.38233303919329));
#56274=CARTESIAN_POINT('Ctrl Pts',(5.04444364874705,-25.6828820642494,8.40020028894091));
#56275=CARTESIAN_POINT('Ctrl Pts',(5.1353882843271,-25.6747327092852,8.42389820985928));
#56276=CARTESIAN_POINT('Ctrl Pts',(5.22284415433159,-25.6666901439998,8.44734605381939));
#56277=CARTESIAN_POINT('Ctrl Pts',(5.30684382899499,-25.658798954923,8.47041084629138));
#56278=CARTESIAN_POINT('Ctrl Pts',(5.42689862195449,-25.6475206365889,8.50337572259565));
#56279=CARTESIAN_POINT('Ctrl Pts',(5.53989390952036,-25.6365524409084,8.53555627122668));
#56280=CARTESIAN_POINT('Ctrl Pts',(5.64592673883416,-25.6260119626618,8.566611887455));
#56281=CARTESIAN_POINT('Ctrl Pts',(5.75378604299005,-25.6152899187768,8.59820245405778));
#56282=CARTESIAN_POINT('Ctrl Pts',(5.85444110836096,-25.6050103706137,8.62862905272502));
#56283=CARTESIAN_POINT('Ctrl Pts',(5.94798673536669,-25.5952771856988,8.65758325353552));
#56284=CARTESIAN_POINT('Ctrl Pts',(6.02496391510624,-25.5872679056435,8.68140919592692));
#56285=CARTESIAN_POINT('Ctrl Pts',(6.09712691820323,-25.5796281937042,8.70423908336207));
#56286=CARTESIAN_POINT('Ctrl Pts',(6.16452391351832,-25.5724066904849,8.72592536702089));
#56287=CARTESIAN_POINT('Ctrl Pts',(6.20165874450665,-25.5684277400839,8.73787421540308));
#56288=CARTESIAN_POINT('Ctrl Pts',(6.23734659792339,-25.5645756329308,8.7494762901245));
#56289=CARTESIAN_POINT('Ctrl Pts',(6.27159479316358,-25.5608580129633,8.76071029005059));
#56290=CARTESIAN_POINT('Ctrl Pts',(-6.390311350308,-25.6807372937616,8.98426028603872));
#56291=CARTESIAN_POINT('Ctrl Pts',(-4.260207566872,-25.9287992192441,8.2768729736642));
#56292=CARTESIAN_POINT('Ctrl Pts',(0.0001663377217942,-26.1774671700566,
7.5688746106888));
#56293=CARTESIAN_POINT('Ctrl Pts',(4.260540242316,-25.9287798010101,8.27692826056537));
#56294=CARTESIAN_POINT('Ctrl Pts',(6.390810363473,-25.680679178753,8.98442601004882));
#56295=CARTESIAN_POINT('Ctrl Pts',(-6.390311350308,-25.114983911886,8.18394866803594));
#56296=CARTESIAN_POINT('Ctrl Pts',(-4.260207566872,-25.3660579697472,7.53598941987455));
#56297=CARTESIAN_POINT('Ctrl Pts',(0.0001663377217942,-25.6190368856695,
6.88615611385154));
#56298=CARTESIAN_POINT('Ctrl Pts',(4.260540242316,-25.3660382148685,7.53604016472075));
#56299=CARTESIAN_POINT('Ctrl Pts',(6.390810363473,-25.114925091227,8.18410046945239));
#56300=CARTESIAN_POINT('Ctrl Pts',(-6.390311350308,-23.7052292153387,6.63374483955243));
#56301=CARTESIAN_POINT('Ctrl Pts',(-4.260207566872,-23.9981327197181,6.09525946370173));
#56302=CARTESIAN_POINT('Ctrl Pts',(0.0001663377217942,-24.290056533388,
5.55782023498321));
#56303=CARTESIAN_POINT('Ctrl Pts',(4.260540242316,-23.9981099236694,6.09530143180341));
#56304=CARTESIAN_POINT('Ctrl Pts',(6.390810363473,-23.7051605950053,6.63387099387303));
#56305=CARTESIAN_POINT('Ctrl Pts',(-6.390311350308,-21.0044950488243,4.89945807532427));
#56306=CARTESIAN_POINT('Ctrl Pts',(-4.260207566872,-21.4424839271908,4.44478852897079));
#56307=CARTESIAN_POINT('Ctrl Pts',(0.0001663377217941,-21.8807691943046,
3.98943207393405));
#56308=CARTESIAN_POINT('Ctrl Pts',(4.260540242316,-21.4424497019158,4.44482408731423));
#56309=CARTESIAN_POINT('Ctrl Pts',(6.390810363473,-21.0043924384536,4.89956459357196));
#56310=CARTESIAN_POINT('Ctrl Pts',(-6.390311350308,-18.1257304172683,4.0264979364763));
#56311=CARTESIAN_POINT('Ctrl Pts',(-4.260207566872,-18.7393860755884,3.53810643694032));
#56312=CARTESIAN_POINT('Ctrl Pts',(0.0001663377217945,-19.353021691043,
3.05102696824815));
#56313=CARTESIAN_POINT('Ctrl Pts',(4.260540242316,-18.7393381573803,3.53814447249922));
#56314=CARTESIAN_POINT('Ctrl Pts',(6.390810363473,-18.1255866523452,4.02661235499138));
#56315=CARTESIAN_POINT('Ctrl Pts',(-6.390311350308,-16.240127474348,3.91822579691448));
#56316=CARTESIAN_POINT('Ctrl Pts',(-4.260207566872,-16.9589011884504,3.34432563173864));
#56317=CARTESIAN_POINT('Ctrl Pts',(0.0001663377217938,-17.6776846679344,
2.76847602232095));
#56318=CARTESIAN_POINT('Ctrl Pts',(4.260540242316,-16.9588450593473,3.34437059927322));
#56319=CARTESIAN_POINT('Ctrl Pts',(6.390810363473,-16.2399590827655,3.91836024805384));
#56320=CARTESIAN_POINT('Ctrl Pts',(-6.390311350308,-15.4599864582096,3.94962394700618));
#56321=CARTESIAN_POINT('Ctrl Pts',(-4.260207566872,-16.2180942529318,3.32898458305284));
#56322=CARTESIAN_POINT('Ctrl Pts',(0.0001663377217938,-16.9762230425391,
2.70679298590865));
#56323=CARTESIAN_POINT('Ctrl Pts',(4.260540242316,-16.2180350513886,3.32903316938923));
#56324=CARTESIAN_POINT('Ctrl Pts',(6.390810363473,-15.4598088515932,3.94976934802855));
#56325=CARTESIAN_POINT('',(-6.26385951335491,-15.8144217941401,3.90574150361402));
#56326=CARTESIAN_POINT('Ctrl Pts',(-6.27159552384235,-25.5608567088111,
8.76070944182656));
#56327=CARTESIAN_POINT('Ctrl Pts',(-6.27195777355281,-25.4158727838719,
8.5645940892268));
#56328=CARTESIAN_POINT('Ctrl Pts',(-6.27229031319814,-25.2662940547189,
8.37478239185605));
#56329=CARTESIAN_POINT('Ctrl Pts',(-6.2725931430244,-25.1127469377871,8.19135374058517));
#56330=CARTESIAN_POINT('Ctrl Pts',(-6.27289863568736,-24.957849653655,8.00631216845018));
#56331=CARTESIAN_POINT('Ctrl Pts',(-6.27317389374662,-24.7989138390075,
7.82776631099681));
#56332=CARTESIAN_POINT('Ctrl Pts',(-6.27341891745478,-24.6365421570524,
7.65576240833124));
#56333=CARTESIAN_POINT('Ctrl Pts',(-6.27366754260897,-24.4717838780882,
7.48123033083415));
#56334=CARTESIAN_POINT('Ctrl Pts',(-6.2738850380896,-24.3034879748336,7.31343388118491));
#56335=CARTESIAN_POINT('Ctrl Pts',(-6.27407140416057,-24.1322430218785,
7.15238617213097));
#56336=CARTESIAN_POINT('Ctrl Pts',(-6.27421804473799,-23.9975003691542,
7.02566713511055));
#56337=CARTESIAN_POINT('Ctrl Pts',(-6.27434541248456,-23.8609310705886,
6.90312565692038));
#56338=CARTESIAN_POINT('Ctrl Pts',(-6.27445350752884,-23.7228045339352,
6.78475354198177));
#56339=CARTESIAN_POINT('Ctrl Pts',(-6.27450262987442,-23.660034778736,6.73096091923787));
#56340=CARTESIAN_POINT('Ctrl Pts',(-6.2745477721635,-23.5969432430862,6.67802913642794));
#56341=CARTESIAN_POINT('Ctrl Pts',(-6.27458893440815,-23.5335576663087,
6.62595263407767));
#56342=CARTESIAN_POINT('Ctrl Pts',(-6.27470712620839,-23.3515545833113,
6.4764220237821));
#56343=CARTESIAN_POINT('Ctrl Pts',(-6.27479250322405,-23.1671310106694,
6.33394454568465));
#56344=CARTESIAN_POINT('Ctrl Pts',(-6.27484506545512,-22.9809083449876,
6.19837392603431));
#56345=CARTESIAN_POINT('Ctrl Pts',(-6.2748976276862,-22.7946856793058,6.06280330638397));
#56346=CARTESIAN_POINT('Ctrl Pts',(-6.2749173751327,-22.6066637586169,5.93413943825559));
#56347=CARTESIAN_POINT('Ctrl Pts',(-6.27490430779461,-22.4174135710649,
5.81221558765903));
#56348=CARTESIAN_POINT('Ctrl Pts',(-6.27489476769251,-22.2792472437393,
5.72320235671738));
#56349=CARTESIAN_POINT('Ctrl Pts',(-6.27486753880225,-22.1401747709447,
5.637625073071));
#56350=CARTESIAN_POINT('Ctrl Pts',(-6.27482283830957,-22.0006690425674,
5.55559585379084));
#56351=CARTESIAN_POINT('Ctrl Pts',(-6.27477792092454,-21.8604864150119,
5.47316861851682));
#56352=CARTESIAN_POINT('Ctrl Pts',(-6.27471536197696,-21.7198666589869,
5.3943240411735));
#56353=CARTESIAN_POINT('Ctrl Pts',(-6.2746353818294,-21.5793028330079,5.31912480394626));
#56354=CARTESIAN_POINT('Ctrl Pts',(-6.27457691192168,-21.476542908408,5.26415000588831));
#56355=CARTESIAN_POINT('Ctrl Pts',(-6.27450913139656,-21.373813168866,5.21112236044329));
#56356=CARTESIAN_POINT('Ctrl Pts',(-6.2744321263511,-21.2713091288939,5.16004897734718));
#56357=CARTESIAN_POINT('Ctrl Pts',(-6.27435635466394,-21.170446854181,5.10979361572676));
#56358=CARTESIAN_POINT('Ctrl Pts',(-6.2742702475298,-21.0681861058318,5.06062331003959));
#56359=CARTESIAN_POINT('Ctrl Pts',(-6.27417380494869,-20.9645377933661,
5.01262251508626));
#56360=CARTESIAN_POINT('Ctrl Pts',(-6.27399075533888,-20.7678115865775,
4.9215162144687));
#56361=CARTESIAN_POINT('Ctrl Pts',(-6.27377047262635,-20.5660839039866,
4.83462179089819));
#56362=CARTESIAN_POINT('Ctrl Pts',(-6.27351295681112,-20.3594970637805,
4.75246067873237));
#56363=CARTESIAN_POINT('Ctrl Pts',(-6.27325823314554,-20.1551501690056,
4.67119040940841));
#56364=CARTESIAN_POINT('Ctrl Pts',(-6.27296707940982,-19.9460488030888,
4.59455135335413));
#56365=CARTESIAN_POINT('Ctrl Pts',(-6.27263949560396,-19.7323748765706,
4.52307277276017));
#56366=CARTESIAN_POINT('Ctrl Pts',(-6.27231699897039,-19.5220191729321,
4.45270420996481));
#56367=CARTESIAN_POINT('Ctrl Pts',(-6.2719591949537,-19.3072317554042,4.38733709853277));
#56368=CARTESIAN_POINT('Ctrl Pts',(-6.2715660835539,-19.0882305285998,4.32750038765547));
#56369=CARTESIAN_POINT('Ctrl Pts',(-6.2713627519632,-18.9749550859819,4.29655065276892));
#56370=CARTESIAN_POINT('Ctrl Pts',(-6.27114997445887,-18.8605530428152,
4.26708087937792));
#56371=CARTESIAN_POINT('Ctrl Pts',(-6.27092775104091,-18.7450594169863,
4.23916682997619));
#56372=CARTESIAN_POINT('Ctrl Pts',(-6.27050608312226,-18.5259107904982,
4.18620004897671));
#56373=CARTESIAN_POINT('Ctrl Pts',(-6.27005040597021,-18.3028291636747,
4.13883321537287));
#56374=CARTESIAN_POINT('Ctrl Pts',(-6.26956071910113,-18.0760881657024,
4.0976017108142));
#56375=CARTESIAN_POINT('Ctrl Pts',(-6.26938505239444,-17.9947487488252,
4.08281062068157));
#56376=CARTESIAN_POINT('Ctrl Pts',(-6.26920500900548,-17.912938840527,4.06880930124582));
#56377=CARTESIAN_POINT('Ctrl Pts',(-6.26902058891192,-17.8306725394492,
4.05562321457882));
#56378=CARTESIAN_POINT('Ctrl Pts',(-6.26850854183986,-17.6022580658327,
4.01901171016394));
#56379=CARTESIAN_POINT('Ctrl Pts',(-6.26796275434394,-17.3703215097504,
3.98868445467322));
#56380=CARTESIAN_POINT('Ctrl Pts',(-6.26738322594624,-17.135214507519,3.96507788638757));
#56381=CARTESIAN_POINT('Ctrl Pts',(-6.26681231403247,-16.903603098796,3.94182230282831));
#56382=CARTESIAN_POINT('Ctrl Pts',(-6.26620865708409,-16.6689147740032,
3.92508906956263));
#56383=CARTESIAN_POINT('Ctrl Pts',(-6.26557225464421,-16.4315352528344,
3.91530352157058));
#56384=CARTESIAN_POINT('Ctrl Pts',(-6.26502584282964,-16.2277224344459,
3.90690170111903));
#56385=CARTESIAN_POINT('Ctrl Pts',(-6.26445529152988,-16.0219264392837,
3.90362174117236));
#56386=CARTESIAN_POINT('Ctrl Pts',(-6.26386060045574,-15.8144217505232,
3.90573752921543));
#56387=CARTESIAN_POINT('Ctrl Pts',(6.2638598901157,-15.8144313886664,3.90573722905719));
#56388=CARTESIAN_POINT('Ctrl Pts',(5.97578930821615,-15.9102534412013,3.8258770779521));
#56389=CARTESIAN_POINT('Ctrl Pts',(5.68589879838239,-15.9988220577541,3.75096628482656));
#56390=CARTESIAN_POINT('Ctrl Pts',(5.39467502935807,-16.0802283700764,3.68127561885453));
#56391=CARTESIAN_POINT('Ctrl Pts',(5.12105868788167,-16.1567128460013,3.61579845975379));
#56392=CARTESIAN_POINT('Ctrl Pts',(4.84626543163589,-16.2268745751674,3.55492987257316));
#56393=CARTESIAN_POINT('Ctrl Pts',(4.57069888658429,-16.2908266780865,3.49887279692821));
#56394=CARTESIAN_POINT('Ctrl Pts',(4.31440697190754,-16.3503056213728,3.44673665955517));
#56395=CARTESIAN_POINT('Ctrl Pts',(4.05744616130298,-16.4044131426885,3.39876274702718));
#56396=CARTESIAN_POINT('Ctrl Pts',(3.80014117125608,-16.4532764068686,3.35508947292147));
#56397=CARTESIAN_POINT('Ctrl Pts',(3.57897012726198,-16.4952776877209,3.31754933960792));
#56398=CARTESIAN_POINT('Ctrl Pts',(3.35754478403803,-16.5334046032886,3.28318655458352));
#56399=CARTESIAN_POINT('Ctrl Pts',(3.1360713681052,-16.5677626949941,3.25207046795645));
#56400=CARTESIAN_POINT('Ctrl Pts',(2.89295359977274,-16.6054785650656,3.21791344054009));
#56401=CARTESIAN_POINT('Ctrl Pts',(2.64979796567082,-16.6386697226143,3.18767332756024));
#56402=CARTESIAN_POINT('Ctrl Pts',(2.40684647802523,-16.6673707732513,3.16139952179199));
#56403=CARTESIAN_POINT('Ctrl Pts',(2.16745577474301,-16.6956511709698,3.13551079436861));
#56404=CARTESIAN_POINT('Ctrl Pts',(1.92826327768186,-16.719572102414,3.1134730048344));
#56405=CARTESIAN_POINT('Ctrl Pts',(1.68950051321017,-16.7392056546265,3.09530109367423));
#56406=CARTESIAN_POINT('Ctrl Pts',(1.45234022335468,-16.7587074347468,3.0772511446903));
#56407=CARTESIAN_POINT('Ctrl Pts',(1.21560391707957,-16.7739791516685,3.06301541739025));
#56408=CARTESIAN_POINT('Ctrl Pts',(0.979518490249757,-16.7851306663667,
3.05257560488626));
#56409=CARTESIAN_POINT('Ctrl Pts',(0.745119696576639,-16.796202512808,3.04221037612153));
#56410=CARTESIAN_POINT('Ctrl Pts',(0.511362515589295,-16.8032128024522,
3.03558705246871));
#56411=CARTESIAN_POINT('Ctrl Pts',(0.278469014867348,-16.8063082581637,
3.03265442154118));
#56412=CARTESIAN_POINT('Ctrl Pts',(0.185645823208615,-16.8075419983836,
3.03148557757684));
#56413=CARTESIAN_POINT('Ctrl Pts',(0.0929598306468264,-16.8081542912968,
3.03090263974755));
#56414=CARTESIAN_POINT('Ctrl Pts',(0.000425097092084769,-16.8081561849884,
3.03090086182255));
#56415=CARTESIAN_POINT('Ctrl Pts',(0.000283398425769262,-16.8081561878882,
3.0309008591));
#56416=CARTESIAN_POINT('Ctrl Pts',(0.000141699394583094,-16.808156189357,
3.03090085774004));
#56417=CARTESIAN_POINT('Ctrl Pts',(-1.42137912181577E-12,-16.8081561893948,
3.03090085774268));
#56418=CARTESIAN_POINT('Ctrl Pts',(-0.229739891951006,-16.8081562505921,
3.03090086201527));
#56419=CARTESIAN_POINT('Ctrl Pts',(-0.46043877177314,-16.8043912206802,
3.03448552365188));
#56420=CARTESIAN_POINT('Ctrl Pts',(-0.691871120056919,-16.7967011224477,
3.04171955588636));
#56421=CARTESIAN_POINT('Ctrl Pts',(-0.925120551421554,-16.7889506456748,
3.04901038587482));
#56422=CARTESIAN_POINT('Ctrl Pts',(-1.15911501406741,-16.7772132199962,
3.0600081021688));
#56423=CARTESIAN_POINT('Ctrl Pts',(-1.39362363479407,-16.76136551204,3.07474453732183));
#56424=CARTESIAN_POINT('Ctrl Pts',(-1.629597578966,-16.7454187799286,3.08957305285921));
#56425=CARTESIAN_POINT('Ctrl Pts',(-1.86609212671074,-16.7253102698,3.10818710540346));
#56426=CARTESIAN_POINT('Ctrl Pts',(-2.10287204990648,-16.7009548892184,
3.13058492596091));
#56427=CARTESIAN_POINT('Ctrl Pts',(-2.34248173396402,-16.6763084370722,
3.15325042325018));
#56428=CARTESIAN_POINT('Ctrl Pts',(-2.58238365528549,-16.6473130159242,
3.17979062465384));
#56429=CARTESIAN_POINT('Ctrl Pts',(-2.82233405091119,-16.613921555402,3.21016945217466));
#56430=CARTESIAN_POINT('Ctrl Pts',(-2.92685480744949,-16.5993764628357,
3.22340226234338));
#56431=CARTESIAN_POINT('Ctrl Pts',(-3.03138476157114,-16.5839977804036,
3.23736298770903));
#56432=CARTESIAN_POINT('Ctrl Pts',(-3.1359037662506,-16.567783992341,3.25204669131969));
#56433=CARTESIAN_POINT('Ctrl Pts',(-3.3986955157854,-16.5270177245736,3.28896587337018));
#56434=CARTESIAN_POINT('Ctrl Pts',(-3.66141401515956,-16.4809448942829,
3.33045628489074));
#56435=CARTESIAN_POINT('Ctrl Pts',(-3.92371507449025,-16.4293937238543,
3.37639868267872));
#56436=CARTESIAN_POINT('Ctrl Pts',(-4.19322219386227,-16.3764263150382,
3.4236032319721));
#56437=CARTESIAN_POINT('Ctrl Pts',(-4.46228862190867,-16.3176757932309,
3.47550729074249));
#56438=CARTESIAN_POINT('Ctrl Pts',(-4.73054101504463,-16.2530046079271,
3.53194531634852));
#56439=CARTESIAN_POINT('Ctrl Pts',(-5.02397088259713,-16.1822635527727,
3.59368046877308));
#56440=CARTESIAN_POINT('Ctrl Pts',(-5.31642673781812,-16.1044383297438,
3.66084025775089));
#56441=CARTESIAN_POINT('Ctrl Pts',(-5.60741993866506,-16.0194038470247,
3.73317123771322));
#56442=CARTESIAN_POINT('Ctrl Pts',(-5.82713749210776,-15.9551976441069,
3.78778552392052));
#56443=CARTESIAN_POINT('Ctrl Pts',(-6.0460211617445,-15.8868825856208,3.84534709603784));
#56444=CARTESIAN_POINT('Ctrl Pts',(-6.26386060045575,-15.8144217505232,
3.90573752921543));
#56445=CARTESIAN_POINT('Ctrl Pts',(6.38290978637461,-15.7742583800757,3.93905205217285));
#56446=CARTESIAN_POINT('Ctrl Pts',(6.3333020539761,-15.7921071431687,3.92502738225168));
#56447=CARTESIAN_POINT('Ctrl Pts',(5.70273749003655,-16.0157853682326,3.74884667445043));
#56448=CARTESIAN_POINT('Ctrl Pts',(4.37427082963316,-16.4041108648871,3.43234872788488));
#56449=CARTESIAN_POINT('Ctrl Pts',(2.28459432793093,-16.7764308999776,3.1131849942996));
#56450=CARTESIAN_POINT('Ctrl Pts',(0.00159936025366462,-16.9132852594445,
2.99188131777531));
#56451=CARTESIAN_POINT('Ctrl Pts',(-2.28164217664832,-16.7767952240661,
3.11286535847525));
#56452=CARTESIAN_POINT('Ctrl Pts',(-4.37189098414695,-16.4046868752343,
3.43186693184216));
#56453=CARTESIAN_POINT('Ctrl Pts',(-5.70139586193533,-16.0162274050497,
3.74849394120053));
#56454=CARTESIAN_POINT('Ctrl Pts',(-6.33273158044223,-15.7923124119726,
3.92486608374166));
#56455=CARTESIAN_POINT('Ctrl Pts',(-6.38291250185657,-15.7742574063264,
3.93905280639695));
#56456=CARTESIAN_POINT('Ctrl Pts',(6.17912845842874,-15.1595937752886,3.89098583450951));
#56457=CARTESIAN_POINT('Ctrl Pts',(6.13107889153985,-15.1768762735422,3.87759665383682));
#56458=CARTESIAN_POINT('Ctrl Pts',(5.52032715675414,-15.393459716353,3.70939428322624));
#56459=CARTESIAN_POINT('Ctrl Pts',(4.23379427768671,-15.7694977771825,3.40711733970962));
#56460=CARTESIAN_POINT('Ctrl Pts',(2.21086559757556,-16.1300032036696,3.10222422277282));
#56461=CARTESIAN_POINT('Ctrl Pts',(0.00154762091081913,-16.2624919144746,
2.98634703116607));
#56462=CARTESIAN_POINT('Ctrl Pts',(-2.20800828847039,-16.1303559293748,
3.10191887675622));
#56463=CARTESIAN_POINT('Ctrl Pts',(-4.23148992251726,-15.7700555537294,
3.40665711311912));
#56464=CARTESIAN_POINT('Ctrl Pts',(-5.51902775455387,-15.3938877517215,
3.7090574686422));
#56465=CARTESIAN_POINT('Ctrl Pts',(-6.13052633629179,-15.1770750297593,
3.87744266458973));
#56466=CARTESIAN_POINT('Ctrl Pts',(-6.17913108867696,-15.1595928319861,
3.89098655522151));
#56467=CARTESIAN_POINT('Ctrl Pts',(6.17606315768169,-14.7496965076852,3.38896273183938));
#56468=CARTESIAN_POINT('Ctrl Pts',(6.12814754427055,-14.7667722774024,3.37574158733111));
#56469=CARTESIAN_POINT('Ctrl Pts',(5.51906854398708,-14.9807801088444,3.20963583670899));
#56470=CARTESIAN_POINT('Ctrl Pts',(4.23523288067283,-15.3527406605511,2.91075424990737));
#56471=CARTESIAN_POINT('Ctrl Pts',(2.21316745047304,-15.7100780789674,2.60855283602971));
#56472=CARTESIAN_POINT('Ctrl Pts',(0.00154976796005158,-15.8416245753242,
2.49347245636735));
#56473=CARTESIAN_POINT('Ctrl Pts',(-2.21030901582472,-15.7104281020419,
2.60824978737707));
#56474=CARTESIAN_POINT('Ctrl Pts',(-4.23293177008851,-15.3532929275836,
2.91029867561449));
#56475=CARTESIAN_POINT('Ctrl Pts',(-5.51777239596502,-14.9812032134454,
3.20930307427043));
#56476=CARTESIAN_POINT('Ctrl Pts',(-6.12759653002278,-14.766968655442,3.37558952923473));
#56477=CARTESIAN_POINT('Ctrl Pts',(-6.17606578034696,-14.749695575192,3.38896344151997));
#56478=CARTESIAN_POINT('Ctrl Pts',(6.37402533240034,-14.8205647331695,2.77721315208895));
#56479=CARTESIAN_POINT('Ctrl Pts',(6.32474120702746,-14.8379302534618,2.7635828203485));
#56480=CARTESIAN_POINT('Ctrl Pts',(5.69822078925919,-15.0555874524055,2.59232277986186));
#56481=CARTESIAN_POINT('Ctrl Pts',(4.3763630139826,-15.4343716381957,2.28380501669291));
#56482=CARTESIAN_POINT('Ctrl Pts',(2.28927089645763,-15.7992586270626,1.97099402057018));
#56483=CARTESIAN_POINT('Ctrl Pts',(0.00160387216188493,-15.9338947894004,
1.85158149042877));
#56484=CARTESIAN_POINT('Ctrl Pts',(-2.28631697573182,-15.7996165966553,
1.97067982535358));
#56485=CARTESIAN_POINT('Ctrl Pts',(-4.37399133895244,-15.4349347419952,
2.28333417339121));
#56486=CARTESIAN_POINT('Ctrl Pts',(-5.69688706113254,-15.0560179588341,
2.59197956119757));
#56487=CARTESIAN_POINT('Ctrl Pts',(-6.32417445620707,-14.8381299631328,
2.76342605380414));
#56488=CARTESIAN_POINT('Ctrl Pts',(-6.37402802959059,-14.8205637846944,
2.77721388049884));
#56489=CARTESIAN_POINT('',(-6.24994617571413,-14.8593872446902,2.7654678483052));
#56490=CARTESIAN_POINT('Ctrl Pts',(-6.26386065059659,-15.8144217484621,
3.90573734578416));
#56491=CARTESIAN_POINT('Ctrl Pts',(-6.25434443086836,-15.785019022528,3.90345726758071));
#56492=CARTESIAN_POINT('Ctrl Pts',(-6.24500662918812,-15.7549893140376,
3.89973771704937));
#56493=CARTESIAN_POINT('Ctrl Pts',(-6.23594957548642,-15.7245054308269,
3.89442892418346));
#56494=CARTESIAN_POINT('Ctrl Pts',(-6.22712015926251,-15.694787721089,3.88925356104624));
#56495=CARTESIAN_POINT('Ctrl Pts',(-6.21855785026409,-15.6646386876711,
3.88256716093373));
#56496=CARTESIAN_POINT('Ctrl Pts',(-6.21036353205397,-15.6342585338879,
3.87425897704415));
#56497=CARTESIAN_POINT('Ctrl Pts',(-6.20229552087963,-15.6043466591088,
3.86607885531336));
#56498=CARTESIAN_POINT('Ctrl Pts',(-6.19458457012074,-15.5742111835533,
3.85632594327575));
#56499=CARTESIAN_POINT('Ctrl Pts',(-6.18732837413158,-15.5440770840101,
3.84493165751364));
#56500=CARTESIAN_POINT('Ctrl Pts',(-6.180199674674,-15.5144724620581,3.83373757746767));
#56501=CARTESIAN_POINT('Ctrl Pts',(-6.17351022859021,-15.484869802774,3.82095886554755));
#56502=CARTESIAN_POINT('Ctrl Pts',(-6.16734911575842,-15.4555073561589,
3.80657432514532));
#56503=CARTESIAN_POINT('Ctrl Pts',(-6.16654991777089,-15.4516985623769,
3.80470841292217));
#56504=CARTESIAN_POINT('Ctrl Pts',(-6.16575960055991,-15.4478938372451,
3.80281554671202));
#56505=CARTESIAN_POINT('Ctrl Pts',(-6.16497834939201,-15.4440937228137,
3.80089574069978));
#56506=CARTESIAN_POINT('Ctrl Pts',(-6.15904704790929,-15.4152430467601,
3.78632046873251));
#56507=CARTESIAN_POINT('Ctrl Pts',(-6.15363922157741,-15.3866574221223,
3.7701883034186));
#56508=CARTESIAN_POINT('Ctrl Pts',(-6.14882946602223,-15.3585798462333,
3.75253320668798));
#56509=CARTESIAN_POINT('Ctrl Pts',(-6.14408132815942,-15.3308619716668,
3.73510428908576));
#56510=CARTESIAN_POINT('Ctrl Pts',(-6.13991630821544,-15.3036400179101,
3.71619123188256));
#56511=CARTESIAN_POINT('Ctrl Pts',(-6.13639290835345,-15.277148689417,3.69587568153761));
#56512=CARTESIAN_POINT('Ctrl Pts',(-6.13289019776972,-15.2508129170595,
3.67567942337934));
#56513=CARTESIAN_POINT('Ctrl Pts',(-6.13002181404631,-15.225200020221,3.65409730611276));
#56514=CARTESIAN_POINT('Ctrl Pts',(-6.1278283387891,-15.2005294760176,3.63125660399451));
#56515=CARTESIAN_POINT('Ctrl Pts',(-6.1256423054971,-15.1759426333883,3.60849339521025));
#56516=CARTESIAN_POINT('Ctrl Pts',(-6.12412674761708,-15.1522925053128,
3.58448055607693));
#56517=CARTESIAN_POINT('Ctrl Pts',(-6.12330229910817,-15.1297736111913,
3.55938616778094));
#56518=CARTESIAN_POINT('Ctrl Pts',(-6.12247859245493,-15.1072749800319,
3.53431435992954));
#56519=CARTESIAN_POINT('Ctrl Pts',(-6.12234479666278,-15.085906170951,3.50816356397118));
#56520=CARTESIAN_POINT('Ctrl Pts',(-6.12290056030017,-15.0658281226386,
3.48113566064486));
#56521=CARTESIAN_POINT('Ctrl Pts',(-6.12345903224633,-15.0456522313754,
3.45397604681679));
#56522=CARTESIAN_POINT('Ctrl Pts',(-6.12471375736229,-15.0267801876162,
3.4259315055787));
#56523=CARTESIAN_POINT('Ctrl Pts',(-6.12664318986121,-15.009333516031,3.39723119924967));
#56524=CARTESIAN_POINT('Ctrl Pts',(-6.12858008763558,-14.9918193405507,
3.36841984695647));
#56525=CARTESIAN_POINT('Ctrl Pts',(-6.13119677248217,-14.9757418273395,
3.33894848911829));
#56526=CARTESIAN_POINT('Ctrl Pts',(-6.13445162804978,-14.9611764966025,
3.30906130288997));
#56527=CARTESIAN_POINT('Ctrl Pts',(-6.13774388041001,-14.9464438169181,
3.27883072664567));
#56528=CARTESIAN_POINT('Ctrl Pts',(-6.1416888291907,-14.9332583176426,3.24817557819826));
#56529=CARTESIAN_POINT('Ctrl Pts',(-6.146225986249,-14.9216474232892,3.21734812083878));
#56530=CARTESIAN_POINT('Ctrl Pts',(-6.14952974350501,-14.9131928831496,
3.1949009287696));
#56531=CARTESIAN_POINT('Ctrl Pts',(-6.15314710801936,-14.9055721093889,
3.17236239654086));
#56532=CARTESIAN_POINT('Ctrl Pts',(-6.15705019295712,-14.8987793902855,
3.1498259448202));
#56533=CARTESIAN_POINT('Ctrl Pts',(-6.16250603101395,-14.8892843431664,
3.11832388095944));
#56534=CARTESIAN_POINT('Ctrl Pts',(-6.16852029995459,-14.8814088706154,
3.08682723960827));
#56535=CARTESIAN_POINT('Ctrl Pts',(-6.17500715596895,-14.8750972650963,
3.05557116825302));
#56536=CARTESIAN_POINT('Ctrl Pts',(-6.18164240267732,-14.8686412778426,
3.0236000956537));
#56537=CARTESIAN_POINT('Ctrl Pts',(-6.18877175292211,-14.8638210169963,
2.9918813640031));
#56538=CARTESIAN_POINT('Ctrl Pts',(-6.19629782114769,-14.8605341134556,
2.96063315662886));
#56539=CARTESIAN_POINT('Ctrl Pts',(-6.20393536255677,-14.8571985255834,
2.92892211300998));
#56540=CARTESIAN_POINT('Ctrl Pts',(-6.21198110770334,-14.8554413379348,
2.89769601725007));
#56541=CARTESIAN_POINT('Ctrl Pts',(-6.22033312083788,-14.8551215609014,
2.86714098770769));
#56542=CARTESIAN_POINT('Ctrl Pts',(-6.22888542845216,-14.8547941151091,
2.8358532002485));
#56543=CARTESIAN_POINT('Ctrl Pts',(-6.23775854302413,-14.855973076702,2.80526926701399));
#56544=CARTESIAN_POINT('Ctrl Pts',(-6.2468481217032,-14.8584831269518,2.77554067017534));
#56545=CARTESIAN_POINT('Ctrl Pts',(-6.24787807581803,-14.8587675445991,
2.77217207722695));
#56546=CARTESIAN_POINT('Ctrl Pts',(-6.24891081743635,-14.8590690353655,
2.76881441496404));
#56547=CARTESIAN_POINT('Ctrl Pts',(-6.2499462014697,-14.8593873322588,2.76546786460251));
#56548=CARTESIAN_POINT('Ctrl Pts',(6.24994600838289,-14.8593877792286,2.76546575478416));
#56549=CARTESIAN_POINT('Ctrl Pts',(6.23977984081587,-14.8628913778696,2.76270639179577));
#56550=CARTESIAN_POINT('Ctrl Pts',(6.22960745928517,-14.8663868331761,2.75995200693042));
#56551=CARTESIAN_POINT('Ctrl Pts',(6.21942887054227,-14.8698741336584,2.75720262586154));
#56552=CARTESIAN_POINT('Ctrl Pts',(5.94045907762464,-14.9654523634053,2.68184893127683));
#56553=CARTESIAN_POINT('Ctrl Pts',(5.65682493353885,-15.0549072042649,2.61025085701354));
#56554=CARTESIAN_POINT('Ctrl Pts',(5.36871986923688,-15.1379883804168,2.54298737950022));
#56555=CARTESIAN_POINT('Ctrl Pts',(5.20701903870747,-15.1846182278223,2.50523531774958));
#56556=CARTESIAN_POINT('Ctrl Pts',(5.043910181019,-15.2292398216681,2.46884935482955));
#56557=CARTESIAN_POINT('Ctrl Pts',(4.87943057404617,-15.271805068122,2.43393717671929));
#56558=CARTESIAN_POINT('Ctrl Pts',(4.73516526186832,-15.3091391101994,2.40331565246725));
#56559=CARTESIAN_POINT('Ctrl Pts',(4.58984788654057,-15.3448914601748,2.37382281843847));
#56560=CARTESIAN_POINT('Ctrl Pts',(4.44350430295742,-15.3790302121371,2.34551947111766));
#56561=CARTESIAN_POINT('Ctrl Pts',(4.35236115826965,-15.4002919110334,2.32789207662009));
#56562=CARTESIAN_POINT('Ctrl Pts',(4.26081996602347,-15.4209276863025,2.31072611327243));
#56563=CARTESIAN_POINT('Ctrl Pts',(4.1688902167991,-15.4409299318026,2.29403520550717));
#56564=CARTESIAN_POINT('Ctrl Pts',(4.04912204636317,-15.4669893126708,2.27228991083569));
#56565=CARTESIAN_POINT('Ctrl Pts',(3.92869265731007,-15.4919737044677,2.25135119194118));
#56566=CARTESIAN_POINT('Ctrl Pts',(3.80762011138965,-15.5158663514278,2.23124760392297));
#56567=CARTESIAN_POINT('Ctrl Pts',(3.74708383842945,-15.5278126749079,2.22119580991386));
#56568=CARTESIAN_POINT('Ctrl Pts',(3.68638677338942,-15.5394860495579,2.21135279662547));
#56569=CARTESIAN_POINT('Ctrl Pts',(3.62553130145798,-15.5508843162348,2.20172186897067));
#56570=CARTESIAN_POINT('Ctrl Pts',(3.59510356549227,-15.5565834495732,2.19690640514328));
#56571=CARTESIAN_POINT('Ctrl Pts',(3.56463622765007,-15.5622138051242,2.19214396260718));
#56572=CARTESIAN_POINT('Ctrl Pts',(3.53412958926692,-15.5677751085979,2.18743494614879));
#56573=CARTESIAN_POINT('Ctrl Pts',(3.51887627007534,-15.5705557603347,2.18508043791959));
#56574=CARTESIAN_POINT('Ctrl Pts',(3.50361312574009,-15.5733191490016,2.18273928620272));
#56575=CARTESIAN_POINT('Ctrl Pts',(3.48834019436521,-15.5760652400543,2.18041154067411));
#56576=CARTESIAN_POINT('Ctrl Pts',(3.48070372867777,-15.5774382855807,2.1792476679098));
#56577=CARTESIAN_POINT('Ctrl Pts',(3.47306481622993,-15.5788070067004,2.17808714669213));
#56578=CARTESIAN_POINT('Ctrl Pts',(3.46542346181371,-15.5801713990796,2.17692998316942));
#56579=CARTESIAN_POINT('Ctrl Pts',(3.4577821073975,-15.5815357914587,2.17577281964672));
#56580=CARTESIAN_POINT('Ctrl Pts',(3.45127968407358,-15.5826934816899,2.17479074328016));
#56581=CARTESIAN_POINT('Ctrl Pts',(3.44249207745967,-15.5842515856498,2.17346857181511));
#56582=CARTESIAN_POINT('Ctrl Pts',(3.14525419878888,-15.6369539352363,2.12874656060334));
#56583=CARTESIAN_POINT('Ctrl Pts',(2.84604223011535,-15.6827939421746,2.0894683825547));
#56584=CARTESIAN_POINT('Ctrl Pts',(2.54514472779552,-15.721727079666,2.05594698807718));
#56585=CARTESIAN_POINT('Ctrl Pts',(2.4748534034894,-15.7308220763761,2.04811620453046));
#56586=CARTESIAN_POINT('Ctrl Pts',(2.40447003318719,-15.7395399859309,2.04059970994486));
#56587=CARTESIAN_POINT('Ctrl Pts',(2.33399818954889,-15.747879930087,2.03340174451536));
#56588=CARTESIAN_POINT('Ctrl Pts',(2.03519724903146,-15.7832413315922,2.00288233805301));
#56589=CARTESIAN_POINT('Ctrl Pts',(1.73480624879659,-15.8118108685873,1.97808668568234));
#56590=CARTESIAN_POINT('Ctrl Pts',(1.43320004594516,-15.8335486239916,1.9591558973543));
#56591=CARTESIAN_POINT('Ctrl Pts',(1.13568028278521,-15.8549918561875,1.94048160084931));
#56592=CARTESIAN_POINT('Ctrl Pts',(0.836977493414725,-15.8697871517185,
1.92751422946157));
#56593=CARTESIAN_POINT('Ctrl Pts',(0.537450111638287,-15.8778586274268,
1.9204227314522));
#56594=CARTESIAN_POINT('Ctrl Pts',(0.359128834569043,-15.8826639171722,
1.91620086374227));
#56595=CARTESIAN_POINT('Ctrl Pts',(0.180515305473063,-15.8850853530742,
1.91406224079188));
#56596=CARTESIAN_POINT('Ctrl Pts',(0.00168608937214161,-15.8851005062438,
1.91404848768711));
#56597=CARTESIAN_POINT('Ctrl Pts',(0.00126561777193262,-15.8851005418727,
1.91404845535017));
#56598=CARTESIAN_POINT('Ctrl Pts',(0.000845144979868073,-15.8851005641965,
1.9140484347624));
#56599=CARTESIAN_POINT('Ctrl Pts',(0.0004246709969564,-15.8851005732151,
1.91404842592356));
#56600=CARTESIAN_POINT('Ctrl Pts',(-0.295959203807716,-15.8851069302863,
1.91404219559918));
#56601=CARTESIAN_POINT('Ctrl Pts',(-0.591744559536345,-15.8785138703217,
1.91980287342502));
#56602=CARTESIAN_POINT('Ctrl Pts',(-0.88659911326893,-15.865406775067,1.93122579775579));
#56603=CARTESIAN_POINT('Ctrl Pts',(-1.17043855201861,-15.8527893319457,
1.94222198685946));
#56604=CARTESIAN_POINT('Ctrl Pts',(-1.45341579891742,-15.8341351371654,
1.9584656897086));
#56605=CARTESIAN_POINT('Ctrl Pts',(-1.73522496589225,-15.8094873093356,
1.97989352216698));
#56606=CARTESIAN_POINT('Ctrl Pts',(-1.93441571348076,-15.7920655224414,
1.9950393245992));
#56607=CARTESIAN_POINT('Ctrl Pts',(-2.13302831950087,-15.7716507168188,
2.01275505402788));
#56608=CARTESIAN_POINT('Ctrl Pts',(-2.33095462708823,-15.7482542956345,
2.03297954855697));
#56609=CARTESIAN_POINT('Ctrl Pts',(-2.41848204551205,-15.737907877457,2.04192327017052));
#56610=CARTESIAN_POINT('Ctrl Pts',(-2.5058752686069,-15.7269782738699,2.05135769349964));
#56611=CARTESIAN_POINT('Ctrl Pts',(-2.59312769529722,-15.7154672816487,
2.06127283737851));
#56612=CARTESIAN_POINT('Ctrl Pts',(-2.73540614215869,-15.6966968456026,
2.07744099825386));
#56613=CARTESIAN_POINT('Ctrl Pts',(-2.8773069640955,-15.6763802934088,2.09489214436736));
#56614=CARTESIAN_POINT('Ctrl Pts',(-3.01879388031371,-15.654524164203,2.11359109983342));
#56615=CARTESIAN_POINT('Ctrl Pts',(-3.08953733842282,-15.6435960996002,
2.12294057756645));
#56616=CARTESIAN_POINT('Ctrl Pts',(-3.16017731874909,-15.6322831201713,
2.13260200512541));
#56617=CARTESIAN_POINT('Ctrl Pts',(-3.23070939172754,-15.6205859822879,
2.14257039117694));
#56618=CARTESIAN_POINT('Ctrl Pts',(-3.26597542821676,-15.6147374133462,
2.14755458420271));
#56619=CARTESIAN_POINT('Ctrl Pts',(-3.30121448775136,-15.6087928035061,
2.15261551669182));
#56620=CARTESIAN_POINT('Ctrl Pts',(-3.33642601923097,-15.6027522412624,
2.15775254825432));
#56621=CARTESIAN_POINT('Ctrl Pts',(-3.35403178497077,-15.5997319601406,
2.16032106403558));
#56622=CARTESIAN_POINT('Ctrl Pts',(-3.37163066868688,-15.5966876908382,
2.16290860457476));
#56623=CARTESIAN_POINT('Ctrl Pts',(-3.38922260183242,-15.5936194441472,
2.16551508782531));
#56624=CARTESIAN_POINT('Ctrl Pts',(-3.39801856840519,-15.5920853208017,
2.16681832945058));
#56625=CARTESIAN_POINT('Ctrl Pts',(-3.40681279733464,-15.5905452031042,
2.16812630675302));
#56626=CARTESIAN_POINT('Ctrl Pts',(-3.41560528007505,-15.5889990923873,
2.16943900934683));
#56627=CARTESIAN_POINT('Ctrl Pts',(-3.42439776281546,-15.5874529816703,
2.17075171194064));
#56628=CARTESIAN_POINT('Ctrl Pts',(-3.43433010001144,-15.5856984969522,
2.17224087292842));
#56629=CARTESIAN_POINT('Ctrl Pts',(-3.44197748118868,-15.5843427824956,
2.17339128257614));
#56630=CARTESIAN_POINT('Ctrl Pts',(-3.7396863674353,-15.5315654680661,2.21817617913244));
#56631=CARTESIAN_POINT('Ctrl Pts',(-4.03372618068042,-15.4722068983851,
2.26813399437449));
#56632=CARTESIAN_POINT('Ctrl Pts',(-4.32379161088466,-15.4065298160674,
2.32277245567381));
#56633=CARTESIAN_POINT('Ctrl Pts',(-4.36297511470441,-15.3976578239653,
2.33015329507794));
#56634=CARTESIAN_POINT('Ctrl Pts',(-4.40208612349489,-15.3886704891556,
2.33761960458001));
#56635=CARTESIAN_POINT('Ctrl Pts',(-4.44112391129496,-15.3795684196056,
2.34517022409203));
#56636=CARTESIAN_POINT('Ctrl Pts',(-4.74647716824373,-15.3083721060159,
2.40423110817141));
#56637=CARTESIAN_POINT('Ctrl Pts',(-5.04734945831461,-15.2301587791586,
2.46844652844401));
#56638=CARTESIAN_POINT('Ctrl Pts',(-5.34351993333399,-15.1452169653489,
2.53722993612569));
#56639=CARTESIAN_POINT('Ctrl Pts',(-5.63969040835337,-15.0602751515392,
2.60601334380737));
#56640=CARTESIAN_POINT('Ctrl Pts',(-5.93115934890157,-14.9686047302175,
2.67936508447682));
#56641=CARTESIAN_POINT('Ctrl Pts',(-6.21771626963549,-14.8704603665138,
2.75674241330942));
#56642=CARTESIAN_POINT('Ctrl Pts',(-6.22846649522594,-14.8667784660818,
2.75964523533308));
#56643=CARTESIAN_POINT('Ctrl Pts',(-6.23920980862789,-14.8630874504706,
2.76255372768559));
#56644=CARTESIAN_POINT('Ctrl Pts',(-6.2499462014697,-14.8593873322588,2.76546786460251));
#56645=CARTESIAN_POINT('Ctrl Pts',(-6.25110470371109,-15.8289287536332,
3.90218662864265));
#56646=CARTESIAN_POINT('Ctrl Pts',(-6.29476787337534,-15.8135896688474,
3.91359102765067));
#56647=CARTESIAN_POINT('Ctrl Pts',(-6.42720364559721,-15.7642107597959,
3.95728968749399));
#56648=CARTESIAN_POINT('Ctrl Pts',(-6.63601152178557,-15.6709885974876,
4.07488311644954));
#56649=CARTESIAN_POINT('Ctrl Pts',(-6.84944948528204,-15.5474618085486,
4.28281049117623));
#56650=CARTESIAN_POINT('Ctrl Pts',(-7.00820034346764,-15.4198890442991,
4.54620357973042));
#56651=CARTESIAN_POINT('Ctrl Pts',(-7.09186675915703,-15.3065623348527,
4.82366122629296));
#56652=CARTESIAN_POINT('Ctrl Pts',(-7.10635949500348,-15.2412500255453,
5.00871313350102));
#56653=CARTESIAN_POINT('Ctrl Pts',(-7.10529849916785,-15.2149614744649,
5.08843009648874));
#56654=CARTESIAN_POINT('Ctrl Pts',(-6.05286305785348,-15.2163005098727,
3.8610994146941));
#56655=CARTESIAN_POINT('Ctrl Pts',(-6.09151808910752,-15.2026886082459,
3.87091449473368));
#56656=CARTESIAN_POINT('Ctrl Pts',(-6.20897986088989,-15.1587870717599,
3.90862214879026));
#56657=CARTESIAN_POINT('Ctrl Pts',(-6.39516878893685,-15.0754962562282,
4.01082172167384));
#56658=CARTESIAN_POINT('Ctrl Pts',(-6.58655600753875,-14.9647336461454,
4.19297762573022));
#56659=CARTESIAN_POINT('Ctrl Pts',(-6.72947207118409,-14.8503179692945,
4.42503188515894));
#56660=CARTESIAN_POINT('Ctrl Pts',(-6.80490807319583,-14.7490641911142,
4.67022341605911));
#56661=CARTESIAN_POINT('Ctrl Pts',(-6.81792929536288,-14.6911932840215,
4.83365326926337));
#56662=CARTESIAN_POINT('Ctrl Pts',(-6.81697819600131,-14.6680366840076,
4.90391474801704));
#56663=CARTESIAN_POINT('Ctrl Pts',(-6.04143776493508,-14.8034131353335,
3.36534479494879));
#56664=CARTESIAN_POINT('Ctrl Pts',(-6.09466994263046,-14.7850570925795,
3.37877528165601));
#56665=CARTESIAN_POINT('Ctrl Pts',(-6.25547105388986,-14.7263459526608,
3.43011952370043));
#56666=CARTESIAN_POINT('Ctrl Pts',(-6.5059867483565,-14.6174407821712,3.56694282528));
#56667=CARTESIAN_POINT('Ctrl Pts',(-6.75879992208355,-14.4756583694627,
3.80561255232722));
#56668=CARTESIAN_POINT('Ctrl Pts',(-6.94511346013031,-14.3309179928438,
4.10493100761516));
#56669=CARTESIAN_POINT('Ctrl Pts',(-7.04295606862131,-14.2029509252661,
4.4186870668889));
#56670=CARTESIAN_POINT('Ctrl Pts',(-7.0600439880215,-14.1289188698671,4.6285048841726));
#56671=CARTESIAN_POINT('Ctrl Pts',(-7.05878639808624,-14.0989674529702,
4.71932477573061));
#56672=CARTESIAN_POINT('Ctrl Pts',(-6.22464327430951,-14.869698639165,2.75012280382206));
#56673=CARTESIAN_POINT('Ctrl Pts',(-6.3021844915154,-14.8433338792577,2.76992975345015));
#56674=CARTESIAN_POINT('Ctrl Pts',(-6.53534318406533,-14.7595365042026,
2.84532114539174));
#56675=CARTESIAN_POINT('Ctrl Pts',(-6.89365005061659,-14.6067847346553,
3.04338350732949));
#56676=CARTESIAN_POINT('Ctrl Pts',(-7.24984556193816,-14.4111653547389,
3.38265482800274));
#56677=CARTESIAN_POINT('Ctrl Pts',(-7.50945482979155,-14.2131151686788,
3.80237713753254));
#56678=CARTESIAN_POINT('Ctrl Pts',(-7.64519560700152,-14.0377040723409,
4.23918626315073));
#56679=CARTESIAN_POINT('Ctrl Pts',(-7.66913959269001,-13.9348315572258,
4.53204878917508));
#56680=CARTESIAN_POINT('Ctrl Pts',(-7.66736629471592,-13.8927511366881,
4.65954565759216));
#56681=CARTESIAN_POINT('',(-7.00000834771932,-14.7967990237358,4.92966193756367));
#56682=CARTESIAN_POINT('',(-7.00000024832194,-14.5427415422438,3.16613142102349));
#56683=CARTESIAN_POINT('Ctrl Pts',(-7.,-14.7967990237703,4.92966193770567));
#56684=CARTESIAN_POINT('Ctrl Pts',(-7.,-14.7557808111679,4.82629817381466));
#56685=CARTESIAN_POINT('Ctrl Pts',(-7.,-14.7211382308601,4.73284571088999));
#56686=CARTESIAN_POINT('Ctrl Pts',(-7.,-14.6931996139855,4.65100396188635));
#56687=CARTESIAN_POINT('Ctrl Pts',(-7.,-14.6792303055482,4.61008308738453));
#56688=CARTESIAN_POINT('Ctrl Pts',(-7.,-14.6668893039443,4.57207807978592));
#56689=CARTESIAN_POINT('Ctrl Pts',(-7.,-14.6560069105721,4.53722371941572));
#56690=CARTESIAN_POINT('Ctrl Pts',(-7.,-14.650565713886,4.51979653923062));
#56691=CARTESIAN_POINT('Ctrl Pts',(-7.,-14.6454875640803,4.50315711223306));
#56692=CARTESIAN_POINT('Ctrl Pts',(-7.,-14.6407442198345,4.48733398590899));
#56693=CARTESIAN_POINT('Ctrl Pts',(-7.,-14.6383725477116,4.47942242274696));
#56694=CARTESIAN_POINT('Ctrl Pts',(-7.,-14.6360845769787,4.47171493475331));
#56695=CARTESIAN_POINT('Ctrl Pts',(-7.,-14.6338764851935,4.46421491609655));
#56696=CARTESIAN_POINT('Ctrl Pts',(-7.,-14.6327724393009,4.46046490676816));
#56697=CARTESIAN_POINT('Ctrl Pts',(-7.,-14.6316883631452,4.45676676477401));
#56698=CARTESIAN_POINT('Ctrl Pts',(-7.,-14.6306237806622,4.45312090459993));
#56699=CARTESIAN_POINT('Ctrl Pts',(-7.,-14.6295591981792,4.44947504442585));
#56700=CARTESIAN_POINT('Ctrl Pts',(-7.,-14.6289879217431,4.44751654562367));
#56701=CARTESIAN_POINT('Ctrl Pts',(-7.,-14.6274880358216,4.44234058010723));
#56702=CARTESIAN_POINT('Ctrl Pts',(-7.,-14.6034898610781,4.35952513184433));
#56703=CARTESIAN_POINT('Ctrl Pts',(-7.,-14.5830030031066,4.27925663787387));
#56704=CARTESIAN_POINT('Ctrl Pts',(-7.,-14.5661061896712,4.20216723805092));
#56705=CARTESIAN_POINT('Ctrl Pts',(-7.,-14.5492093762358,4.12507783822797));
#56706=CARTESIAN_POINT('Ctrl Pts',(-7.,-14.536122312737,4.05276435033893));
#56707=CARTESIAN_POINT('Ctrl Pts',(-7.,-14.5256426270648,3.98124825300832));
#56708=CARTESIAN_POINT('Ctrl Pts',(-7.,-14.5046832557203,3.8382160583471));
#56709=CARTESIAN_POINT('Ctrl Pts',(-7.,-14.4945097492703,3.69572700311663));
#56710=CARTESIAN_POINT('Ctrl Pts',(-7.,-14.4974000293464,3.55811099350387));
#56711=CARTESIAN_POINT('Ctrl Pts',(-7.,-14.5002903094225,3.4204949838911));
#56712=CARTESIAN_POINT('Ctrl Pts',(-7.,-14.5162124657349,3.28797540399407));
#56713=CARTESIAN_POINT('Ctrl Pts',(-7.,-14.5427409643167,3.16613181594226));
#56714=CARTESIAN_POINT('Ctrl Pts',(-6.249946124203,-14.8593870695528,2.7654678157106));
#56715=CARTESIAN_POINT('Ctrl Pts',(-6.343283744982,-14.8272204162322,2.79079893610273));
#56716=CARTESIAN_POINT('Ctrl Pts',(-6.523195179618,-14.7609017514799,2.85471778320166));
#56717=CARTESIAN_POINT('Ctrl Pts',(-6.77477936719767,-14.6549005700431,
2.9891531637239));
#56718=CARTESIAN_POINT('Ctrl Pts',(-6.92743954945432,-14.5808182851627,
3.10289863010712));
#56719=CARTESIAN_POINT('Ctrl Pts',(-7.00000073074686,-14.5427415372861,
3.166130864439));
#56720=CARTESIAN_POINT('Ctrl Pts',(-6.26385620203836,-15.8144219269702,
3.90575361027663));
#56721=CARTESIAN_POINT('Ctrl Pts',(-6.29878849880756,-15.7919498083394,
3.9155545662544));
#56722=CARTESIAN_POINT('Ctrl Pts',(-6.33342137746813,-15.7685324070384,
3.92737928356594));
#56723=CARTESIAN_POINT('Ctrl Pts',(-6.36751124742063,-15.7442057457572,
3.94126218049215));
#56724=CARTESIAN_POINT('Ctrl Pts',(-6.41221172875109,-15.7123073117078,
3.95946618583823));
#56725=CARTESIAN_POINT('Ctrl Pts',(-6.45597990026991,-15.6788445993522,
3.98120981151469));
#56726=CARTESIAN_POINT('Ctrl Pts',(-6.49830303351248,-15.6439338049921,
4.00642789449063));
#56727=CARTESIAN_POINT('Ctrl Pts',(-6.51773444154521,-15.6279055519308,
4.01800602735948));
#56728=CARTESIAN_POINT('Ctrl Pts',(-6.53686061955037,-15.6115723297184,
4.03031648655404));
#56729=CARTESIAN_POINT('Ctrl Pts',(-6.55562848922986,-15.5949468145626,
4.04335300963381));
#56730=CARTESIAN_POINT('Ctrl Pts',(-6.56693295578168,-15.5849327541927,
4.05120530942191));
#56731=CARTESIAN_POINT('Ctrl Pts',(-6.5781074009999,-15.5748126648585,4.05932104211864));
#56732=CARTESIAN_POINT('Ctrl Pts',(-6.58913980261017,-15.564589480158,4.06769890657097));
#56733=CARTESIAN_POINT('Ctrl Pts',(-6.6224247220355,-15.5337459801617,4.09297504798636));
#56734=CARTESIAN_POINT('Ctrl Pts',(-6.65441844741923,-15.5019631749137,
4.12063740177302));
#56735=CARTESIAN_POINT('Ctrl Pts',(-6.68483583877449,-15.4693356416747,
4.1505725029576));
#56736=CARTESIAN_POINT('Ctrl Pts',(-6.70508550921129,-15.4476146207122,
4.17050109993688));
#56737=CARTESIAN_POINT('Ctrl Pts',(-6.72463611746707,-15.425519458277,4.19143689346209));
#56738=CARTESIAN_POINT('Ctrl Pts',(-6.74339683172981,-15.4030811212164,
4.21334656021343));
#56739=CARTESIAN_POINT('Ctrl Pts',(-6.75277718886118,-15.3918619526861,
4.22430139358911));
#56740=CARTESIAN_POINT('Ctrl Pts',(-6.76196001583808,-15.380556992843,4.2354997441859));
#56741=CARTESIAN_POINT('Ctrl Pts',(-6.77093332222585,-15.3691703979231,
4.24693746861905));
#56742=CARTESIAN_POINT('Ctrl Pts',(-6.77168679657353,-15.3682142835536,
4.24789787625296));
#56743=CARTESIAN_POINT('Ctrl Pts',(-6.77243879339467,-15.3672575937706,
4.24885997164811));
#56744=CARTESIAN_POINT('Ctrl Pts',(-6.77318930549531,-15.3663003310321,
4.24982375242268));
#56745=CARTESIAN_POINT('Ctrl Pts',(-6.77690780753395,-15.3615574582103,
4.2545989196345));
#56746=CARTESIAN_POINT('Ctrl Pts',(-6.7805898630739,-15.3568005199061,4.2594154600463));
#56747=CARTESIAN_POINT('Ctrl Pts',(-6.78423480615889,-15.3520298334718,
4.26427287788366));
#56748=CARTESIAN_POINT('Ctrl Pts',(-6.78642511048231,-15.3491630520492,
4.26719177758709));
#56749=CARTESIAN_POINT('Ctrl Pts',(-6.78860201371202,-15.3462913058629,
4.27012543865483));
#56750=CARTESIAN_POINT('Ctrl Pts',(-6.79076536854309,-15.3434146664145,
4.27307375201837));
#56751=CARTESIAN_POINT('Ctrl Pts',(-6.79256527438427,-15.3410213095449,
4.27552674140709));
#56752=CARTESIAN_POINT('Ctrl Pts',(-6.79472129741818,-15.3381328046024,
4.27849606180966));
#56753=CARTESIAN_POINT('Ctrl Pts',(-6.79632073241739,-15.3359765995829,
4.28071849115757));
#56754=CARTESIAN_POINT('Ctrl Pts',(-6.79664370099805,-15.335541204287,4.28116725891148));
#56755=CARTESIAN_POINT('Ctrl Pts',(-6.79694411509937,-15.3351356778824,
4.28158545805962));
#56756=CARTESIAN_POINT('Ctrl Pts',(-6.79721464032234,-15.3347701387616,
4.28196254138343));
#56757=CARTESIAN_POINT('Ctrl Pts',(-6.813641421115,-15.3125739422593,4.30485972277292));
#56758=CARTESIAN_POINT('Ctrl Pts',(-6.8298628224892,-15.2892413668964,4.32945828123986));
#56759=CARTESIAN_POINT('Ctrl Pts',(-6.84559240418816,-15.264799690596,4.35586039075551));
#56760=CARTESIAN_POINT('Ctrl Pts',(-6.86049447053488,-15.2416438630078,
4.38087351540342));
#56761=CARTESIAN_POINT('Ctrl Pts',(-6.87495525595165,-15.217492469619,4.40750543899532));
#56762=CARTESIAN_POINT('Ctrl Pts',(-6.88869160911252,-15.1923864352567,
4.43582616937284));
#56763=CARTESIAN_POINT('Ctrl Pts',(-6.89525615325614,-15.1803883693281,
4.44936052471195));
#56764=CARTESIAN_POINT('Ctrl Pts',(-6.9016546372832,-15.168172554529,4.46328032005208));
#56765=CARTESIAN_POINT('Ctrl Pts',(-6.90785249150635,-15.1557451069306,
4.47759170963739));
#56766=CARTESIAN_POINT('Ctrl Pts',(-6.91793699586261,-15.1355244555679,
4.50087771563573));
#56767=CARTESIAN_POINT('Ctrl Pts',(-6.927490981232,-15.114742987979,4.52520121964848));
#56768=CARTESIAN_POINT('Ctrl Pts',(-6.93637014188753,-15.0934359688446,
4.55056606232792));
#56769=CARTESIAN_POINT('Ctrl Pts',(-6.94680888543516,-15.0683864718102,
4.58038612056639));
#56770=CARTESIAN_POINT('Ctrl Pts',(-6.95631603183839,-15.0426099666793,
4.61164611650852));
#56771=CARTESIAN_POINT('Ctrl Pts',(-6.96462796028164,-15.0161820172215,
4.64433003797493));
#56772=CARTESIAN_POINT('Ctrl Pts',(-6.97210085492414,-14.9924217931937,
4.67371473531559));
#56773=CARTESIAN_POINT('Ctrl Pts',(-6.97860757742105,-14.9681351353331,
4.70425016069309));
#56774=CARTESIAN_POINT('Ctrl Pts',(-6.98392953768413,-14.9433927148096,
4.73590672977319));
#56775=CARTESIAN_POINT('Ctrl Pts',(-6.9894513026938,-14.9177213784697,4.76875179565718));
#56776=CARTESIAN_POINT('Ctrl Pts',(-6.99369738134614,-14.8915589743126,
4.80280473163056));
#56777=CARTESIAN_POINT('Ctrl Pts',(-6.99643896516185,-14.8650099262391,
4.83797412724184));
#56778=CARTESIAN_POINT('Ctrl Pts',(-6.99876094637331,-14.8425242409736,
4.86776080578873));
#56779=CARTESIAN_POINT('Ctrl Pts',(-7.00000353949097,-14.8197614873671,
4.89834788628858));
#56780=CARTESIAN_POINT('Ctrl Pts',(-7.0000090556196,-14.7967990238705,4.92966193753773));
#56781=CARTESIAN_POINT('Ctrl Pts',(-6.23412951824369,-25.6421123574084,
8.85535208221471));
#56782=CARTESIAN_POINT('Ctrl Pts',(-6.23490481866159,-25.3447917649169,
8.44426386352628));
#56783=CARTESIAN_POINT('Ctrl Pts',(-6.23649261565224,-24.5993905992671,
7.54006472228264));
#56784=CARTESIAN_POINT('Ctrl Pts',(-6.23803947015578,-23.2351584307484,
6.3068279708346));
#56785=CARTESIAN_POINT('Ctrl Pts',(-6.23759227455821,-21.5545925361952,
5.23225202843968));
#56786=CARTESIAN_POINT('Ctrl Pts',(-6.23570310449509,-19.7179594361743,
4.44990383975616));
#56787=CARTESIAN_POINT('Ctrl Pts',(-6.23204929482609,-17.7794287558552,
3.98190995592453));
#56788=CARTESIAN_POINT('Ctrl Pts',(-6.22726074605045,-16.0460358301738,
3.85975953085696));
#56789=CARTESIAN_POINT('Ctrl Pts',(-6.22400119816621,-14.9771498623589,
3.9271878537008));
#56790=CARTESIAN_POINT('Ctrl Pts',(-6.2226656607601,-14.5714122496638,3.9737494255116));
#56791=CARTESIAN_POINT('Ctrl Pts',(-6.72598973094391,-25.5461080305609,
8.92473407566849));
#56792=CARTESIAN_POINT('Ctrl Pts',(-6.726682888266,-25.2514056837406,8.51794194318656));
#56793=CARTESIAN_POINT('Ctrl Pts',(-6.72805115220009,-24.5127390076592,
7.6231901818145));
#56794=CARTESIAN_POINT('Ctrl Pts',(-6.72941870118895,-23.1617868482333,
6.40302824892384));
#56795=CARTESIAN_POINT('Ctrl Pts',(-6.72902370101902,-21.4982080380591,
5.33903634346242));
#56796=CARTESIAN_POINT('Ctrl Pts',(-6.72736764457739,-19.6804284777096,
4.56367588073428));
#56797=CARTESIAN_POINT('Ctrl Pts',(-6.72416397934811,-17.7615746380771,
4.09849087757912));
#56798=CARTESIAN_POINT('Ctrl Pts',(-6.71993311440092,-16.0451960532337,
3.97507643032026));
#56799=CARTESIAN_POINT('Ctrl Pts',(-6.71707859590867,-14.9863242428538,
4.04021097259499));
#56800=CARTESIAN_POINT('Ctrl Pts',(-6.71588986670998,-14.5843406118397,
4.08565752022343));
#56801=CARTESIAN_POINT('Ctrl Pts',(-7.02718519799001,-25.2169072632673,
9.16264676213727));
#56802=CARTESIAN_POINT('Ctrl Pts',(-7.02756389243507,-24.9320799770197,
8.76993802976445));
#56803=CARTESIAN_POINT('Ctrl Pts',(-7.02824880449839,-24.2181494335702,
7.90599874558347));
#56804=CARTESIAN_POINT('Ctrl Pts',(-7.02897712669706,-22.9136314295433,
6.72847692729127));
#56805=CARTESIAN_POINT('Ctrl Pts',(-7.02876720163468,-21.3070953687618,
5.70076837624308));
#56806=CARTESIAN_POINT('Ctrl Pts',(-7.02790266440921,-19.5522398659708,
4.95159468384772));
#56807=CARTESIAN_POINT('Ctrl Pts',(-7.02622931287819,-17.699530350317,4.50113364131783));
#56808=CARTESIAN_POINT('Ctrl Pts',(-7.02397928601801,-16.0419249094978,
4.38032070770886));
#56809=CARTESIAN_POINT('Ctrl Pts',(-7.02249260484221,-15.0188815943411,
4.44215073383211));
#56810=CARTESIAN_POINT('Ctrl Pts',(-7.0218496413372,-14.6305434261105,4.48559561596503));
#56811=CARTESIAN_POINT('Ctrl Pts',(-6.99838063007145,-24.8079471174881,
9.45820150662415));
#56812=CARTESIAN_POINT('Ctrl Pts',(-6.99835913456694,-24.5356483643624,
9.0827998521431));
#56813=CARTESIAN_POINT('Ctrl Pts',(-6.99821532660071,-23.8529250977185,
8.25667796475706));
#56814=CARTESIAN_POINT('Ctrl Pts',(-6.99814245616926,-22.6063522384878,
7.13148910279274));
#56815=CARTESIAN_POINT('Ctrl Pts',(-6.99816421969244,-21.0703284717052,
6.1488519358181));
#56816=CARTESIAN_POINT('Ctrl Pts',(-6.99828069431127,-19.3931405999627,
5.43285699124196));
#56817=CARTESIAN_POINT('Ctrl Pts',(-6.99850457242363,-17.6222147137414,
5.00216844902164));
#56818=CARTESIAN_POINT('Ctrl Pts',(-6.99873523795064,-16.0377473415385,
4.88660477570714));
#56819=CARTESIAN_POINT('Ctrl Pts',(-6.99894168314433,-15.0596464417134,
4.94565629804127));
#56820=CARTESIAN_POINT('Ctrl Pts',(-6.99898903502728,-14.6884846235588,
4.98714444975514));
#56821=CARTESIAN_POINT('',(-7.00000308919771,-24.7867179209035,9.33251796322023));
#56822=CARTESIAN_POINT('Origin',(-5.99998370363654,-24.7867138051394,9.33252808558063));
#56823=CARTESIAN_POINT('Ctrl Pts',(-7.00001101651462,-24.7867134185486,
9.33251828870258));
#56824=CARTESIAN_POINT('Ctrl Pts',(-7.00001786889336,-24.6735525617516,
9.17932101458571));
#56825=CARTESIAN_POINT('Ctrl Pts',(-7.00001802523742,-24.5580142816453,
9.03121151943847));
#56826=CARTESIAN_POINT('Ctrl Pts',(-7.00001556840049,-24.4406110956016,
8.88816527848438));
#56827=CARTESIAN_POINT('Ctrl Pts',(-7.00001306418049,-24.3209436477261,
8.74236021850253));
#56828=CARTESIAN_POINT('Ctrl Pts',(-7.00000784357216,-24.1993386409877,
8.60181549568451));
#56829=CARTESIAN_POINT('Ctrl Pts',(-7.00000354839216,-24.0762963462373,
8.4664716215797));
#56830=CARTESIAN_POINT('Ctrl Pts',(-7.00000225631055,-24.039282603626,8.42575730192));
#56831=CARTESIAN_POINT('Ctrl Pts',(-7.00000104345735,-24.0021385108519,
8.38551340481799));
#56832=CARTESIAN_POINT('Ctrl Pts',(-6.99999999753998,-23.9648769610003,
8.34573775584444));
#56833=CARTESIAN_POINT('Ctrl Pts',(-6.99999887666308,-23.9249449244552,
8.30311143797125));
#56834=CARTESIAN_POINT('Ctrl Pts',(-6.99999794690458,-23.8848779940374,
8.26102288192524));
#56835=CARTESIAN_POINT('Ctrl Pts',(-6.99999718086705,-23.8446913250953,
8.21946685878418));
#56836=CARTESIAN_POINT('Ctrl Pts',(-6.99999462214246,-23.7104594977578,
8.08066110379241));
#56837=CARTESIAN_POINT('Ctrl Pts',(-6.99999387750223,-23.5748954425034,
7.94779834684371));
#56838=CARTESIAN_POINT('Ctrl Pts',(-6.99999403434674,-23.4385318409074,
7.82067014042885));
#56839=CARTESIAN_POINT('Ctrl Pts',(-6.99999406716637,-23.4099978376986,
7.79406863821478));
#56840=CARTESIAN_POINT('Ctrl Pts',(-6.99999414003187,-23.3814286575789,
7.76771815577077));
#56841=CARTESIAN_POINT('Ctrl Pts',(-6.99999424548609,-23.3528289165217,
7.74161667605472));
#56842=CARTESIAN_POINT('Ctrl Pts',(-6.9999943242214,-23.3314754878549,7.72212852460256));
#56843=CARTESIAN_POINT('Ctrl Pts',(-6.99999441863055,-23.3106151793539,
7.70323910621462));
#56844=CARTESIAN_POINT('Ctrl Pts',(-6.99999453138906,-23.2890698214933,
7.68388256127447));
#56845=CARTESIAN_POINT('Ctrl Pts',(-6.99999463682087,-23.268924416221,7.66578374643865));
#56846=CARTESIAN_POINT('Ctrl Pts',(-6.99999475847195,-23.2481799802744,
7.64727659129448));
#56847=CARTESIAN_POINT('Ctrl Pts',(-6.99999490350867,-23.2258462584489,
7.62752046795438));
#56848=CARTESIAN_POINT('Ctrl Pts',(-6.99999520366107,-23.1796267908374,
7.58663532082214));
#56849=CARTESIAN_POINT('Ctrl Pts',(-6.99999556265701,-23.1331495398512,
7.5462152702438));
#56850=CARTESIAN_POINT('Ctrl Pts',(-6.99999595370187,-23.086424366087,7.50626141913471));
#56851=CARTESIAN_POINT('Ctrl Pts',(-6.99999673579158,-22.9929740185586,
7.42635371691654));
#56852=CARTESIAN_POINT('Ctrl Pts',(-6.99999764537285,-22.8985319799185,
7.34831081257529));
#56853=CARTESIAN_POINT('Ctrl Pts',(-6.9999984763219,-22.803174991709,7.27213995952607));
#56854=CARTESIAN_POINT('Ctrl Pts',(-6.99999902465916,-22.7402496061458,
7.22187536553239));
#56855=CARTESIAN_POINT('Ctrl Pts',(-6.99999953898004,-22.6769257511323,
7.17242593768393));
#56856=CARTESIAN_POINT('Ctrl Pts',(-6.99999996276703,-22.6132249339512,
7.123793362472));
#56857=CARTESIAN_POINT('Ctrl Pts',(-7.00000126736887,-22.4171259390615,
6.97408101120292));
#56858=CARTESIAN_POINT('Ctrl Pts',(-7.00000171385138,-22.2174580789129,
6.83211162083866));
#56859=CARTESIAN_POINT('Ctrl Pts',(-7.00000170643233,-22.0149140870436,
6.69789048236768));
#56860=CARTESIAN_POINT('Ctrl Pts',(-7.00000169893394,-21.8102044420194,
6.56223421649901));
#56861=CARTESIAN_POINT('Ctrl Pts',(-7.00000122940959,-21.6025568059502,
6.43449274577891));
#56862=CARTESIAN_POINT('Ctrl Pts',(-7.00000072342098,-21.3926392985623,
6.31464641178277));
#56863=CARTESIAN_POINT('Ctrl Pts',(-7.00000046988466,-21.2874556815005,
6.25459486554357));
#56864=CARTESIAN_POINT('Ctrl Pts',(-7.00000020716533,-21.181701431279,6.19652518159974));
#56865=CARTESIAN_POINT('Ctrl Pts',(-6.99999998766531,-21.0754562644221,
6.14043259863199));
#56866=CARTESIAN_POINT('Ctrl Pts',(-6.99999993929023,-21.0520411488934,
6.12807048984769));
#56867=CARTESIAN_POINT('Ctrl Pts',(-6.99999989300831,-21.0286021782591,
6.11580440433564));
#56868=CARTESIAN_POINT('Ctrl Pts',(-6.99999984878695,-21.0051402164893,
6.10363414171722));
#56869=CARTESIAN_POINT('Ctrl Pts',(-6.99999965374734,-20.9016605318255,
6.04995683415067));
#56870=CARTESIAN_POINT('Ctrl Pts',(-6.9999994986378,-20.7977338128376,5.99814360645079));
#56871=CARTESIAN_POINT('Ctrl Pts',(-6.99999938184552,-20.6934325505225,
5.94817680192591));
#56872=CARTESIAN_POINT('Ctrl Pts',(-6.99999932344938,-20.6412819193649,
5.92319339966347));
#56873=CARTESIAN_POINT('Ctrl Pts',(-6.99999927466388,-20.5890376523755,
5.89867160319478));
#56874=CARTESIAN_POINT('Ctrl Pts',(-6.99999923547139,-20.5367085182238,
5.8746091226682));
#56875=CARTESIAN_POINT('Ctrl Pts',(-6.99999921587514,-20.5105439511479,
5.86257788240491));
#56876=CARTESIAN_POINT('Ctrl Pts',(-6.99999919867917,-20.4843581672814,
5.85066147112715));
#56877=CARTESIAN_POINT('Ctrl Pts',(-6.99999918389325,-20.4581522540645,
5.83885960020213));
#56878=CARTESIAN_POINT('Ctrl Pts',(-6.99999917282793,-20.4385405914925,
5.83002745959391));
#56879=CARTESIAN_POINT('Ctrl Pts',(-6.99999916268469,-20.4179924212598,
5.82084773391597));
#56880=CARTESIAN_POINT('Ctrl Pts',(-6.99999915445603,-20.3985849927827,
5.8122457053959));
#56881=CARTESIAN_POINT('Ctrl Pts',(-6.99999915168922,-20.3920594140724,
5.80935334826356));
#56882=CARTESIAN_POINT('Ctrl Pts',(-6.99999914912883,-20.3856629887566,
5.80652589257862));
#56883=CARTESIAN_POINT('Ctrl Pts',(-6.99999914678339,-20.3794752088658,
5.80379731846812));
#56884=CARTESIAN_POINT('Ctrl Pts',(-6.9999990752884,-20.1908565965901,5.72062372934665));
#56885=CARTESIAN_POINT('Ctrl Pts',(-6.99999912491181,-19.9974675950207,
5.64168486729232));
#56886=CARTESIAN_POINT('Ctrl Pts',(-6.99999933315404,-19.7994486766844,
5.56752055257987));
#56887=CARTESIAN_POINT('Ctrl Pts',(-6.99999947285256,-19.6666084304028,
5.51776770111255));
#56888=CARTESIAN_POINT('Ctrl Pts',(-6.99999968442926,-19.5316854129743,
5.47016413546951));
#56889=CARTESIAN_POINT('Ctrl Pts',(-6.99999998816764,-19.3947330689576,
5.42488006668253));
#56890=CARTESIAN_POINT('Ctrl Pts',(-7.00000042904106,-19.1959480205455,
5.35915066372301));
#56891=CARTESIAN_POINT('Ctrl Pts',(-7.0000010678187,-18.9928853289915,5.29830714986745));
#56892=CARTESIAN_POINT('Ctrl Pts',(-7.00000153332806,-18.7857678324651,
5.24286449209894));
#56893=CARTESIAN_POINT('Ctrl Pts',(-7.00000199136829,-18.5819735465795,
5.18831141456069));
#56894=CARTESIAN_POINT('Ctrl Pts',(-7.0000022813417,-18.3742534735699,5.1389872835667));
#56895=CARTESIAN_POINT('Ctrl Pts',(-7.00000202664213,-18.1628647433994,
5.09540490049247));
#56896=CARTESIAN_POINT('Ctrl Pts',(-7.00000181210257,-17.9848069480198,
5.0586944143595));
#56897=CARTESIAN_POINT('Ctrl Pts',(-7.00000121063512,-17.80414691375,5.02605811832913));
#56898=CARTESIAN_POINT('Ctrl Pts',(-6.99999998662393,-17.6210641954966,
4.99781497974106));
#56899=CARTESIAN_POINT('Ctrl Pts',(-6.99999852879723,-17.4030082841283,
4.96417672385608));
#56900=CARTESIAN_POINT('Ctrl Pts',(-6.99999617282082,-17.1815143987631,
4.93677080855326));
#56901=CARTESIAN_POINT('Ctrl Pts',(-6.99999449839284,-16.9569257604897,
4.91605443614732));
#56902=CARTESIAN_POINT('Ctrl Pts',(-6.99999284818756,-16.7355860789202,
4.89563775208504));
#56903=CARTESIAN_POINT('Ctrl Pts',(-6.99999186150308,-16.5112404840694,
4.88171848973955));
#56904=CARTESIAN_POINT('Ctrl Pts',(-6.9999932006316,-16.2842668363519,4.87474450554359));
#56905=CARTESIAN_POINT('Ctrl Pts',(-6.99999413392928,-16.1260788998259,
4.8698840286538));
#56906=CARTESIAN_POINT('Ctrl Pts',(-6.99999620010592,-15.9666154533927,
4.86839729985613));
#56907=CARTESIAN_POINT('Ctrl Pts',(-6.99999999965515,-15.8060191439725,
4.87043884530665));
#56908=CARTESIAN_POINT('Ctrl Pts',(-7.00000506889193,-15.5917566964629,
4.87316260979731));
#56909=CARTESIAN_POINT('Ctrl Pts',(-7.00001329864027,-15.3754753370598,
4.88216671427478));
#56910=CARTESIAN_POINT('Ctrl Pts',(-7.00001657745847,-15.1576383201127,
4.89779557471497));
#56911=CARTESIAN_POINT('Ctrl Pts',(-7.00001838122166,-15.0378005094032,
4.90639341747505));
#56912=CARTESIAN_POINT('Ctrl Pts',(-7.00001867169788,-14.9174927908483,
4.91699624309555));
#56913=CARTESIAN_POINT('Ctrl Pts',(-7.00001598753836,-14.7967990235774,
4.92966193743282));
#56914=CARTESIAN_POINT('Origin',(-5.9999949808,-24.7867195890602,9.33250914740362));
#56915=CARTESIAN_POINT('Origin',(-6.,-24.7867243677925,9.33251101143268));
#56916=CARTESIAN_POINT('Ctrl Pts',(-7.10781849754849,-14.3668282424248,
7.15238423961458));
#56917=CARTESIAN_POINT('Ctrl Pts',(-7.10965591494416,-14.3272645751604,
7.23049518234384));
#56918=CARTESIAN_POINT('Ctrl Pts',(-7.09650767034188,-14.24557459556,7.40084939111339));
#56919=CARTESIAN_POINT('Ctrl Pts',(-7.01932069946779,-14.1324746587623,
7.66783513591697));
#56920=CARTESIAN_POINT('Ctrl Pts',(-6.87393093371095,-14.0363207135332,
7.93731276018294));
#56921=CARTESIAN_POINT('Ctrl Pts',(-6.66554647804556,-13.9714533100044,
8.17907214581632));
#56922=CARTESIAN_POINT('Ctrl Pts',(-6.44497304084988,-13.9492960538378,
8.34416343581852));
#56923=CARTESIAN_POINT('Ctrl Pts',(-6.29831086878765,-13.953178773167,8.41811502993441));
#56924=CARTESIAN_POINT('Ctrl Pts',(-6.24287185695061,-13.9569870722888,
8.44159546966128));
#56925=CARTESIAN_POINT('Ctrl Pts',(-6.81486607622036,-13.8484436165447,
6.89720921192514));
#56926=CARTESIAN_POINT('Ctrl Pts',(-6.81651062161729,-13.8136823565901,
6.96578564019607));
#56927=CARTESIAN_POINT('Ctrl Pts',(-6.80473712754382,-13.741909218052,7.11584392961594));
#56928=CARTESIAN_POINT('Ctrl Pts',(-6.7353831908826,-13.643029562488,7.35172242011219));
#56929=CARTESIAN_POINT('Ctrl Pts',(-6.60489822284063,-13.5599007723076,
7.58977897617138));
#56930=CARTESIAN_POINT('Ctrl Pts',(-6.41858681323947,-13.505035812957,7.80278611967251));
#56931=CARTESIAN_POINT('Ctrl Pts',(-6.22251417761433,-13.4875789839717,
7.94757981332609));
#56932=CARTESIAN_POINT('Ctrl Pts',(-6.09292712352008,-13.4919494706142,
8.01216517570182));
#56933=CARTESIAN_POINT('Ctrl Pts',(-6.04406306240266,-13.4955820115897,
8.0326475226799));
#56934=CARTESIAN_POINT('Ctrl Pts',(-7.05538134256208,-13.3135799379892,
6.62096627384063));
#56935=CARTESIAN_POINT('Ctrl Pts',(-7.05754284225227,-13.2686353298782,
6.70971021341623));
#56936=CARTESIAN_POINT('Ctrl Pts',(-7.04209110909695,-13.1762830686347,
6.90226166240641));
#56937=CARTESIAN_POINT('Ctrl Pts',(-6.9520659029282,-13.0486741093228,7.20315705962764));
#56938=CARTESIAN_POINT('Ctrl Pts',(-6.78206031637936,-12.9397227967065,
7.50801065543884));
#56939=CARTESIAN_POINT('Ctrl Pts',(-6.53634723568671,-12.8656252761574,
7.78417451392731));
#56940=CARTESIAN_POINT('Ctrl Pts',(-6.27298557965835,-12.8402907688676,
7.9756085032952));
#56941=CARTESIAN_POINT('Ctrl Pts',(-6.09561262360936,-12.8453667962591,
8.062709846792));
#56942=CARTESIAN_POINT('Ctrl Pts',(-6.02821754662008,-12.8501126777228,
8.09054371314276));
#56943=CARTESIAN_POINT('Ctrl Pts',(-7.66703304794012,-13.1269739075718,
6.51199213102435));
#56944=CARTESIAN_POINT('Ctrl Pts',(-7.67007102305416,-13.0637575588475,
6.63694586878494));
#56945=CARTESIAN_POINT('Ctrl Pts',(-7.64838054872756,-12.9342681399641,
6.90599900256435));
#56946=CARTESIAN_POINT('Ctrl Pts',(-7.52318691258873,-12.7544370130884,
7.32399978402674));
#56947=CARTESIAN_POINT('Ctrl Pts',(-7.28601524548368,-12.5983028452235,
7.74862544742454));
#56948=CARTESIAN_POINT('Ctrl Pts',(-6.93967858002702,-12.4887613326707,
8.13707451048743));
#56949=CARTESIAN_POINT('Ctrl Pts',(-6.56283725787951,-12.4483035827522,
8.41049095674551));
#56950=CARTESIAN_POINT('Ctrl Pts',(-6.30520108143084,-12.4538224255438,
8.53673601561792));
#56951=CARTESIAN_POINT('Ctrl Pts',(-6.20672732870885,-12.4602155439728,
8.57729019941276));
#56952=CARTESIAN_POINT('',(-6.26386059986259,-13.9442583573832,8.42071137118441));
#56953=CARTESIAN_POINT('',(-6.24994545432675,-12.4626524975511,8.55169100423493));
#56954=CARTESIAN_POINT('Origin',(-6.52772494237969,-13.2547636785371,9.09519306561096));
#56955=CARTESIAN_POINT('',(-7.00000135336109,-12.5220631623039,8.04447892959546));
#56956=CARTESIAN_POINT('Ctrl Pts',(-7.00000153557987,-12.5220620192528,
8.04447883033673));
#56957=CARTESIAN_POINT('Ctrl Pts',(-6.9736472239779,-12.5156013106946,8.0704984015701));
#56958=CARTESIAN_POINT('Ctrl Pts',(-6.94679742848067,-12.5096416804742,
8.09581844410209));
#56959=CARTESIAN_POINT('Ctrl Pts',(-6.91946610248342,-12.5041754138501,
8.12045448285676));
#56960=CARTESIAN_POINT('Ctrl Pts',(-6.87663070275667,-12.495608331672,8.15906565627172));
#56961=CARTESIAN_POINT('Ctrl Pts',(-6.83261494727981,-12.4882516839534,
8.19599819466153));
#56962=CARTESIAN_POINT('Ctrl Pts',(-6.78747035871098,-12.4820825574771,
8.23129874241077));
#56963=CARTESIAN_POINT('Ctrl Pts',(-6.74232577014216,-12.4759134310009,
8.26659929016002));
#56964=CARTESIAN_POINT('Ctrl Pts',(-6.69605167293783,-12.4709316730476,
8.30026835769235));
#56965=CARTESIAN_POINT('Ctrl Pts',(-6.64865479374424,-12.4671424045176,
8.33232175516477));
#56966=CARTESIAN_POINT('Ctrl Pts',(-6.60367902495548,-12.4635466980453,
8.36273781246942));
#56967=CARTESIAN_POINT('Ctrl Pts',(-6.55771208302904,-12.4610209442456,
8.39169360394873));
#56968=CARTESIAN_POINT('Ctrl Pts',(-6.51072389279704,-12.4595935857182,
8.41917670458322));
#56969=CARTESIAN_POINT('Ctrl Pts',(-6.50378457842987,-12.4593827904207,
8.42323546645818));
#56970=CARTESIAN_POINT('Ctrl Pts',(-6.49682294524356,-12.4591959993429,
8.42726204404947));
#56971=CARTESIAN_POINT('Ctrl Pts',(-6.48983885120465,-12.4590333548863,
8.43125632799246));
#56972=CARTESIAN_POINT('Ctrl Pts',(-6.44329072590013,-12.4579493496445,
8.45787773779083));
#56973=CARTESIAN_POINT('Ctrl Pts',(-6.39574619449289,-12.4579357605457,
8.48306789533459));
#56974=CARTESIAN_POINT('Ctrl Pts',(-6.34718929544507,-12.4590305456602,
8.50678437708271));
#56975=CARTESIAN_POINT('Ctrl Pts',(-6.31521661803976,-12.4597514156494,
8.52240068362187));
#56976=CARTESIAN_POINT('Ctrl Pts',(-6.28280462400267,-12.4609533800672,
8.53737727819511));
#56977=CARTESIAN_POINT('Ctrl Pts',(-6.24994591358957,-12.4626538072098,
8.55169190289375));
#56978=CARTESIAN_POINT('',(-7.000010673963,-13.9487142990898,6.9771195274227));
#56979=CARTESIAN_POINT('Ctrl Pts',(-7.000010673963,-13.9487142990898,6.9771195274227));
#56980=CARTESIAN_POINT('Ctrl Pts',(-7.,-13.8626205647626,7.0142375300983));
#56981=CARTESIAN_POINT('Ctrl Pts',(-7.,-13.7400113857744,7.0701796840634));
#56982=CARTESIAN_POINT('Ctrl Pts',(-7.,-13.62719934054,7.12651956295606));
#56983=CARTESIAN_POINT('Ctrl Pts',(-7.,-13.554168451218,7.16416786553508));
#56984=CARTESIAN_POINT('Ctrl Pts',(-7.,-13.5206011121911,7.18201203080913));
#56985=CARTESIAN_POINT('Ctrl Pts',(-7.,-13.3396119169715,7.28169559221322));
#56986=CARTESIAN_POINT('Ctrl Pts',(-7.,-13.2055602061295,7.36747030450435));
#56987=CARTESIAN_POINT('Ctrl Pts',(-7.,-12.8482282269687,7.63349452399642));
#56988=CARTESIAN_POINT('Ctrl Pts',(-7.,-12.6600994729296,7.82960565015868));
#56989=CARTESIAN_POINT('Ctrl Pts',(-7.000002992026,-12.522063284292,8.04447842282183));
#56990=CARTESIAN_POINT('Ctrl Pts',(-7.00001531395507,-13.9487142989349,
6.97711952775229));
#56991=CARTESIAN_POINT('Ctrl Pts',(-7.00001196725436,-13.9419375604996,
7.02105067161363));
#56992=CARTESIAN_POINT('Ctrl Pts',(-6.99838322763679,-13.9356769258173,
7.06398945097686));
#56993=CARTESIAN_POINT('Ctrl Pts',(-6.99539547590856,-13.9299187481022,
7.105781119514));
#56994=CARTESIAN_POINT('Ctrl Pts',(-6.99268063142182,-13.9246865339005,
7.14375545314008));
#56995=CARTESIAN_POINT('Ctrl Pts',(-6.98884285794656,-13.9198691503561,
7.18078335947894));
#56996=CARTESIAN_POINT('Ctrl Pts',(-6.98405836629357,-13.915452598832,7.21677715725527));
#56997=CARTESIAN_POINT('Ctrl Pts',(-6.97840508132026,-13.9102340665039,
7.25930689935957));
#56998=CARTESIAN_POINT('Ctrl Pts',(-6.97143142900756,-13.9055749039963,
7.30039272111852));
#56999=CARTESIAN_POINT('Ctrl Pts',(-6.96343342004341,-13.9014293624605,
7.3399541376309));
#57000=CARTESIAN_POINT('Ctrl Pts',(-6.95719888813531,-13.8981978693356,
7.37079267690755));
#57001=CARTESIAN_POINT('Ctrl Pts',(-6.95034090819598,-13.8952784336576,
7.40070575569444));
#57002=CARTESIAN_POINT('Ctrl Pts',(-6.94298357137251,-13.8926482456883,
7.42966983265612));
#57003=CARTESIAN_POINT('Ctrl Pts',(-6.93534013200227,-13.8899157783895,
7.45976022697728));
#57004=CARTESIAN_POINT('Ctrl Pts',(-6.92715768677458,-13.8874955281492,
7.488826375215));
#57005=CARTESIAN_POINT('Ctrl Pts',(-6.91856207099106,-13.8853606243187,
7.51685480666478));
#57006=CARTESIAN_POINT('Ctrl Pts',(-6.90689557450206,-13.8824630020109,
7.55489671143773));
#57007=CARTESIAN_POINT('Ctrl Pts',(-6.89447015028134,-13.880090679705,7.59102645975311));
#57008=CARTESIAN_POINT('Ctrl Pts',(-6.88159132787961,-13.8781602348909,
7.62525966990753));
#57009=CARTESIAN_POINT('Ctrl Pts',(-6.87269851637784,-13.87682726505,7.64889766067311));
#57010=CARTESIAN_POINT('Ctrl Pts',(-6.86358844439265,-13.8757050158038,
7.67163205004271));
#57011=CARTESIAN_POINT('Ctrl Pts',(-6.85434935575237,-13.8747664057238,
7.69347522038107));
#57012=CARTESIAN_POINT('Ctrl Pts',(-6.84893640315561,-13.8742164973868,
7.7062725914431));
#57013=CARTESIAN_POINT('Ctrl Pts',(-6.8434789870505,-13.8737296282504,7.71876415637358));
#57014=CARTESIAN_POINT('Ctrl Pts',(-6.83799343682602,-13.8733003913515,
7.73095321827998));
#57015=CARTESIAN_POINT('Ctrl Pts',(-6.83525066171379,-13.8730857729021,
7.73704774923319));
#57016=CARTESIAN_POINT('Ctrl Pts',(-6.83250084470304,-13.8728855666253,
7.74306665076591));
#57017=CARTESIAN_POINT('Ctrl Pts',(-6.82974592766377,-13.872699095121,7.74901040061493));
#57018=CARTESIAN_POINT('Ctrl Pts',(-6.82836846914414,-13.8726058593689,
7.75198227553944));
#57019=CARTESIAN_POINT('Ctrl Pts',(-6.82698973509903,-13.872516057556,7.75493536232424));
#57020=CARTESIAN_POINT('Ctrl Pts',(-6.82560996394253,-13.872429605776,7.75786972160125));
#57021=CARTESIAN_POINT('Ctrl Pts',(-6.82452960945506,-13.8723619144287,
7.76016731145725));
#57022=CARTESIAN_POINT('Ctrl Pts',(-6.82391452016856,-13.8723244082979,
7.76147074725261));
#57023=CARTESIAN_POINT('Ctrl Pts',(-6.82267100507654,-13.8722506715508,
7.76408867684986));
#57024=CARTESIAN_POINT('Ctrl Pts',(-6.8223263689862,-13.8722302356555,7.76481422736948));
#57025=CARTESIAN_POINT('Ctrl Pts',(-6.82193326623848,-13.8722071152214,
7.76564063362551));
#57026=CARTESIAN_POINT('Ctrl Pts',(-6.82146777483655,-13.8721802171765,
7.76661667804998));
#57027=CARTESIAN_POINT('Ctrl Pts',(-6.81268227350425,-13.8716725540741,
7.78503815598937));
#57028=CARTESIAN_POINT('Ctrl Pts',(-6.80362642075091,-13.8712922492689,
7.80321393195674));
#57029=CARTESIAN_POINT('Ctrl Pts',(-6.79431175107884,-13.8710418067265,
7.82113300705971));
#57030=CARTESIAN_POINT('Ctrl Pts',(-6.76482339153055,-13.8702489563092,
7.87786117327623));
#57031=CARTESIAN_POINT('Ctrl Pts',(-6.73274529262462,-13.8707559817329,
7.93201589777643));
#57032=CARTESIAN_POINT('Ctrl Pts',(-6.69853355487696,-13.8725797524819,
7.98334468488858));
#57033=CARTESIAN_POINT('Ctrl Pts',(-6.67146133661983,-13.8740229273399,
8.02396185955019));
#57034=CARTESIAN_POINT('Ctrl Pts',(-6.64305173670006,-13.8762911892378,
8.06280960604313));
#57035=CARTESIAN_POINT('Ctrl Pts',(-6.61350999833252,-13.8794004662696,
8.09976844127926));
#57036=CARTESIAN_POINT('Ctrl Pts',(-6.57430865524071,-13.8835264196638,
8.14881213540246));
#57037=CARTESIAN_POINT('Ctrl Pts',(-6.53311592434715,-13.8891322960673,
8.19452984729646));
#57038=CARTESIAN_POINT('Ctrl Pts',(-6.49047916504889,-13.8961820066511,
8.23675918782889));
#57039=CARTESIAN_POINT('Ctrl Pts',(-6.45748241493318,-13.9016378044732,
8.26944063501282));
#57040=CARTESIAN_POINT('Ctrl Pts',(-6.42361956793115,-13.9079589374026,
8.30003283848111));
#57041=CARTESIAN_POINT('Ctrl Pts',(-6.38912483192341,-13.9151350828458,
8.3284657400435));
#57042=CARTESIAN_POINT('Ctrl Pts',(-6.34811702764754,-13.923666180684,8.36226715432317));
#57043=CARTESIAN_POINT('Ctrl Pts',(-6.3062172665435,-13.9334050780639,8.39301733581296));
#57044=CARTESIAN_POINT('Ctrl Pts',(-6.26385533693063,-13.944272110215,8.42069791742242));
#57045=CARTESIAN_POINT('Ctrl Pts',(-6.22266624523242,-13.1134067202412,
7.49367548860228));
#57046=CARTESIAN_POINT('Ctrl Pts',(-6.22400178812049,-13.3673833259686,
7.81350053545753));
#57047=CARTESIAN_POINT('Ctrl Pts',(-6.22726137937113,-14.0755222713343,
8.61699794739643));
#57048=CARTESIAN_POINT('Ctrl Pts',(-6.23204990885402,-15.3875902517813,
9.75631894437));
#57049=CARTESIAN_POINT('Ctrl Pts',(-6.23570372463157,-17.0892601163741,
10.7961455412244));
#57050=CARTESIAN_POINT('Ctrl Pts',(-6.23759289250501,-18.9411594552768,
11.5416374931887));
#57051=CARTESIAN_POINT('Ctrl Pts',(-6.23804008865557,-20.8893388524382,
11.9701371034134));
#57052=CARTESIAN_POINT('Ctrl Pts',(-6.23649323743614,-22.7260228677799,
12.0627646689595));
#57053=CARTESIAN_POINT('Ctrl Pts',(-6.23490544880393,-23.8924620062907,
11.9504784886639));
#57054=CARTESIAN_POINT('Ctrl Pts',(-6.23413015604773,-24.3933788481534,
11.8700337879013));
#57055=CARTESIAN_POINT('Ctrl Pts',(-6.71588929286535,-13.2016794929268,
7.4236862634343));
#57056=CARTESIAN_POINT('Ctrl Pts',(-6.7170780227433,-13.4537900664687,7.74006838987067));
#57057=CARTESIAN_POINT('Ctrl Pts',(-6.71993255761527,-14.1564698677512,
8.53486272988918));
#57058=CARTESIAN_POINT('Ctrl Pts',(-6.72416341759993,-15.4574006729724,
9.66125897962087));
#57059=CARTESIAN_POINT('Ctrl Pts',(-6.72736708396084,-17.1431707229581,
10.6891581223397));
#57060=CARTESIAN_POINT('Ctrl Pts',(-6.72902314017145,-18.9767975202637,
11.4262596780397));
#57061=CARTESIAN_POINT('Ctrl Pts',(-6.729418137548,-20.9054811851494,11.8502316486358));
#57062=CARTESIAN_POINT('Ctrl Pts',(-6.72805060186563,-22.7235295527145,
11.9427141202896));
#57063=CARTESIAN_POINT('Ctrl Pts',(-6.72668232438883,-23.8785264249907,
11.8323462288572));
#57064=CARTESIAN_POINT('Ctrl Pts',(-6.72598917760879,-24.3745541293715,
11.7530879245913));
#57065=CARTESIAN_POINT('Ctrl Pts',(-7.02184873732211,-13.5171480157836,
7.17355847929394));
#57066=CARTESIAN_POINT('Ctrl Pts',(-7.02249169755403,-13.761025178858,7.47887640233898));
#57067=CARTESIAN_POINT('Ctrl Pts',(-7.02397836398706,-14.4407070320375,
8.24599948969163));
#57068=CARTESIAN_POINT('Ctrl Pts',(-7.02622840850876,-15.6982395182498,
9.33267651195289));
#57069=CARTESIAN_POINT('Ctrl Pts',(-7.02790175945528,-17.3268272034312,
10.324216053706));
#57070=CARTESIAN_POINT('Ctrl Pts',(-7.02876630077243,-19.0974433038976,
11.0353404974063));
#57071=CARTESIAN_POINT('Ctrl Pts',(-7.02897622079789,-20.9601356307836,
11.4446333981564));
#57072=CARTESIAN_POINT('Ctrl Pts',(-7.02824791678565,-22.715199269257,11.5344330888327));
#57073=CARTESIAN_POINT('Ctrl Pts',(-7.02756296992534,-23.8309176176107,
11.428361781308));
#57074=CARTESIAN_POINT('Ctrl Pts',(-7.02718428486759,-24.3100043035356,
11.3520791719536));
#57075=CARTESIAN_POINT('Ctrl Pts',(-6.99898915412488,-13.9127665915938,
6.85988131050602));
#57076=CARTESIAN_POINT('Ctrl Pts',(-6.99894179668946,-14.145881846675,7.15167007590343));
#57077=CARTESIAN_POINT('Ctrl Pts',(-6.99873531343826,-14.7957492487078,
7.88504931885052));
#57078=CARTESIAN_POINT('Ctrl Pts',(-6.99850468231058,-15.9978536408711,
8.92372179840947));
#57079=CARTESIAN_POINT('Ctrl Pts',(-6.99828080313005,-17.5546304272577,
9.87141292198114));
#57080=CARTESIAN_POINT('Ctrl Pts',(-6.99816433581835,-19.2468664594383,
10.5510790379293));
#57081=CARTESIAN_POINT('Ctrl Pts',(-6.99814256681603,-21.0278289481731,
10.9423825331985));
#57082=CARTESIAN_POINT('Ctrl Pts',(-6.99821545410145,-22.7049144947482,
11.0282138212458));
#57083=CARTESIAN_POINT('Ctrl Pts',(-6.99835921777661,-23.7718253340107,
10.9268165340741));
#57084=CARTESIAN_POINT('Ctrl Pts',(-6.99838071860773,-24.2298152555024,
10.8539128099021));
#57085=CARTESIAN_POINT('',(-7.00000355772208,-24.1259406808709,10.9277699403668));
#57086=CARTESIAN_POINT('Ctrl Pts',(-7.00001601661638,-13.9487142989383,
6.97711952757068));
#57087=CARTESIAN_POINT('Ctrl Pts',(-7.0000208899967,-14.0875641914622,7.14852817466841));
#57088=CARTESIAN_POINT('Ctrl Pts',(-7.00001598309392,-14.2303294492748,
7.31421349415626));
#57089=CARTESIAN_POINT('Ctrl Pts',(-7.00000988157693,-14.3764171187408,
7.47407283197781));
#57090=CARTESIAN_POINT('Ctrl Pts',(-7.00000652467739,-14.4567908408787,
7.56202337596396));
#57091=CARTESIAN_POINT('Ctrl Pts',(-7.00000279094487,-14.5381709421536,
7.64821104957978));
#57092=CARTESIAN_POINT('Ctrl Pts',(-6.99999999965532,-14.6204637846073,
7.73262309097843));
#57093=CARTESIAN_POINT('Ctrl Pts',(-6.99999455422719,-14.7810059823021,
7.89729955899171));
#57094=CARTESIAN_POINT('Ctrl Pts',(-6.99999266080992,-14.945019436017,8.05521668450506));
#57095=CARTESIAN_POINT('Ctrl Pts',(-6.99999257345228,-15.1118937759786,
8.20640356290913));
#57096=CARTESIAN_POINT('Ctrl Pts',(-6.9999924848297,-15.2811844415535,8.35977961387709));
#57097=CARTESIAN_POINT('Ctrl Pts',(-6.99999425319344,-15.4534194630651,
8.50622915340521));
#57098=CARTESIAN_POINT('Ctrl Pts',(-6.99999619757815,-15.6280064747247,
8.64581249887252));
#57099=CARTESIAN_POINT('Ctrl Pts',(-6.99999754424659,-15.748924324796,8.74248703313042));
#57100=CARTESIAN_POINT('Ctrl Pts',(-6.99999897835357,-15.8709713329882,
8.83586857884188));
#57101=CARTESIAN_POINT('Ctrl Pts',(-6.99999998662269,-15.9939629279854,
8.9259851708091));
#57102=CARTESIAN_POINT('Ctrl Pts',(-7.00000143709205,-16.1708953932809,
9.05562452365383));
#57103=CARTESIAN_POINT('Ctrl Pts',(-7.00000201442324,-16.3497802017751,
9.17850669010871));
#57104=CARTESIAN_POINT('Ctrl Pts',(-7.00000210876028,-16.5300360475593,
9.29479664869584));
#57105=CARTESIAN_POINT('Ctrl Pts',(-7.00000220461145,-16.7131850374667,
9.41295308550352));
#57106=CARTESIAN_POINT('Ctrl Pts',(-7.00000180216989,-16.8977494586252,
9.52430405378974));
#57107=CARTESIAN_POINT('Ctrl Pts',(-7.00000129011899,-17.0831708595521,
9.62904042803331));
#57108=CARTESIAN_POINT('Ctrl Pts',(-7.00000086166997,-17.2383187546504,
9.71667663357862));
#57109=CARTESIAN_POINT('Ctrl Pts',(-7.00000035619232,-17.3940675908991,
9.79968217694013));
#57110=CARTESIAN_POINT('Ctrl Pts',(-6.99999998816673,-17.5501167583814,
9.87817778675338));
#57111=CARTESIAN_POINT('Ctrl Pts',(-6.99999970373341,-17.6707213695673,
9.93884413091956));
#57112=CARTESIAN_POINT('Ctrl Pts',(-6.99999950019767,-17.7915058619037,
9.99681685260602));
#57113=CARTESIAN_POINT('Ctrl Pts',(-6.99999936067302,-17.9123403031843,
10.0521635783821));
#57114=CARTESIAN_POINT('Ctrl Pts',(-6.99999924478736,-18.012702337443,10.0981331705744));
#57115=CARTESIAN_POINT('Ctrl Pts',(-6.99999917321303,-18.113098981996,10.1422912426454));
#57116=CARTESIAN_POINT('Ctrl Pts',(-6.99999913936356,-18.2134600364446,
10.1846774364508));
#57117=CARTESIAN_POINT('Ctrl Pts',(-6.99999912243883,-18.263640563669,10.2058705333535));
#57118=CARTESIAN_POINT('Ctrl Pts',(-6.99999911498667,-18.3138121933672,
10.2266206606898));
#57119=CARTESIAN_POINT('Ctrl Pts',(-6.99999911640001,-18.363966570749,10.2469328594148));
#57120=CARTESIAN_POINT('Ctrl Pts',(-6.99999911710669,-18.38904375944,10.2570889587773));
#57121=CARTESIAN_POINT('Ctrl Pts',(-6.99999912003194,-18.4141166350518,
10.267135575987));
#57122=CARTESIAN_POINT('Ctrl Pts',(-6.99999912511209,-18.4391841642749,
10.2770733432481));
#57123=CARTESIAN_POINT('Ctrl Pts',(-6.99999912765217,-18.4517179288864,
10.2820422268787));
#57124=CARTESIAN_POINT('Ctrl Pts',(-6.9999991307311,-18.4642503569007,10.2869838980222));
#57125=CARTESIAN_POINT('Ctrl Pts',(-6.99999913434161,-18.4767813206209,
10.2918984359962));
#57126=CARTESIAN_POINT('Ctrl Pts',(-6.99999913749792,-18.4877358923424,
10.2961947263628));
#57127=CARTESIAN_POINT('Ctrl Pts',(-6.99999914056844,-18.4972872792251,
10.2999248791717));
#57128=CARTESIAN_POINT('Ctrl Pts',(-6.99999914483372,-18.5091123692525,
10.304519538847));
#57129=CARTESIAN_POINT('Ctrl Pts',(-6.99999914544751,-18.51081403115,10.3051807225913));
#57130=CARTESIAN_POINT('Ctrl Pts',(-6.99999914608798,-18.5125628082469,
10.3058597278899));
#57131=CARTESIAN_POINT('Ctrl Pts',(-6.99999914676108,-18.5143696916372,
10.3065607298132));
#57132=CARTESIAN_POINT('Ctrl Pts',(-6.99999923697285,-18.7565377825937,
10.4005127238446));
#57133=CARTESIAN_POINT('Ctrl Pts',(-6.99999952144574,-19.0001638637106,
10.4851669222284));
#57134=CARTESIAN_POINT('Ctrl Pts',(-6.99999999018471,-19.244534524912,10.5606726979753));
#57135=CARTESIAN_POINT('Ctrl Pts',(-7.00000044364542,-19.4809400670551,
10.6337174070357));
#57136=CARTESIAN_POINT('Ctrl Pts',(-7.00000106797163,-19.7180423326575,
10.6982012217175));
#57137=CARTESIAN_POINT('Ctrl Pts',(-7.0000014259335,-19.9551820387299,10.7543686705225));
#57138=CARTESIAN_POINT('Ctrl Pts',(-7.00000178765883,-20.1948149383802,
10.8111266417876));
#57139=CARTESIAN_POINT('Ctrl Pts',(-7.00000187627607,-20.434486106489,10.8593924797692));
#57140=CARTESIAN_POINT('Ctrl Pts',(-7.00000131559751,-20.6735682031901,
10.8994248121704));
#57141=CARTESIAN_POINT('Ctrl Pts',(-7.0000010387385,-20.7916252129104,10.9191924882977));
#57142=CARTESIAN_POINT('Ctrl Pts',(-7.00000060481346,-20.9095393943468,
10.9369526723741));
#57143=CARTESIAN_POINT('Ctrl Pts',(-6.99999997635832,-21.0272398537476,
10.9527370359073));
#57144=CARTESIAN_POINT('Ctrl Pts',(-6.9999988792805,-21.232706487677,10.980291389224));
#57145=CARTESIAN_POINT('Ctrl Pts',(-6.99999719586413,-21.4375204945477,
11.0018248526799));
#57146=CARTESIAN_POINT('Ctrl Pts',(-6.99999590263476,-21.6413538432379,
11.0175572522402));
#57147=CARTESIAN_POINT('Ctrl Pts',(-6.9999956817133,-21.6761745497693,11.0202448069099));
#57148=CARTESIAN_POINT('Ctrl Pts',(-6.99999546002091,-21.7128790072846,
11.0229065232472));
#57149=CARTESIAN_POINT('Ctrl Pts',(-6.99999525388523,-21.7501370397694,
11.0254108052772));
#57150=CARTESIAN_POINT('Ctrl Pts',(-6.99999512029735,-21.774282404631,11.0270337252034));
#57151=CARTESIAN_POINT('Ctrl Pts',(-6.9999949932366,-21.7986601648793,11.0285915128656));
#57152=CARTESIAN_POINT('Ctrl Pts',(-6.99999487630705,-21.8229073894779,
11.030060139636));
#57153=CARTESIAN_POINT('Ctrl Pts',(-6.99999457894682,-21.8845698234527,
11.0337949630133));
#57154=CARTESIAN_POINT('Ctrl Pts',(-6.99999434327587,-21.9460668090055,
11.0369990881757));
#57155=CARTESIAN_POINT('Ctrl Pts',(-6.99999419420496,-22.0073890961152,
11.0396820791216));
#57156=CARTESIAN_POINT('Ctrl Pts',(-6.99999365475099,-22.2293006052878,
11.0493912174785));
#57157=CARTESIAN_POINT('Ctrl Pts',(-6.99999426200478,-22.448925295387,11.0522756893275));
#57158=CARTESIAN_POINT('Ctrl Pts',(-6.99999708872338,-22.6658896614926,
11.048779376235));
#57159=CARTESIAN_POINT('Ctrl Pts',(-6.99999738650878,-22.6887461356942,
11.0484110512818));
#57160=CARTESIAN_POINT('Ctrl Pts',(-6.9999977087728,-22.7115731328884,11.0479719059811));
#57161=CARTESIAN_POINT('Ctrl Pts',(-6.99999805666166,-22.7343702493888,
11.0474624543948));
#57162=CARTESIAN_POINT('Ctrl Pts',(-6.99999863110505,-22.7720134588844,
11.0466212342873));
#57163=CARTESIAN_POINT('Ctrl Pts',(-6.99999927542386,-22.8095751947521,
11.0455883208263));
#57164=CARTESIAN_POINT('Ctrl Pts',(-6.99999999465561,-22.8470536771216,
11.0443660224837));
#57165=CARTESIAN_POINT('Ctrl Pts',(-7.00000393348179,-23.0523021636611,
11.037672184605));
#57166=CARTESIAN_POINT('Ctrl Pts',(-7.00001006471103,-23.2550496791979,
11.0252996505177));
#57167=CARTESIAN_POINT('Ctrl Pts',(-7.00001375741216,-23.4549524564073,
11.0076812098584));
#57168=CARTESIAN_POINT('Ctrl Pts',(-7.00001750460198,-23.6578049557541,
10.9898027953));
#57169=CARTESIAN_POINT('Ctrl Pts',(-7.00001874206956,-23.8577282246578,
10.9665225331668));
#57170=CARTESIAN_POINT('Ctrl Pts',(-7.00001328593478,-24.0544142486451,
10.9382773269549));
#57171=CARTESIAN_POINT('Ctrl Pts',(-7.00001262322331,-24.0783040696869,
10.9348466158753));
#57172=CARTESIAN_POINT('Ctrl Pts',(-7.00001186252947,-24.1021461920723,
10.931342638763));
#57173=CARTESIAN_POINT('Ctrl Pts',(-7.00001099698697,-24.1259401133989,
10.9277661632342));
#57174=CARTESIAN_POINT('',(-6.271594443024,-24.2690120587724,11.8794941632625));
#57175=CARTESIAN_POINT('Origin',(-5.99998362344489,-24.1259473025315,10.9277594521136));
#57176=CARTESIAN_POINT('Ctrl Pts',(-6.26386059994277,-13.9442583574975,
8.42071137126985));
#57177=CARTESIAN_POINT('Ctrl Pts',(-6.26455151926992,-14.1129907025116,
8.59292006661441));
#57178=CARTESIAN_POINT('Ctrl Pts',(-6.26520985451036,-14.2852415147495,
8.75834742231281));
#57179=CARTESIAN_POINT('Ctrl Pts',(-6.26583560625273,-14.4604056907354,
8.91699490798369));
#57180=CARTESIAN_POINT('Ctrl Pts',(-6.2664706593002,-14.6381735437629,9.07800056314788));
#57181=CARTESIAN_POINT('Ctrl Pts',(-6.26707215299456,-14.8189420279879,
9.23202334515509));
#57182=CARTESIAN_POINT('Ctrl Pts',(-6.26764008795109,-15.002122358651,9.37909676806481));
#57183=CARTESIAN_POINT('Ctrl Pts',(-6.2681246797852,-15.1584214055542,9.50458751121598));
#57184=CARTESIAN_POINT('Ctrl Pts',(-6.26858483953038,-15.3164771401929,
9.62501942153129));
#57185=CARTESIAN_POINT('Ctrl Pts',(-6.26902056756885,-15.4759481442486,
9.74043079561972));
#57186=CARTESIAN_POINT('Ctrl Pts',(-6.26953467271229,-15.6641041869533,
9.87660192942662));
#57187=CARTESIAN_POINT('Ctrl Pts',(-6.27001476628493,-15.854228787839,10.0057843668122));
#57188=CARTESIAN_POINT('Ctrl Pts',(-6.27046084891459,-16.0457320728812,
10.1281573929876));
#57189=CARTESIAN_POINT('Ctrl Pts',(-6.27062083229436,-16.1144129421647,
10.1720453388927));
#57190=CARTESIAN_POINT('Ctrl Pts',(-6.27077644107981,-16.1832716087534,
10.2150575890123));
#57191=CARTESIAN_POINT('Ctrl Pts',(-6.27092767529992,-16.2522824065319,
10.2572029123285));
#57192=CARTESIAN_POINT('Ctrl Pts',(-6.27136815555626,-16.4532811875826,
10.3799541177375));
#57193=CARTESIAN_POINT('Ctrl Pts',(-6.27177152514005,-16.6555663828579,
10.4953498370541));
#57194=CARTESIAN_POINT('Ctrl Pts',(-6.27213778405132,-16.8585418317145,
10.6036186785427));
#57195=CARTESIAN_POINT('Ctrl Pts',(-6.27250404296258,-17.0615172805711,
10.7118875200312));
#57196=CARTESIAN_POINT('Ctrl Pts',(-6.27283319120131,-17.2651831715053,
10.8130295873899));
#57197=CARTESIAN_POINT('Ctrl Pts',(-6.2731252287675,-17.4689976408962,10.9072900318684));
#57198=CARTESIAN_POINT('Ctrl Pts',(-6.27334042212229,-17.6191821530989,
10.9767476072619));
#57199=CARTESIAN_POINT('Ctrl Pts',(-6.27353526468669,-17.7691757844474,
11.0423478542931));
#57200=CARTESIAN_POINT('Ctrl Pts',(-6.27370997818747,-17.9190755247098,
11.1043414442314));
#57201=CARTESIAN_POINT('Ctrl Pts',(-6.27388469168824,-18.0689752649722,
11.1663350341698));
#57202=CARTESIAN_POINT('Ctrl Pts',(-6.27403927612539,-18.2187815399094,
11.2247220111681));
#57203=CARTESIAN_POINT('Ctrl Pts',(-6.27417395322568,-18.3686262123569,
11.2797074203491));
#57204=CARTESIAN_POINT('Ctrl Pts',(-6.27427013793896,-18.4756434173988,
11.318977317053));
#57205=CARTESIAN_POINT('Ctrl Pts',(-6.27435616863818,-18.5826809229142,
11.3565113020647));
#57206=CARTESIAN_POINT('Ctrl Pts',(-6.27443212609425,-18.6897917166758,
11.3923810248371));
#57207=CARTESIAN_POINT('Ctrl Pts',(-6.27457884517869,-18.8966864496993,
11.4616668218703));
#57208=CARTESIAN_POINT('Ctrl Pts',(-6.27469165501223,-19.1080556828696,
11.5261455889694));
#57209=CARTESIAN_POINT('Ctrl Pts',(-6.2747705555949,-19.3236952442391,11.5853118140797));
#57210=CARTESIAN_POINT('Ctrl Pts',(-6.27484862874764,-19.5370733948855,
11.6438575633595));
#57211=CARTESIAN_POINT('Ctrl Pts',(-6.27489350013246,-19.7546328883749,
11.6972016144136));
#57212=CARTESIAN_POINT('Ctrl Pts',(-6.27490516974936,-19.9761300584837,
11.744833566385));
#57213=CARTESIAN_POINT('Ctrl Pts',(-6.2749166457757,-20.1939527499269,11.7916753385486));
#57214=CARTESIAN_POINT('Ctrl Pts',(-6.27489601248373,-20.4155836081791,
11.8329929400541));
#57215=CARTESIAN_POINT('Ctrl Pts',(-6.27484326987345,-20.640745185411,11.8682810499045));
#57216=CARTESIAN_POINT('Ctrl Pts',(-6.27479056731688,-20.865735770765,11.9035423613098));
#57217=CARTESIAN_POINT('Ctrl Pts',(-6.2747058041923,-21.0942518881818,11.9327833696204));
#57218=CARTESIAN_POINT('Ctrl Pts',(-6.2745889804997,-21.3259688314451,11.955479670973));
#57219=CARTESIAN_POINT('Ctrl Pts',(-6.27454781420096,-21.4076211803764,
11.9634773870286));
#57220=CARTESIAN_POINT('Ctrl Pts',(-6.27450266694103,-21.4896705313667,
11.9706622510988));
#57221=CARTESIAN_POINT('Ctrl Pts',(-6.27445353870782,-21.5721011963865,
11.9770107061869));
#57222=CARTESIAN_POINT('Ctrl Pts',(-6.2743162410566,-21.8024684609395,11.9947526015415));
#57223=CARTESIAN_POINT('Ctrl Pts',(-6.27414785108124,-22.0358175732131,
12.0059621189159));
#57224=CARTESIAN_POINT('Ctrl Pts',(-6.27394836851762,-22.2717646560156,
12.0102364739125));
#57225=CARTESIAN_POINT('Ctrl Pts',(-6.27375072701035,-22.5055341456103,
12.014471380206));
#57226=CARTESIAN_POINT('Ctrl Pts',(-6.27352256418332,-22.7418539653979,
12.0118985200148));
#57227=CARTESIAN_POINT('Ctrl Pts',(-6.27326387977963,-22.9803003340606,
12.0021219084666));
#57228=CARTESIAN_POINT('Ctrl Pts',(-6.27300884334362,-23.2153841318392,
11.9924831667023));
#57229=CARTESIAN_POINT('Ctrl Pts',(-6.27272414009183,-23.4525349673461,
11.9758423891121));
#57230=CARTESIAN_POINT('Ctrl Pts',(-6.27240976977808,-23.6912965484798,
11.9518163423101));
#57231=CARTESIAN_POINT('Ctrl Pts',(-6.27215746674537,-23.8829185572408,
11.9325338458174));
#57232=CARTESIAN_POINT('Ctrl Pts',(-6.27188605478029,-24.0755771485926,
11.908494328387));
#57233=CARTESIAN_POINT('Ctrl Pts',(-6.27159553375559,-24.2690121689631,
11.8794980525033));
#57234=CARTESIAN_POINT('Origin',(-5.999994993365,-24.1259380195517,10.9277770074801));
#57235=CARTESIAN_POINT('',(-5.98852246669737,-25.0410395151948,11.3308498388632));
#57236=CARTESIAN_POINT('Origin',(-5.999994993365,-24.1259380195517,10.9277770074801));
#57237=CARTESIAN_POINT('Origin',(-6.,-24.1259427050578,10.9277790633915));
#57238=CARTESIAN_POINT('Ctrl Pts',(-5.98841833134947,-25.040839011132,11.3313022852623));
#57239=CARTESIAN_POINT('Ctrl Pts',(-5.98810627250653,-25.0938945818823,
11.2108442590279));
#57240=CARTESIAN_POINT('Ctrl Pts',(-5.98726405053642,-25.2768814418996,
10.7897532298672));
#57241=CARTESIAN_POINT('Ctrl Pts',(-5.98726405053548,-25.5029619538456,
10.2439465916472));
#57242=CARTESIAN_POINT('Ctrl Pts',(-5.98810627252386,-25.6713270271153,
9.81679901787702));
#57243=CARTESIAN_POINT('Ctrl Pts',(-5.98841833138214,-25.71898776185,9.69410637308692));
#57244=CARTESIAN_POINT('Ctrl Pts',(-6.58019637691559,-25.0471116824598,
11.3340652823765));
#57245=CARTESIAN_POINT('Ctrl Pts',(-6.57988216951981,-25.1003453872547,
11.2136609948753));
#57246=CARTESIAN_POINT('Ctrl Pts',(-6.57903377822269,-25.2838224184272,
10.7926927033354));
#57247=CARTESIAN_POINT('Ctrl Pts',(-6.57903377822185,-25.5099484870406,
10.2467760815894));
#57248=CARTESIAN_POINT('Ctrl Pts',(-6.57988216953611,-25.6778801683539,
9.81936869307563));
#57249=CARTESIAN_POINT('Ctrl Pts',(-6.58019637694761,-25.725376944262,9.69658808751447));
#57250=CARTESIAN_POINT('Ctrl Pts',(-7.0007967752053,-24.6661026364245,11.1662377678248));
#57251=CARTESIAN_POINT('Ctrl Pts',(-7.00061249054646,-24.7189023956179,
11.0471442791618));
#57252=CARTESIAN_POINT('Ctrl Pts',(-7.00011449005887,-24.9007955979718,
10.6307100883018));
#57253=CARTESIAN_POINT('Ctrl Pts',(-7.00011449005883,-25.1245686193591,
10.0904742250701));
#57254=CARTESIAN_POINT('Ctrl Pts',(-7.00061249055608,-25.2904141434231,
9.66739286602032));
#57255=CARTESIAN_POINT('Ctrl Pts',(-7.00079677522358,-25.3372908904342,
9.54584598112046));
#57256=CARTESIAN_POINT('Ctrl Pts',(-6.99999917318215,-24.1245144769952,
10.9276780913239));
#57257=CARTESIAN_POINT('Ctrl Pts',(-6.99999957776327,-24.1765264223433,
10.8103725336039));
#57258=CARTESIAN_POINT('Ctrl Pts',(-7.00000004362099,-24.3557042137786,
10.4001860031049));
#57259=CARTESIAN_POINT('Ctrl Pts',(-7.00000004362179,-24.5761256613181,
9.86804155492472));
#57260=CARTESIAN_POINT('Ctrl Pts',(-6.99999957776352,-24.739473507827,9.45129804439077));
#57261=CARTESIAN_POINT('Ctrl Pts',(-6.99999917318139,-24.7856430652418,
9.33157248614975));
#57262=CARTESIAN_POINT('Origin',(-5.98852353414946,11.4730434400575,-4.75229019210214));
#57263=CARTESIAN_POINT('Origin',(-7.00021006969032,11.4504602414792,-4.74293587756365));
#57264=CARTESIAN_POINT('Ctrl Pts',(-6.05508738338625,-24.9010197753632,
11.6467810610876));
#57265=CARTESIAN_POINT('Ctrl Pts',(-4.03672492225717,-24.6398368704069,
12.1727625868536));
#57266=CARTESIAN_POINT('Ctrl Pts',(7.59697586626834E-7,-24.4085091422409,
12.7121411857612));
#57267=CARTESIAN_POINT('Ctrl Pts',(4.03672644165275,-24.6398369574816,12.1727623838323));
#57268=CARTESIAN_POINT('Ctrl Pts',(6.05508966247912,-24.9010200702845,11.646780467159));
#57269=CARTESIAN_POINT('Ctrl Pts',(-6.05508738338625,-25.2386170700518,
10.8984824909014));
#57270=CARTESIAN_POINT('Ctrl Pts',(-4.03672492225717,-25.1429604961832,
11.0706884016279));
#57271=CARTESIAN_POINT('Ctrl Pts',(7.59697586626834E-7,-25.1800058610512,
11.3017462712826));
#57272=CARTESIAN_POINT('Ctrl Pts',(4.03672644165275,-25.1429604822486,11.0706883146625));
#57273=CARTESIAN_POINT('Ctrl Pts',(6.05508966247912,-25.2386171780669,10.8984822964536));
#57274=CARTESIAN_POINT('Ctrl Pts',(-6.05508738338625,-25.5530349402587,
10.1393926838645));
#57275=CARTESIAN_POINT('Ctrl Pts',(-4.03672492225717,-25.6072797194157,
9.94969240521292));
#57276=CARTESIAN_POINT('Ctrl Pts',(7.59697586626834E-7,-25.7969468737938,
9.81219748812645));
#57277=CARTESIAN_POINT('Ctrl Pts',(4.03672644165275,-25.6072796480323,9.94969245696381));
#57278=CARTESIAN_POINT('Ctrl Pts',(6.05508966247912,-25.5530348790098,10.1393928980646));
#57279=CARTESIAN_POINT('Ctrl Pts',(-6.05508738338625,-25.8434316995194,
9.37154365087387));
#57280=CARTESIAN_POINT('Ctrl Pts',(-4.03672492225717,-26.0307798045846,
8.81463859944452));
#57281=CARTESIAN_POINT('Ctrl Pts',(7.59697586626834E-7,-26.2486273875397,
8.2693384925856));
#57282=CARTESIAN_POINT('Ctrl Pts',(4.03672644165275,-26.0307797225905,8.81463880469617));
#57283=CARTESIAN_POINT('Ctrl Pts',(6.05508966247912,-25.8434314879758,9.37154427972115));
#57284=CARTESIAN_POINT('Ctrl Pts',(-5.98852262888505,-25.0410393032183,
11.3308502499282));
#57285=CARTESIAN_POINT('Ctrl Pts',(-5.93906438611487,-25.0335296633685,
11.3464916934807));
#57286=CARTESIAN_POINT('Ctrl Pts',(-5.88263517116821,-25.025051050658,11.3641929089859));
#57287=CARTESIAN_POINT('Ctrl Pts',(-5.81916415490276,-25.0156980212809,
11.3837859022183));
#57288=CARTESIAN_POINT('Ctrl Pts',(-5.7580450642156,-25.0066915694493,11.4026528749038));
#57289=CARTESIAN_POINT('Ctrl Pts',(-5.69039610968652,-24.9968744776098,
11.4232739318758));
#57290=CARTESIAN_POINT('Ctrl Pts',(-5.61614355559872,-24.9863500316491,
11.4454588047106));
#57291=CARTESIAN_POINT('Ctrl Pts',(-5.5404621080218,-24.9756230564625,11.4680705964675));
#57292=CARTESIAN_POINT('Ctrl Pts',(-5.45792024476691,-24.9641612467195,
11.4923073176096));
#57293=CARTESIAN_POINT('Ctrl Pts',(-5.36843222079314,-24.9520928381922,
11.5179224145699));
#57294=CARTESIAN_POINT('Ctrl Pts',(-5.32368820880625,-24.9460586339285,
11.5307299630501));
#57295=CARTESIAN_POINT('Ctrl Pts',(-5.27720755800021,-24.9398730715649,
11.543881375116));
#57296=CARTESIAN_POINT('Ctrl Pts',(-5.22897913546587,-24.9335538910092,
11.5573412753069));
#57297=CARTESIAN_POINT('Ctrl Pts',(-5.2048649241987,-24.9303943007313,11.5640712254024));
#57298=CARTESIAN_POINT('Ctrl Pts',(-5.18031377002017,-24.9272013022212,
11.5708782958756));
#57299=CARTESIAN_POINT('Ctrl Pts',(-5.155324265948,-24.9239772467556,11.57775769834));
#57300=CARTESIAN_POINT('Ctrl Pts',(-5.13033476187583,-24.92075319129,11.5846371008043));
#57301=CARTESIAN_POINT('Ctrl Pts',(-5.10370559285897,-24.9173455615374,
11.5919148457444));
#57302=CARTESIAN_POINT('Ctrl Pts',(-5.07903930494025,-24.9142142529198,
11.5986080780921));
#57303=CARTESIAN_POINT('Ctrl Pts',(-5.0641312898593,-24.9123217267218,11.602653389211));
#57304=CARTESIAN_POINT('Ctrl Pts',(-5.04933271581953,-24.9104524028187,
11.6066511137227));
#57305=CARTESIAN_POINT('Ctrl Pts',(-5.03464390372513,-24.9086058757351,
11.610601946104));
#57306=CARTESIAN_POINT('Ctrl Pts',(-4.9171682275508,-24.8938380363538,11.6421992395044));
#57307=CARTESIAN_POINT('Ctrl Pts',(-4.80671569496028,-24.8805262788085,
11.670799962657));
#57308=CARTESIAN_POINT('Ctrl Pts',(-4.70342530185199,-24.8684850080852,
11.6967442810817));
#57309=CARTESIAN_POINT('Ctrl Pts',(-4.60047418857305,-24.8564832895424,
11.7226033797327));
#57310=CARTESIAN_POINT('Ctrl Pts',(-4.50463793164033,-24.8457437447952,
11.7458237648518));
#57311=CARTESIAN_POINT('Ctrl Pts',(-4.41602613739422,-24.8361073394874,
11.7667065466625));
#57312=CARTESIAN_POINT('Ctrl Pts',(-4.3839468301148,-24.8326187609119,11.774266546776));
#57313=CARTESIAN_POINT('Ctrl Pts',(-4.3528141094931,-24.8292749926518,11.7815198237035));
#57314=CARTESIAN_POINT('Ctrl Pts',(-4.32263238067729,-24.8260692849391,
11.7884794050893));
#57315=CARTESIAN_POINT('Ctrl Pts',(-4.28802312693375,-24.8223933142107,
11.7964599260065));
#57316=CARTESIAN_POINT('Ctrl Pts',(-4.25466435340653,-24.8188988662361,
11.8040542901814));
#57317=CARTESIAN_POINT('Ctrl Pts',(-4.22256207115286,-24.815576452521,11.811280988239));
#57318=CARTESIAN_POINT('Ctrl Pts',(-4.20651093002602,-24.8139152456634,
11.8148943372678));
#57319=CARTESIAN_POINT('Ctrl Pts',(-4.190773911718,-24.8122970494496,11.8184157707246));
#57320=CARTESIAN_POINT('Ctrl Pts',(-4.1753516959697,-24.8107207574243,11.8218474581548));
#57321=CARTESIAN_POINT('Ctrl Pts',(-4.16764058809556,-24.8099326114116,
11.8235633018699));
#57322=CARTESIAN_POINT('Ctrl Pts',(-4.16000818086133,-24.8091549415643,
11.8252567091328));
#57323=CARTESIAN_POINT('Ctrl Pts',(-4.15245455747703,-24.8083876122322,
11.8269279471741));
#57324=CARTESIAN_POINT('Ctrl Pts',(-4.14867774578487,-24.8080039475662,
11.8277635661948));
#57325=CARTESIAN_POINT('Ctrl Pts',(-4.1449206300552,-24.8076228680358,11.8285936429134));
#57326=CARTESIAN_POINT('Ctrl Pts',(-4.14118322045561,-24.807244356959,11.8294182102471));
#57327=CARTESIAN_POINT('Ctrl Pts',(-4.13931451565582,-24.8070551014206,
11.8298304939139));
#57328=CARTESIAN_POINT('Ctrl Pts',(-4.13745073738855,-24.806866487996,11.8302414002347));
#57329=CARTESIAN_POINT('Ctrl Pts',(-4.13559188690975,-24.8066785146178,
11.8306509332919));
#57330=CARTESIAN_POINT('Ctrl Pts',(-4.13373303643096,-24.8064905412396,
11.8310604663492));
#57331=CARTESIAN_POINT('Ctrl Pts',(-4.13363444561665,-24.8064804460971,
11.8310824417452));
#57332=CARTESIAN_POINT('Ctrl Pts',(-4.1300301200903,-24.8061165125615,11.8318754167459));
#57333=CARTESIAN_POINT('Ctrl Pts',(-4.08661760546933,-24.8017330933015,
11.8414264516245));
#57334=CARTESIAN_POINT('Ctrl Pts',(-4.04433457950343,-24.7975362580896,
11.85058237988));
#57335=CARTESIAN_POINT('Ctrl Pts',(-4.00318800196471,-24.7935150283471,
11.8593643927378));
#57336=CARTESIAN_POINT('Ctrl Pts',(-3.9000460902361,-24.783435032684,11.8813782186539));
#57337=CARTESIAN_POINT('Ctrl Pts',(-3.80404668802037,-24.7744568319423,
11.9010453906012));
#57338=CARTESIAN_POINT('Ctrl Pts',(-3.71528285757527,-24.7664251263882,
11.9186746484402));
#57339=CARTESIAN_POINT('Ctrl Pts',(-3.62703564900393,-24.7584401668426,
11.9362013007452));
#57340=CARTESIAN_POINT('Ctrl Pts',(-3.54593976635268,-24.7513907266947,
11.9517138490167));
#57341=CARTESIAN_POINT('Ctrl Pts',(-3.47206599162342,-24.7451472110363,
11.9654746815673));
#57342=CARTESIAN_POINT('Ctrl Pts',(-3.41362152570288,-24.7402077187812,
11.9763614206299));
#57343=CARTESIAN_POINT('Ctrl Pts',(-3.35969695735051,-24.7357731021218,
11.9861509848192));
#57344=CARTESIAN_POINT('Ctrl Pts',(-3.31031960817658,-24.7317894362562,
11.9949540482286));
#57345=CARTESIAN_POINT('Ctrl Pts',(-3.27705079452021,-24.7291053748482,
12.0008852592206));
#57346=CARTESIAN_POINT('Ctrl Pts',(-3.24584610621182,-24.7266262149396,
12.0063682825194));
#57347=CARTESIAN_POINT('Ctrl Pts',(-3.2167123660793,-24.7243378077796,12.0114324025904));
#57348=CARTESIAN_POINT('Ctrl Pts',(-3.20214549601304,-24.7231936041996,
12.0139644626259));
#57349=CARTESIAN_POINT('Ctrl Pts',(-3.18809636299643,-24.7220970904731,
12.0163917976402));
#57350=CARTESIAN_POINT('Ctrl Pts',(-3.174565693027,-24.7210467076192,12.018717647553));
#57351=CARTESIAN_POINT('Ctrl Pts',(-3.16780035804229,-24.7205215161922,
12.0198805725094));
#57352=CARTESIAN_POINT('Ctrl Pts',(-3.16116463881965,-24.7200078575691,
12.0210181262307));
#57353=CARTESIAN_POINT('Ctrl Pts',(-3.15465862315445,-24.7195055430928,
12.0221307017735));
#57354=CARTESIAN_POINT('Ctrl Pts',(-3.15140561532184,-24.7192543858547,
12.0226869895449));
#57355=CARTESIAN_POINT('Ctrl Pts',(-3.14818503337862,-24.7190060646578,
12.0232370327738));
#57356=CARTESIAN_POINT('Ctrl Pts',(-3.14499688787088,-24.7187605566668,
12.0237808790813));
#57357=CARTESIAN_POINT('Ctrl Pts',(-3.14180874236315,-24.7185150486758,
12.0243247253888));
#57358=CARTESIAN_POINT('Ctrl Pts',(-3.13695795616954,-24.7181421515035,
12.0251508337765));
#57359=CARTESIAN_POINT('Ctrl Pts',(-3.13552977107616,-24.718032449711,12.0253938744076));
#57360=CARTESIAN_POINT('Ctrl Pts',(-3.11970258360824,-24.7168167313537,
12.0280872575323));
#57361=CARTESIAN_POINT('Ctrl Pts',(-3.0967945756905,-24.7150575346586,12.0319848511427));
#57362=CARTESIAN_POINT('Ctrl Pts',(-3.06678983441689,-24.7127900582804,
12.037012281578));
#57363=CARTESIAN_POINT('Ctrl Pts',(-3.03690027360432,-24.7105312861591,
12.0420204130049));
#57364=CARTESIAN_POINT('Ctrl Pts',(-2.99996827922771,-24.707768137808,12.0481497555868));
#57365=CARTESIAN_POINT('Ctrl Pts',(-2.95596932035526,-24.7045569191481,
12.0552806302816));
#57366=CARTESIAN_POINT('Ctrl Pts',(-2.93821869684115,-24.703261408188,12.0581574590812));
#57367=CARTESIAN_POINT('Ctrl Pts',(-2.91931777485785,-24.7018932144384,
12.0611967667851));
#57368=CARTESIAN_POINT('Ctrl Pts',(-2.89926458877209,-24.7004570277544,
12.0643885313884));
#57369=CARTESIAN_POINT('Ctrl Pts',(-2.84971550087531,-24.6969083776826,
12.0722750100853));
#57370=CARTESIAN_POINT('Ctrl Pts',(-2.79313189875029,-24.6929431371324,
12.0810955571872));
#57371=CARTESIAN_POINT('Ctrl Pts',(-2.72948003773908,-24.6886468787094,
12.0906663764175));
#57372=CARTESIAN_POINT('Ctrl Pts',(-2.66624670467554,-24.6843788693304,
12.100174264961));
#57373=CARTESIAN_POINT('Ctrl Pts',(-2.59603758471431,-24.6797842017353,
12.110422630762));
#57374=CARTESIAN_POINT('Ctrl Pts',(-2.51881566037573,-24.67496750317,12.121184550676));
#57375=CARTESIAN_POINT('Ctrl Pts',(-2.46592222634894,-24.671668288213,12.1285559663179));
#57376=CARTESIAN_POINT('Ctrl Pts',(-2.40973856920156,-24.6682653336581,
12.136167357517));
#57377=CARTESIAN_POINT('Ctrl Pts',(-2.3502524094774,-24.6647978642146,12.143932829769));
#57378=CARTESIAN_POINT('Ctrl Pts',(-2.3184758099704,-24.6629455949083,12.1480810266417));
#57379=CARTESIAN_POINT('Ctrl Pts',(-2.28575682874977,-24.6610749935103,
12.1522730098206));
#57380=CARTESIAN_POINT('Ctrl Pts',(-2.25209361403474,-24.6591925761609,
12.1564944153469));
#57381=CARTESIAN_POINT('Ctrl Pts',(-2.23526200667722,-24.6582513674861,
12.1586051181101));
#57382=CARTESIAN_POINT('Ctrl Pts',(-2.21819434094244,-24.6573072040779,
12.1607231760983));
#57383=CARTESIAN_POINT('Ctrl Pts',(-2.2008903895958,-24.6563609431785,12.1628466938195));
#57384=CARTESIAN_POINT('Ctrl Pts',(-2.19223841392248,-24.6558878127288,
12.1639084526802));
#57385=CARTESIAN_POINT('Ctrl Pts',(-2.18352736684596,-24.6554141578566,
12.1649715764499));
#57386=CARTESIAN_POINT('Ctrl Pts',(-2.17475722021796,-24.6549400867563,
12.1660358252666));
#57387=CARTESIAN_POINT('Ctrl Pts',(-2.16817961024697,-24.6545845334311,
12.1668340118791));
#57388=CARTESIAN_POINT('Ctrl Pts',(-2.16156875677825,-24.6542287459733,
12.1676328313285));
#57389=CARTESIAN_POINT('Ctrl Pts',(-2.15492464800644,-24.6538727705109,
12.1684321812269));
#57390=CARTESIAN_POINT('Ctrl Pts',(-2.1527099450825,-24.6537541120234,12.168698631193));
#57391=CARTESIAN_POINT('Ctrl Pts',(-2.14918581021379,-24.653565683547,12.169121777238));
#57392=CARTESIAN_POINT('Ctrl Pts',(-2.14826945370353,-24.6535167341359,
12.1692317040438));
#57393=CARTESIAN_POINT('Ctrl Pts',(-2.01266622343075,-24.6462731578717,
12.1854987680001));
#57394=CARTESIAN_POINT('Ctrl Pts',(-1.87302045099594,-24.6395508390581,
12.2006547806672));
#57395=CARTESIAN_POINT('Ctrl Pts',(-1.7293456167262,-24.6334657709698,12.2144316569476));
#57396=CARTESIAN_POINT('Ctrl Pts',(-1.55031236472622,-24.6258831658879,
12.2315990264137));
#57397=CARTESIAN_POINT('Ctrl Pts',(-1.36502203923827,-24.6192903798497,
12.2466257338115));
#57398=CARTESIAN_POINT('Ctrl Pts',(-1.17351855249445,-24.6139000937111,
12.2589747504868));
#57399=CARTESIAN_POINT('Ctrl Pts',(-0.994986211747918,-24.6088749089587,
12.2704873286149));
#57400=CARTESIAN_POINT('Ctrl Pts',(-0.811053939099326,-24.6048949710037,
12.2796723335614));
#57401=CARTESIAN_POINT('Ctrl Pts',(-0.621782179049804,-24.6021357649185,
12.2860623894005));
#57402=CARTESIAN_POINT('Ctrl Pts',(-0.437696294019074,-24.5994521585842,
12.2922773634898));
#57403=CARTESIAN_POINT('Ctrl Pts',(-0.24855786948701,-24.5979230965636,
12.2958478190973));
#57404=CARTESIAN_POINT('Ctrl Pts',(-0.0545118224166704,-24.5977239499185,
12.2963372967855));
#57405=CARTESIAN_POINT('Ctrl Pts',(0.0790731766073289,-24.5975868535705,
12.2966742625598));
#57406=CARTESIAN_POINT('Ctrl Pts',(0.214983132282025,-24.5980801350522,
12.2955506236401));
#57407=CARTESIAN_POINT('Ctrl Pts',(0.35315773706709,-24.5992622024089,12.2928178531011));
#57408=CARTESIAN_POINT('Ctrl Pts',(0.484497401462059,-24.6003857976611,
12.2902202616984));
#57409=CARTESIAN_POINT('Ctrl Pts',(0.617882884816372,-24.6021314640099,
12.2861686774687));
#57410=CARTESIAN_POINT('Ctrl Pts',(0.753271902750463,-24.604568076601,12.2805367715706));
#57411=CARTESIAN_POINT('Ctrl Pts',(0.832469025839653,-24.6059933968392,
12.2772423334289));
#57412=CARTESIAN_POINT('Ctrl Pts',(0.912351596562833,-24.6076552162223,
12.2734070861427));
#57413=CARTESIAN_POINT('Ctrl Pts',(0.992910109818521,-24.6095679523229,
12.2690052580806));
#57414=CARTESIAN_POINT('Ctrl Pts',(1.03318936644636,-24.6105243203733,12.2668043440495));
#57415=CARTESIAN_POINT('Ctrl Pts',(1.0736376087202,-24.6115434212917,12.2644617866549));
#57416=CARTESIAN_POINT('Ctrl Pts',(1.1142535593614,-24.6126271063427,12.2619743229869));
#57417=CARTESIAN_POINT('Ctrl Pts',(1.13456153468199,-24.6131689488682,12.260730591153));
#57418=CARTESIAN_POINT('Ctrl Pts',(1.15491143709519,-24.6137269376663,12.2594506328696));
#57419=CARTESIAN_POINT('Ctrl Pts',(1.17530310430095,-24.6143013063295,12.2581340395361));
#57420=CARTESIAN_POINT('Ctrl Pts',(1.18549893790384,-24.6145884906612,12.2574757428694));
#57421=CARTESIAN_POINT('Ctrl Pts',(1.19570521270492,-24.6148797699744,12.2568082874476));
#57422=CARTESIAN_POINT('Ctrl Pts',(1.20592190810774,-24.6151751736556,12.2561316220514));
#57423=CARTESIAN_POINT('Ctrl Pts',(1.20990015198545,-24.6152901998789,12.2558681376404));
#57424=CARTESIAN_POINT('Ctrl Pts',(1.21387997585457,-24.6154058514412,12.2556032568084));
#57425=CARTESIAN_POINT('Ctrl Pts',(1.21786137849036,-24.6155221300862,12.2553369765201));
#57426=CARTESIAN_POINT('Ctrl Pts',(1.2189923796257,-24.6155551614803,12.2552613340051));
#57427=CARTESIAN_POINT('Ctrl Pts',(1.22012350816173,-24.6155882434778,12.2551855785591));
#57428=CARTESIAN_POINT('Ctrl Pts',(1.2212547640704,-24.6156213761122,12.2551097101167));
#57429=CARTESIAN_POINT('Ctrl Pts',(1.22381154177509,-24.6156962599473,12.254938238091));
#57430=CARTESIAN_POINT('Ctrl Pts',(1.2263689701191,-24.6157714024532,12.2547661888437));
#57431=CARTESIAN_POINT('Ctrl Pts',(1.22892704877899,-24.6158468040031,12.254593561651));
#57432=CARTESIAN_POINT('Ctrl Pts',(1.23148512743888,-24.6159222055531,12.2544209344582));
#57433=CARTESIAN_POINT('Ctrl Pts',(1.23542074363146,-24.6160387093936,12.254154237574));
#57434=CARTESIAN_POINT('Ctrl Pts',(1.23660323538095,-24.6160737861916,12.2540739454465));
#57435=CARTESIAN_POINT('Ctrl Pts',(1.30395072286034,-24.6180715457704,12.2495009976367));
#57436=CARTESIAN_POINT('Ctrl Pts',(1.37844758369426,-24.6204559223908,12.2440559080745));
#57437=CARTESIAN_POINT('Ctrl Pts',(1.46006213674872,-24.6233396542443,12.2374902403641));
#57438=CARTESIAN_POINT('Ctrl Pts',(1.54172913328555,-24.6262252391121,12.2309203537189));
#57439=CARTESIAN_POINT('Ctrl Pts',(1.63052319423837,-24.6296108041441,12.2232283669695));
#57440=CARTESIAN_POINT('Ctrl Pts',(1.72639935501991,-24.6336315012617,12.2141200251773));
#57441=CARTESIAN_POINT('Ctrl Pts',(1.81110721698522,-24.6371838405884,12.2060726841807));
#57442=CARTESIAN_POINT('Ctrl Pts',(1.90134326521786,-24.6412322703028,12.1969190487345));
#57443=CARTESIAN_POINT('Ctrl Pts',(1.99706565552425,-24.6458845705382,12.1864276028006));
#57444=CARTESIAN_POINT('Ctrl Pts',(2.1063522091672,-24.6511961163281,12.1744494860281));
#57445=CARTESIAN_POINT('Ctrl Pts',(2.22279079040698,-24.6572943924893,12.160728092125));
#57446=CARTESIAN_POINT('Ctrl Pts',(2.34629928875798,-24.6643605682681,12.1448817120011));
#57447=CARTESIAN_POINT('Ctrl Pts',(2.46252853931017,-24.6710102832757,12.1299692735021));
#57448=CARTESIAN_POINT('Ctrl Pts',(2.58501895958527,-24.6785173574658,12.1131744638724));
#57449=CARTESIAN_POINT('Ctrl Pts',(2.7136812410372,-24.687051272543,12.0941475403894));
#57450=CARTESIAN_POINT('Ctrl Pts',(2.74250184071604,-24.6889628860117,12.0898854727606));
#57451=CARTESIAN_POINT('Ctrl Pts',(2.77163203546633,-24.6909260947847,12.0855112874804));
#57452=CARTESIAN_POINT('Ctrl Pts',(2.80107067398166,-24.6929429031056,12.0810209004385));
#57453=CARTESIAN_POINT('Ctrl Pts',(2.82649119466277,-24.6946844346511,12.0771434121299));
#57454=CARTESIAN_POINT('Ctrl Pts',(2.85493634185601,-24.6966591221582,12.0727493060695));
#57455=CARTESIAN_POINT('Ctrl Pts',(2.88361400236558,-24.6986826338651,12.0682498311971));
#57456=CARTESIAN_POINT('Ctrl Pts',(2.89878517922108,-24.6997531205585,12.0658695000323));
#57457=CARTESIAN_POINT('Ctrl Pts',(2.91402157098735,-24.7008369188883,12.0634604317022));
#57458=CARTESIAN_POINT('Ctrl Pts',(2.9289108422853,-24.7019042081627,12.0610888880559));
#57459=CARTESIAN_POINT('Ctrl Pts',(3.02425374484228,-24.7087385558787,12.0459027953142));
#57460=CARTESIAN_POINT('Ctrl Pts',(3.11262116651476,-24.7154092679509,12.0311145311352));
#57461=CARTESIAN_POINT('Ctrl Pts',(3.19406216944735,-24.7217849183696,12.0170066694321));
#57462=CARTESIAN_POINT('Ctrl Pts',(3.25118406449557,-24.7262567350341,12.0071115580442));
#57463=CARTESIAN_POINT('Ctrl Pts',(3.30489854444122,-24.7305838293824,11.9975501317833));
#57464=CARTESIAN_POINT('Ctrl Pts',(3.35522197545394,-24.7347269021394,11.9884058881509));
#57465=CARTESIAN_POINT('Ctrl Pts',(3.42777339920782,-24.7406999811044,11.9752226078909));
#57466=CARTESIAN_POINT('Ctrl Pts',(3.49327682573633,-24.7462896487671,11.9629084824941));
#57467=CARTESIAN_POINT('Ctrl Pts',(3.55177749153045,-24.7513962548883,11.9516733020361));
#57468=CARTESIAN_POINT('Ctrl Pts',(3.61056547644036,-24.7565279415028,11.9403829413153));
#57469=CARTESIAN_POINT('Ctrl Pts',(3.662281897611,-24.7611718011313,11.9301820645786));
#57470=CARTESIAN_POINT('Ctrl Pts',(3.70696561522605,-24.765248372565,11.9212359999113));
#57471=CARTESIAN_POINT('Ctrl Pts',(3.75187520563725,-24.7693455507575,11.9122447135671));
#57472=CARTESIAN_POINT('Ctrl Pts',(3.78968093527517,-24.7728696794522,11.9045208998948));
#57473=CARTESIAN_POINT('Ctrl Pts',(3.82041308244611,-24.7757620715134,11.898185551049));
#57474=CARTESIAN_POINT('Ctrl Pts',(3.82688038828348,-24.7763707495846,11.896852333479));
#57475=CARTESIAN_POINT('Ctrl Pts',(3.83303440166048,-24.7769515284611,11.8955804417933));
#57476=CARTESIAN_POINT('Ctrl Pts',(3.83887534622704,-24.7775039851309,11.8943707442518));
#57477=CARTESIAN_POINT('Ctrl Pts',(3.851141932702,-24.7786642011604,11.8918302545531));
#57478=CARTESIAN_POINT('Ctrl Pts',(3.86202777749022,-24.7796994500888,11.889564179342));
#57479=CARTESIAN_POINT('Ctrl Pts',(3.87153463878721,-24.780606438657,11.8875792653162));
#57480=CARTESIAN_POINT('Ctrl Pts',(3.8762880694357,-24.7810599329411,11.8865868083033));
#57481=CARTESIAN_POINT('Ctrl Pts',(3.88069675421204,-24.7814813625433,11.8856646417763));
#57482=CARTESIAN_POINT('Ctrl Pts',(3.88476086456357,-24.7818704094171,11.884813414653));
#57483=CARTESIAN_POINT('Ctrl Pts',(3.88679291973933,-24.782064932854,11.8843878010913));
#57484=CARTESIAN_POINT('Ctrl Pts',(3.88873883130893,-24.7822513606371,11.8839799223937));
#57485=CARTESIAN_POINT('Ctrl Pts',(3.89059861927939,-24.7824296556881,11.8835898543782));
#57486=CARTESIAN_POINT('Ctrl Pts',(3.89152851326463,-24.7825188032136,11.8833948203705));
#57487=CARTESIAN_POINT('Ctrl Pts',(3.89243687635008,-24.7826059175579,11.8832042390341));
#57488=CARTESIAN_POINT('Ctrl Pts',(3.89332371087025,-24.7826909944048,11.8830181191914));
#57489=CARTESIAN_POINT('Ctrl Pts',(3.89376712813033,-24.7827335328282,11.88292505927));
#57490=CARTESIAN_POINT('Ctrl Pts',(3.89420516323368,-24.7827755619058,11.8828331146642));
#57491=CARTESIAN_POINT('Ctrl Pts',(3.89463512744225,-24.7828168226514,11.8827428518383));
#57492=CARTESIAN_POINT('Ctrl Pts',(3.89506509165082,-24.782858083397,11.8826525890124));
#57493=CARTESIAN_POINT('Ctrl Pts',(3.89549238168182,-24.7828990583497,11.8825629473677));
#57494=CARTESIAN_POINT('Ctrl Pts',(3.89721720804704,-24.7830646888322,11.8822006266423));
#57495=CARTESIAN_POINT('Ctrl Pts',(3.90600392129834,-24.7839084535057,11.8803548708123));
#57496=CARTESIAN_POINT('Ctrl Pts',(3.91477185417485,-24.7847533414518,11.8785070705958));
#57497=CARTESIAN_POINT('Ctrl Pts',(3.92352101537525,-24.7855993188514,11.8766573015967));
#57498=CARTESIAN_POINT('Ctrl Pts',(4.08352595353532,-24.8010705804277,11.8428286673394));
#57499=CARTESIAN_POINT('Ctrl Pts',(4.23725160174758,-24.8169049778325,11.8083456468854));
#57500=CARTESIAN_POINT('Ctrl Pts',(4.38475855196937,-24.8329052578264,11.77364883758));
#57501=CARTESIAN_POINT('Ctrl Pts',(4.40472994463671,-24.835071582017,11.7689511362046));
#57502=CARTESIAN_POINT('Ctrl Pts',(4.42458735895512,-24.8372409692867,11.7642494432575));
#57503=CARTESIAN_POINT('Ctrl Pts',(4.44433096146912,-24.8394129509478,11.7595447848344));
#57504=CARTESIAN_POINT('Ctrl Pts',(4.59308062634943,-24.8557768107853,11.7240995633596));
#57505=CARTESIAN_POINT('Ctrl Pts',(4.73536929916207,-24.872286764384,11.6884901115367));
#57506=CARTESIAN_POINT('Ctrl Pts',(4.87127286564285,-24.888754267773,11.6531293828841));
#57507=CARTESIAN_POINT('Ctrl Pts',(4.89543477694101,-24.8916819786969,11.6468426987943));
#57508=CARTESIAN_POINT('Ctrl Pts',(4.91939488858616,-24.8946083844813,11.6405637505741));
#57509=CARTESIAN_POINT('Ctrl Pts',(4.94315365408059,-24.8975324732694,11.6342946976842));
#57510=CARTESIAN_POINT('Ctrl Pts',(5.07994862119384,-24.9143683913517,11.5981996032611));
#57511=CARTESIAN_POINT('Ctrl Pts',(5.21006827964491,-24.9311264234348,11.562436664669));
#57512=CARTESIAN_POINT('Ctrl Pts',(5.33360073781613,-24.9476267914863,11.5273895893518));
#57513=CARTESIAN_POINT('Ctrl Pts',(5.36979448451348,-24.9524612305521,11.5171211547615));
#57514=CARTESIAN_POINT('Ctrl Pts',(5.40542280601805,-24.957273639452,11.5069138426419));
#57515=CARTESIAN_POINT('Ctrl Pts',(5.44048800083792,-24.9620597200354,11.4967765000317));
#57516=CARTESIAN_POINT('Ctrl Pts',(5.56340175383617,-24.9788363308507,11.4612421523103));
#57517=CARTESIAN_POINT('Ctrl Pts',(5.67939602405027,-24.9952885190694,11.4265714871969));
#57518=CARTESIAN_POINT('Ctrl Pts',(5.78856809304377,-25.0112461300498,11.3931131709817));
#57519=CARTESIAN_POINT('Ctrl Pts',(5.84238475164958,-25.0191124763617,11.3766198059857));
#57520=CARTESIAN_POINT('Ctrl Pts',(5.89454365912036,-25.0268588293931,11.3604202503116));
#57521=CARTESIAN_POINT('Ctrl Pts',(5.94505661807441,-25.034465991728,11.344551800168));
#57522=CARTESIAN_POINT('Ctrl Pts',(5.95968428646052,-25.036668892732,11.3399565748772));
#57523=CARTESIAN_POINT('Ctrl Pts',(5.97417392859596,-25.0388601269703,11.3353890972023));
#57524=CARTESIAN_POINT('Ctrl Pts',(5.98852581858791,-25.0410392599716,11.3308502293489));
#57525=CARTESIAN_POINT('Ctrl Pts',(-6.39567215687499,-24.2657748885789,
11.8440001031121));
#57526=CARTESIAN_POINT('Ctrl Pts',(-6.35564925762009,-24.2594187411299,
11.8565901649694));
#57527=CARTESIAN_POINT('Ctrl Pts',(-5.98525024769625,-24.2012639131291,
11.9719907509251));
#57528=CARTESIAN_POINT('Ctrl Pts',(-5.2561684893674,-24.0987569285165,12.1789670347241));
#57529=CARTESIAN_POINT('Ctrl Pts',(-4.17576488270491,-23.9769549473289,
12.4300237910532));
#57530=CARTESIAN_POINT('Ctrl Pts',(-3.01937236748527,-23.8792990190897,
12.6350405053752));
#57531=CARTESIAN_POINT('Ctrl Pts',(-1.83578745066896,-23.813668726209,12.7756187739789));
#57532=CARTESIAN_POINT('Ctrl Pts',(-0.697920992868922,-23.7825581791349,
12.8441383465189));
#57533=CARTESIAN_POINT('Ctrl Pts',(0.331415178970398,-23.7794558007235,
12.8512034394307));
#57534=CARTESIAN_POINT('Ctrl Pts',(1.24581749162491,-23.7959569070388,12.8144567277242));
#57535=CARTESIAN_POINT('Ctrl Pts',(2.07031043589906,-23.8272323667122,12.7465802066477));
#57536=CARTESIAN_POINT('Ctrl Pts',(2.81707948231361,-23.8693935680378,12.6564381575931));
#57537=CARTESIAN_POINT('Ctrl Pts',(3.49019584745524,-23.9189819909321,12.5517016211412));
#57538=CARTESIAN_POINT('Ctrl Pts',(4.09498188363305,-23.9729956946651,12.4387764844399));
#57539=CARTESIAN_POINT('Ctrl Pts',(4.65006137436846,-24.0305553196469,12.3195511568429));
#57540=CARTESIAN_POINT('Ctrl Pts',(5.18050883581102,-24.0928860470317,12.1916386147714));
#57541=CARTESIAN_POINT('Ctrl Pts',(5.70542717899815,-24.161879716131,12.0514948116598));
#57542=CARTESIAN_POINT('Ctrl Pts',(6.10978536005174,-24.2209477044549,11.9329722451569));
#57543=CARTESIAN_POINT('Ctrl Pts',(6.34031713732058,-24.2569838550135,11.8614125115549));
#57544=CARTESIAN_POINT('Ctrl Pts',(6.39541677308294,-24.2657356646736,11.8440802215452));
#57545=CARTESIAN_POINT('Ctrl Pts',(-6.33018760820761,-24.6384834345141,
11.8153028757991));
#57546=CARTESIAN_POINT('Ctrl Pts',(-6.29063887131025,-24.632207888034,11.8278584824185));
#57547=CARTESIAN_POINT('Ctrl Pts',(-5.92460081410956,-24.5747868495937,
11.9429531771344));
#57548=CARTESIAN_POINT('Ctrl Pts',(-5.20363827142956,-24.4735116632754,
12.1495424295994));
#57549=CARTESIAN_POINT('Ctrl Pts',(-4.13466637437114,-24.3531178682958,
12.400332283845));
#57550=CARTESIAN_POINT('Ctrl Pts',(-2.99013371612863,-24.2565650775772,
12.6052500696659));
#57551=CARTESIAN_POINT('Ctrl Pts',(-1.81835067631736,-24.1916608618674,
12.7458212153212));
#57552=CARTESIAN_POINT('Ctrl Pts',(-0.691523858728446,-24.1608836285925,
12.8143591049538));
#57553=CARTESIAN_POINT('Ctrl Pts',(0.328416326781379,-24.1578130063956,
12.8214277182404));
#57554=CARTESIAN_POINT('Ctrl Pts',(1.23411374818715,-24.1741398737994,12.7846682205713));
#57555=CARTESIAN_POINT('Ctrl Pts',(2.05053453853478,-24.2050743152816,12.716783758354));
#57556=CARTESIAN_POINT('Ctrl Pts',(2.78984559896008,-24.2467682391815,12.626650714225));
#57557=CARTESIAN_POINT('Ctrl Pts',(3.45612791133979,-24.2957999436839,12.5219504369033));
#57558=CARTESIAN_POINT('Ctrl Pts',(4.05467909050439,-24.3492003014555,12.4090946277549));
#57559=CARTESIAN_POINT('Ctrl Pts',(4.60394317864352,-24.4060984734748,12.2899771959904));
#57560=CARTESIAN_POINT('Ctrl Pts',(5.12872579761141,-24.467702523329,12.1622226552969));
#57561=CARTESIAN_POINT('Ctrl Pts',(5.64789551167839,-24.5358760477359,12.0223078678906));
#57562=CARTESIAN_POINT('Ctrl Pts',(6.04766431615617,-24.594221541182,11.9040400248831));
#57563=CARTESIAN_POINT('Ctrl Pts',(6.27548853220886,-24.6298039142637,11.8326675985416));
#57564=CARTESIAN_POINT('Ctrl Pts',(6.32993492750253,-24.6384446244456,11.815382831619));
#57565=CARTESIAN_POINT('Ctrl Pts',(-6.21932807476777,-24.9339439082172,
11.604605690097));
#57566=CARTESIAN_POINT('Ctrl Pts',(-6.18048319098318,-24.927839570483,11.6170311210407));
#57567=CARTESIAN_POINT('Ctrl Pts',(-5.82094596454687,-24.8719851686731,
11.7309382763999));
#57568=CARTESIAN_POINT('Ctrl Pts',(-5.11256521760226,-24.7734765152896,
11.935486217029));
#57569=CARTESIAN_POINT('Ctrl Pts',(-4.06220012775385,-24.656438577069,12.183872436982));
#57570=CARTESIAN_POINT('Ctrl Pts',(-2.93773661033481,-24.5626423516593,
12.3868519818438));
#57571=CARTESIAN_POINT('Ctrl Pts',(-1.78661031468882,-24.4996269921563,
12.5261022238268));
#57572=CARTESIAN_POINT('Ctrl Pts',(-0.679624998569868,-24.469749998326,
12.5940022893219));
#57573=CARTESIAN_POINT('Ctrl Pts',(0.322797658949184,-24.4667682564501,
12.6010062443498));
#57574=CARTESIAN_POINT('Ctrl Pts',(1.21266000790277,-24.4826189620022,12.5645869597438));
#57575=CARTESIAN_POINT('Ctrl Pts',(2.01470259299457,-24.5126494340044,12.4973377775454));
#57576=CARTESIAN_POINT('Ctrl Pts',(2.74098505384707,-24.5531332040697,12.4080520697349));
#57577=CARTESIAN_POINT('Ctrl Pts',(3.39555710185985,-24.6007563884208,12.3043401270959));
#57578=CARTESIAN_POINT('Ctrl Pts',(3.98362867469768,-24.6526406766682,12.1925548621677));
#57579=CARTESIAN_POINT('Ctrl Pts',(4.52330902376504,-24.7079423472852,12.0745750879856));
#57580=CARTESIAN_POINT('Ctrl Pts',(5.0389522756289,-24.7678368988428,11.9480529624072));
#57581=CARTESIAN_POINT('Ctrl Pts',(5.54907007392285,-24.8341368734838,11.8095087077752));
#57582=CARTESIAN_POINT('Ctrl Pts',(5.94182116608985,-24.8908896280395,11.6924277333148));
#57583=CARTESIAN_POINT('Ctrl Pts',(6.16560261557379,-24.9255012171011,11.6217903445456));
#57584=CARTESIAN_POINT('Ctrl Pts',(6.21907959854346,-24.9339060769377,11.6046848718899));
#57585=CARTESIAN_POINT('Ctrl Pts',(-6.09477939299971,-25.0678698905147,
11.2722082266352));
#57586=CARTESIAN_POINT('Ctrl Pts',(-6.05666692574621,-25.0619784177097,
11.2844450029348));
#57587=CARTESIAN_POINT('Ctrl Pts',(-5.70391276856255,-25.0080755673627,
11.3966227162906));
#57588=CARTESIAN_POINT('Ctrl Pts',(-5.00898083431377,-24.9130771230655,
11.5980591809797));
#57589=CARTESIAN_POINT('Ctrl Pts',(-3.97907981782851,-24.8003830729569,
11.8425929828331));
#57590=CARTESIAN_POINT('Ctrl Pts',(-2.87715857378435,-24.7102085307339,
12.0423498167333));
#57591=CARTESIAN_POINT('Ctrl Pts',(-1.74963945844598,-24.6497046156879,
12.1793435465576));
#57592=CARTESIAN_POINT('Ctrl Pts',(-0.665625857014882,-24.6210373185601,
12.2461322723438));
#57593=CARTESIAN_POINT('Ctrl Pts',(0.316165362967699,-24.6181761604121,
12.2530219051821));
#57594=CARTESIAN_POINT('Ctrl Pts',(1.18758896401542,-24.6333849650858,12.2171984183309));
#57595=CARTESIAN_POINT('Ctrl Pts',(1.97305721071989,-24.6622070463197,12.1510458485583));
#57596=CARTESIAN_POINT('Ctrl Pts',(2.68446448312266,-24.701083874296,12.0632032212655));
#57597=CARTESIAN_POINT('Ctrl Pts',(3.32579714717992,-24.7468495445224,11.9611487557751));
#57598=CARTESIAN_POINT('Ctrl Pts',(3.90213960567858,-24.796748592875,11.8511288088831));
#57599=CARTESIAN_POINT('Ctrl Pts',(4.43120697430717,-24.849975255363,11.7349908279827));
#57600=CARTESIAN_POINT('Ctrl Pts',(4.93684832779728,-24.9076663275402,11.6104228168409));
#57601=CARTESIAN_POINT('Ctrl Pts',(5.43719781099491,-24.9715750789933,11.473998412235));
#57602=CARTESIAN_POINT('Ctrl Pts',(5.82250829244893,-25.0263202652274,11.3586968561321));
#57603=CARTESIAN_POINT('Ctrl Pts',(6.04206701108784,-25.0597216307159,11.2891319452229));
#57604=CARTESIAN_POINT('Ctrl Pts',(6.09453542110593,-25.0678333230897,11.2722862444664));
#57605=CARTESIAN_POINT('',(6.27159454870745,-24.2690137147412,11.8794923467063));
#57606=CARTESIAN_POINT('Origin',(5.999999949026,-24.1259420052077,10.9277802669262));
#57607=CARTESIAN_POINT('Ctrl Pts',(-6.27159387328071,-24.2690123753742,
11.8794984953283));
#57608=CARTESIAN_POINT('Ctrl Pts',(-6.13239662717945,-24.2474082695837,
11.9224692255698));
#57609=CARTESIAN_POINT('Ctrl Pts',(-5.98564488051794,-24.22550253681,11.9663158871379));
#57610=CARTESIAN_POINT('Ctrl Pts',(-5.83132857677373,-24.2035349707518,
12.010553920225));
#57611=CARTESIAN_POINT('Ctrl Pts',(-5.67907400589207,-24.1818609009202,
12.0542009139703));
#57612=CARTESIAN_POINT('Ctrl Pts',(-5.51945536419364,-24.1601268679718,
12.0982289236256));
#57613=CARTESIAN_POINT('Ctrl Pts',(-5.35247229680066,-24.1385689747149,
12.1421228901419));
#57614=CARTESIAN_POINT('Ctrl Pts',(-5.32566767336653,-24.1351084369502,
12.1491688814623));
#57615=CARTESIAN_POINT('Ctrl Pts',(-5.29867331120474,-24.1316524459909,
12.1562113129512));
#57616=CARTESIAN_POINT('Ctrl Pts',(-5.27148923945306,-24.1282019864977,
12.1632479318689));
#57617=CARTESIAN_POINT('Ctrl Pts',(-5.14595591333737,-24.1122681094553,
12.1957423346728));
#57618=CARTESIAN_POINT('Ctrl Pts',(-5.01637663573241,-24.0964518554399,
12.2281140196681));
#57619=CARTESIAN_POINT('Ctrl Pts',(-4.88275737830249,-24.0808623948862,
12.2601325393302));
#57620=CARTESIAN_POINT('Ctrl Pts',(-4.71106404886683,-24.0608308033472,
12.3012745599501));
#57621=CARTESIAN_POINT('Ctrl Pts',(-4.53269546252188,-24.041172933994,12.3418362502158));
#57622=CARTESIAN_POINT('Ctrl Pts',(-4.34764543253218,-24.0221340484763,
12.3812950907415));
#57623=CARTESIAN_POINT('Ctrl Pts',(-4.29584179753053,-24.0168042277989,
12.3923413541347));
#57624=CARTESIAN_POINT('Ctrl Pts',(-4.24351464833661,-24.0115229877401,
12.4033009024142));
#57625=CARTESIAN_POINT('Ctrl Pts',(-4.19066409785601,-24.0062958742251,
12.4141615963694));
#57626=CARTESIAN_POINT('Ctrl Pts',(-4.14338773419268,-24.0016200682552,
12.4238768048658));
#57627=CARTESIAN_POINT('Ctrl Pts',(-4.09569255318101,-23.9969875734089,
12.4335129069651));
#57628=CARTESIAN_POINT('Ctrl Pts',(-4.04757898340068,-23.9924025346269,
12.4430611439712));
#57629=CARTESIAN_POINT('Ctrl Pts',(-3.90056246597125,-23.9783924240263,
12.472236874615));
#57630=CARTESIAN_POINT('Ctrl Pts',(-3.74963596560522,-23.9648249549461,
12.5005941124992));
#57631=CARTESIAN_POINT('Ctrl Pts',(-3.59479965791586,-23.9518214662445,
12.527874772864));
#57632=CARTESIAN_POINT('Ctrl Pts',(-3.51738150407117,-23.9453197218937,
12.5415151030463));
#57633=CARTESIAN_POINT('Ctrl Pts',(-3.43898588978398,-23.9389590682647,
12.5548860386607));
#57634=CARTESIAN_POINT('Ctrl Pts',(-3.35961278769273,-23.9327552481046,
12.5679537443453));
#57635=CARTESIAN_POINT('Ctrl Pts',(-3.3199262366471,-23.9296533380245,12.5744875971876));
#57636=CARTESIAN_POINT('Ctrl Pts',(-3.27999531125928,-23.9265906345002,
12.5809456267339));
#57637=CARTESIAN_POINT('Ctrl Pts',(-3.23982000755822,-23.923569150133,12.5873234975459));
#57638=CARTESIAN_POINT('Ctrl Pts',(-3.21973235570769,-23.9220584079494,
12.5905124329519));
#57639=CARTESIAN_POINT('Ctrl Pts',(-3.19958360912905,-23.9205579704376,
12.5936813276397));
#57640=CARTESIAN_POINT('Ctrl Pts',(-3.17937376683442,-23.9190680900284,
12.5968296331371));
#57641=CARTESIAN_POINT('Ctrl Pts',(-3.16169015482662,-23.9177644446704,
12.5995844004473));
#57642=CARTESIAN_POINT('Ctrl Pts',(-3.14395976640254,-23.9164688820872,
12.6023234040973));
#57643=CARTESIAN_POINT('Ctrl Pts',(-3.12618260080716,-23.9151815721529,
12.605046273797));
#57644=CARTESIAN_POINT('Ctrl Pts',(-3.1236430057221,-23.9149976707337,12.6054352551827));
#57645=CARTESIAN_POINT('Ctrl Pts',(-3.11986203063022,-23.9147243461149,
12.6060134344833));
#57646=CARTESIAN_POINT('Ctrl Pts',(-3.11856095164605,-23.9146303736825,
12.6062122290604));
#57647=CARTESIAN_POINT('Ctrl Pts',(-3.09161417126445,-23.9126841009898,
12.6103294839506));
#57648=CARTESIAN_POINT('Ctrl Pts',(-3.0634423340961,-23.9106768776393,12.6145803991693));
#57649=CARTESIAN_POINT('Ctrl Pts',(-3.0340454669724,-23.9086159226008,12.6189497247918));
#57650=CARTESIAN_POINT('Ctrl Pts',(-2.96197963940193,-23.9035635328408,
12.6296610385376));
#57651=CARTESIAN_POINT('Ctrl Pts',(-2.88255172211161,-23.8981867199339,
12.6410872436616));
#57652=CARTESIAN_POINT('Ctrl Pts',(-2.79576134945282,-23.8926070410898,
12.6529712009058));
#57653=CARTESIAN_POINT('Ctrl Pts',(-2.70930123057302,-23.8870485939787,
12.6648099374455));
#57654=CARTESIAN_POINT('Ctrl Pts',(-2.61553433409856,-23.8812888577212,
12.6771029777179));
#57655=CARTESIAN_POINT('Ctrl Pts',(-2.51446139230001,-23.875469340143,12.6895489825356));
#57656=CARTESIAN_POINT('Ctrl Pts',(-2.50259873636493,-23.8747863192127,
12.6910097362278));
#57657=CARTESIAN_POINT('Ctrl Pts',(-2.49063544288681,-23.8741024986736,
12.6924725431445));
#57658=CARTESIAN_POINT('Ctrl Pts',(-2.47857151659949,-23.8734181263219,
12.6939368729798));
#57659=CARTESIAN_POINT('Ctrl Pts',(-2.37688570196303,-23.8676496096352,
12.7062795853488));
#57660=CARTESIAN_POINT('Ctrl Pts',(-2.26804989959386,-23.8618405802166,
12.7187343033419));
#57661=CARTESIAN_POINT('Ctrl Pts',(-2.15206290281673,-23.8561525055082,
12.7309579405412));
#57662=CARTESIAN_POINT('Ctrl Pts',(-2.11969744814923,-23.8545652834123,
12.7343688709613));
#57663=CARTESIAN_POINT('Ctrl Pts',(-2.08677520819492,-23.8529876000154,
12.7377615251891));
#57664=CARTESIAN_POINT('Ctrl Pts',(-2.05329627690419,-23.8514232428241,
12.7411277870223));
#57665=CARTESIAN_POINT('Ctrl Pts',(-1.97656814841425,-23.8478379969708,
12.7488426978787));
#57666=CARTESIAN_POINT('Ctrl Pts',(-1.89691554236842,-23.8443225623912,
12.7564195700191));
#57667=CARTESIAN_POINT('Ctrl Pts',(-1.81433841354751,-23.840925217303,12.7637550184601));
#57668=CARTESIAN_POINT('Ctrl Pts',(-1.81240189321798,-23.8408455459954,
12.7639270424241));
#57669=CARTESIAN_POINT('Ctrl Pts',(-1.81046376456493,-23.8407659396075,
12.7640989332609));
#57670=CARTESIAN_POINT('Ctrl Pts',(-1.80852402756924,-23.8406863988239,
12.7642706895808));
#57671=CARTESIAN_POINT('Ctrl Pts',(-1.76910661759122,-23.8390700499663,
12.7677609510392));
#57672=CARTESIAN_POINT('Ctrl Pts',(-1.72902504057366,-23.8374807808731,
12.7711956978237));
#57673=CARTESIAN_POINT('Ctrl Pts',(-1.68827931980546,-23.8359241930247,
12.7745632605405));
#57674=CARTESIAN_POINT('Ctrl Pts',(-1.6669039077312,-23.8351075991331,12.7763299010466));
#57675=CARTESIAN_POINT('Ctrl Pts',(-1.64534571527873,-23.8342999985571,
12.7780780457792));
#57676=CARTESIAN_POINT('Ctrl Pts',(-1.6236047433072,-23.8335022087906,12.7798059678567));
#57677=CARTESIAN_POINT('Ctrl Pts',(-1.61273425732144,-23.8331033139073,
12.7806699288955));
#57678=CARTESIAN_POINT('Ctrl Pts',(-1.60181807642095,-23.8327068716801,
12.7815288338303));
#57679=CARTESIAN_POINT('Ctrl Pts',(-1.59085620070828,-23.8323129856556,
12.7823824639616));
#57680=CARTESIAN_POINT('Ctrl Pts',(-1.58537526285195,-23.8321160426433,
12.7828092790273));
#57681=CARTESIAN_POINT('Ctrl Pts',(-1.5798829012904,-23.8319197386788,12.7832347753643));
#57682=CARTESIAN_POINT('Ctrl Pts',(-1.57437911603661,-23.8317240867953,
12.7836589254565));
#57683=CARTESIAN_POINT('Ctrl Pts',(-1.56887533078281,-23.8315284349118,
12.7840830755486));
#57684=CARTESIAN_POINT('Ctrl Pts',(-1.56205960344969,-23.8312877045765,
12.7846050496261));
#57685=CARTESIAN_POINT('Ctrl Pts',(-1.55783348920669,-23.8311391004417,
12.7849273093667));
#57686=CARTESIAN_POINT('Ctrl Pts',(-1.33210031965717,-23.8232015766445,
12.8021404532776));
#57687=CARTESIAN_POINT('Ctrl Pts',(-1.11005377605612,-23.8171220368827,
12.8153351581337));
#57688=CARTESIAN_POINT('Ctrl Pts',(-0.891696916844576,-23.8127291071686,
12.8248709177998));
#57689=CARTESIAN_POINT('Ctrl Pts',(-0.848420688569367,-23.8118584707719,
12.8267608136042));
#57690=CARTESIAN_POINT('Ctrl Pts',(-0.805289283440663,-23.8110541627737,
12.8285068905267));
#57691=CARTESIAN_POINT('Ctrl Pts',(-0.762302573188932,-23.8103149647013,
12.8301118032893));
#57692=CARTESIAN_POINT('Ctrl Pts',(-0.724715167136212,-23.8096686128884,
12.8315151325353));
#57693=CARTESIAN_POINT('Ctrl Pts',(-0.687238375249081,-23.8090720098778,
12.8328105347313));
#57694=CARTESIAN_POINT('Ctrl Pts',(-0.649872395356749,-23.8085242237602,
12.8339997614218));
#57695=CARTESIAN_POINT('Ctrl Pts',(-0.558062474711744,-23.8071782882292,
12.8369217457616));
#57696=CARTESIAN_POINT('Ctrl Pts',(-0.466921580641413,-23.8061270274871,
12.8392028078876));
#57697=CARTESIAN_POINT('Ctrl Pts',(-0.376448947681508,-23.8053581703231,
12.8408704270691));
#57698=CARTESIAN_POINT('Ctrl Pts',(-0.312801774508532,-23.8048172820626,
12.8420435911891));
#57699=CARTESIAN_POINT('Ctrl Pts',(-0.249485488676972,-23.8044160906664,
12.8429131418859));
#57700=CARTESIAN_POINT('Ctrl Pts',(-0.186500090506563,-23.8041502798702,
12.8434883989328));
#57701=CARTESIAN_POINT('Ctrl Pts',(-0.155007391421359,-23.8040173744721,
12.8437760274562));
#57702=CARTESIAN_POINT('Ctrl Pts',(-0.123597414128386,-23.8039183139151,
12.8439900795266));
#57703=CARTESIAN_POINT('Ctrl Pts',(-0.0922701582487795,-23.8038525597042,
12.844131701988));
#57704=CARTESIAN_POINT('Ctrl Pts',(-0.0647192913967876,-23.8037947319289,
12.8442562523664));
#57705=CARTESIAN_POINT('Ctrl Pts',(-0.038338200399373,-23.8037631769384,
12.8443236937221));
#57706=CARTESIAN_POINT('Ctrl Pts',(-0.0102093966637263,-23.8037560884165,
12.8443378682552));
#57707=CARTESIAN_POINT('Ctrl Pts',(-0.0063537900014073,-23.8037551167949,
12.8443398111542));
#57708=CARTESIAN_POINT('Ctrl Pts',(-0.00246534702685521,-23.8037546375739,
12.8443406806357));
#57709=CARTESIAN_POINT('Ctrl Pts',(0.00146344560311196,-23.8037546780383,
12.8443404156627));
#57710=CARTESIAN_POINT('Ctrl Pts',(0.123999816234775,-23.8037559400956,
12.8443321513353));
#57711=CARTESIAN_POINT('Ctrl Pts',(0.246532789977683,-23.8042792177409,
12.843219982003));
#57712=CARTESIAN_POINT('Ctrl Pts',(0.369067470033404,-23.8053128677452,
12.841003900385));
#57713=CARTESIAN_POINT('Ctrl Pts',(0.644882197439504,-23.8076395224852,
12.8360156966607));
#57714=CARTESIAN_POINT('Ctrl Pts',(0.920705383073052,-23.8125504903585,
12.8254375262026));
#57715=CARTESIAN_POINT('Ctrl Pts',(1.19652643908533,-23.8200738774936,12.8092721265147));
#57716=CARTESIAN_POINT('Ctrl Pts',(1.22212487701974,-23.8207721090261,12.8077718459104));
#57717=CARTESIAN_POINT('Ctrl Pts',(1.24772329839335,-23.8214928587271,12.8062234073577));
#57718=CARTESIAN_POINT('Ctrl Pts',(1.27332169550815,-23.82223615935,12.8046267927066));
#57719=CARTESIAN_POINT('Ctrl Pts',(1.37083378686327,-23.825067617817,12.7985448012044));
#57720=CARTESIAN_POINT('Ctrl Pts',(1.46834552751173,-23.8282262803923,12.7917637905529));
#57721=CARTESIAN_POINT('Ctrl Pts',(1.56585687062987,-23.8317101409852,12.7842847834704));
#57722=CARTESIAN_POINT('Ctrl Pts',(1.74018381696187,-23.8379384500126,12.7709141085869));
#57723=CARTESIAN_POINT('Ctrl Pts',(1.91451114826108,-23.8452074329911,12.7553127104155));
#57724=CARTESIAN_POINT('Ctrl Pts',(2.08883802674333,-23.8535168166396,12.7374798377617));
#57725=CARTESIAN_POINT('Ctrl Pts',(2.17524324653907,-23.8576353675296,12.728640963948));
#57726=CARTESIAN_POINT('Ctrl Pts',(2.26164833787826,-23.8620095716639,12.7192537731417));
#57727=CARTESIAN_POINT('Ctrl Pts',(2.34805359177696,-23.8666392626977,12.7093187483884));
#57728=CARTESIAN_POINT('Ctrl Pts',(2.47841969236965,-23.8736244255182,12.6943290298475));
#57729=CARTESIAN_POINT('Ctrl Pts',(2.60878583208634,-23.8811913884664,12.6780923256736));
#57730=CARTESIAN_POINT('Ctrl Pts',(2.73915198362006,-23.8893399953416,12.660608688594));
#57731=CARTESIAN_POINT('Ctrl Pts',(2.7725502745386,-23.8914275735955,12.6561295842358));
#57732=CARTESIAN_POINT('Ctrl Pts',(2.80594857215928,-23.8935533167625,12.6515686306175));
#57733=CARTESIAN_POINT('Ctrl Pts',(2.83934685804531,-23.8957172371731,12.6469258080376));
#57734=CARTESIAN_POINT('Ctrl Pts',(2.87113163810424,-23.8977766163445,12.6425072850314));
#57735=CARTESIAN_POINT('Ctrl Pts',(2.90291640750853,-23.8998705731464,12.6380146122504));
#57736=CARTESIAN_POINT('Ctrl Pts',(2.93470118226597,-23.9019990913401,12.6334478151434));
#57737=CARTESIAN_POINT('Ctrl Pts',(2.98358847357062,-23.9052729068628,12.6264237496215));
#57738=CARTESIAN_POINT('Ctrl Pts',(3.03247576140564,-23.9086285029917,12.6192243322693));
#57739=CARTESIAN_POINT('Ctrl Pts',(3.08136305166664,-23.9120658769088,12.6118496265356));
#57740=CARTESIAN_POINT('Ctrl Pts',(3.09765881508698,-23.9132116682146,12.609391391291));
#57741=CARTESIAN_POINT('Ctrl Pts',(3.11203760514041,-23.9142296214825,12.6072074391805));
#57742=CARTESIAN_POINT('Ctrl Pts',(3.13025034275502,-23.9155305097556,12.6044164919562));
#57743=CARTESIAN_POINT('Ctrl Pts',(3.25877662891664,-23.9247108066441,12.5847209311238));
#57744=CARTESIAN_POINT('Ctrl Pts',(3.38588318064259,-23.9344233066419,12.5640238714892));
#57745=CARTESIAN_POINT('Ctrl Pts',(3.51155623328943,-23.9446289514687,12.5424066115913));
#57746=CARTESIAN_POINT('Ctrl Pts',(3.71381534700374,-23.9610539895661,12.5076156382218));
#57747=CARTESIAN_POINT('Ctrl Pts',(3.9123606482021,-23.9787560995128,12.4704422691085));
#57748=CARTESIAN_POINT('Ctrl Pts',(4.10715837540687,-23.9975763260287,12.4312175040207));
#57749=CARTESIAN_POINT('Ctrl Pts',(4.29250871339822,-24.0154838005966,12.3938950795192));
#57750=CARTESIAN_POINT('Ctrl Pts',(4.4744664469351,-24.0344036515817,12.3547152777956));
#57751=CARTESIAN_POINT('Ctrl Pts',(4.65302175618388,-24.0542061396187,12.313950313393));
#57752=CARTESIAN_POINT('Ctrl Pts',(4.83066123702135,-24.0739070586727,12.2733944366549));
#57753=CARTESIAN_POINT('Ctrl Pts',(5.0049332557109,-24.0944816891167,12.2312695841911));
#57754=CARTESIAN_POINT('Ctrl Pts',(5.17584377090454,-24.1158122573969,12.1878294987181));
#57755=CARTESIAN_POINT('Ctrl Pts',(5.35321544777451,-24.1379492140385,12.1427471888614));
#57756=CARTESIAN_POINT('Ctrl Pts',(5.52696673869725,-24.1609005245582,12.0962483800698));
#57757=CARTESIAN_POINT('Ctrl Pts',(5.69711918676627,-24.1845490788121,12.0485987285614));
#57758=CARTESIAN_POINT('Ctrl Pts',(5.87745056229334,-24.2096123462892,11.998098560639));
#57759=CARTESIAN_POINT('Ctrl Pts',(6.05373965431679,-24.235459144335,11.9463058423981));
#57760=CARTESIAN_POINT('Ctrl Pts',(6.22602530087827,-24.2619717767003,11.8935134849131));
#57761=CARTESIAN_POINT('Ctrl Pts',(6.24124677966984,-24.2643141742204,11.8888492672847));
#57762=CARTESIAN_POINT('Ctrl Pts',(6.25643701466579,-24.2666617667428,11.8841772329832));
#57763=CARTESIAN_POINT('Ctrl Pts',(6.27159604017702,-24.2690144967309,11.8794975712369));
#57764=CARTESIAN_POINT('Origin',(5.999999999061,-24.1259421376201,10.9277802195584));
#57765=CARTESIAN_POINT('Origin',(5.99996968604825,-24.1259230378211,10.9277552844787));
#57766=CARTESIAN_POINT('Ctrl Pts',(6.24176941899738,-13.957654817887,8.44269195219273));
#57767=CARTESIAN_POINT('Ctrl Pts',(6.29480662257667,-13.9539758868461,8.42029737038065));
#57768=CARTESIAN_POINT('Ctrl Pts',(6.43873776769985,-13.9497948794457,8.34843305972531));
#57769=CARTESIAN_POINT('Ctrl Pts',(6.65746053635757,-13.9704924485183,8.18719582107129));
#57770=CARTESIAN_POINT('Ctrl Pts',(6.86734070108195,-14.0338129508464,7.94766158322873));
#57771=CARTESIAN_POINT('Ctrl Pts',(7.01531431986487,-14.12893286126,7.67885700588408));
#57772=CARTESIAN_POINT('Ctrl Pts',(7.09527319749003,-14.2420002632323,7.41047463185613));
#57773=CARTESIAN_POINT('Ctrl Pts',(7.10994675708914,-14.3254890997433,7.23571490121343));
#57774=CARTESIAN_POINT('Ctrl Pts',(7.10820126656667,-14.3668778615597,7.15390513393751));
#57775=CARTESIAN_POINT('Ctrl Pts',(7.10813647714078,-14.3682028206859,7.15129096938794));
#57776=CARTESIAN_POINT('Ctrl Pts',(6.04288613265708,-13.4963640462423,8.03309250552645));
#57777=CARTESIAN_POINT('Ctrl Pts',(6.08960516161976,-13.4928601309614,8.01356864824412));
#57778=CARTESIAN_POINT('Ctrl Pts',(6.2166906694153,-13.4882574395743,7.95084472145826));
#57779=CARTESIAN_POINT('Ctrl Pts',(6.41097422058303,-13.5044523004311,7.80952772694627));
#57780=CARTESIAN_POINT('Ctrl Pts',(6.59849710701976,-13.5579129738396,7.59861108001617));
#57781=CARTESIAN_POINT('Ctrl Pts',(6.73122626769599,-13.6400563468318,7.36127071899955));
#57782=CARTESIAN_POINT('Ctrl Pts',(6.80304010187831,-13.7388311824901,7.12425047056187));
#57783=CARTESIAN_POINT('Ctrl Pts',(6.81617738657188,-13.8121459300844,6.9703554643886));
#57784=CARTESIAN_POINT('Ctrl Pts',(6.81461542349125,-13.8484941084794,6.89855976198674));
#57785=CARTESIAN_POINT('Ctrl Pts',(6.81455744755899,-13.8496577047512,6.89626585280356));
#57786=CARTESIAN_POINT('Ctrl Pts',(6.02645468922222,-12.8504950003107,8.09088772242199));
#57787=CARTESIAN_POINT('Ctrl Pts',(6.09090484391799,-12.8459131881969,8.06435034383859));
#57788=CARTESIAN_POINT('Ctrl Pts',(6.26494844742361,-12.8404855791265,7.97971703923798));
#57789=CARTESIAN_POINT('Ctrl Pts',(6.52611211563489,-12.8641139638988,7.79272678876749));
#57790=CARTESIAN_POINT('Ctrl Pts',(6.77358744402654,-12.9364281019538,7.51909413889916));
#57791=CARTESIAN_POINT('Ctrl Pts',(6.9465841611291,-13.0441857127227,7.21504636510149));
#57792=CARTESIAN_POINT('Ctrl Pts',(7.03980001104882,-13.1717068625044,6.91269989963593));
#57793=CARTESIAN_POINT('Ctrl Pts',(7.05702528395121,-13.266031894225,6.71530137399919));
#57794=CARTESIAN_POINT('Ctrl Pts',(7.05497402265406,-13.3130233822045,6.62240791160254));
#57795=CARTESIAN_POINT('Ctrl Pts',(7.05489787988465,-13.3145279375336,6.61943905343894));
#57796=CARTESIAN_POINT('Ctrl Pts',(6.20434282365839,-12.4603649383441,8.57827987685632));
#57797=CARTESIAN_POINT('Ctrl Pts',(6.2985528389579,-12.4541838053812,8.53959812679702));
#57798=CARTESIAN_POINT('Ctrl Pts',(6.55152409727625,-12.4480898317399,8.41685409211037));
#57799=CARTESIAN_POINT('Ctrl Pts',(6.9255489507725,-12.4860551148184,8.14954765545105));
#57800=CARTESIAN_POINT('Ctrl Pts',(7.2746460694698,-12.5931657472206,7.76436053208526));
#57801=CARTESIAN_POINT('Ctrl Pts',(7.51612672467238,-12.747777253834,7.34062969290588));
#57802=CARTESIAN_POINT('Ctrl Pts',(7.64578430161563,-12.9276098455488,6.92052689466441));
#57803=CARTESIAN_POINT('Ctrl Pts',(7.6699507152677,-13.0598954694388,6.64473012363261));
#57804=CARTESIAN_POINT('Ctrl Pts',(7.66706901025419,-13.1260031184009,6.51392112449348));
#57805=CARTESIAN_POINT('Ctrl Pts',(7.66696203505706,-13.1281199481508,6.50973940142776));
#57806=CARTESIAN_POINT('',(6.9999997358385,-13.9487123452115,6.97710990117158));
#57807=CARTESIAN_POINT('',(7.00000022915234,-12.52206486378,8.04447615962587));
#57808=CARTESIAN_POINT('Ctrl Pts',(7.,-13.9487123452086,6.97710990118712));
#57809=CARTESIAN_POINT('Ctrl Pts',(7.,-13.8452746480186,7.02168653880504));
#57810=CARTESIAN_POINT('Ctrl Pts',(7.,-13.7540053535313,7.06360287625015));
#57811=CARTESIAN_POINT('Ctrl Pts',(7.,-13.6763761579061,7.10177115731546));
#57812=CARTESIAN_POINT('Ctrl Pts',(7.,-13.6375615600935,7.12085529784811));
#57813=CARTESIAN_POINT('Ctrl Pts',(7.,-13.6021311738989,7.13895532994855));
#57814=CARTESIAN_POINT('Ctrl Pts',(7.,-13.5701291793535,7.15576042707438));
#57815=CARTESIAN_POINT('Ctrl Pts',(7.,-13.5541281820809,7.16416297563729));
#57816=CARTESIAN_POINT('Ctrl Pts',(7.,-13.5389831154623,7.17224067284011));
#57817=CARTESIAN_POINT('Ctrl Pts',(7.,-13.5246936731342,7.17995082951218));
#57818=CARTESIAN_POINT('Ctrl Pts',(7.,-13.5175489519701,7.18380590784822));
#57819=CARTESIAN_POINT('Ctrl Pts',(7.,-13.5106181368786,7.18756910105157));
#57820=CARTESIAN_POINT('Ctrl Pts',(7.,-13.5039008551055,7.19123504735637));
#57821=CARTESIAN_POINT('Ctrl Pts',(7.,-13.500542214219,7.19306802050878));
#57822=CARTESIAN_POINT('Ctrl Pts',(7.,-13.497236956662,7.19487668193654));
#57823=CARTESIAN_POINT('Ctrl Pts',(7.,-13.4939850306347,7.19666037209525));
#57824=CARTESIAN_POINT('Ctrl Pts',(7.,-13.4907331046074,7.19844406225396));
#57825=CARTESIAN_POINT('Ctrl Pts',(7.,-13.4891059090995,7.19933693116375));
#57826=CARTESIAN_POINT('Ctrl Pts',(7.,-13.4843891909902,7.20193587147612));
#57827=CARTESIAN_POINT('Ctrl Pts',(7.,-13.4089217012407,7.24351891647397));
#57828=CARTESIAN_POINT('Ctrl Pts',(7.,-13.3377088629193,7.28578459273304));
#57829=CARTESIAN_POINT('Ctrl Pts',(7.,-13.2712546130133,7.32835053042459));
#57830=CARTESIAN_POINT('Ctrl Pts',(7.,-13.2048003631073,7.37091646811614));
#57831=CARTESIAN_POINT('Ctrl Pts',(7.,-13.1443230524494,7.41286004032249));
#57832=CARTESIAN_POINT('Ctrl Pts',(7.,-13.0863568342088,7.45600927554525));
#57833=CARTESIAN_POINT('Ctrl Pts',(7.,-12.9704243977276,7.54230774599077));
#57834=CARTESIAN_POINT('Ctrl Pts',(7.,-12.8624865195397,7.63585224400371));
#57835=CARTESIAN_POINT('Ctrl Pts',(7.,-12.7672168886966,7.73520351279626));
#57836=CARTESIAN_POINT('Ctrl Pts',(7.,-12.6719472578536,7.83455478158881));
#57837=CARTESIAN_POINT('Ctrl Pts',(7.,-12.5894810216966,7.93953249757783));
#57838=CARTESIAN_POINT('Ctrl Pts',(7.,-12.5220651723765,8.04447541337249));
#57839=CARTESIAN_POINT('',(6.24994411212243,-12.4626497324863,8.55169576993692));
#57840=CARTESIAN_POINT('Ctrl Pts',(6.24994458392592,-12.4626510779178,8.55169669313912));
#57841=CARTESIAN_POINT('Ctrl Pts',(6.29980713482775,-12.4600704144922,8.52997497958608));
#57842=CARTESIAN_POINT('Ctrl Pts',(6.34865158794145,-12.4586352046275,8.50672736958435));
#57843=CARTESIAN_POINT('Ctrl Pts',(6.39650052995822,-12.4582919652257,8.48202083011274));
#57844=CARTESIAN_POINT('Ctrl Pts',(6.42315482381289,-12.458100763425,8.46825803128267));
#57845=CARTESIAN_POINT('Ctrl Pts',(6.44950004849653,-12.4582489082855,8.45404171252757));
#57846=CARTESIAN_POINT('Ctrl Pts',(6.47553829213457,-12.4587308389966,8.43937781738155));
#57847=CARTESIAN_POINT('Ctrl Pts',(6.52301980353868,-12.4596096539763,8.41263776861777));
#57848=CARTESIAN_POINT('Ctrl Pts',(6.56948206886044,-12.4615968089396,8.38441151778665));
#57849=CARTESIAN_POINT('Ctrl Pts',(6.61495853931863,-12.4646596198119,8.35471776067509));
#57850=CARTESIAN_POINT('Ctrl Pts',(6.62617140476325,-12.4654147990474,8.34739634589328));
#57851=CARTESIAN_POINT('Ctrl Pts',(6.63732421927012,-12.4662355009643,8.33998554122602));
#57852=CARTESIAN_POINT('Ctrl Pts',(6.64841723331421,-12.467121485517,8.33248529664793));
#57853=CARTESIAN_POINT('Ctrl Pts',(6.69398634271207,-12.4707610308061,8.301674962835));
#57854=CARTESIAN_POINT('Ctrl Pts',(6.73853003492269,-12.4755031700154,8.26936384606336));
#57855=CARTESIAN_POINT('Ctrl Pts',(6.78203915041949,-12.4813450910741,8.23553650332579));
#57856=CARTESIAN_POINT('Ctrl Pts',(6.82408117528156,-12.4869900274878,8.20284979002096));
#57857=CARTESIAN_POINT('Ctrl Pts',(6.86515751416727,-12.4936620603136,8.16874687499731));
#57858=CARTESIAN_POINT('Ctrl Pts',(6.90522598975078,-12.5013798136185,8.13319060703869));
#57859=CARTESIAN_POINT('Ctrl Pts',(6.93747899993367,-12.5075921981004,8.10456968608188));
#57860=CARTESIAN_POINT('Ctrl Pts',(6.96907832789861,-12.514482605464,8.07500655154155));
#57861=CARTESIAN_POINT('Ctrl Pts',(7.0000006857802,-12.5220636286664,8.04447631542505));
#57862=CARTESIAN_POINT('',(6.26385800258875,-13.9442712228614,8.42072567770104));
#57863=CARTESIAN_POINT('Origin',(6.52767709685874,-13.2547595885169,9.09522362637851));
#57864=CARTESIAN_POINT('Ctrl Pts',(6.26385556499199,-13.9442775931717,8.42071944622816));
#57865=CARTESIAN_POINT('Ctrl Pts',(6.30364986918725,-13.9340686569687,8.3947165152949));
#57866=CARTESIAN_POINT('Ctrl Pts',(6.34303408262301,-13.9248559416285,8.36600596164334));
#57867=CARTESIAN_POINT('Ctrl Pts',(6.38165189810817,-13.916706545455,8.33460109009556));
#57868=CARTESIAN_POINT('Ctrl Pts',(6.42679322248454,-13.9071805137124,8.29789115516716));
#57869=CARTESIAN_POINT('Ctrl Pts',(6.47088804817601,-13.8991074859413,8.25749861371456));
#57870=CARTESIAN_POINT('Ctrl Pts',(6.5134097964521,-13.8925137453288,8.21357735272315));
#57871=CARTESIAN_POINT('Ctrl Pts',(6.53319105122902,-13.8894463158774,8.19314504010624));
#57872=CARTESIAN_POINT('Ctrl Pts',(6.55263123592839,-13.8866991949207,8.17194929236314));
#57873=CARTESIAN_POINT('Ctrl Pts',(6.57167372767561,-13.8842762175336,8.15000655423389));
#57874=CARTESIAN_POINT('Ctrl Pts',(6.58329061004541,-13.8827980788707,8.13662037499314));
#57875=CARTESIAN_POINT('Ctrl Pts',(6.59475945253126,-13.881440596437,8.12295619689224));
#57876=CARTESIAN_POINT('Ctrl Pts',(6.60606692691309,-13.8802048332916,8.1090178202598));
#57877=CARTESIAN_POINT('Ctrl Pts',(6.64408883391461,-13.8760495224057,8.0621493824305));
#57878=CARTESIAN_POINT('Ctrl Pts',(6.68028935710774,-13.8732694357406,8.01217942416458));
#57879=CARTESIAN_POINT('Ctrl Pts',(6.71423356137519,-13.8718345738079,7.95935553048294));
#57880=CARTESIAN_POINT('Ctrl Pts',(6.73210548380837,-13.871079106366,7.93154328533327));
#57881=CARTESIAN_POINT('Ctrl Pts',(6.74935123905505,-13.8706967808737,7.90294015228878));
#57882=CARTESIAN_POINT('Ctrl Pts',(6.76590192403628,-13.8706852165941,7.87358370287777));
#57883=CARTESIAN_POINT('Ctrl Pts',(6.77350230243503,-13.8706799060647,7.86010268235081));
#57884=CARTESIAN_POINT('Ctrl Pts',(6.7809560457977,-13.8707528051892,7.84646281264733));
#57885=CARTESIAN_POINT('Ctrl Pts',(6.78825616054251,-13.870903806069,7.8326677959974));
#57886=CARTESIAN_POINT('Ctrl Pts',(6.79013419613901,-13.8709426527224,7.82911887475046));
#57887=CARTESIAN_POINT('Ctrl Pts',(6.79200206297191,-13.8709866688481,7.82555968552902));
#57888=CARTESIAN_POINT('Ctrl Pts',(6.79385967091336,-13.8710358344652,7.82199031382253));
#57889=CARTESIAN_POINT('Ctrl Pts',(6.7983988300735,-13.8711559731425,7.81326837313962));
#57890=CARTESIAN_POINT('Ctrl Pts',(6.80287674779809,-13.8713068589087,7.80448560945556));
#57891=CARTESIAN_POINT('Ctrl Pts',(6.80729207758989,-13.871488207311,7.79564330332061));
#57892=CARTESIAN_POINT('Ctrl Pts',(6.80949974248579,-13.8715788815121,7.79122215025313));
#57893=CARTESIAN_POINT('Ctrl Pts',(6.81169175993162,-13.8716771712627,7.78678611169662));
#57894=CARTESIAN_POINT('Ctrl Pts',(6.8138679617779,-13.8717830418694,7.7823353433877));
#57895=CARTESIAN_POINT('Ctrl Pts',(6.81548499128459,-13.8718617091563,7.77902819442299));
#57896=CARTESIAN_POINT('Ctrl Pts',(6.81751780310369,-13.8719669126278,7.77483363831133));
#57897=CARTESIAN_POINT('Ctrl Pts',(6.81901903974428,-13.8720493090388,7.7717112155293));
#57898=CARTESIAN_POINT('Ctrl Pts',(6.81953817065756,-13.8720778018979,7.77063147490302));
#57899=CARTESIAN_POINT('Ctrl Pts',(6.81999417830938,-13.8721033441437,7.76968019404295));
#57900=CARTESIAN_POINT('Ctrl Pts',(6.82034895003808,-13.8721233622159,7.76893900667714));
#57901=CARTESIAN_POINT('Ctrl Pts',(6.83460306900321,-13.8729276539882,7.73915937083463));
#57902=CARTESIAN_POINT('Ctrl Pts',(6.84880155763395,-13.874076872251,7.70735440476999));
#57903=CARTESIAN_POINT('Ctrl Pts',(6.86266124201387,-13.8756671067256,7.67346133410921));
#57904=CARTESIAN_POINT('Ctrl Pts',(6.87577619130936,-13.8771718916782,7.64138947078245));
#57905=CARTESIAN_POINT('Ctrl Pts',(6.88858789184152,-13.879071573022,7.60744770501848));
#57906=CARTESIAN_POINT('Ctrl Pts',(6.90081551644704,-13.8814491338862,7.57160537737455));
#57907=CARTESIAN_POINT('Ctrl Pts',(6.90556286907159,-13.8823722174918,7.5576896599969));
#57908=CARTESIAN_POINT('Ctrl Pts',(6.91022171578473,-13.8833673525982,7.54348772154589));
#57909=CARTESIAN_POINT('Ctrl Pts',(6.91477373911994,-13.8844394701365,7.52899884039857));
#57910=CARTESIAN_POINT('Ctrl Pts',(6.92451243856034,-13.8867331821194,7.49800100749425));
#57911=CARTESIAN_POINT('Ctrl Pts',(6.93376338705338,-13.8893794429974,7.46568845724205));
#57912=CARTESIAN_POINT('Ctrl Pts',(6.9423487824454,-13.8924173078754,7.43207739625192));
#57913=CARTESIAN_POINT('Ctrl Pts',(6.95179578557956,-13.8957600448972,7.39509321742059));
#57914=CARTESIAN_POINT('Ctrl Pts',(6.96043782096829,-13.8995769584793,7.35653610866358));
#57915=CARTESIAN_POINT('Ctrl Pts',(6.96800709073418,-13.9039173172265,7.3164568676453));
#57916=CARTESIAN_POINT('Ctrl Pts',(6.97344669462717,-13.9070364863232,7.28765419549672));
#57917=CARTESIAN_POINT('Ctrl Pts',(6.97833164672333,-13.9104259232775,7.25806603815568));
#57918=CARTESIAN_POINT('Ctrl Pts',(6.98254998067605,-13.9141031142514,7.22772233871471));
#57919=CARTESIAN_POINT('Ctrl Pts',(6.98802445798619,-13.9188753060166,7.18834283582162));
#57920=CARTESIAN_POINT('Ctrl Pts',(6.99237688811927,-13.9241325304546,7.14768911906493));
#57921=CARTESIAN_POINT('Ctrl Pts',(6.99536960209117,-13.9298949208174,7.10587570796624));
#57922=CARTESIAN_POINT('Ctrl Pts',(6.99836231606306,-13.9356573111802,7.06406229686755));
#57923=CARTESIAN_POINT('Ctrl Pts',(6.9999959467022,-13.9419248200711,7.02108887996642));
#57924=CARTESIAN_POINT('Ctrl Pts',(6.99999920776358,-13.9487123452195,6.97710990114864));
#57925=CARTESIAN_POINT('Ctrl Pts',(6.99990231887538,-13.8881494970745,6.87915686262218));
#57926=CARTESIAN_POINT('Ctrl Pts',(6.99990231887538,-14.0922215836893,7.13653119174548));
#57927=CARTESIAN_POINT('Ctrl Pts',(6.99990231887538,-14.6760168117915,7.80839106751792));
#57928=CARTESIAN_POINT('Ctrl Pts',(6.99990231887538,-15.7555521603482,8.78349827542946));
#57929=CARTESIAN_POINT('Ctrl Pts',(6.99990231887538,-17.1681240962604,9.71000741139101));
#57930=CARTESIAN_POINT('Ctrl Pts',(6.99990231887538,-18.7078310635836,10.4112072238231));
#57931=CARTESIAN_POINT('Ctrl Pts',(6.99990231887538,-20.3372561090755,10.8675680762032));
#57932=CARTESIAN_POINT('Ctrl Pts',(6.99990231887538,-22.0150940179141,11.0696961448058));
#57933=CARTESIAN_POINT('Ctrl Pts',(6.99990231887538,-23.3220434090589,11.025041445511));
#57934=CARTESIAN_POINT('Ctrl Pts',(6.99990231887538,-24.0577258216087,10.9251841086137));
#57935=CARTESIAN_POINT('Ctrl Pts',(6.99990231887538,-24.2367488249382,10.8963634460966));
#57936=CARTESIAN_POINT('Ctrl Pts',(7.00658753983221,-13.5133853982884,7.17628812110414));
#57937=CARTESIAN_POINT('Ctrl Pts',(7.00658753983221,-13.7263815573694,7.44491987418102));
#57938=CARTESIAN_POINT('Ctrl Pts',(7.00658753983221,-14.335562627462,8.14597361895549));
#57939=CARTESIAN_POINT('Ctrl Pts',(7.00658753983221,-15.461958137829,9.16342028926661));
#57940=CARTESIAN_POINT('Ctrl Pts',(7.00658753983221,-16.9363739076172,10.1305345660181));
#57941=CARTESIAN_POINT('Ctrl Pts',(7.00658753983221,-18.5431139524402,10.8622018415741));
#57942=CARTESIAN_POINT('Ctrl Pts',(7.00658753983221,-20.2433891695497,11.3384606731685));
#57943=CARTESIAN_POINT('Ctrl Pts',(7.00658753983221,-21.9947090334009,11.5494067320141));
#57944=CARTESIAN_POINT('Ctrl Pts',(7.00658753983221,-23.3583198226927,11.502805648718));
#57945=CARTESIAN_POINT('Ctrl Pts',(7.00658753983221,-24.1259502087164,11.3986200459028));
#57946=CARTESIAN_POINT('Ctrl Pts',(7.00658753983221,-24.3127635599996,11.3685459961419));
#57947=CARTESIAN_POINT('Ctrl Pts',(6.71725767918123,-13.214799698687,7.41302142873519));
#57948=CARTESIAN_POINT('Ctrl Pts',(6.71725767918123,-13.4349059316249,7.69062230617901));
#57949=CARTESIAN_POINT('Ctrl Pts',(6.71725767918123,-14.0643126567709,8.41493567435489));
#57950=CARTESIAN_POINT('Ctrl Pts',(6.71725767918123,-15.2280430512571,9.46611545314552));
#57951=CARTESIAN_POINT('Ctrl Pts',(6.71725767918123,-16.7517316421631,10.4655810527814));
#57952=CARTESIAN_POINT('Ctrl Pts',(6.71725767918123,-18.4118789327983,11.2215226620502));
#57953=CARTESIAN_POINT('Ctrl Pts',(6.71725767918123,-20.1686025880746,11.7136348052723));
#57954=CARTESIAN_POINT('Ctrl Pts',(6.71725767918123,-21.9784677101774,11.9316064191023));
#57955=CARTESIAN_POINT('Ctrl Pts',(6.71725767918123,-23.3872223199659,11.883454593803));
#57956=CARTESIAN_POINT('Ctrl Pts',(6.71725767918123,-24.1803066063053,11.7758205328527));
#57957=CARTESIAN_POINT('Ctrl Pts',(6.71725767918123,-24.3733267594099,11.7447478722026));
#57958=CARTESIAN_POINT('Ctrl Pts',(6.25443115695018,-13.1193849311526,7.48867091075995));
#57959=CARTESIAN_POINT('Ctrl Pts',(6.25443115695018,-13.3417632288447,7.76913792317712));
#57960=CARTESIAN_POINT('Ctrl Pts',(6.25443115695018,-13.9776331777085,8.50088403700404));
#57961=CARTESIAN_POINT('Ctrl Pts',(6.25443115695018,-15.1532941478884,9.56284342348165));
#57962=CARTESIAN_POINT('Ctrl Pts',(6.25443115695018,-16.6927281505116,10.5726470733296));
#57963=CARTESIAN_POINT('Ctrl Pts',(6.25443115695018,-18.3699420319087,11.3363456847244));
#57964=CARTESIAN_POINT('Ctrl Pts',(6.25443115695018,-20.1447041083536,11.8335238443235));
#57965=CARTESIAN_POINT('Ctrl Pts',(6.25443115695018,-21.9732777024755,12.0537405144227));
#57966=CARTESIAN_POINT('Ctrl Pts',(6.25443115695018,-23.3964582782285,12.0050931406458));
#57967=CARTESIAN_POINT('Ctrl Pts',(6.25443115695018,-24.1976765039544,11.8963571051786));
#57968=CARTESIAN_POINT('Ctrl Pts',(6.25443115695018,-24.3926800760654,11.864965332708));
#57969=CARTESIAN_POINT('Ctrl Pts',(6.99999999975193,-13.9487123452043,6.97710990119063));
#57970=CARTESIAN_POINT('Ctrl Pts',(6.99999999975356,-14.0537865445291,7.10682522671275));
#57971=CARTESIAN_POINT('Ctrl Pts',(6.99999999939392,-14.1614773187861,7.23374878526825));
#57972=CARTESIAN_POINT('Ctrl Pts',(6.9999999987102,-14.271796727239,7.35798005418243));
#57973=CARTESIAN_POINT('Ctrl Pts',(6.99999999819793,-14.3544522543465,7.45105888010567));
#57974=CARTESIAN_POINT('Ctrl Pts',(6.99999999754858,-14.4385843437506,7.54262579415969));
#57975=CARTESIAN_POINT('Ctrl Pts',(6.99999999746792,-14.5242127791809,7.63271038363396));
#57976=CARTESIAN_POINT('Ctrl Pts',(6.99999999735988,-14.6388965267303,7.7533623407257));
#57977=CARTESIAN_POINT('Ctrl Pts',(6.99999999919156,-14.7562632766479,7.87135693200949));
#57978=CARTESIAN_POINT('Ctrl Pts',(6.99999999987966,-14.8764168439348,7.98675539947756));
#57979=CARTESIAN_POINT('Ctrl Pts',(6.9999999999543,-14.889450370199,7.99927312151074));
#57980=CARTESIAN_POINT('Ctrl Pts',(7.0000000000004,-14.9025167201923,8.01176025725755));
#57981=CARTESIAN_POINT('Ctrl Pts',(7.0000000000004,-14.9156160496649,8.02421685618018));
#57982=CARTESIAN_POINT('Ctrl Pts',(7.0000000000004,-15.0670348546121,8.16820615933681));
#57983=CARTESIAN_POINT('Ctrl Pts',(6.99999999546748,-15.2227875870624,8.30815817490327));
#57984=CARTESIAN_POINT('Ctrl Pts',(6.99999999503653,-15.3825084355945,8.44364293588376));
#57985=CARTESIAN_POINT('Ctrl Pts',(6.99999999469253,-15.5100021830308,8.55179074536915));
#57986=CARTESIAN_POINT('Ctrl Pts',(6.9999999963596,-15.640023426811,8.65709269262027));
#57987=CARTESIAN_POINT('Ctrl Pts',(6.99999999805392,-15.7723691311277,8.75934684041249));
#57988=CARTESIAN_POINT('Ctrl Pts',(6.99999999906437,-15.8512969250208,8.82032875397988));
#57989=CARTESIAN_POINT('Ctrl Pts',(7.0000000000004,-15.9310511663872,8.88022697138982));
#57990=CARTESIAN_POINT('Ctrl Pts',(7.0000000000004,-16.0115798553702,8.93900894895164));
#57991=CARTESIAN_POINT('Ctrl Pts',(7.0000000000004,-16.2272079359332,9.09640682979922));
#57992=CARTESIAN_POINT('Ctrl Pts',(6.9999999976986,-16.4484492824618,9.24573591234888));
#57993=CARTESIAN_POINT('Ctrl Pts',(6.9999999985899,-16.6747881471727,9.38679488637287));
#57994=CARTESIAN_POINT('Ctrl Pts',(6.99999999924458,-16.8410388017354,9.4904056683452));
#57995=CARTESIAN_POINT('Ctrl Pts',(6.99999999995148,-17.0100406501369,9.58955400758841));
#57996=CARTESIAN_POINT('Ctrl Pts',(6.99999999999604,-17.1816029459403,9.68414853143226));
#57997=CARTESIAN_POINT('Ctrl Pts',(6.99999999999906,-17.1932035655252,9.69054477998316));
#57998=CARTESIAN_POINT('Ctrl Pts',(7.0000000000004,-17.204815895814,9.69692020378814));
#57999=CARTESIAN_POINT('Ctrl Pts',(7.0000000000004,-17.2164398762232,9.70327477688506));
#58000=CARTESIAN_POINT('Ctrl Pts',(7.0000000000004,-17.5356664538813,9.8777888891596));
#58001=CARTESIAN_POINT('Ctrl Pts',(6.9999999999951,-17.8636599576002,10.0365925445825));
#58002=CARTESIAN_POINT('Ctrl Pts',(6.9999999999726,-18.1987775349499,10.1787296000036));
#58003=CARTESIAN_POINT('Ctrl Pts',(6.99999999996567,-18.3020189970942,10.2225185219175));
#58004=CARTESIAN_POINT('Ctrl Pts',(7.0000000000004,-18.4059362502178,10.2647257190842));
#58005=CARTESIAN_POINT('Ctrl Pts',(7.0000000000004,-18.5104803250287,10.3053235815522));
#58006=CARTESIAN_POINT('Ctrl Pts',(7.0000000000004,-18.5793538172857,10.3320693973376));
#58007=CARTESIAN_POINT('Ctrl Pts',(6.99999999997084,-18.6484986914509,10.3581192795794));
#58008=CARTESIAN_POINT('Ctrl Pts',(6.99999999992955,-18.7179006488757,10.3834661744317));
#58009=CARTESIAN_POINT('Ctrl Pts',(6.99999999970469,-19.0957945309358,10.5214800986681));
#58010=CARTESIAN_POINT('Ctrl Pts',(7.0000000000004,-19.481310861725,10.6386470274233));
#58011=CARTESIAN_POINT('Ctrl Pts',(7.0000000000004,-19.8719302299936,10.7344092108449));
#58012=CARTESIAN_POINT('Ctrl Pts',(7.0000000000004,-20.028335196057,10.7727526271343));
#58013=CARTESIAN_POINT('Ctrl Pts',(6.99999999962046,-20.1855590343142,10.8076629791835));
#58014=CARTESIAN_POINT('Ctrl Pts',(6.9999999991226,-20.3434794936074,10.8391040063824));
#58015=CARTESIAN_POINT('Ctrl Pts',(6.9999999982468,-20.6212770476484,10.894411852443));
#58016=CARTESIAN_POINT('Ctrl Pts',(6.99999999886194,-20.9012308716709,10.9389870155385));
#58017=CARTESIAN_POINT('Ctrl Pts',(6.99999999981873,-21.1826749476473,10.9726474512991));
#58018=CARTESIAN_POINT('Ctrl Pts',(6.99999999992592,-21.2142039018405,10.9764182833323));
#58019=CARTESIAN_POINT('Ctrl Pts',(7.0000000000004,-21.2457515479638,10.9800520854491));
#58020=CARTESIAN_POINT('Ctrl Pts',(7.0000000000004,-21.2773169407793,10.9835485617856));
#58021=CARTESIAN_POINT('Ctrl Pts',(7.0000000000004,-21.4971771481314,11.007902322147));
#58022=CARTESIAN_POINT('Ctrl Pts',(6.99999999634339,-21.7179002558227,11.0256402092761));
#58023=CARTESIAN_POINT('Ctrl Pts',(6.99999999542,-21.9388779061459,11.0366879235032));
#58024=CARTESIAN_POINT('Ctrl Pts',(6.9999999953102,-21.9651560171461,11.0380016901232));
#58025=CARTESIAN_POINT('Ctrl Pts',(6.99999999523508,-21.991437727015,11.0392209091003));
#58026=CARTESIAN_POINT('Ctrl Pts',(6.99999999519962,-22.0177220131473,11.0403455046552));
#58027=CARTESIAN_POINT('Ctrl Pts',(6.99999999489106,-22.2464396793239,11.0501313846829));
#58028=CARTESIAN_POINT('Ctrl Pts',(7.0000000000004,-22.4753517979991,11.0527476023975));
#58029=CARTESIAN_POINT('Ctrl Pts',(7.0000000000004,-22.7037893032828,11.0482957738581));
#58030=CARTESIAN_POINT('Ctrl Pts',(7.0000000000004,-22.8739866007358,11.0449789402883));
#58031=CARTESIAN_POINT('Ctrl Pts',(6.99999999741537,-23.0439121332079,11.0376823617801));
#58032=CARTESIAN_POINT('Ctrl Pts',(6.99999999745857,-23.2136663743515,11.0264413935634));
#58033=CARTESIAN_POINT('Ctrl Pts',(6.99999999749981,-23.3756611564429,11.0157142495198));
#58034=CARTESIAN_POINT('Ctrl Pts',(6.99999999865199,-23.5375002857097,11.0013947135119));
#58035=CARTESIAN_POINT('Ctrl Pts',(6.99999999924109,-23.6992706986834,10.9834692572149));
#58036=CARTESIAN_POINT('Ctrl Pts',(6.99999999975915,-23.8415340467228,10.9677053398146));
#58037=CARTESIAN_POINT('Ctrl Pts',(6.99999999990903,-23.9837444368193,10.9491520850644));
#58038=CARTESIAN_POINT('Ctrl Pts',(6.99999999989437,-24.1259362010629,10.9277733094969));
#58039=CARTESIAN_POINT('Ctrl Pts',(6.26386081916884,-13.9442638623473,8.42073287747484));
#58040=CARTESIAN_POINT('Ctrl Pts',(6.26460715538793,-14.1256643553291,8.60589469623759));
#58041=CARTESIAN_POINT('Ctrl Pts',(6.26531568179332,-14.3114846099631,8.78358334204671));
#58042=CARTESIAN_POINT('Ctrl Pts',(6.26598638151121,-14.5010840416007,8.95374216520787));
#58043=CARTESIAN_POINT('Ctrl Pts',(6.26666473066603,-14.6928458849018,9.1258416768018));
#58044=CARTESIAN_POINT('Ctrl Pts',(6.2673043853985,-14.8884736297165,9.29023867958107));
#58045=CARTESIAN_POINT('Ctrl Pts',(6.26790533159812,-15.0873464622826,9.4469072536487));
#58046=CARTESIAN_POINT('Ctrl Pts',(6.26800176179048,-15.1192583797085,9.47204690965087));
#58047=CARTESIAN_POINT('Ctrl Pts',(6.2680971952959,-15.1512539400177,9.49698763549614));
#58048=CARTESIAN_POINT('Ctrl Pts',(6.26819163206334,-15.1833306763749,9.52172939986302));
#58049=CARTESIAN_POINT('Ctrl Pts',(6.26876871803122,-15.3793457979045,9.67292183712407));
#58050=CARTESIAN_POINT('Ctrl Pts',(6.26930858350217,-15.5783882018843,9.81668297483491));
#58051=CARTESIAN_POINT('Ctrl Pts',(6.26981121831375,-15.7798035976635,9.95308941123838));
#58052=CARTESIAN_POINT('Ctrl Pts',(6.27017912497558,-15.9272308434424,10.0529329467719));
#58053=CARTESIAN_POINT('Ctrl Pts',(6.27052708500013,-16.0759304839668,10.148836571751));
#58054=CARTESIAN_POINT('Ctrl Pts',(6.27085509519045,-16.2256622310779,10.2408371358993));
#58055=CARTESIAN_POINT('Ctrl Pts',(6.27121137948388,-16.3883006834675,10.3407680434105));
#58056=CARTESIAN_POINT('Ctrl Pts',(6.27154412512549,-16.5521566156048,10.436093917001));
#58057=CARTESIAN_POINT('Ctrl Pts',(6.27185332803515,-16.7169398449731,10.5268692971855));
#58058=CARTESIAN_POINT('Ctrl Pts',(6.27227096956888,-16.9395131730253,10.6494799448244));
#58059=CARTESIAN_POINT('Ctrl Pts',(6.27264565965075,-17.1637762166304,10.7637883382869));
#58060=CARTESIAN_POINT('Ctrl Pts',(6.27297739034783,-17.3890719580496,10.8699987576102));
#58061=CARTESIAN_POINT('Ctrl Pts',(6.27330912104492,-17.6143676994688,10.9762091769336));
#58062=CARTESIAN_POINT('Ctrl Pts',(6.27359789237642,-17.840696315615,11.0743217071008));
#58063=CARTESIAN_POINT('Ctrl Pts',(6.27384369855202,-18.0674568527804,11.164557360519));
#58064=CARTESIAN_POINT('Ctrl Pts',(6.27395596457378,-18.1710242401169,11.2057703113523));
#58065=CARTESIAN_POINT('Ctrl Pts',(6.27405926819507,-18.2746824802254,11.2453403802785));
#58066=CARTESIAN_POINT('Ctrl Pts',(6.27415361604219,-18.3783780729687,11.283289714812));
#58067=CARTESIAN_POINT('Ctrl Pts',(6.27415652049381,-18.3815702902948,11.2844579662295));
#58068=CARTESIAN_POINT('Ctrl Pts',(6.27415941639736,-18.3847625430648,11.2856246817208));
#58069=CARTESIAN_POINT('Ctrl Pts',(6.27416230375866,-18.3879548297647,11.2867898619452));
#58070=CARTESIAN_POINT('Ctrl Pts',(6.27420631274101,-18.4366114662014,11.3045494668581));
#58071=CARTESIAN_POINT('Ctrl Pts',(6.27424833721605,-18.4852759753122,11.3219524031927));
#58072=CARTESIAN_POINT('Ctrl Pts',(6.27428839779756,-18.5339427586306,11.3390018888015));
#58073=CARTESIAN_POINT('Ctrl Pts',(6.27431785032599,-18.5697225642477,11.351536665899));
#58074=CARTESIAN_POINT('Ctrl Pts',(6.27434670203493,-18.6061342790989,11.364096691144));
#58075=CARTESIAN_POINT('Ctrl Pts',(6.27437398879412,-18.6418708872981,11.3762338190514));
#58076=CARTESIAN_POINT('Ctrl Pts',(6.27438625183395,-18.6579314039148,11.3816884090155));
#58077=CARTESIAN_POINT('Ctrl Pts',(6.27439819879666,-18.6738553337517,11.3870582624603));
#58078=CARTESIAN_POINT('Ctrl Pts',(6.27440974216804,-18.6895229537664,11.3923059388776));
#58079=CARTESIAN_POINT('Ctrl Pts',(6.2745606464126,-18.8943426971077,11.4609077900793));
#58080=CARTESIAN_POINT('Ctrl Pts',(6.27467736446985,-19.1037514751474,11.5248694916449));
#58081=CARTESIAN_POINT('Ctrl Pts',(6.27475989460005,-19.3175737472424,11.5836612187159));
#58082=CARTESIAN_POINT('Ctrl Pts',(6.27484107125348,-19.5278893790404,11.6414887738264));
#58083=CARTESIAN_POINT('Ctrl Pts',(6.27488917214012,-19.7424750147591,11.6943145252498));
#58084=CARTESIAN_POINT('Ctrl Pts',(6.27490419657665,-19.9611187691495,11.7416109919988));
#58085=CARTESIAN_POINT('Ctrl Pts',(6.27490863040175,-20.0256421983445,11.7555685378339));
#58086=CARTESIAN_POINT('Ctrl Pts',(6.27491018365523,-20.0905187370529,11.7690443907007));
#58087=CARTESIAN_POINT('Ctrl Pts',(6.27490885633516,-20.1557421590437,11.7820245992169));
#58088=CARTESIAN_POINT('Ctrl Pts',(6.27490450759592,-20.3694356466198,11.8245520524328));
#58089=CARTESIAN_POINT('Ctrl Pts',(6.27486923773407,-20.5868563220246,11.8617604278984));
#58090=CARTESIAN_POINT('Ctrl Pts',(6.27480304721734,-20.8077282531982,11.8931697209086));
#58091=CARTESIAN_POINT('Ctrl Pts',(6.27475276868315,-20.9755032984753,11.9170283231715));
#58092=CARTESIAN_POINT('Ctrl Pts',(6.27468464903527,-21.1452687904443,11.9375405125988));
#58093=CARTESIAN_POINT('Ctrl Pts',(6.27459868879999,-21.3168849074982,11.9544888627757));
#58094=CARTESIAN_POINT('Ctrl Pts',(6.27448994477113,-21.5339879426928,11.9759293797162));
#58095=CARTESIAN_POINT('Ctrl Pts',(6.27435264840743,-21.7540541848264,11.9916670215249));
#58096=CARTESIAN_POINT('Ctrl Pts',(6.27418680218902,-21.9767610896238,12.0012473074002));
#58097=CARTESIAN_POINT('Ctrl Pts',(6.27401315229541,-22.2099471742547,12.0112783809986));
#58098=CARTESIAN_POINT('Ctrl Pts',(6.27380820257276,-22.4460283952983,12.0145579437078));
#58099=CARTESIAN_POINT('Ctrl Pts',(6.27357195679918,-22.6846248575645,12.0106606645995));
#58100=CARTESIAN_POINT('Ctrl Pts',(6.27333930405051,-22.9195925436593,12.0068226585978));
#58101=CARTESIAN_POINT('Ctrl Pts',(6.27307629996098,-23.156999600613,11.9960244224841));
#58102=CARTESIAN_POINT('Ctrl Pts',(6.27278294912994,-23.3964330132993,11.9778552766724));
#58103=CARTESIAN_POINT('Ctrl Pts',(6.27261681982308,-23.5320280165442,11.9675657963629));
#58104=CARTESIAN_POINT('Ctrl Pts',(6.27244095791103,-23.6682719810853,11.9549122836599));
#58105=CARTESIAN_POINT('Ctrl Pts',(6.27225536438287,-23.8050824682318,11.9398195552085));
#58106=CARTESIAN_POINT('Ctrl Pts',(6.27204648910949,-23.9590551211918,11.9228335222769));
#58107=CARTESIAN_POINT('Ctrl Pts',(6.27182528751364,-24.1137456239823,11.9027579534488));
#58108=CARTESIAN_POINT('Ctrl Pts',(6.27159176118849,-24.269011967666,11.87948072114));
#58109=CARTESIAN_POINT('Ctrl Pts',(-6.390310997256,-13.7249660551165,8.13937950337913));
#58110=CARTESIAN_POINT('Ctrl Pts',(-4.260207331504,-13.822173858898,9.11426650159885));
#58111=CARTESIAN_POINT('Ctrl Pts',(0.0001535201704872,-13.9182984617654,
10.0902631575042));
#58112=CARTESIAN_POINT('Ctrl Pts',(4.260514371845,-13.8221669310363,9.11419615987158));
#58113=CARTESIAN_POINT('Ctrl Pts',(6.390771557767,-13.7249450365591,8.1391687105328));
#58114=CARTESIAN_POINT('Ctrl Pts',(-6.390310997256,-14.2543287817417,8.7130969045735));
#58115=CARTESIAN_POINT('Ctrl Pts',(-4.260207331504,-14.3567676707194,9.62713419180754));
#58116=CARTESIAN_POINT('Ctrl Pts',(0.0001535201704872,-14.4578350530966,
10.5425537312277));
#58117=CARTESIAN_POINT('Ctrl Pts',(4.260514371845,-14.3567603866204,9.62706821596995));
#58118=CARTESIAN_POINT('Ctrl Pts',(6.390771557767,-14.2543066321015,8.71289926882854));
#58119=CARTESIAN_POINT('Ctrl Pts',(-6.390310997256,-15.6641218055026,9.9697330099508));
#58120=CARTESIAN_POINT('Ctrl Pts',(-4.260207331504,-15.7526919792921,10.7489906364295));
#58121=CARTESIAN_POINT('Ctrl Pts',(0.0001535201704857,-15.8421753984647,
11.5273040839031));
#58122=CARTESIAN_POINT('Ctrl Pts',(4.260514371845,-15.7526855300687,10.7489345420609));
#58123=CARTESIAN_POINT('Ctrl Pts',(6.390771557767,-15.6641026546149,9.96956451662773));
#58124=CARTESIAN_POINT('Ctrl Pts',(-6.390310997256,-18.3168609125049,11.387980958503));
#58125=CARTESIAN_POINT('Ctrl Pts',(-4.260207331504,-18.3050659003902,12.0191857141868));
#58126=CARTESIAN_POINT('Ctrl Pts',(0.0001535201704865,-18.2929947853426,
12.6510838649568));
#58127=CARTESIAN_POINT('Ctrl Pts',(4.260514371845,-18.3050667703783,12.019140172221));
#58128=CARTESIAN_POINT('Ctrl Pts',(6.390771557767,-18.3168634628512,11.3878444776082));
#58129=CARTESIAN_POINT('Ctrl Pts',(-6.390310997256,-21.4528914163396,12.0713618431172));
#58130=CARTESIAN_POINT('Ctrl Pts',(-4.260207331504,-21.2792389757099,12.6592425323955));
#58131=CARTESIAN_POINT('Ctrl Pts',(0.0001535201704863,-21.1056340488841,
13.2456889758127));
#58132=CARTESIAN_POINT('Ctrl Pts',(4.260514371845,-21.2792514877097,12.6592002662086));
#58133=CARTESIAN_POINT('Ctrl Pts',(6.390771557767,-21.4529289639657,12.0712347298623));
#58134=CARTESIAN_POINT('Ctrl Pts',(-6.390310997256,-23.5458951845813,11.9720502124476));
#58135=CARTESIAN_POINT('Ctrl Pts',(-4.260207331504,-23.2652553028773,12.6077625569466));
#58136=CARTESIAN_POINT('Ctrl Pts',(0.0001535201704863,-22.9846380445226,
13.2461450660854));
#58137=CARTESIAN_POINT('Ctrl Pts',(4.260514371845,-23.2652755274378,12.6077165476319));
#58138=CARTESIAN_POINT('Ctrl Pts',(6.390771557767,-23.5459558653483,11.9719127569248));
#58139=CARTESIAN_POINT('Ctrl Pts',(-6.390310997256,-24.5118462831682,11.8061936875796));
#58140=CARTESIAN_POINT('Ctrl Pts',(-4.260207331504,-24.187054612813,12.4817978962137));
#58141=CARTESIAN_POINT('Ctrl Pts',(0.0001535201704863,-23.8622603664262,
13.1582606881552));
#58142=CARTESIAN_POINT('Ctrl Pts',(4.260514371845,-24.187078021279,12.4817491423984));
#58143=CARTESIAN_POINT('Ctrl Pts',(6.390771557767,-24.5119165105465,11.8060476065166));
#58144=CARTESIAN_POINT('Ctrl Pts',(-6.26386059986259,-13.9442583573832,
8.42071137118441));
#58145=CARTESIAN_POINT('Ctrl Pts',(-5.97374970119676,-13.9556246846561,
8.54581702332281));
#58146=CARTESIAN_POINT('Ctrl Pts',(-5.68169246539988,-13.9653430040926,
8.66221523046253));
#58147=CARTESIAN_POINT('Ctrl Pts',(-5.38818163422549,-13.9736733100379,
8.76975971946819));
#58148=CARTESIAN_POINT('Ctrl Pts',(-5.1130280735255,-13.9814826073419,8.87057797195028));
#58149=CARTESIAN_POINT('Ctrl Pts',(-4.83659705802325,-13.9880722696807,
8.96361469734395));
#58150=CARTESIAN_POINT('Ctrl Pts',(-4.55929453756362,-13.993667873811,9.04879103044236));
#58151=CARTESIAN_POINT('Ctrl Pts',(-4.30183369063218,-13.9988630987808,
9.12787278859474));
#58152=CARTESIAN_POINT('Ctrl Pts',(-4.04362159347591,-14.0032015562529,
9.20017851794789));
#58153=CARTESIAN_POINT('Ctrl Pts',(-3.78498314220327,-14.0068718216736,
9.26568816177216));
#58154=CARTESIAN_POINT('Ctrl Pts',(-3.57030053449505,-14.0099183220977,
9.3200643811511));
#58155=CARTESIAN_POINT('Ctrl Pts',(-3.35532417670103,-14.0125045919245,
9.3697587733089));
#58156=CARTESIAN_POINT('Ctrl Pts',(-3.14023987314758,-14.0147423985495,
9.41478705629016));
#58157=CARTESIAN_POINT('Ctrl Pts',(-2.90175388934231,-14.017223683821,9.46471452281576));
#58158=CARTESIAN_POINT('Ctrl Pts',(-2.66312286525269,-14.0192917524254,
9.50892010592155));
#58159=CARTESIAN_POINT('Ctrl Pts',(-2.42459507108778,-14.0210013809793,
9.54737540544549));
#58160=CARTESIAN_POINT('Ctrl Pts',(-2.18947802829743,-14.0226865632502,
9.58528082579845));
#58161=CARTESIAN_POINT('Ctrl Pts',(-1.95446128433272,-14.0240235028694,
9.6175991989134));
#58162=CARTESIAN_POINT('Ctrl Pts',(-1.71978261078597,-14.0250694407982,
9.64435373630295));
#58163=CARTESIAN_POINT('Ctrl Pts',(-1.48662499776981,-14.0261085995218,
9.67093486521775));
#58164=CARTESIAN_POINT('Ctrl Pts',(-1.25380108699366,-14.0268605301828,
9.69202397759681));
#58165=CARTESIAN_POINT('Ctrl Pts',(-1.02154405662948,-14.0273858808287,
9.70769485074321));
#58166=CARTESIAN_POINT('Ctrl Pts',(-0.790903926706924,-14.0279075741485,
9.72325662819648));
#58167=CARTESIAN_POINT('Ctrl Pts',(-0.560822811783745,-14.0282058441238,
9.7334753107035));
#58168=CARTESIAN_POINT('Ctrl Pts',(-0.331529053916802,-14.0283443468537,
9.73847438258332));
#58169=CARTESIAN_POINT('Ctrl Pts',(-0.220829317145543,-14.0284112139846,
9.74088786276849));
#58170=CARTESIAN_POINT('Ctrl Pts',(-0.110313099121724,-14.028440904815,
9.74208551519516));
#58171=CARTESIAN_POINT('Ctrl Pts',(-6.09486637782099E-6,-14.0284409294581,
9.74208557977705));
#58172=CARTESIAN_POINT('Ctrl Pts',(-4.06324399737009E-6,-14.0284409294585,
9.74208557977824));
#58173=CARTESIAN_POINT('Ctrl Pts',(-2.03162154622285E-6,-14.028440929459,
9.74208557977902));
#58174=CARTESIAN_POINT('Ctrl Pts',(9.73437423716373E-13,-14.0284409294594,
9.7420855797794));
#58175=CARTESIAN_POINT('Ctrl Pts',(0.230469086304145,-14.0284409786639,
9.7420856225606));
#58176=CARTESIAN_POINT('Ctrl Pts',(0.461828188180037,-14.0283111792431,
9.736854391521));
#58177=CARTESIAN_POINT('Ctrl Pts',(0.693853393917424,-14.0279844554711,
9.72624208054898));
#58178=CARTESIAN_POINT('Ctrl Pts',(0.927890614266204,-14.0276548985026,
9.71553774455464));
#58179=CARTESIAN_POINT('Ctrl Pts',(1.16260554084993,-14.0271249736896,9.69935860948583));
#58180=CARTESIAN_POINT('Ctrl Pts',(1.39776838632542,-14.0263301126495,9.67760396297315));
#58181=CARTESIAN_POINT('Ctrl Pts',(1.63451272885995,-14.0255299060779,9.65570301397203));
#58182=CARTESIAN_POINT('Ctrl Pts',(1.87171103515599,-14.0244611738864,9.62815137182254));
#58183=CARTESIAN_POINT('Ctrl Pts',(2.10912885058401,-14.0230625490103,9.59489921480226));
#58184=CARTESIAN_POINT('Ctrl Pts',(2.34955154624848,-14.0216462224287,9.56122620162479));
#58185=CARTESIAN_POINT('Ctrl Pts',(2.59019934264518,-14.0198915802255,9.52170750950915));
#58186=CARTESIAN_POINT('Ctrl Pts',(2.83082876986943,-14.0177397699997,9.47634475584401));
#58187=CARTESIAN_POINT('Ctrl Pts',(2.93381742979539,-14.016818801795,9.45692963582143));
#58188=CARTESIAN_POINT('Ctrl Pts',(3.03680272483088,-14.0158251417994,9.43644464777512));
#58189=CARTESIAN_POINT('Ctrl Pts',(3.13976556667399,-14.0147544567981,9.41489280609712));
#58190=CARTESIAN_POINT('Ctrl Pts',(3.40252021405499,-14.0120221365268,9.35989387192684));
#58191=CARTESIAN_POINT('Ctrl Pts',(3.66512390726434,-14.0087696417089,9.29792768492639));
#58192=CARTESIAN_POINT('Ctrl Pts',(3.92723730947002,-14.0047935953969,9.22896929728601));
#58193=CARTESIAN_POINT('Ctrl Pts',(4.19824548982516,-14.0006826225623,9.15767081732511));
#58194=CARTESIAN_POINT('Ctrl Pts',(4.46872953867013,-13.9957980909824,9.07889806286959));
#58195=CARTESIAN_POINT('Ctrl Pts',(4.73831438756763,-13.989924171619,8.99268353198578));
#58196=CARTESIAN_POINT('Ctrl Pts',(5.03386704909763,-13.9834844458385,8.89816436976476));
#58197=CARTESIAN_POINT('Ctrl Pts',(5.32833893619776,-13.9758553153082,8.79470102870764));
#58198=CARTESIAN_POINT('Ctrl Pts',(5.62123581932587,-13.966765452181,8.68240143317886));
#58199=CARTESIAN_POINT('Ctrl Pts',(5.83635809277611,-13.9600892731776,8.59992140116319));
#58200=CARTESIAN_POINT('Ctrl Pts',(6.05063074977934,-13.9526253913755,8.51267626970352));
#58201=CARTESIAN_POINT('Ctrl Pts',(6.26385797775638,-13.9442712877421,8.42072561436248));
#58202=CARTESIAN_POINT('Ctrl Pts',(-6.38246443203547,-13.9383908459212,
8.36787486373552));
#58203=CARTESIAN_POINT('Ctrl Pts',(-5.84028083115186,-13.9679405559834,
8.61420389076076));
#58204=CARTESIAN_POINT('Ctrl Pts',(-4.52658547446533,-14.0220197310707,
9.12779052120603));
#58205=CARTESIAN_POINT('Ctrl Pts',(-2.38698044041613,-14.0625412099017,
9.65161902433709));
#58206=CARTESIAN_POINT('Ctrl Pts',(0.000170347585844104,-14.074148905673,
9.84433435176279));
#58207=CARTESIAN_POINT('Ctrl Pts',(2.38732116864064,-14.0625376336816,9.6515638422071));
#58208=CARTESIAN_POINT('Ctrl Pts',(4.52680602897707,-14.0220126621885,9.12771374035583));
#58209=CARTESIAN_POINT('Ctrl Pts',(5.8403891997243,-13.9679346096076,8.61415461209718));
#58210=CARTESIAN_POINT('Ctrl Pts',(6.3824653352414,-13.9383907598281,8.36787438517324));
#58211=CARTESIAN_POINT('Ctrl Pts',(-6.17792169704451,-13.4668082109749,
7.96586380831044));
#58212=CARTESIAN_POINT('Ctrl Pts',(-5.65283597290228,-13.4968949842233,
8.20286290735405));
#58213=CARTESIAN_POINT('Ctrl Pts',(-4.38071778940755,-13.5523312148905,
8.69705174761694));
#58214=CARTESIAN_POINT('Ctrl Pts',(-2.30965986038465,-13.594711467794,9.20104086192968));
#58215=CARTESIAN_POINT('Ctrl Pts',(0.000164816889377721,-13.6071139576131,
9.38641545191658));
#58216=CARTESIAN_POINT('Ctrl Pts',(2.30998959809195,-13.5947076725133,9.20098777798778));
#58217=CARTESIAN_POINT('Ctrl Pts',(4.38093134257534,-13.5523239111862,8.69697786471346));
#58218=CARTESIAN_POINT('Ctrl Pts',(5.6529409239163,-13.496888930705,8.20281549558108));
#58219=CARTESIAN_POINT('Ctrl Pts',(6.17792257224339,-13.4668081241968,7.9658633476716));
#58220=CARTESIAN_POINT('Ctrl Pts',(-6.17627932975538,-12.819634948171,8.03444485753682));
#58221=CARTESIAN_POINT('Ctrl Pts',(-5.6525453615486,-12.8494142008257,8.26859095498002));
#58222=CARTESIAN_POINT('Ctrl Pts',(-4.38305006790979,-12.9043210586211,
8.75729081380155));
#58223=CARTESIAN_POINT('Ctrl Pts',(-2.31263925115347,-12.9463212003266,
9.25691132133251));
#58224=CARTESIAN_POINT('Ctrl Pts',(0.000165084886385522,-12.9586088807456,
9.44103069662757));
#58225=CARTESIAN_POINT('Ctrl Pts',(2.31296921096063,-12.9463174397802,9.25685862519176));
#58226=CARTESIAN_POINT('Ctrl Pts',(4.38326327239891,-12.9043138199759,8.75721768025679));
#58227=CARTESIAN_POINT('Ctrl Pts',(5.65265004295757,-12.8494082113494,8.26854411454389));
#58228=CARTESIAN_POINT('Ctrl Pts',(6.17628020062437,-12.8196348638585,8.03444440429756));
#58229=CARTESIAN_POINT('Ctrl Pts',(-6.37611008149986,-12.4394857929392,
8.52104497605786));
#58230=CARTESIAN_POINT('Ctrl Pts',(-5.83725935363331,-12.4683328075045,
8.76067527638475));
#58231=CARTESIAN_POINT('Ctrl Pts',(-4.53013633532534,-12.5212077719813,
9.26135585406044));
#58232=CARTESIAN_POINT('Ctrl Pts',(-2.39288391276903,-12.5608756708728,
9.77485740321018));
#58233=CARTESIAN_POINT('Ctrl Pts',(0.000170896469408238,-12.5722284770212,
9.96458495286569));
#58234=CARTESIAN_POINT('Ctrl Pts',(2.39322501551571,-12.5608721720362,9.77480314203578));
#58235=CARTESIAN_POINT('Ctrl Pts',(4.53035599764022,-12.5212008502468,9.26128083830177));
#58236=CARTESIAN_POINT('Ctrl Pts',(5.83736705737718,-12.4683270075272,8.76062733918381));
#58237=CARTESIAN_POINT('Ctrl Pts',(6.37611097436569,-12.4394857125263,8.52104451479218));
#58238=CARTESIAN_POINT('Ctrl Pts',(-6.24994453580111,-12.4626498782336,
8.5516892069173));
#58239=CARTESIAN_POINT('Ctrl Pts',(-5.92266396136831,-12.4795853537977,
8.69426559471729));
#58240=CARTESIAN_POINT('Ctrl Pts',(-5.59137421024021,-12.4941004954635,
8.82614963762332));
#58241=CARTESIAN_POINT('Ctrl Pts',(-5.25652165743914,-12.5066279941841,
8.94692518664224));
#58242=CARTESIAN_POINT('Ctrl Pts',(-5.07745905565674,-12.5133270815764,
9.01150998331803));
#58243=CARTESIAN_POINT('Ctrl Pts',(-4.89737714265432,-12.5194574385904,
9.07291754746856));
#58244=CARTESIAN_POINT('Ctrl Pts',(-4.71634131068421,-12.5250830890805,
9.13107930125512));
#58245=CARTESIAN_POINT('Ctrl Pts',(-4.71594239822594,-12.5250954852015,
9.1312074606804));
#58246=CARTESIAN_POINT('Ctrl Pts',(-4.71554348114866,-12.5251078788533,
9.13133560436434));
#58247=CARTESIAN_POINT('Ctrl Pts',(-4.7151445594529,-12.5251202700365,9.13146373230635));
#58248=CARTESIAN_POINT('Ctrl Pts',(-4.45574827245172,-12.5331775578975,
9.21477810896677));
#58249=CARTESIAN_POINT('Ctrl Pts',(-4.19440038798913,-12.5401916346868,
9.29143869421521));
#58250=CARTESIAN_POINT('Ctrl Pts',(-3.93132276388625,-12.546313096607,9.3612957382668));
#58251=CARTESIAN_POINT('Ctrl Pts',(-3.79958166025011,-12.5493785346198,
9.39627797634766));
#58252=CARTESIAN_POINT('Ctrl Pts',(-3.66740695004575,-12.5522194472211,
9.42955435298118));
#58253=CARTESIAN_POINT('Ctrl Pts',(-3.5348275049362,-12.5548507179461,9.46110763365611));
#58254=CARTESIAN_POINT('Ctrl Pts',(-3.46853778238143,-12.5561663533086,
9.47688427399358));
#58255=CARTESIAN_POINT('Ctrl Pts',(-3.4021468725808,-12.5574295616256,9.49223012786894));
#58256=CARTESIAN_POINT('Ctrl Pts',(-3.33565847252883,-12.558641923233,9.50714318309749));
#58257=CARTESIAN_POINT('Ctrl Pts',(-3.29270944041516,-12.5594250637142,
9.51677646179608));
#58258=CARTESIAN_POINT('Ctrl Pts',(-3.24894270553966,-12.5602006274725,
9.52639899722143));
#58259=CARTESIAN_POINT('Ctrl Pts',(-3.20586447642415,-12.5609423146399,
9.5356786207993));
#58260=CARTESIAN_POINT('Ctrl Pts',(-3.18225429860695,-12.5613488161666,
9.5407645671636));
#58261=CARTESIAN_POINT('Ctrl Pts',(-3.15885115696836,-12.5617452452138,
9.54574841261899));
#58262=CARTESIAN_POINT('Ctrl Pts',(-3.13590449255282,-12.5621279759528,
9.55058190565942));
#58263=CARTESIAN_POINT('Ctrl Pts',(-2.87752273695214,-12.5664375626741,
9.60500752477578));
#58264=CARTESIAN_POINT('Ctrl Pts',(-2.61833357770723,-12.5700171693122,
9.65275239225978));
#58265=CARTESIAN_POINT('Ctrl Pts',(-2.35853328291647,-12.5730079702202,
9.69372098322824));
#58266=CARTESIAN_POINT('Ctrl Pts',(-2.05844140245972,-12.5764626047473,
9.74104326018444));
#58267=CARTESIAN_POINT('Ctrl Pts',(-1.75753439943394,-12.5791314749656,
9.77932590839172));
#58268=CARTESIAN_POINT('Ctrl Pts',(-1.45620395938076,-12.5811117327101,
9.80856738526045));
#58269=CARTESIAN_POINT('Ctrl Pts',(-1.15288133180468,-12.583105082543,9.83800218645898));
#58270=CARTESIAN_POINT('Ctrl Pts',(-0.849129087484969,-12.5844006107004,
9.85827601809503));
#58271=CARTESIAN_POINT('Ctrl Pts',(-0.545330181918182,-12.5850917275183,
9.86933760207849));
#58272=CARTESIAN_POINT('Ctrl Pts',(-0.3635454901294,-12.5855052723185,9.87595654177276));
#58273=CARTESIAN_POINT('Ctrl Pts',(-0.181743814745408,-12.5857023049162,
9.87927608634575));
#58274=CARTESIAN_POINT('Ctrl Pts',(-5.66486730211472E-6,-12.5857020422594,
9.87927649696493));
#58275=CARTESIAN_POINT('Ctrl Pts',(5.22870906782938E-5,-12.5857020421756,
9.87927649709586));
#58276=CARTESIAN_POINT('Ctrl Pts',(0.000110239054679118,-12.585702042071,
9.87927649689034));
#58277=CARTESIAN_POINT('Ctrl Pts',(0.000168191024690234,-12.5857020419454,
9.87927649634836));
#58278=CARTESIAN_POINT('Ctrl Pts',(0.297743100998625,-12.5857013970017,
9.87927371333765));
#58279=CARTESIAN_POINT('Ctrl Pts',(0.595477788875134,-12.585149424772,9.87040370035765));
#58280=CARTESIAN_POINT('Ctrl Pts',(0.89302731170243,-12.5839914134569,9.85270610253088));
#58281=CARTESIAN_POINT('Ctrl Pts',(1.11957567025123,-12.5831097264016,9.83923149937973));
#58282=CARTESIAN_POINT('Ctrl Pts',(1.34601651728224,-12.5818766562194,9.82063849533055));
#58283=CARTESIAN_POINT('Ctrl Pts',(1.57219035281345,-12.5802662194557,9.79692574624548));
#58284=CARTESIAN_POINT('Ctrl Pts',(1.83383500759072,-12.5784032180608,9.76949412917265));
#58285=CARTESIAN_POINT('Ctrl Pts',(2.09512554905751,-12.5760265328939,9.7352226106913));
#58286=CARTESIAN_POINT('Ctrl Pts',(2.35582217161252,-12.5730392452114,9.69414814227475));
#58287=CARTESIAN_POINT('Ctrl Pts',(2.3568381888416,-12.5730276028061,9.69398806207434));
#58288=CARTESIAN_POINT('Ctrl Pts',(2.35785419704612,-12.5730159510797,9.69382787855833));
#58289=CARTESIAN_POINT('Ctrl Pts',(2.35887019620811,-12.5730042900304,9.69366759172347));
#58290=CARTESIAN_POINT('Ctrl Pts',(2.48820019043544,-12.571519915339,9.67326413451434));
#58291=CARTESIAN_POINT('Ctrl Pts',(2.61738376537167,-12.5698845033371,9.65118661417029));
#58292=CARTESIAN_POINT('Ctrl Pts',(2.74639207799835,-12.5680849993724,9.62744286702406));
#58293=CARTESIAN_POINT('Ctrl Pts',(2.81140297034884,-12.5671781790586,9.61547772959771));
#58294=CARTESIAN_POINT('Ctrl Pts',(2.87636935570031,-12.5662296769901,9.60308945563726));
#58295=CARTESIAN_POINT('Ctrl Pts',(2.94128757520422,-12.5652375797244,9.59027920264321));
#58296=CARTESIAN_POINT('Ctrl Pts',(2.98336724997286,-12.5645945070923,9.58197565883359));
#58297=CARTESIAN_POINT('Ctrl Pts',(3.024643377431,-12.5639455463812,9.57365373262523));
#58298=CARTESIAN_POINT('Ctrl Pts',(3.06663870624113,-12.5632662467228,9.56500710690005));
#58299=CARTESIAN_POINT('Ctrl Pts',(3.08943147260578,-12.5628975600415,9.56031419162636));
#58300=CARTESIAN_POINT('Ctrl Pts',(3.11243591374572,-12.5625198480753,9.5555247743268));
#58301=CARTESIAN_POINT('Ctrl Pts',(3.13589407750061,-12.562128525598,9.55058363765296));
#58302=CARTESIAN_POINT('Ctrl Pts',(3.45792607029556,-12.5567564786418,9.48275206710139));
#58303=CARTESIAN_POINT('Ctrl Pts',(3.77778411279328,-12.5502797008164,9.40471925064032));
#58304=CARTESIAN_POINT('Ctrl Pts',(4.09504715332939,-12.5424384023626,9.31680416471889));
#58305=CARTESIAN_POINT('Ctrl Pts',(4.30300519283459,-12.5372986260721,9.2591780104708));
#58306=CARTESIAN_POINT('Ctrl Pts',(4.50984798325849,-12.531572438382,9.19730493485485));
#58307=CARTESIAN_POINT('Ctrl Pts',(4.71545186718156,-12.5251843761894,9.13126398304479));
#58308=CARTESIAN_POINT('Ctrl Pts',(5.031472821928,-12.5153656827164,9.02975653948312));
#58309=CARTESIAN_POINT('Ctrl Pts',(5.3445683477536,-12.5039841300981,8.9184043282054));
#58310=CARTESIAN_POINT('Ctrl Pts',(5.65441445792807,-12.4907289039645,8.79751201703659));
#58311=CARTESIAN_POINT('Ctrl Pts',(5.854308371056,-12.4821774362061,8.71951963193611));
#58312=CARTESIAN_POINT('Ctrl Pts',(6.05284931410823,-12.4728458597741,8.63755576109365));
#58313=CARTESIAN_POINT('Ctrl Pts',(6.24994316851036,-12.4626470416234,8.55169392353473));
#58314=CARTESIAN_POINT('Ctrl Pts',(6.99927526292643,9.44704415986502,24.8232802776653));
#58315=CARTESIAN_POINT('Ctrl Pts',(6.99927526292643,9.41629241490398,24.801050302151));
#58316=CARTESIAN_POINT('Ctrl Pts',(6.99927526292643,8.91758329726219,24.4365954978806));
#58317=CARTESIAN_POINT('Ctrl Pts',(6.99927526292643,8.00909875236458,23.647769984431));
#58318=CARTESIAN_POINT('Ctrl Pts',(6.99927526292643,6.88884119794498,22.3080781927806));
#58319=CARTESIAN_POINT('Ctrl Pts',(6.99927526292643,5.9930919361781,20.8057475120462));
#58320=CARTESIAN_POINT('Ctrl Pts',(6.99927526292643,5.34745705503301,19.1796203432765));
#58321=CARTESIAN_POINT('Ctrl Pts',(6.99927526292643,4.96742028329228,17.4733110856848));
#58322=CARTESIAN_POINT('Ctrl Pts',(6.99927526292643,4.87762649267095,15.9617880871282));
#58323=CARTESIAN_POINT('Ctrl Pts',(6.99927526292643,4.94001610509403,15.0339554789579));
#58324=CARTESIAN_POINT('Ctrl Pts',(6.99927526292643,4.98003572958382,14.6874887993379));
#58325=CARTESIAN_POINT('Ctrl Pts',(7.01783962573763,9.16157764065615,25.2182708006853));
#58326=CARTESIAN_POINT('Ctrl Pts',(7.01783962573763,9.12945983384568,25.1950528668925));
#58327=CARTESIAN_POINT('Ctrl Pts',(7.01783962573763,8.60860591634158,24.8144101938525));
#58328=CARTESIAN_POINT('Ctrl Pts',(7.01783962573763,7.66002850735824,23.9908049285709));
#58329=CARTESIAN_POINT('Ctrl Pts',(7.01783962573763,6.48952991797069,22.5910607154748));
#58330=CARTESIAN_POINT('Ctrl Pts',(7.01783962573763,5.55415345536922,21.0221777162444));
#58331=CARTESIAN_POINT('Ctrl Pts',(7.01783962573763,4.87968438631774,19.3235982272894));
#58332=CARTESIAN_POINT('Ctrl Pts',(7.01783962573763,4.48273427219063,17.5411348960416));
#58333=CARTESIAN_POINT('Ctrl Pts',(7.01783962573763,4.38895295266063,15.9624836593832));
#58334=CARTESIAN_POINT('Ctrl Pts',(7.01783962573763,4.45409550855552,14.9934905513188));
#58335=CARTESIAN_POINT('Ctrl Pts',(7.01783962573763,4.49590504859499,14.6315514586941));
#58336=CARTESIAN_POINT('Ctrl Pts',(6.72784681146792,8.9312011144958,25.5370351335853));
#58337=CARTESIAN_POINT('Ctrl Pts',(6.72784681146792,8.89798087162717,25.5130199000031));
#58338=CARTESIAN_POINT('Ctrl Pts',(6.72784681146792,8.35925570926948,25.119313330773));
#58339=CARTESIAN_POINT('Ctrl Pts',(6.72784681146792,7.37832265037781,24.267640191082));
#58340=CARTESIAN_POINT('Ctrl Pts',(6.72784681146792,6.16727865785568,22.8194326125491));
#58341=CARTESIAN_POINT('Ctrl Pts',(6.72784681146792,5.19992234383034,21.1968407160822));
#58342=CARTESIAN_POINT('Ctrl Pts',(6.72784681146792,4.50218357554392,19.4397909242666));
#58343=CARTESIAN_POINT('Ctrl Pts',(6.72784681146792,4.09158409519261,17.5958699096704));
#58344=CARTESIAN_POINT('Ctrl Pts',(6.72784681146792,3.99458476935429,15.9630449984808));
#58345=CARTESIAN_POINT('Ctrl Pts',(6.72784681146792,4.06194899928686,14.9608346395659));
#58346=CARTESIAN_POINT('Ctrl Pts',(6.72784681146792,4.10520303280751,14.5864090361991));
#58347=CARTESIAN_POINT('Ctrl Pts',(6.25435484201992,8.85825656412263,25.6379660805211));
#58348=CARTESIAN_POINT('Ctrl Pts',(6.25435484201992,8.82468725486408,25.6136983964164));
#58349=CARTESIAN_POINT('Ctrl Pts',(6.25435484201992,8.28030348682288,25.2158553812985));
#58350=CARTESIAN_POINT('Ctrl Pts',(6.25435484201992,7.28912559798158,24.3552950580346));
#58351=CARTESIAN_POINT('Ctrl Pts',(6.25435484201992,6.06524363863058,22.8917424334598));
#58352=CARTESIAN_POINT('Ctrl Pts',(6.25435484201992,5.08776148443815,21.2521445884091));
#58353=CARTESIAN_POINT('Ctrl Pts',(6.25435484201992,4.38265478775795,19.47658123523));
#58354=CARTESIAN_POINT('Ctrl Pts',(6.25435484201992,3.96773348304226,17.6132007594115));
#58355=CARTESIAN_POINT('Ctrl Pts',(6.25435484201992,3.86971523385333,15.963222736331));
#58356=CARTESIAN_POINT('Ctrl Pts',(6.25435484201992,3.93778291659275,14.9504947371498));
#58357=CARTESIAN_POINT('Ctrl Pts',(6.25435484201992,3.9814943227866,14.5721155065288));
#58358=CARTESIAN_POINT('',(7.00000000000001,9.33250976924427,24.7867247203051));
#58359=CARTESIAN_POINT('',(6.99999999999964,4.92969295105241,14.7967973165495));
#58360=CARTESIAN_POINT('Ctrl Pts',(7.00000000000005,9.33250976255615,24.7867247293583));
#58361=CARTESIAN_POINT('Ctrl Pts',(7.00000000000005,9.20047769609296,24.6891841303334));
#58362=CARTESIAN_POINT('Ctrl Pts',(7.00000000006095,9.07102168308161,24.5890317436279));
#58363=CARTESIAN_POINT('Ctrl Pts',(6.99999999867112,8.94403923540431,24.486233382507));
#58364=CARTESIAN_POINT('Ctrl Pts',(6.99999999727843,8.81679607174416,24.3832239593358));
#58365=CARTESIAN_POINT('Ctrl Pts',(6.99999999421914,8.69203630445828,24.2775573748931));
#58366=CARTESIAN_POINT('Ctrl Pts',(6.99999999313357,8.56968906002076,24.1691580041023));
#58367=CARTESIAN_POINT('Ctrl Pts',(6.99999999205182,8.44777245597257,24.0611401796836));
#58368=CARTESIAN_POINT('Ctrl Pts',(6.99999999470457,8.32825110191426,23.9504084532141));
#58369=CARTESIAN_POINT('Ctrl Pts',(6.99999999802626,8.21109171686694,23.8368518662112));
#58370=CARTESIAN_POINT('Ctrl Pts',(6.99999999906757,8.17436385458824,23.8012534317657));
#58371=CARTESIAN_POINT('Ctrl Pts',(7.00000000000005,8.13786840392794,23.7653771393012));
#58372=CARTESIAN_POINT('Ctrl Pts',(7.00000000000005,8.10160516772495,23.7292189109433));
#58373=CARTESIAN_POINT('Ctrl Pts',(7.00000000000005,8.07267838292857,23.7003758897502));
#58374=CARTESIAN_POINT('Ctrl Pts',(6.99999999938506,8.04389549916536,23.671356721074));
#58375=CARTESIAN_POINT('Ctrl Pts',(6.99999999847366,8.01526107836191,23.6421641904065));
#58376=CARTESIAN_POINT('Ctrl Pts',(6.99999999415778,7.87966422274191,23.5039244336721));
#58377=CARTESIAN_POINT('Ctrl Pts',(6.99999998570413,7.7473991572233,23.3617938511783));
#58378=CARTESIAN_POINT('Ctrl Pts',(6.99999998494294,7.61883545625649,23.2161013823617));
#58379=CARTESIAN_POINT('Ctrl Pts',(6.99999998418015,7.49000000656178,23.0701009592567));
#58380=CARTESIAN_POINT('Ctrl Pts',(6.99999998976665,7.36488188650251,22.9205238664381));
#58381=CARTESIAN_POINT('Ctrl Pts',(6.99999999468264,7.24381793950226,22.7677399422963));
#58382=CARTESIAN_POINT('Ctrl Pts',(6.99999999757253,7.17264988363522,22.6779251368291));
#58383=CARTESIAN_POINT('Ctrl Pts',(7.00000000000005,7.10288215896253,22.5870028455032));
#58384=CARTESIAN_POINT('Ctrl Pts',(7.00000000000005,7.03457692457189,22.4950538009022));
#58385=CARTESIAN_POINT('Ctrl Pts',(7.00000000000005,6.98764067308348,22.4318705980333));
#58386=CARTESIAN_POINT('Ctrl Pts',(6.99999999889749,6.94140041000313,22.3681993760895));
#58387=CARTESIAN_POINT('Ctrl Pts',(6.99999999756676,6.89586168253803,22.3040493688111));
#58388=CARTESIAN_POINT('Ctrl Pts',(6.99999999341046,6.75362945488333,22.1036880731148));
#58389=CARTESIAN_POINT('Ctrl Pts',(6.99999998911106,6.61823772701506,21.8986585551687));
#58390=CARTESIAN_POINT('Ctrl Pts',(6.99999999137286,6.48987017006242,21.6892961098581));
#58391=CARTESIAN_POINT('Ctrl Pts',(6.99999999340019,6.37480992104594,21.5016373613082));
#58392=CARTESIAN_POINT('Ctrl Pts',(7.00000000000005,6.26539334235283,21.3104967513935));
#58393=CARTESIAN_POINT('Ctrl Pts',(7.00000000000005,6.16178267245402,21.1160965407411));
#58394=CARTESIAN_POINT('Ctrl Pts',(7.00000000000005,6.10658746605843,21.0125361664979));
#58395=CARTESIAN_POINT('Ctrl Pts',(6.99999999798935,6.0530248573596,20.9080563407882));
#58396=CARTESIAN_POINT('Ctrl Pts',(6.99999999626516,6.00114000791266,20.8027233076497));
#58397=CARTESIAN_POINT('Ctrl Pts',(6.99999999250274,5.88792037752004,20.5728726439744));
#58398=CARTESIAN_POINT('Ctrl Pts',(6.99999999167263,5.78269282412516,20.3389576788273));
#58399=CARTESIAN_POINT('Ctrl Pts',(6.99999999476594,5.68575403995867,20.1017228715802));
#58400=CARTESIAN_POINT('Ctrl Pts',(6.99999999683534,5.6209025782142,19.943014216846));
#58401=CARTESIAN_POINT('Ctrl Pts',(7.00000000000005,5.55975985482664,19.7828203356804));
#58402=CARTESIAN_POINT('Ctrl Pts',(7.00000000000005,5.50240279152306,19.6213693832778));
#58403=CARTESIAN_POINT('Ctrl Pts',(7.00000000000005,5.45009099025049,19.4741200359279));
#58404=CARTESIAN_POINT('Ctrl Pts',(6.99999999705134,5.40094158554649,19.3258230175821));
#58405=CARTESIAN_POINT('Ctrl Pts',(6.99999999409828,5.35498665730465,19.1765629015957));
#58406=CARTESIAN_POINT('Ctrl Pts',(6.99999998947404,5.2830251860527,18.9428343776582));
#58407=CARTESIAN_POINT('Ctrl Pts',(6.99999998692731,5.21889427230412,18.7067443810182));
#58408=CARTESIAN_POINT('Ctrl Pts',(6.99999999182212,5.1627249648281,18.4686326355673));
#58409=CARTESIAN_POINT('Ctrl Pts',(6.99999999469964,5.12970466676817,18.3286536833662));
#58410=CARTESIAN_POINT('Ctrl Pts',(7.00000000000005,5.09943680476764,18.1879758874761));
#58411=CARTESIAN_POINT('Ctrl Pts',(7.00000000000005,5.07195641421797,18.0466678965669));
#58412=CARTESIAN_POINT('Ctrl Pts',(7.00000000000005,5.03480694334795,17.8556401496179));
#58413=CARTESIAN_POINT('Ctrl Pts',(6.99999998960188,5.00268470340247,17.6634616339159));
#58414=CARTESIAN_POINT('Ctrl Pts',(6.99999998461861,4.97570501838642,17.4706050373956));
#58415=CARTESIAN_POINT('Ctrl Pts',(6.99999997943762,4.94765482772354,17.2700962360598));
#58416=CARTESIAN_POINT('Ctrl Pts',(6.99999998080576,4.92516373828694,17.0688548847934));
#58417=CARTESIAN_POINT('Ctrl Pts',(6.99999998755707,4.90822419654875,16.8674168812407));
#58418=CARTESIAN_POINT('Ctrl Pts',(6.99999999250474,4.89581014344996,16.7197941113412));
#58419=CARTESIAN_POINT('Ctrl Pts',(7.00000000000005,4.88637652011908,16.5720658725087));
#58420=CARTESIAN_POINT('Ctrl Pts',(7.00000000000005,4.87990258513925,16.4244427931237));
#58421=CARTESIAN_POINT('Ctrl Pts',(7.00000000000005,4.87262550786042,16.2585059154486));
#58422=CARTESIAN_POINT('Ctrl Pts',(6.99999999328029,4.86916233836076,16.0927162210766));
#58423=CARTESIAN_POINT('Ctrl Pts',(6.99999999271624,4.86945768018416,15.9269562920536));
#58424=CARTESIAN_POINT('Ctrl Pts',(6.99999999249361,4.86957425256143,15.8615303095054));
#58425=CARTESIAN_POINT('Ctrl Pts',(6.99999999280638,4.87027693192223,15.7961088794921));
#58426=CARTESIAN_POINT('Ctrl Pts',(6.99999999341992,4.87156453058809,15.7306845305713));
#58427=CARTESIAN_POINT('Ctrl Pts',(6.99999999496892,4.87481533850375,15.5655072925178));
#58428=CARTESIAN_POINT('Ctrl Pts',(6.99999999795329,4.88179088200453,15.4003113655275));
#58429=CARTESIAN_POINT('Ctrl Pts',(6.99999999909603,4.89250690007613,15.2350111867318));
#58430=CARTESIAN_POINT('Ctrl Pts',(7.00000000010515,4.9019698574621,15.0890401238441));
#58431=CARTESIAN_POINT('Ctrl Pts',(6.99999999999946,4.91435036442321,14.9429875256047));
#58432=CARTESIAN_POINT('Ctrl Pts',(6.99999999999946,4.92969295105302,14.7967973165496));
#58433=CARTESIAN_POINT('',(6.2715946948284,8.76071067545968,25.5608579362149));
#58434=CARTESIAN_POINT('Origin',(5.999999877386,9.33250977407517,24.7867246592848));
#58435=CARTESIAN_POINT('',(6.263859499331,3.90573865723227,15.8144314043406));
#58436=CARTESIAN_POINT('Ctrl Pts',(6.27159470456883,8.76071047658687,25.5608577604478));
#58437=CARTESIAN_POINT('Ctrl Pts',(6.27193966898912,8.57412216343359,25.4228903957121));
#58438=CARTESIAN_POINT('Ctrl Pts',(6.27225782564642,8.39339832660335,25.280910240924));
#58439=CARTESIAN_POINT('Ctrl Pts',(6.27254917025225,8.21861683396742,25.1354918255172));
#58440=CARTESIAN_POINT('Ctrl Pts',(6.27284515814358,8.04104977277711,24.9877558136701));
#58441=CARTESIAN_POINT('Ctrl Pts',(6.273113472547,7.86961592067851,24.8364710622416));
#58442=CARTESIAN_POINT('Ctrl Pts',(6.27335410990005,7.70435956582304,24.6822006939131));
#58443=CARTESIAN_POINT('Ctrl Pts',(6.27354178806678,7.57547263564886,24.5618819672409));
#58444=CARTESIAN_POINT('Ctrl Pts',(6.27371263093874,7.4503425644811,24.4397463543931));
#58445=CARTESIAN_POINT('Ctrl Pts',(6.27386663718526,7.32897538003059,24.3160449569086));
#58446=CARTESIAN_POINT('Ctrl Pts',(6.27406868749697,7.16974627079252,24.1537534493471));
#58447=CARTESIAN_POINT('Ctrl Pts',(6.27424175784606,7.01699420978249,23.9887688320545));
#58448=CARTESIAN_POINT('Ctrl Pts',(6.27438584597958,6.87062082868007,23.8216790784536));
#58449=CARTESIAN_POINT('Ctrl Pts',(6.27447251908614,6.78257308076604,23.7211698438286));
#58450=CARTESIAN_POINT('Ctrl Pts',(6.27454870538725,6.69683289921858,23.6198979734037));
#58451=CARTESIAN_POINT('Ctrl Pts',(6.27461440453154,6.61337480174416,23.5179833665145));
#58452=CARTESIAN_POINT('Ctrl Pts',(6.27472591356408,6.47172407237543,23.3450070006969));
#58453=CARTESIAN_POINT('Ctrl Pts',(6.27480721202419,6.33664860500451,23.170181629431));
#58454=CARTESIAN_POINT('Ctrl Pts',(6.27485829885037,6.20800497223007,22.9940551814749));
#58455=CARTESIAN_POINT('Ctrl Pts',(6.27487121255017,6.17548650555785,22.9495340349212));
#58456=CARTESIAN_POINT('Ctrl Pts',(6.2748821958076,6.14337890295727,22.9049295182343));
#58457=CARTESIAN_POINT('Ctrl Pts',(6.27489124861356,6.11167962107519,22.8602500105962));
#58458=CARTESIAN_POINT('Ctrl Pts',(6.27492812667764,5.9825474874977,22.6782408354367));
#58459=CARTESIAN_POINT('Ctrl Pts',(6.27493296938054,5.86019259786137,22.4949912131483));
#58460=CARTESIAN_POINT('Ctrl Pts',(6.27490577665586,5.74438889409281,22.311044212034));
#58461=CARTESIAN_POINT('Ctrl Pts',(6.27488257757821,5.64559264810312,22.154112502773));
#58462=CARTESIAN_POINT('Ctrl Pts',(6.27483606184547,5.55156428911671,21.9966722845104));
#58463=CARTESIAN_POINT('Ctrl Pts',(6.2747662299236,5.46215434352605,21.8390322558468));
#58464=CARTESIAN_POINT('Ctrl Pts',(6.27472435194041,5.40853548128942,21.7444960280921));
#58465=CARTESIAN_POINT('Ctrl Pts',(6.27467408868735,5.35657741163384,21.6498874448625));
#58466=CARTESIAN_POINT('Ctrl Pts',(6.27461544167778,5.30624656452333,21.5552687339916));
#58467=CARTESIAN_POINT('Ctrl Pts',(6.27458611817299,5.28108114096807,21.5079593785561));
#58468=CARTESIAN_POINT('Ctrl Pts',(6.2745546960971,5.25632253120737,21.4606474869213));
#58469=CARTESIAN_POINT('Ctrl Pts',(6.27452117889509,5.23196642427779,21.4133404892521));
#58470=CARTESIAN_POINT('Ctrl Pts',(6.27450442029408,5.21978837081299,21.3896869904175));
#58471=CARTESIAN_POINT('Ctrl Pts',(6.27448713773378,5.20771094360307,21.3660347147777));
#58472=CARTESIAN_POINT('Ctrl Pts',(6.27446933121476,5.19573360226955,21.3423845802045));
#58473=CARTESIAN_POINT('Ctrl Pts',(6.27445391938858,5.18536702234589,21.3219150115889));
#58474=CARTESIAN_POINT('Ctrl Pts',(6.2744387297381,5.17546073754221,21.302217342206));
#58475=CARTESIAN_POINT('Ctrl Pts',(6.27442216601483,5.16501365433626,21.281292176439));
#58476=CARTESIAN_POINT('Ctrl Pts',(6.27441959233996,5.16339038430915,21.2780408196983));
#58477=CARTESIAN_POINT('Ctrl Pts',(6.27441698549086,5.16175414864423,21.2747597818786));
#58478=CARTESIAN_POINT('Ctrl Pts',(6.27441433947949,5.16010129477184,21.2714415111871));
#58479=CARTESIAN_POINT('Ctrl Pts',(6.27440279750611,5.15289150132369,21.2569671243763));
#58480=CARTESIAN_POINT('Ctrl Pts',(6.27439106570806,5.14570665026556,21.2424690495645));
#58481=CARTESIAN_POINT('Ctrl Pts',(6.27437914408635,5.13854692001712,21.2279473420534));
#58482=CARTESIAN_POINT('Ctrl Pts',(6.2742001112939,5.03102576804095,21.0098677963058));
#58483=CARTESIAN_POINT('Ctrl Pts',(6.27397826838863,4.92916789617758,20.7864547547487));
#58484=CARTESIAN_POINT('Ctrl Pts',(6.27371361964825,4.83351597227066,20.5579710708369));
#58485=CARTESIAN_POINT('Ctrl Pts',(6.27345239286638,4.73910084591757,20.3324417243792));
#58486=CARTESIAN_POINT('Ctrl Pts',(6.27314946005732,4.65073221455464,20.1019719667757));
#58487=CARTESIAN_POINT('Ctrl Pts',(6.27280482717338,4.56895654665535,19.8668588618551));
#58488=CARTESIAN_POINT('Ctrl Pts',(6.27260798328253,4.52224875585436,19.7325693598394));
#58489=CARTESIAN_POINT('Ctrl Pts',(6.27239753540531,4.47769227178865,19.5967658531892));
#58490=CARTESIAN_POINT('Ctrl Pts',(6.27217348494914,4.4353926019923,19.4595104126762));
#58491=CARTESIAN_POINT('Ctrl Pts',(6.27177013693201,4.35924239801633,19.2124155809151));
#58492=CARTESIAN_POINT('Ctrl Pts',(6.27132270389783,4.29040507220786,18.9606117357067));
#58493=CARTESIAN_POINT('Ctrl Pts',(6.27083119604893,4.22947047055946,18.7045320508306));
#58494=CARTESIAN_POINT('Ctrl Pts',(6.27036732538413,4.17196218409212,18.4628515691678));
#58495=CARTESIAN_POINT('Ctrl Pts',(6.26986419841394,4.12149304373649,18.217362945302));
#58496=CARTESIAN_POINT('Ctrl Pts',(6.26932182509284,4.07857892143672,17.9684782794355));
#58497=CARTESIAN_POINT('Ctrl Pts',(6.26905884935212,4.05777153165553,17.847803779394));
#58498=CARTESIAN_POINT('Ctrl Pts',(6.2687866472112,4.03874054889739,17.7263316145486));
#58499=CARTESIAN_POINT('Ctrl Pts',(6.26850522002609,4.02154646450729,17.6041128541433));
#58500=CARTESIAN_POINT('Ctrl Pts',(6.26791729738518,3.98562672385184,17.348788634639));
#58501=CARTESIAN_POINT('Ctrl Pts',(6.26728911425905,3.95772350439215,17.0902028081567));
#58502=CARTESIAN_POINT('Ctrl Pts',(6.26662068529587,3.93824701803358,16.8288403534343));
#58503=CARTESIAN_POINT('Ctrl Pts',(6.26595956850197,3.91898359151107,16.5703370305252));
#58504=CARTESIAN_POINT('Ctrl Pts',(6.26525908155454,3.90796355341187,16.3091174478807));
#58505=CARTESIAN_POINT('Ctrl Pts',(6.26451924198579,3.90559007207061,16.0457015126995));
#58506=CARTESIAN_POINT('Ctrl Pts',(6.2643032360479,3.90489710283129,15.9687937498052));
#58507=CARTESIAN_POINT('Ctrl Pts',(6.26408387561693,3.90494122833423,15.8916990992977));
#58508=CARTESIAN_POINT('Ctrl Pts',(6.26386116118917,3.90573258256842,15.8144313373355));
#58509=CARTESIAN_POINT('Ctrl Pts',(6.99999999999946,4.92969295105265,14.7967973165499));
#58510=CARTESIAN_POINT('Ctrl Pts',(7.00000003182991,4.89790687011507,14.8200962579317));
#58511=CARTESIAN_POINT('Ctrl Pts',(6.99872202620472,4.86684766352378,14.843151536839));
#58512=CARTESIAN_POINT('Ctrl Pts',(6.9963283798615,4.83663262564484,14.8659154105751));
#58513=CARTESIAN_POINT('Ctrl Pts',(6.99385186988673,4.80537159875714,14.8894673277293));
#58514=CARTESIAN_POINT('Ctrl Pts',(6.99018212459228,4.77501418352712,14.9127071669234));
#58515=CARTESIAN_POINT('Ctrl Pts',(6.98550026819671,4.74563468961346,14.9355742924579));
#58516=CARTESIAN_POINT('Ctrl Pts',(6.98072065912985,4.71564178004406,14.9589188616422));
#58517=CARTESIAN_POINT('Ctrl Pts',(6.97488710906418,4.68666762354792,14.98187480912));
#58518=CARTESIAN_POINT('Ctrl Pts',(6.96817910818256,4.65873797521076,15.0043722661871));
#58519=CARTESIAN_POINT('Ctrl Pts',(6.9612398354513,4.62984539595801,15.0276453684277));
#58520=CARTESIAN_POINT('Ctrl Pts',(6.95336553314029,4.6020700174534,15.0504276449154));
#58521=CARTESIAN_POINT('Ctrl Pts',(6.94472806264123,4.57539155224688,15.0726388605227));
#58522=CARTESIAN_POINT('Ctrl Pts',(6.94166914281976,4.56594349844046,15.0805048587553));
#58523=CARTESIAN_POINT('Ctrl Pts',(6.93851421614368,4.55663262766185,15.0882992220146));
#58524=CARTESIAN_POINT('Ctrl Pts',(6.93526991044448,4.54745686940672,15.096018363856));
#58525=CARTESIAN_POINT('Ctrl Pts',(6.92517489872626,4.51890549487626,15.1200373172373));
#58526=CARTESIAN_POINT('Ctrl Pts',(6.9142321383047,4.49170592042528,15.1433602032958));
#58527=CARTESIAN_POINT('Ctrl Pts',(6.90266739083218,4.46584896584675,15.1659445078881));
#58528=CARTESIAN_POINT('Ctrl Pts',(6.89228282415092,4.44263070970818,15.1862240874939));
#58529=CARTESIAN_POINT('Ctrl Pts',(6.88139666907031,4.42049387796962,15.2059080622683));
#58530=CARTESIAN_POINT('Ctrl Pts',(6.87015182633685,4.39940255498227,15.2249667510503));
#58531=CARTESIAN_POINT('Ctrl Pts',(6.85826800906539,4.37711274316933,15.2451084266866));
#58532=CARTESIAN_POINT('Ctrl Pts',(6.84598542356712,4.35599382686861,15.2645550463613));
#58533=CARTESIAN_POINT('Ctrl Pts',(6.83346225158623,4.33599910281022,15.2832873166577));
#58534=CARTESIAN_POINT('Ctrl Pts',(6.82720066559579,4.32600174078102,15.2926534518059));
#58535=CARTESIAN_POINT('Ctrl Pts',(6.82087870508477,4.31628525721843,15.3018411349062));
#58536=CARTESIAN_POINT('Ctrl Pts',(6.81451474301598,4.30684284344094,15.3108487116038));
#58537=CARTESIAN_POINT('Ctrl Pts',(6.81133276198159,4.30212163655219,15.3153524999526));
#58538=CARTESIAN_POINT('Ctrl Pts',(6.80814027492826,4.29746895059205,15.3198112619028));
#58539=CARTESIAN_POINT('Ctrl Pts',(6.80493947884344,4.29288386412139,15.3242248417572));
#58540=CARTESIAN_POINT('Ctrl Pts',(6.80333908080103,4.29059132088605,15.3264316316844));
#58541=CARTESIAN_POINT('Ctrl Pts',(6.80173660508477,4.28831567774204,15.3286271261022));
#58542=CARTESIAN_POINT('Ctrl Pts',(6.80013232216023,4.28605681842174,15.3308113069044));
#58543=CARTESIAN_POINT('Ctrl Pts',(6.79874993359117,4.28411039035989,15.3326933855126));
#58544=CARTESIAN_POINT('Ctrl Pts',(6.79775798456452,4.28272134681384,15.3340389472113));
#58545=CARTESIAN_POINT('Ctrl Pts',(6.79614408876686,4.28048077370916,15.3362131510563));
#58546=CARTESIAN_POINT('Ctrl Pts',(6.79588503398598,4.28012112770504,15.3365621437865));
#58547=CARTESIAN_POINT('Ctrl Pts',(6.79560987565501,4.27973960727994,15.3369325016948));
#58548=CARTESIAN_POINT('Ctrl Pts',(6.79531431958812,4.27933047508902,15.337329891204));
#58549=CARTESIAN_POINT('Ctrl Pts',(6.76951420699996,4.24361590932029,15.3720193976253));
#58550=CARTESIAN_POINT('Ctrl Pts',(6.74173255827647,4.21000266490947,15.4059751937068));
#58551=CARTESIAN_POINT('Ctrl Pts',(6.71227734444122,4.17864917320428,15.439110835369));
#58552=CARTESIAN_POINT('Ctrl Pts',(6.68190104901643,4.14631523966156,15.4732826477296));
#58553=CARTESIAN_POINT('Ctrl Pts',(6.64974534687681,4.11638416653758,15.5065819374885));
#58554=CARTESIAN_POINT('Ctrl Pts',(6.6161493421093,4.08897088661842,15.5389140150329));
#58555=CARTESIAN_POINT('Ctrl Pts',(6.58093661722554,4.06023841409273,15.572801989492));
#58556=CARTESIAN_POINT('Ctrl Pts',(6.54414181559471,4.03427162417726,15.6056271410108));
#58557=CARTESIAN_POINT('Ctrl Pts',(6.50615167047959,4.01114470028624,15.6372849612645));
#58558=CARTESIAN_POINT('Ctrl Pts',(6.4749471911299,3.99214862599401,15.6632881732915));
#58559=CARTESIAN_POINT('Ctrl Pts',(6.44293613655435,3.975067367133,15.6885038655809));
#58560=CARTESIAN_POINT('Ctrl Pts',(6.41033062344876,3.95991630293878,15.7128780676492));
#58561=CARTESIAN_POINT('Ctrl Pts',(6.36985327840053,3.94110737172364,15.7431368457949));
#58562=CARTESIAN_POINT('Ctrl Pts',(6.32845982679951,3.92527454314398,15.7720983393468));
#58563=CARTESIAN_POINT('Ctrl Pts',(6.28655299478072,3.91240124871222,15.7996692510339));
#58564=CARTESIAN_POINT('Ctrl Pts',(6.27900493180689,3.91008257100812,15.8046351949537));
#58565=CARTESIAN_POINT('Ctrl Pts',(6.27144020631059,3.90785977293139,15.8095560578491));
#58566=CARTESIAN_POINT('Ctrl Pts',(6.26386116118917,3.90573258256842,15.8144313373355));
#58567=CARTESIAN_POINT('Ctrl Pts',(7.10569404143661,5.09054165125083,15.2151876877299));
#58568=CARTESIAN_POINT('Ctrl Pts',(7.10698751687283,5.00269310760996,15.2441266563576));
#58569=CARTESIAN_POINT('Ctrl Pts',(7.0902945199642,4.80945364231557,15.312718885045));
#58570=CARTESIAN_POINT('Ctrl Pts',(6.99969996992157,4.52705209321443,15.4294190158596));
#58571=CARTESIAN_POINT('Ctrl Pts',(6.83798590956392,4.26863790102804,15.5561021331105));
#58572=CARTESIAN_POINT('Ctrl Pts',(6.62407657918662,4.06622759758902,15.6779599862762));
#58573=CARTESIAN_POINT('Ctrl Pts',(6.41886258694164,3.95388203420082,15.7685510741009));
#58574=CARTESIAN_POINT('Ctrl Pts',(6.29029260882867,3.91233292862259,15.8162139975417));
#58575=CARTESIAN_POINT('Ctrl Pts',(6.24978854300632,3.9018220331908,15.8304216839861));
#58576=CARTESIAN_POINT('Ctrl Pts',(6.81662658173112,4.90577014638609,14.6682465297021));
#58577=CARTESIAN_POINT('Ctrl Pts',(6.81778595104908,4.82838688483558,14.6937210486444));
#58578=CARTESIAN_POINT('Ctrl Pts',(6.80279186069882,4.65778890045996,14.754496390137));
#58579=CARTESIAN_POINT('Ctrl Pts',(6.72115173917901,4.4083902191048,14.8587571478518));
#58580=CARTESIAN_POINT('Ctrl Pts',(6.57567845311055,4.18091900980098,14.9723280494875));
#58581=CARTESIAN_POINT('Ctrl Pts',(6.384034670463,4.00376978964618,15.081523231443));
#58582=CARTESIAN_POINT('Ctrl Pts',(6.20121810832221,3.9062350109221,15.1623974452969));
#58583=CARTESIAN_POINT('Ctrl Pts',(6.08727994870383,3.87041481062267,15.204739989342));
#58584=CARTESIAN_POINT('Ctrl Pts',(6.05144712941405,3.86137576219619,15.2173393578419));
#58585=CARTESIAN_POINT('Ctrl Pts',(7.05823304509093,4.72145803038867,14.0984567957104));
#58586=CARTESIAN_POINT('Ctrl Pts',(7.05976380412154,4.62141948135273,14.1314134593268));
#58587=CARTESIAN_POINT('Ctrl Pts',(7.04010452168148,4.40252217185232,14.2090883142289));
#58588=CARTESIAN_POINT('Ctrl Pts',(6.93421353969746,4.08329669950976,14.3408115984512));
#58589=CARTESIAN_POINT('Ctrl Pts',(6.7444197293285,3.78963037230628,14.4845606457827));
#58590=CARTESIAN_POINT('Ctrl Pts',(6.4910049093302,3.55726100403775,14.6244807199787));
#58591=CARTESIAN_POINT('Ctrl Pts',(6.24476176461835,3.4265307786445,14.7303629781109));
#58592=CARTESIAN_POINT('Ctrl Pts',(6.08867719634714,3.37773039761847,14.7870387478717));
#58593=CARTESIAN_POINT('Ctrl Pts',(6.0393188304862,3.36535861577285,14.8040347283816));
#58594=CARTESIAN_POINT('Ctrl Pts',(7.66731039910081,4.66246517745525,13.8917937410857));
#58595=CARTESIAN_POINT('Ctrl Pts',(7.66946689865306,4.52196894416207,13.9381201648513));
#58596=CARTESIAN_POINT('Ctrl Pts',(7.64193305760113,4.21648837384924,14.0459844860487));
#58597=CARTESIAN_POINT('Ctrl Pts',(7.49498492088685,3.77181855920877,14.2265034331141));
#58598=CARTESIAN_POINT('Ctrl Pts',(7.23027996478551,3.35957593531508,14.423315567559));
#58599=CARTESIAN_POINT('Ctrl Pts',(6.87282901199206,3.02884202226372,14.6165723783504));
#58600=CARTESIAN_POINT('Ctrl Pts',(6.52022670404055,2.83935539051515,14.7652770063116));
#58601=CARTESIAN_POINT('Ctrl Pts',(6.29371870310657,2.76764241383735,14.8462471717371));
#58602=CARTESIAN_POINT('Ctrl Pts',(6.22178457189615,2.74938677633292,14.8706715897612));
#58603=CARTESIAN_POINT('',(6.24994594247521,2.765465712864,14.8593875553346));
#58604=CARTESIAN_POINT('Ctrl Pts',(6.26385699586341,3.90574781113883,15.8144315048343));
#58605=CARTESIAN_POINT('Ctrl Pts',(6.25434798380003,3.90347005541746,15.7850252855376));
#58606=CARTESIAN_POINT('Ctrl Pts',(6.24501496153337,3.89975208452744,15.7549930856709));
#58607=CARTESIAN_POINT('Ctrl Pts',(6.23596108667827,3.89444439028301,15.7245073673137));
#58608=CARTESIAN_POINT('Ctrl Pts',(6.22713383888874,3.88926955265422,15.6947847353702));
#58609=CARTESIAN_POINT('Ctrl Pts',(6.21857222852935,3.88258290074168,15.6646313129789));
#58610=CARTESIAN_POINT('Ctrl Pts',(6.21037775698272,3.87427382466893,15.6342471001828));
#58611=CARTESIAN_POINT('Ctrl Pts',(6.20230962221974,3.8660928522744,15.6043313304947));
#58612=CARTESIAN_POINT('Ctrl Pts',(6.19459771432488,3.85633847793405,15.5741922828855));
#58613=CARTESIAN_POINT('Ctrl Pts',(6.18734021170931,3.84494221012623,15.5440547858302));
#58614=CARTESIAN_POINT('Ctrl Pts',(6.18021026865726,3.83374624578704,15.5144469924724));
#58615=CARTESIAN_POINT('Ctrl Pts',(6.17351923089785,3.82096516393263,15.4848413319623));
#58616=CARTESIAN_POINT('Ctrl Pts',(6.16735661573876,3.80657784168717,15.455475932425));
#58617=CARTESIAN_POINT('Ctrl Pts',(6.1665592055774,3.80471619745706,15.4516762033523));
#58618=CARTESIAN_POINT('Ctrl Pts',(6.16577063373331,3.80282772589229,15.4478805235924));
#58619=CARTESIAN_POINT('Ctrl Pts',(6.16499108510522,3.80091244122259,15.4440894309064));
#58620=CARTESIAN_POINT('Ctrl Pts',(6.15905868185249,3.78633703104931,15.415239029827));
#58621=CARTESIAN_POINT('Ctrl Pts',(6.15364986165422,3.77020476525735,15.3866536317792));
#58622=CARTESIAN_POINT('Ctrl Pts',(6.14883921111318,3.75254960135707,15.3585762389554));
#58623=CARTESIAN_POINT('Ctrl Pts',(6.14409019033999,3.7351206196838,15.3308585486681));
#58624=CARTESIAN_POINT('Ctrl Pts',(6.1399243836778,3.716207531236,15.3036367366627));
#58625=CARTESIAN_POINT('Ctrl Pts',(6.13640028093367,3.69589197713741,15.2771455138267));
#58626=CARTESIAN_POINT('Ctrl Pts',(6.13289687262579,3.67569572118926,15.2508098542537));
#58627=CARTESIAN_POINT('Ctrl Pts',(6.1300278736233,3.65411363410035,15.2251970341261));
#58628=CARTESIAN_POINT('Ctrl Pts',(6.12783385014554,3.63127298396052,15.2005265382343));
#58629=CARTESIAN_POINT('Ctrl Pts',(6.1256472714576,3.60850983702044,15.1759397545994));
#58630=CARTESIAN_POINT('Ctrl Pts',(6.12413123414268,3.58449708246778,15.1522896565134));
#58631=CARTESIAN_POINT('Ctrl Pts',(6.1233063543654,3.55940279460655,15.1297707718731));
#58632=CARTESIAN_POINT('Ctrl Pts',(6.12248221725878,3.53433110008748,15.1072721618415));
#58633=CARTESIAN_POINT('Ctrl Pts',(6.12234803831525,3.50818043438343,15.0859033522775));
#58634=CARTESIAN_POINT('Ctrl Pts',(6.12290344669521,3.48115267077958,15.0658252908192));
#58635=CARTESIAN_POINT('Ctrl Pts',(6.12346156137084,3.45399321107174,15.0456493965359));
#58636=CARTESIAN_POINT('Ctrl Pts',(6.12471595661025,3.42594883438446,15.0267773356849));
#58637=CARTESIAN_POINT('Ctrl Pts',(6.12664506630351,3.39724869516408,15.0093306421183));
#58638=CARTESIAN_POINT('Ctrl Pts',(6.12858163947937,3.36843751871722,14.99181644949));
#58639=CARTESIAN_POINT('Ctrl Pts',(6.13119800640248,3.33896633964887,14.9757389134287));
#58640=CARTESIAN_POINT('Ctrl Pts',(6.1344525305991,3.3090793273335,14.9611735632068));
#58641=CARTESIAN_POINT('Ctrl Pts',(6.13774444965242,3.27884890981502,14.9464408554384));
#58642=CARTESIAN_POINT('Ctrl Pts',(6.14168905204685,3.24819391461928,14.9332553333186));
#58643=CARTESIAN_POINT('Ctrl Pts',(6.14622583015071,3.21736659817575,14.9216444301484));
#58644=CARTESIAN_POINT('Ctrl Pts',(6.14953012183543,3.19491400229062,14.9131878096306));
#58645=CARTESIAN_POINT('Ctrl Pts',(6.1531481575373,3.17237001510414,14.9055653725594));
#58646=CARTESIAN_POINT('Ctrl Pts',(6.15705202271518,3.14982812311891,14.8987714044217));
#58647=CARTESIAN_POINT('Ctrl Pts',(6.1625076467821,3.11832598797211,14.8892768818413));
#58648=CARTESIAN_POINT('Ctrl Pts',(6.1685214499985,3.08682925243436,14.8814020376996));
#58649=CARTESIAN_POINT('Ctrl Pts',(6.17500783915478,3.05557312923402,14.8750910675516));
#58650=CARTESIAN_POINT('Ctrl Pts',(6.18164262016742,3.02360194654021,14.8686357186816));
#58651=CARTESIAN_POINT('Ctrl Pts',(6.18877150533514,2.99188314996284,14.863816109299));
#58652=CARTESIAN_POINT('Ctrl Pts',(6.19629722070769,2.96063494824442,14.8605298222474));
#58653=CARTESIAN_POINT('Ctrl Pts',(6.20393441429794,2.92892386776148,14.8571948555148));
#58654=CARTESIAN_POINT('Ctrl Pts',(6.21197992740394,2.89769780882519,14.85543825752));
#58655=CARTESIAN_POINT('Ctrl Pts',(6.22033178841968,2.86714287327628,14.8551190429553));
#58656=CARTESIAN_POINT('Ctrl Pts',(6.22888396322111,2.83585509808839,14.8547921722434));
#58657=CARTESIAN_POINT('Ctrl Pts',(6.23775702918233,2.80527124043204,14.8559716889506));
#58658=CARTESIAN_POINT('Ctrl Pts',(6.24684646258028,2.7755427257783,14.8584823292218));
#58659=CARTESIAN_POINT('Ctrl Pts',(6.24787684252207,2.77217269556219,14.8587669358923));
#58660=CARTESIAN_POINT('Ctrl Pts',(6.2489100109869,2.76881360546945,14.859068630846));
#58661=CARTESIAN_POINT('Ctrl Pts',(6.24994582233798,2.76546563683757,14.8593871468619));
#58662=CARTESIAN_POINT('',(6.99999997823011,3.16613311195312,14.5427407175274));
#58663=CARTESIAN_POINT('Ctrl Pts',(6.99999993220815,3.16613252794448,14.5427396600064));
#58664=CARTESIAN_POINT('Ctrl Pts',(6.96231762727278,3.13329554641419,14.5625135410054));
#58665=CARTESIAN_POINT('Ctrl Pts',(6.92360816603438,3.10217170226233,14.5820110124235));
#58666=CARTESIAN_POINT('Ctrl Pts',(6.88387823383206,3.07270488837879,14.6012599053988));
#58667=CARTESIAN_POINT('Ctrl Pts',(6.87356165203147,3.065053307342,14.6062582219814));
#58668=CARTESIAN_POINT('Ctrl Pts',(6.86317604426154,3.05751362050396,14.6112397769873));
#58669=CARTESIAN_POINT('Ctrl Pts',(6.8527210844064,3.05008520711899,14.6162050497553));
#58670=CARTESIAN_POINT('Ctrl Pts',(6.82600907014904,3.0311059009334,14.6288911278282));
#58671=CARTESIAN_POINT('Ctrl Pts',(6.79884483386461,3.0128524446524,14.641470956376));
#58672=CARTESIAN_POINT('Ctrl Pts',(6.77122670154749,2.99531605711247,14.6539509876441));
#58673=CARTESIAN_POINT('Ctrl Pts',(6.70346621716213,2.95229091332536,14.6845704717628));
#58674=CARTESIAN_POINT('Ctrl Pts',(6.63297634616849,2.91356612828382,14.7145915227367));
#58675=CARTESIAN_POINT('Ctrl Pts',(6.56020276160944,2.87939117496359,14.7438671099234));
#58676=CARTESIAN_POINT('Ctrl Pts',(6.54699691805475,2.87318962408809,14.7491795983311));
#58677=CARTESIAN_POINT('Ctrl Pts',(6.53371574536084,2.8671379488153,14.7544675514922));
#58678=CARTESIAN_POINT('Ctrl Pts',(6.52036174280708,2.86123771480371,14.7597301048116));
#58679=CARTESIAN_POINT('Ctrl Pts',(6.4904965666444,2.84804230560353,14.7714993913094));
#58680=CARTESIAN_POINT('Ctrl Pts',(6.46026959312842,2.83560758267573,14.7831403452059));
#58681=CARTESIAN_POINT('Ctrl Pts',(6.42966397675873,2.82393755775448,14.7946591670874));
#58682=CARTESIAN_POINT('Ctrl Pts',(6.38476129492752,2.80681601347085,14.8115588755516));
#58683=CARTESIAN_POINT('Ctrl Pts',(6.33904417176279,2.79133823120731,14.8281961702507));
#58684=CARTESIAN_POINT('Ctrl Pts',(6.2924722492654,2.77753576511219,14.8445798018293));
#58685=CARTESIAN_POINT('Ctrl Pts',(6.27837566303401,2.77335797636992,14.8495388686436));
#58686=CARTESIAN_POINT('Ctrl Pts',(6.26420064751584,2.76933401082123,14.8544746304912));
#58687=CARTESIAN_POINT('Ctrl Pts',(6.24994582233798,2.76546563683757,14.8593871468619));
#58688=CARTESIAN_POINT('Ctrl Pts',(7.,4.9296929510512,14.7967973165494));
#58689=CARTESIAN_POINT('Ctrl Pts',(7.,4.79879097364903,14.7447999429358));
#58690=CARTESIAN_POINT('Ctrl Pts',(7.,4.67469316982841,14.7000467303213));
#58691=CARTESIAN_POINT('Ctrl Pts',(7.,4.55739953958936,14.6625376787058));
#58692=CARTESIAN_POINT('Ctrl Pts',(7.,4.51830166284301,14.6500346615006));
#58693=CARTESIAN_POINT('Ctrl Pts',(7.,4.4820605631409,14.6389453969358));
#58694=CARTESIAN_POINT('Ctrl Pts',(7.,4.44237396721083,14.6274433474232));
#58695=CARTESIAN_POINT('Ctrl Pts',(7.,4.28362758349054,14.5814351493728));
#58696=CARTESIAN_POINT('Ctrl Pts',(7.,4.12819843211269,14.5472955039941));
#58697=CARTESIAN_POINT('Ctrl Pts',(7.,3.9812641135579,14.5257824769341));
#58698=CARTESIAN_POINT('Ctrl Pts',(7.,3.68739547644833,14.4827564228141));
#58699=CARTESIAN_POINT('Ctrl Pts',(7.,3.41568526058562,14.488409179345));
#58700=CARTESIAN_POINT('Ctrl Pts',(7.,3.16613346596978,14.5427407465266));
#58701=CARTESIAN_POINT('Ctrl Pts',(6.38289431678474,3.93904937645538,15.7741367696646));
#58702=CARTESIAN_POINT('Ctrl Pts',(6.33037402857394,3.92420127911889,15.7930335494319));
#58703=CARTESIAN_POINT('Ctrl Pts',(5.6967036132714,3.74727551077352,16.0176262814828));
#58704=CARTESIAN_POINT('Ctrl Pts',(4.3653537707354,3.43062433292629,16.4060367717622));
#58705=CARTESIAN_POINT('Ctrl Pts',(2.27852928213159,3.11272070634599,16.7768273765144));
#58706=CARTESIAN_POINT('Ctrl Pts',(0.00160600171922482,2.99217538455127,
16.9128348891133));
#58707=CARTESIAN_POINT('Ctrl Pts',(-2.27556282787673,3.11240056823132,16.777192259624));
#58708=CARTESIAN_POINT('Ctrl Pts',(-4.36295887685328,3.43014050386403,16.4066150670817));
#58709=CARTESIAN_POINT('Ctrl Pts',(-5.6953528158905,3.74692061286735,16.0180709627932));
#58710=CARTESIAN_POINT('Ctrl Pts',(-6.32980048790067,3.9240391095482,15.7932399281334));
#58711=CARTESIAN_POINT('Ctrl Pts',(-6.3828984100613,3.93905052008556,15.7741353000131));
#58712=CARTESIAN_POINT('Ctrl Pts',(6.18023342351759,3.89116773501399,15.1627904562897));
#58713=CARTESIAN_POINT('Ctrl Pts',(6.12935373465988,3.87698876809142,15.1810909844233));
#58714=CARTESIAN_POINT('Ctrl Pts',(5.5154849218392,3.70803107728603,15.3985987917746));
#58715=CARTESIAN_POINT('Ctrl Pts',(4.22593147396741,3.40552953667279,15.7747860843702));
#58716=CARTESIAN_POINT('Ctrl Pts',(2.2054008109767,3.10176244037637,16.1338745651197));
#58717=CARTESIAN_POINT('Ctrl Pts',(0.00155433447093668,2.98658018383598,
16.2655671789925));
#58718=CARTESIAN_POINT('Ctrl Pts',(-2.20252913753767,3.10145653633292,16.1342278953521));
#58719=CARTESIAN_POINT('Ctrl Pts',(-4.22361213522192,3.40506724930268,15.7753461730261));
#58720=CARTESIAN_POINT('Ctrl Pts',(-5.51417640650268,3.70769210772978,15.3990294647388));
#58721=CARTESIAN_POINT('Ctrl Pts',(-6.12879810980744,3.87683390721015,15.1812908509248));
#58722=CARTESIAN_POINT('Ctrl Pts',(-6.18023738901782,3.89116882781119,15.1627890325264));
#58723=CARTESIAN_POINT('Ctrl Pts',(6.17613448039233,3.39302982546975,14.7530757616085));
#58724=CARTESIAN_POINT('Ctrl Pts',(6.12540401856028,3.379030795255,14.77115610782));
#58725=CARTESIAN_POINT('Ctrl Pts',(5.51330412368829,3.2122020990137,14.9860629206928));
#58726=CARTESIAN_POINT('Ctrl Pts',(4.22664027251003,2.91314014013688,15.3581450830883));
#58727=CARTESIAN_POINT('Ctrl Pts',(2.20729613110763,2.61210322269024,15.7140461237668));
#58728=CARTESIAN_POINT('Ctrl Pts',(0.00155619864217923,2.49773465424207,
15.8447871362558));
#58729=CARTESIAN_POINT('Ctrl Pts',(-2.20442381705102,2.61179967411732,15.7143967100113));
#58730=CARTESIAN_POINT('Ctrl Pts',(-4.22432454682835,2.91268259313759,15.3586995966211));
#58731=CARTESIAN_POINT('Ctrl Pts',(-5.51199907533185,3.21186725438272,14.9864886029628));
#58732=CARTESIAN_POINT('Ctrl Pts',(-6.12485002384382,3.37887789813221,14.7713535689273));
#58733=CARTESIAN_POINT('Ctrl Pts',(-6.17613843389023,3.39303090233569,14.753074354535));
#58734=CARTESIAN_POINT('Ctrl Pts',(6.37215938761968,2.78307364974066,14.8198971917583));
#58735=CARTESIAN_POINT('Ctrl Pts',(6.3199952273895,2.76864705353836,14.8382795416226));
#58736=CARTESIAN_POINT('Ctrl Pts',(5.69054844857231,2.59670875603571,15.056795096808));
#58737=CARTESIAN_POINT('Ctrl Pts',(4.36615521637009,2.28812300275669,15.435607729357));
#58738=CARTESIAN_POINT('Ctrl Pts',(2.2824842989152,1.97663889786705,15.7989326795465));
#58739=CARTESIAN_POINT('Ctrl Pts',(0.00161001422916566,1.85801376889573,
15.9327063761786));
#58740=CARTESIAN_POINT('Ctrl Pts',(-2.27951693148397,1.97632431053655,15.7992911267141));
#58741=CARTESIAN_POINT('Ctrl Pts',(-4.36376916166503,2.28765030166368,15.43617298023));
#58742=CARTESIAN_POINT('Ctrl Pts',(-5.68920595027655,2.59636352431106,15.0572281149511));
#58743=CARTESIAN_POINT('Ctrl Pts',(-6.31942557697566,2.76848948409855,14.8384803004125));
#58744=CARTESIAN_POINT('Ctrl Pts',(-6.37216345227932,2.78307475611255,14.8198957610868));
#58745=CARTESIAN_POINT('',(-6.26386065629335,3.90573732468848,15.8144217481535));
#58746=CARTESIAN_POINT('',(-6.249946130096,2.76546781932625,14.8593870899707));
#58747=CARTESIAN_POINT('Ctrl Pts',(-6.26386066455461,3.90573729438309,15.8144217478187));
#58748=CARTESIAN_POINT('Ctrl Pts',(-6.25434831141213,3.90345828807139,15.7850176820746));
#58749=CARTESIAN_POINT('Ctrl Pts',(-6.24501346021768,3.89973955504434,15.754986953564));
#58750=CARTESIAN_POINT('Ctrl Pts',(-6.23595867491624,3.89443139082405,15.724502287951));
#58751=CARTESIAN_POINT('Ctrl Pts',(-6.22713146317302,3.88925663648362,15.6947837922242));
#58752=CARTESIAN_POINT('Ctrl Pts',(-6.21857071083251,3.8825706633106,15.6646341979587));
#58753=CARTESIAN_POINT('Ctrl Pts',(-6.21037751462733,3.87426278352997,15.634253634215));
#58754=CARTESIAN_POINT('Ctrl Pts',(-6.20231060850718,3.86608296156923,15.6043413570694));
#58755=CARTESIAN_POINT('Ctrl Pts',(-6.19460034139449,3.85633023035241,15.5742056254424));
#58756=CARTESIAN_POINT('Ctrl Pts',(-6.18734460751122,3.844936061604,15.5440713466953));
#58757=CARTESIAN_POINT('Ctrl Pts',(-6.18021636223641,3.83374209682414,15.5144665495039));
#58758=CARTESIAN_POINT('Ctrl Pts',(-6.17352715644783,3.82096343865695,15.4848637891835));
#58759=CARTESIAN_POINT('Ctrl Pts',(-6.16736625649837,3.80657894180169,15.4555012511846));
#58760=CARTESIAN_POINT('Ctrl Pts',(-6.16656710070447,3.80471306926708,15.4516925150328));
#58761=CARTESIAN_POINT('Ctrl Pts',(-6.16577682489813,3.80282024355606,15.4478878475468));
#58762=CARTESIAN_POINT('Ctrl Pts',(-6.16499561473955,3.8009004789636,15.4440877906076));
#58763=CARTESIAN_POINT('Ctrl Pts',(-6.15906452005692,3.78632526454647,15.4152370424981));
#58764=CARTESIAN_POINT('Ctrl Pts',(-6.15365690109852,3.77019315686551,15.3866513455472));
#58765=CARTESIAN_POINT('Ctrl Pts',(-6.14884735387733,3.75253811793426,15.3585736969602));
#58766=CARTESIAN_POINT('Ctrl Pts',(-6.1440994216987,3.73510925746118,15.3308557507387));
#58767=CARTESIAN_POINT('Ctrl Pts',(-6.13993460837156,3.71619625756151,15.3036337249475));
#58768=CARTESIAN_POINT('Ctrl Pts',(-6.1364114164295,3.69588076477368,15.2771423239223));
#58769=CARTESIAN_POINT('Ctrl Pts',(-6.1329089125532,3.67568456388303,15.2508064795219));
#58770=CARTESIAN_POINT('Ctrl Pts',(-6.13004073682332,3.65410250414156,15.2251935101448));
#58771=CARTESIAN_POINT('Ctrl Pts',(-6.12784747118893,3.63126185987898,15.2005228928044));
#58772=CARTESIAN_POINT('Ctrl Pts',(-6.12566164681365,3.60849870880713,15.1759359773436));
#58773=CARTESIAN_POINT('Ctrl Pts',(-6.12414629946667,3.58448592772055,15.1522857758375));
#58774=CARTESIAN_POINT('Ctrl Pts',(-6.12332206340787,3.55939159786993,15.1297668076039));
#58775=CARTESIAN_POINT('Ctrl Pts',(-6.12249856901549,3.53431984847043,15.1072681024522));
#58776=CARTESIAN_POINT('Ctrl Pts',(-6.12236498739556,3.50816911136713,15.0858992186932));
#58777=CARTESIAN_POINT('Ctrl Pts',(-6.12292096736125,3.48114126735242,15.0658210949586));
#58778=CARTESIAN_POINT('Ctrl Pts',(-6.12347965668713,3.45398171325965,15.0456451280056));
#58779=CARTESIAN_POINT('Ctrl Pts',(-6.12473460135381,3.42593723222674,15.0267730077924));
#58780=CARTESIAN_POINT('Ctrl Pts',(-6.1266642557543,3.39723698661223,15.0093262589561));
#58781=CARTESIAN_POINT('Ctrl Pts',(-6.12860137628395,3.36842569534072,14.9918120059699));
#58782=CARTESIAN_POINT('Ctrl Pts',(-6.13121828625185,3.33895439904086,14.9757344144424));
#58783=CARTESIAN_POINT('Ctrl Pts',(-6.13447336941178,3.30906727489292,14.9611690045746));
#58784=CARTESIAN_POINT('Ctrl Pts',(-6.13776585195478,3.27883676166707,14.9464362449598));
#58785=CARTESIAN_POINT('Ctrl Pts',(-6.1417110334367,3.24818167679902,14.9332506648979));
#58786=CARTESIAN_POINT('Ctrl Pts',(-6.14624842574256,3.2173542835874,14.9216396889257));
#58787=CARTESIAN_POINT('Ctrl Pts',(-6.14955235103642,3.19490716036996,14.9131850976946));
#58788=CARTESIAN_POINT('Ctrl Pts',(-6.15316988431773,3.17236869747348,14.9055642707548));
#58789=CARTESIAN_POINT('Ctrl Pts',(-6.15707313882021,3.14983231529049,14.8987714964257));
#58790=CARTESIAN_POINT('Ctrl Pts',(-6.16252922916163,3.11833026051006,14.8892763455498));
#58791=CARTESIAN_POINT('Ctrl Pts',(-6.1685437480149,3.08683362732814,14.881400776874));
#58792=CARTESIAN_POINT('Ctrl Pts',(-6.1750305166369,3.05557747107911,14.8750891980218));
#58793=CARTESIAN_POINT('Ctrl Pts',(-6.18166567463506,3.02360630836121,14.8686332373822));
#58794=CARTESIAN_POINT('Ctrl Pts',(-6.18879458347136,2.99188738929926,14.8638131319262));
#58795=CARTESIAN_POINT('Ctrl Pts',(-6.19631949447585,2.96063879745935,14.8605266373239));
#58796=CARTESIAN_POINT('Ctrl Pts',(-6.20395586199788,2.9289273617104,14.8571914642398));
#58797=CARTESIAN_POINT('Ctrl Pts',(-6.21199969621026,2.89770067096357,14.8554349526722));
#58798=CARTESIAN_POINT('Ctrl Pts',(-6.22034867567113,2.86714473778872,14.8551162453579));
#58799=CARTESIAN_POINT('Ctrl Pts',(-6.22889787688057,2.83585602494922,14.8547898949376));
#58800=CARTESIAN_POINT('Ctrl Pts',(-6.23776670786458,2.80527084272535,14.8559703646471));
#58801=CARTESIAN_POINT('Ctrl Pts',(-6.24685040422301,2.77554055782156,14.8584824801066));
#58802=CARTESIAN_POINT('Ctrl Pts',(-6.24787961953862,2.77217201011222,14.8587671117811));
#58803=CARTESIAN_POINT('Ctrl Pts',(-6.24891160143422,2.76881438591469,14.8590688213317));
#58804=CARTESIAN_POINT('Ctrl Pts',(-6.24994620423252,2.76546786623744,14.8593873420339));
#58805=CARTESIAN_POINT('Ctrl Pts',(6.24994601128656,2.76546575640966,14.8593877892967));
#58806=CARTESIAN_POINT('Ctrl Pts',(6.23688268274706,2.76192003125581,14.8638898479677));
#58807=CARTESIAN_POINT('Ctrl Pts',(6.22381281177066,2.758383592908,14.8683771686433));
#58808=CARTESIAN_POINT('Ctrl Pts',(6.21073642273195,2.75485647619773,14.8728497532653));
#58809=CARTESIAN_POINT('Ctrl Pts',(5.89583157450962,2.66991665458339,14.9805582787141));
#58810=CARTESIAN_POINT('Ctrl Pts',(5.57714884580729,2.59038142383472,15.0797242785993));
#58811=CARTESIAN_POINT('Ctrl Pts',(5.25507847391284,2.51679039840292,15.1703536776165));
#58812=CARTESIAN_POINT('Ctrl Pts',(5.12540270308979,2.48716031199542,15.2068439549048));
#58813=CARTESIAN_POINT('Ctrl Pts',(4.99517746302832,2.4584940523232,15.2419498660761));
#58814=CARTESIAN_POINT('Ctrl Pts',(4.86442719004076,2.430827743042,15.2756698507746));
#58815=CARTESIAN_POINT('Ctrl Pts',(4.72158141783862,2.40060206761544,15.3125092174759));
#58816=CARTESIAN_POINT('Ctrl Pts',(4.57811215030979,2.37156574348657,15.3476943597705));
#58817=CARTESIAN_POINT('Ctrl Pts',(4.43405184968593,2.3437574901839,15.3812229418945));
#58818=CARTESIAN_POINT('Ctrl Pts',(4.34163140552557,2.32591738357279,15.4027328682138));
#58819=CARTESIAN_POINT('Ctrl Pts',(4.2489676810377,2.30858273346186,15.4235609671336));
#58820=CARTESIAN_POINT('Ctrl Pts',(4.1560722555045,2.29176233052638,15.4437067653028));
#58821=CARTESIAN_POINT('Ctrl Pts',(4.03722420398995,2.27024273359146,15.4694807885648));
#58822=CARTESIAN_POINT('Ctrl Pts',(3.91799531497457,2.24956537429438,15.4941382888263));
#58823=CARTESIAN_POINT('Ctrl Pts',(3.7984066156939,2.2297482034648,15.5176780933186));
#58824=CARTESIAN_POINT('Ctrl Pts',(3.73861226605356,2.21983961805001,15.5294479955647));
#58825=CARTESIAN_POINT('Ctrl Pts',(3.67872796073169,2.21014607752472,15.540938459558));
#58826=CARTESIAN_POINT('Ctrl Pts',(3.61875638520038,2.20066963256445,15.5521492675595));
#58827=CARTESIAN_POINT('Ctrl Pts',(3.58877059743473,2.19593141008432,15.5577546715602));
#58828=CARTESIAN_POINT('Ctrl Pts',(3.55876299195175,2.19124746136859,15.5632901606998));
#58829=CARTESIAN_POINT('Ctrl Pts',(3.52873390545623,2.18661803702737,15.568755703007));
#58830=CARTESIAN_POINT('Ctrl Pts',(3.51371936220847,2.18430332485676,15.5714884741606));
#58831=CARTESIAN_POINT('Ctrl Pts',(3.49869944869878,2.18200224377232,15.5742037585528));
#58832=CARTESIAN_POINT('Ctrl Pts',(3.48367420720818,2.1797148244456,15.5769015519158));
#58833=CARTESIAN_POINT('Ctrl Pts',(3.47616158646288,2.17857111478224,15.5782504485973));
#58834=CARTESIAN_POINT('Ctrl Pts',(3.46864763372183,2.17743082055785,15.5795949725182));
#58835=CARTESIAN_POINT('Ctrl Pts',(3.46113235428294,2.17629394556369,15.5809351231284));
#58836=CARTESIAN_POINT('Ctrl Pts',(3.45361707484405,2.17515707056953,15.5822752737386));
#58837=CARTESIAN_POINT('Ctrl Pts',(3.44743233343186,2.17422380971264,15.5833751816107));
#58838=CARTESIAN_POINT('Ctrl Pts',(3.43858254117336,2.17289358204932,15.5849424544647));
#58839=CARTESIAN_POINT('Ctrl Pts',(3.14008338800505,2.12802565527505,15.6378057992805));
#58840=CARTESIAN_POINT('Ctrl Pts',(2.84023806810342,2.08874745949898,15.6836350337927));
#58841=CARTESIAN_POINT('Ctrl Pts',(2.53936105399959,2.05530037816818,15.7224748688494));
#58842=CARTESIAN_POINT('Ctrl Pts',(2.46824426694122,2.04739465972102,15.7316552453808));
#58843=CARTESIAN_POINT('Ctrl Pts',(2.397069716932,2.03981481366109,15.740444968727));
#58844=CARTESIAN_POINT('Ctrl Pts',(2.32584133863707,2.03256421704252,15.7488443180986));
#58845=CARTESIAN_POINT('Ctrl Pts',(2.02872663239869,2.00231982659104,15.7838804972295));
#58846=CARTESIAN_POINT('Ctrl Pts',(1.73067698408626,1.97780192424327,15.8121272568313));
#58847=CARTESIAN_POINT('Ctrl Pts',(1.43206897838644,1.95907405420351,15.8336317426784));
#58848=CARTESIAN_POINT('Ctrl Pts',(1.13260365157316,1.94029241534949,15.8551979691667));
#58849=CARTESIAN_POINT('Ctrl Pts',(0.832576211040715,1.92733393854369,15.8699832033154));
#58850=CARTESIAN_POINT('Ctrl Pts',(0.532350103633079,1.92029402808205,15.8779965148456));
#58851=CARTESIAN_POINT('Ctrl Pts',(0.355508731868288,1.91614732866977,15.8827165740556));
#58852=CARTESIAN_POINT('Ctrl Pts',(0.178598162966609,1.91405469724503,15.8850863636833));
#58853=CARTESIAN_POINT('Ctrl Pts',(0.00169119634424886,1.91404105211554,
15.8851013992713));
#58854=CARTESIAN_POINT('Ctrl Pts',(0.00127018941862394,1.91404101964257,
15.8851014350533));
#58855=CARTESIAN_POINT('Ctrl Pts',(0.000849182513112402,1.91404099894601,
15.8851014574968));
#58856=CARTESIAN_POINT('Ctrl Pts',(0.000428175628690854,1.91404099002539,
15.885101466602));
#58857=CARTESIAN_POINT('Ctrl Pts',(-0.295821261727005,1.91403471286351,
15.8851078735931));
#58858=CARTESIAN_POINT('Ctrl Pts',(-0.592082537846746,1.91982817586115,
15.8785163704752));
#58859=CARTESIAN_POINT('Ctrl Pts',(-0.888018597841453,1.93134935298145,
15.8653354740815));
#58860=CARTESIAN_POINT('Ctrl Pts',(-1.16781466674178,1.94224217917986,15.8528734476707));
#58861=CARTESIAN_POINT('Ctrl Pts',(-1.44732031479291,1.95825540061563,15.8345208284142));
#58862=CARTESIAN_POINT('Ctrl Pts',(-1.72623621321286,1.97935406242927,15.8102539049019));
#58863=CARTESIAN_POINT('Ctrl Pts',(-1.92541348354479,1.99442087608708,15.7929245966339));
#58864=CARTESIAN_POINT('Ctrl Pts',(-2.12429486350001,2.01206591538091,15.772580171839));
#58865=CARTESIAN_POINT('Ctrl Pts',(-2.32276918863322,2.03225621732713,15.749205779174));
#58866=CARTESIAN_POINT('Ctrl Pts',(-2.41024261755301,2.04115467278718,15.7389040019846));
#58867=CARTESIAN_POINT('Ctrl Pts',(-2.49763694585371,2.05054760835353,15.7280135760389));
#58868=CARTESIAN_POINT('Ctrl Pts',(-2.5849451592377,2.06042746753833,15.7165340406164));
#58869=CARTESIAN_POINT('Ctrl Pts',(-2.72764899419556,2.07657593444503,15.6977709292798));
#58870=CARTESIAN_POINT('Ctrl Pts',(-2.8701197132973,2.09403058809539,15.6774337170849));
#58871=CARTESIAN_POINT('Ctrl Pts',(-3.0123190135386,2.11276975943822,15.6555185530409));
#58872=CARTESIAN_POINT('Ctrl Pts',(-3.08341866365925,2.12213934510964,15.6445609710189));
#58873=CARTESIAN_POINT('Ctrl Pts',(-3.15445045723932,2.13183005722226,15.6332088769221));
#58874=CARTESIAN_POINT('Ctrl Pts',(-3.22540966173381,2.14183879526575,15.621461681064));
#58875=CARTESIAN_POINT('Ctrl Pts',(-3.26088926398105,2.1468431642875,15.615588083135));
#58876=CARTESIAN_POINT('Ctrl Pts',(-3.29635071879944,2.15192703959139,15.6096157081738));
#58877=CARTESIAN_POINT('Ctrl Pts',(-3.33179343581059,2.15709002170296,15.603544473918));
#58878=CARTESIAN_POINT('Ctrl Pts',(-3.34951479431616,2.15967151275875,15.6005088567902));
#58879=CARTESIAN_POINT('Ctrl Pts',(-3.3672314683567,2.16227278050301,15.5974485247369));
#58880=CARTESIAN_POINT('Ctrl Pts',(-3.38494338430507,2.16489377364487,15.5943634669989));
#58881=CARTESIAN_POINT('Ctrl Pts',(-3.39379934227925,2.16620427021581,15.5928209381299));
#58882=CARTESIAN_POINT('Ctrl Pts',(-3.4026541107295,2.16751969813528,15.5912722278333));
#58883=CARTESIAN_POINT('Ctrl Pts',(-3.41150768046408,2.16884005090279,15.5897173347344));
#58884=CARTESIAN_POINT('Ctrl Pts',(-3.42036125019866,2.17016040367029,15.5881624416356));
#58885=CARTESIAN_POINT('Ctrl Pts',(-3.43054576231002,2.17168588194971,15.5863654858208));
#58886=CARTESIAN_POINT('Ctrl Pts',(-3.43806478433061,2.17281587722003,15.5850341056336));
#58887=CARTESIAN_POINT('Ctrl Pts',(-3.77201242870819,2.22300315658308,15.5259025754879));
#58888=CARTESIAN_POINT('Ctrl Pts',(-4.10337711699034,2.27999983117208,15.4581331881754));
#58889=CARTESIAN_POINT('Ctrl Pts',(-4.43166424742788,2.34336085642193,15.3817687090566));
#58890=CARTESIAN_POINT('Ctrl Pts',(-4.75049586433221,2.40489692121435,15.3076037233045));
#58891=CARTESIAN_POINT('Ctrl Pts',(-5.0664249048189,2.47243665009828,15.2253313086487));
#58892=CARTESIAN_POINT('Ctrl Pts',(-5.37910815822552,2.54552983393255,15.1349700559336));
#58893=CARTESIAN_POINT('Ctrl Pts',(-5.65842118622162,2.61082235689373,15.0542523493268));
#58894=CARTESIAN_POINT('Ctrl Pts',(-5.93514414538488,2.68054677629062,14.9670796084188));
#58895=CARTESIAN_POINT('Ctrl Pts',(-6.20901142408678,2.754393574655,14.8734392389871));
#58896=CARTESIAN_POINT('Ctrl Pts',(-6.22266346129535,2.75807477104978,14.8687713508999));
#58897=CARTESIAN_POINT('Ctrl Pts',(-6.23630839772604,2.76176621297451,14.8640873862658));
#58898=CARTESIAN_POINT('Ctrl Pts',(-6.24994620423252,2.76546786623744,14.8593873420339));
#58899=CARTESIAN_POINT('Ctrl Pts',(6.26385989004508,3.90573722903797,15.8144313886596));
#58900=CARTESIAN_POINT('Ctrl Pts',(5.97575428768946,3.82586736882485,15.9102651438246));
#58901=CARTESIAN_POINT('Ctrl Pts',(5.68582534910169,3.75094724810674,15.9988446813235));
#58902=CARTESIAN_POINT('Ctrl Pts',(5.3945598678898,3.6812480626751,16.0802607757235));
#58903=CARTESIAN_POINT('Ctrl Pts',(5.12091588958906,3.61576566391478,16.1567512128211));
#58904=CARTESIAN_POINT('Ctrl Pts',(4.84609219773543,3.55489216164144,16.2269184315589));
#58905=CARTESIAN_POINT('Ctrl Pts',(4.57049247071768,3.49883082501622,16.2908752458165));
#58906=CARTESIAN_POINT('Ctrl Pts',(4.3141786584873,3.44669254801345,16.3503564908012));
#58907=CARTESIAN_POINT('Ctrl Pts',(4.05719362167251,3.39871677068944,16.4044660162595));
#58908=CARTESIAN_POINT('Ctrl Pts',(3.79986208486601,3.35504215638728,16.4533307302619));
#58909=CARTESIAN_POINT('Ctrl Pts',(3.5788250075668,3.31752748089386,16.4953034853318));
#58910=CARTESIAN_POINT('Ctrl Pts',(3.35753227928865,3.28318603588267,16.5334069594315));
#58911=CARTESIAN_POINT('Ctrl Pts',(3.13618969347213,3.25208718836777,16.5677462998486));
#58912=CARTESIAN_POINT('Ctrl Pts',(2.89302858237386,3.21792281693557,16.6054705910844));
#58913=CARTESIAN_POINT('Ctrl Pts',(2.64982777084286,3.18767649632752,16.6386688269005));
#58914=CARTESIAN_POINT('Ctrl Pts',(2.40682922976721,3.16139780783334,16.6673754459146));
#58915=CARTESIAN_POINT('Ctrl Pts',(2.16739919224934,3.13550502944781,16.6956604999612));
#58916=CARTESIAN_POINT('Ctrl Pts',(1.9281655280082,3.11346424917113,16.7195848778018));
#58917=CARTESIAN_POINT('Ctrl Pts',(1.68935970347767,3.09529058551682,16.7392205017433));
#58918=CARTESIAN_POINT('Ctrl Pts',(1.45216061585603,3.07723919817726,16.758724012987));
#58919=CARTESIAN_POINT('Ctrl Pts',(1.21538363011777,3.06300312649857,16.7739962464026));
#58920=CARTESIAN_POINT('Ctrl Pts',(0.97925557199319,3.05256423844098,16.7851468963415));
#58921=CARTESIAN_POINT('Ctrl Pts',(0.744819945335308,3.04220017038896,16.796217624771));
#58922=CARTESIAN_POINT('Ctrl Pts',(0.511023977340595,3.03557908285324,16.8032256251656));
#58923=CARTESIAN_POINT('Ctrl Pts',(0.278089651340314,3.0326499369104,16.8063174478311));
#58924=CARTESIAN_POINT('Ctrl Pts',(0.185394849023527,3.03148430104732,16.8075478199093));
#58925=CARTESIAN_POINT('Ctrl Pts',(0.0928364957948917,3.03090294439015,
16.8081584672785));
#58926=CARTESIAN_POINT('Ctrl Pts',(0.000428580633955471,3.03090115441879,
16.8081603748149));
#58927=CARTESIAN_POINT('Ctrl Pts',(0.000285720792900251,3.03090115165155,
16.8081603777639));
#58928=CARTESIAN_POINT('Ctrl Pts',(0.000142860581873481,3.0309011502693,
16.8081603792583));
#58929=CARTESIAN_POINT('Ctrl Pts',(9.25926002537381E-13,3.03090115027208,
16.8081603792981));
#58930=CARTESIAN_POINT('Ctrl Pts',(-0.229766623293178,3.03090115473717,
16.8081604432517));
#58931=CARTESIAN_POINT('Ctrl Pts',(-0.460490123967034,3.0344866432905,16.8043944620728));
#58932=CARTESIAN_POINT('Ctrl Pts',(-0.69194503962102,3.04172214172834,16.7967026659101));
#58933=CARTESIAN_POINT('Ctrl Pts',(-0.925222791853488,3.04901462375271,
16.7889502925616));
#58934=CARTESIAN_POINT('Ctrl Pts',(-1.15924352503365,3.06001481866249,16.7772100212543));
#58935=CARTESIAN_POINT('Ctrl Pts',(-1.39377640777272,3.07475437006698,16.7613587211585));
#58936=CARTESIAN_POINT('Ctrl Pts',(-1.62977802676596,3.08958622628291,16.745408154048));
#58937=CARTESIAN_POINT('Ctrl Pts',(-1.86629822996335,3.10820436967548,16.7252949381079));
#58938=CARTESIAN_POINT('Ctrl Pts',(-2.10310182209333,3.13060683891653,16.7009341835963));
#58939=CARTESIAN_POINT('Ctrl Pts',(-2.34274022974235,3.15327749187429,16.6762818024065));
#58940=CARTESIAN_POINT('Ctrl Pts',(-2.58266885192898,3.17982357446078,16.6472795948639));
#58941=CARTESIAN_POINT('Ctrl Pts',(-2.82264394517536,3.21020880819815,16.6138806971338));
#58942=CARTESIAN_POINT('Ctrl Pts',(-2.92710054047309,3.2234349227111,16.5993427919855));
#58943=CARTESIAN_POINT('Ctrl Pts',(-3.031565940621,3.23738800871796,16.5839723683053));
#58944=CARTESIAN_POINT('Ctrl Pts',(-3.13602004348828,3.25206312380919,16.5677679300934));
#58945=CARTESIAN_POINT('Ctrl Pts',(-3.39881199848447,3.28898366669603,16.5269998235238));
#58946=CARTESIAN_POINT('Ctrl Pts',(-3.66152807655967,3.330475068804,16.4809254841673));
#58947=CARTESIAN_POINT('Ctrl Pts',(-3.92382420254392,3.37641784233135,16.4293734954318));
#58948=CARTESIAN_POINT('Ctrl Pts',(-4.19336752573358,3.42363000685205,16.3763971340439));
#58949=CARTESIAN_POINT('Ctrl Pts',(-4.46246736982849,3.47554247180431,16.3176366166871));
#58950=CARTESIAN_POINT('Ctrl Pts',(-4.73075034417782,3.53198937119391,16.2529547001071));
#58951=CARTESIAN_POINT('Ctrl Pts',(-5.02422899918551,3.59373745696935,16.182198209028));
#58952=CARTESIAN_POINT('Ctrl Pts',(-5.31673014775518,3.66091130547962,16.1043559293831));
#58953=CARTESIAN_POINT('Ctrl Pts',(-5.60776500962217,3.73325701383207,16.0193031511413));
#58954=CARTESIAN_POINT('Ctrl Pts',(-5.82736838303714,3.78784621838432,15.9551256952159));
#58955=CARTESIAN_POINT('Ctrl Pts',(-6.04613690946994,3.84537918370047,15.8868441243541));
#58956=CARTESIAN_POINT('Ctrl Pts',(-6.26386060035812,3.90573752918775,15.8144217504419));
#58957=CARTESIAN_POINT('Ctrl Pts',(-6.390311350216,8.98426037265861,25.6807373550228));
#58958=CARTESIAN_POINT('Ctrl Pts',(-4.260207566811,8.27687305387726,25.9287992801895));
#58959=CARTESIAN_POINT('Ctrl Pts',(0.0001663376447509,7.56887468463083,
26.1774672305152));
#58960=CARTESIAN_POINT('Ctrl Pts',(4.2605402421,8.27692834075613,25.9287798619571));
#58961=CARTESIAN_POINT('Ctrl Pts',(6.39081036315,8.98442609659955,25.6806792400505));
#58962=CARTESIAN_POINT('Ctrl Pts',(-6.390311350216,8.18394872075491,25.1149839598735));
#58963=CARTESIAN_POINT('Ctrl Pts',(-4.260207566811,7.53598946889127,25.3660580162986));
#58964=CARTESIAN_POINT('Ctrl Pts',(0.0001663376447509,6.88615615907008,
25.6190369308858));
#58965=CARTESIAN_POINT('Ctrl Pts',(4.2605402421,7.53604021371134,25.3660382614307));
#58966=CARTESIAN_POINT('Ctrl Pts',(6.39081036315,8.18410052210986,25.1149251392324));
#58967=CARTESIAN_POINT('Ctrl Pts',(-6.390311350216,6.63374485883001,23.7052292454154));
#58968=CARTESIAN_POINT('Ctrl Pts',(-4.260207566811,6.0952594820613,23.9981327481698));
#58969=CARTESIAN_POINT('Ctrl Pts',(0.0001663376447509,5.55782025246395,
24.2900565601985));
#58970=CARTESIAN_POINT('Ctrl Pts',(4.2605402421,6.09530145014608,23.9981099521357));
#58971=CARTESIAN_POINT('Ctrl Pts',(6.39081036315,6.63387101309451,23.7051606251128));
#58972=CARTESIAN_POINT('Ctrl Pts',(-6.390311350216,4.89945807530355,21.0044950488482));
#58973=CARTESIAN_POINT('Ctrl Pts',(-4.260207566811,4.44478852897079,21.4424839271908));
#58974=CARTESIAN_POINT('Ctrl Pts',(0.0001663376447509,3.9894320739417,21.8807691942861));
#58975=CARTESIAN_POINT('Ctrl Pts',(4.2605402421,4.44482408729352,21.4424497019397));
#58976=CARTESIAN_POINT('Ctrl Pts',(6.39081036315,4.89956459350057,21.0043924385214));
#58977=CARTESIAN_POINT('Ctrl Pts',(-6.390311350216,4.02649740779966,18.1257286739828));
#58978=CARTESIAN_POINT('Ctrl Pts',(-4.260207566811,3.53810588786846,18.7393844386643));
#58979=CARTESIAN_POINT('Ctrl Pts',(0.0001663376447509,3.05102639999064,
19.3530201602777));
#58980=CARTESIAN_POINT('Ctrl Pts',(4.2605402421,3.53814392341047,18.7393365204708));
#58981=CARTESIAN_POINT('Ctrl Pts',(6.39081036315,4.02661182627713,18.1255849090983));
#58982=CARTESIAN_POINT('Ctrl Pts',(-6.390311350216,3.91822558910252,16.240123855731));
#58983=CARTESIAN_POINT('Ctrl Pts',(-4.260207566811,3.34432525984736,16.9588977715367));
#58984=CARTESIAN_POINT('Ctrl Pts',(0.0001663376447509,2.76847548009877,
17.6776814527756));
#58985=CARTESIAN_POINT('Ctrl Pts',(4.2605402421,3.34437022737152,16.9588416424509));
#58986=CARTESIAN_POINT('Ctrl Pts',(6.39081036315,3.91836004022115,16.2399554641724));
#58987=CARTESIAN_POINT('Ctrl Pts',(-6.390311350216,3.94962416452014,15.4599810530666));
#58988=CARTESIAN_POINT('Ctrl Pts',(-4.260207566811,3.32898447675662,16.2180891202845));
#58989=CARTESIAN_POINT('Ctrl Pts',(0.0001663376447509,2.70679255855811,
16.9762181824682));
#58990=CARTESIAN_POINT('Ctrl Pts',(4.2605402421,3.32903306309379,16.2180299187524));
#58991=CARTESIAN_POINT('Ctrl Pts',(6.39081036315,3.94976956555253,15.4598034464652));
#58992=CARTESIAN_POINT('',(-6.27159361731543,8.76070973784035,25.560856303641));
#58993=CARTESIAN_POINT('Ctrl Pts',(-6.27159386307865,8.7607092746329,25.560857167973));
#58994=CARTESIAN_POINT('Ctrl Pts',(-6.19789584443463,8.73653383838215,25.5688564326203));
#58995=CARTESIAN_POINT('Ctrl Pts',(-6.11723339296007,8.71055314298554,25.5775121686293));
#58996=CARTESIAN_POINT('Ctrl Pts',(-6.02951379280947,8.6830033204438,25.5867458367231));
#58997=CARTESIAN_POINT('Ctrl Pts',(-5.94295765287483,8.65581890224077,25.595857034976));
#58998=CARTESIAN_POINT('Ctrl Pts',(-5.84953032636904,8.62710668875392,25.6055309450653));
#58999=CARTESIAN_POINT('Ctrl Pts',(-5.74914273791409,8.5971414490545,25.6156747169211));
#59000=CARTESIAN_POINT('Ctrl Pts',(-5.64673108221044,8.56657203446444,25.6260230128292));
#59001=CARTESIAN_POINT('Ctrl Pts',(-5.53707566211109,8.53469824792391,25.6368604233356));
#59002=CARTESIAN_POINT('Ctrl Pts',(-5.42008190491958,8.50186484299704,25.6480690713867));
#59003=CARTESIAN_POINT('Ctrl Pts',(-5.30308814772807,8.46903143807017,25.6592777194379));
#59004=CARTESIAN_POINT('Ctrl Pts',(-5.1787560534444,8.43523827313954,25.6708576585075));
#59005=CARTESIAN_POINT('Ctrl Pts',(-5.04699104937212,8.40088573760002,25.6826707313487));
#59006=CARTESIAN_POINT('Ctrl Pts',(-4.91609386884737,8.36675945287322,25.694406001568));
#59007=CARTESIAN_POINT('Ctrl Pts',(-4.77785368976756,8.33207908056211,25.7063721043635));
#59008=CARTESIAN_POINT('Ctrl Pts',(-4.63217381914409,8.29729989669217,25.7184182727122));
#59009=CARTESIAN_POINT('Ctrl Pts',(-4.48649394852062,8.26252071282223,25.7304644410609));
#59010=CARTESIAN_POINT('Ctrl Pts',(-4.33337438635348,8.22764256319013,25.7425907306237));
#59011=CARTESIAN_POINT('Ctrl Pts',(-4.17271843965407,8.19317938183559,25.754624827507));
#59012=CARTESIAN_POINT('Ctrl Pts',(-4.01206249295466,8.15871620048106,25.7666589243902));
#59013=CARTESIAN_POINT('Ctrl Pts',(-3.84387131200249,8.12466886539935,25.7786011414393));
#59014=CARTESIAN_POINT('Ctrl Pts',(-3.66807400178512,8.0916212708232,25.7902592314014));
#59015=CARTESIAN_POINT('Ctrl Pts',(-3.58017534667644,8.07509747353512,25.7960882763825));
#59016=CARTESIAN_POINT('Ctrl Pts',(-3.49037543354537,8.05882467347477,25.8018459904061));
#59017=CARTESIAN_POINT('Ctrl Pts',(-3.39866732483497,8.04288236229473,25.8075066450451));
#59018=CARTESIAN_POINT('Ctrl Pts',(-3.35281327047977,8.0349112067047,25.8103369723646));
#59019=CARTESIAN_POINT('Ctrl Pts',(-3.30648215931862,8.02702270521989,25.8131429946146));
#59020=CARTESIAN_POINT('Ctrl Pts',(-3.25967330048623,8.01922725194684,25.8159214242958));
#59021=CARTESIAN_POINT('Ctrl Pts',(-3.23626887107004,8.01532952531032,25.8173106391365));
#59022=CARTESIAN_POINT('Ctrl Pts',(-3.21274500420225,8.01145506267285,25.8186929533658));
#59023=CARTESIAN_POINT('Ctrl Pts',(-3.18910161784883,8.00760518302979,25.8200679461676));
#59024=CARTESIAN_POINT('Ctrl Pts',(-3.17727992467212,8.00568024320826,25.8207554425686));
#59025=CARTESIAN_POINT('Ctrl Pts',(-3.16542835159289,8.00376144925788,25.8214411084579));
#59026=CARTESIAN_POINT('Ctrl Pts',(-3.1535468890103,8.00184896775755,25.8221248909217));
#59027=CARTESIAN_POINT('Ctrl Pts',(-3.14166542642771,7.99993648625723,25.8228086733855));
#59028=CARTESIAN_POINT('Ctrl Pts',(-3.12814002921763,7.99777354469439,25.8235824798023));
#59029=CARTESIAN_POINT('Ctrl Pts',(-3.11781282328897,7.99613062797019,25.8241705346935));
#59030=CARTESIAN_POINT('Ctrl Pts',(-2.86369606000897,7.95570413863917,25.8386405284771));
#59031=CARTESIAN_POINT('Ctrl Pts',(-2.61950244535401,7.92184254420193,25.8508203757612));
#59032=CARTESIAN_POINT('Ctrl Pts',(-2.38554390379139,7.89344260645399,25.8610830655099));
#59033=CARTESIAN_POINT('Ctrl Pts',(-2.16264725215207,7.86638545783056,25.8708605208082));
#59034=CARTESIAN_POINT('Ctrl Pts',(-1.94904069704484,7.84428557582742,25.878897909814));
#59035=CARTESIAN_POINT('Ctrl Pts',(-1.74499397723141,7.82623317289244,25.8855028517309));
#59036=CARTESIAN_POINT('Ctrl Pts',(-1.60616344485852,7.81395057059251,25.8899967617701));
#59037=CARTESIAN_POINT('Ctrl Pts',(-1.4717584003362,7.80354254385131,25.8938272527317));
#59038=CARTESIAN_POINT('Ctrl Pts',(-1.34186380268046,7.7947356937536,25.8970866460556));
#59039=CARTESIAN_POINT('Ctrl Pts',(-1.16964671100351,7.78305937974182,25.9014080208395));
#59040=CARTESIAN_POINT('Ctrl Pts',(-1.00532510305835,7.77419108036862,25.9047256080539));
#59041=CARTESIAN_POINT('Ctrl Pts',(-0.848989845323112,7.76752305953098,
25.9072401816312));
#59042=CARTESIAN_POINT('Ctrl Pts',(-0.768759682953442,7.76410107780889,
25.9085306432284));
#59043=CARTESIAN_POINT('Ctrl Pts',(-0.690632862249034,7.76125935835357,
25.90960933956));
#59044=CARTESIAN_POINT('Ctrl Pts',(-0.6146216645542,7.7589208015061,25.9105016070156));
#59045=CARTESIAN_POINT('Ctrl Pts',(-0.502558941606541,7.75547308516901,
25.9118170700488));
#59046=CARTESIAN_POINT('Ctrl Pts',(-0.395091323682923,7.75311817417789,
25.9127277681256));
#59047=CARTESIAN_POINT('Ctrl Pts',(-0.292241207601631,7.75162351521975,
25.913310108436));
#59048=CARTESIAN_POINT('Ctrl Pts',(-0.240816149560984,7.75087618574069,
25.9136012785912));
#59049=CARTESIAN_POINT('Ctrl Pts',(-0.19054531473662,7.75034420169172,25.913810266976));
#59050=CARTESIAN_POINT('Ctrl Pts',(-0.141430651316284,7.7500001640364,25.9139459993008));
#59051=CARTESIAN_POINT('Ctrl Pts',(-0.102793828366503,7.74972952140035,
25.9140527752703));
#59052=CARTESIAN_POINT('Ctrl Pts',(-0.0657687540226224,7.74957755785452,
25.9141133378556));
#59053=CARTESIAN_POINT('Ctrl Pts',(-0.0282408776468195,7.74952492844427,
25.9141339361307));
#59054=CARTESIAN_POINT('Ctrl Pts',(-0.0188695811777211,7.74951178605909,
25.9141390798415));
#59055=CARTESIAN_POINT('Ctrl Pts',(-0.00946693103737975,7.74950507576206,
25.9141416457731));
#59056=CARTESIAN_POINT('Ctrl Pts',(9.29034748332288E-13,7.74950497091013,
25.9141415602278));
#59057=CARTESIAN_POINT('Ctrl Pts',(0.000814034408002238,7.74950496189421,
25.914141552872));
#59058=CARTESIAN_POINT('Ctrl Pts',(0.00162854409452201,7.74950500183509,
25.9141415258694));
#59059=CARTESIAN_POINT('Ctrl Pts',(0.00244354999465827,7.74950509090949,
25.9141414791492));
#59060=CARTESIAN_POINT('Ctrl Pts',(0.132296585289549,7.74951928293074,25.9141340353286));
#59061=CARTESIAN_POINT('Ctrl Pts',(0.269950165813914,7.75078018591596,25.9136311334706));
#59062=CARTESIAN_POINT('Ctrl Pts',(0.415338008371231,7.75379326809187,25.9124697500803));
#59063=CARTESIAN_POINT('Ctrl Pts',(0.562124815418347,7.75683534302876,25.9112971915182));
#59064=CARTESIAN_POINT('Ctrl Pts',(0.716795443280676,7.76166350274542,25.9094534038994));
#59065=CARTESIAN_POINT('Ctrl Pts',(0.879281676902341,7.76884826647791,25.9067525338815));
#59066=CARTESIAN_POINT('Ctrl Pts',(1.03425298681161,7.7757007377439,25.9041765780282));
#59067=CARTESIAN_POINT('Ctrl Pts',(1.19633368294311,7.78469728741838,25.900820828321));
#59068=CARTESIAN_POINT('Ctrl Pts',(1.36546458400579,7.79637447397498,25.8965091992107));
#59069=CARTESIAN_POINT('Ctrl Pts',(1.56040862413761,7.80983385904544,25.8915395195541));
#59070=CARTESIAN_POINT('Ctrl Pts',(1.76469848348762,7.82685195067153,25.8852992336672));
#59071=CARTESIAN_POINT('Ctrl Pts',(1.97810882769652,7.84828951177721,25.877498195159));
#59072=CARTESIAN_POINT('Ctrl Pts',(2.05047989003362,7.85555935184465,25.8748527308715));
#59073=CARTESIAN_POINT('Ctrl Pts',(2.12389981084038,7.86333785656272,25.8720276315337));
#59074=CARTESIAN_POINT('Ctrl Pts',(2.19835980240383,7.87165986000744,25.8690111431811));
#59075=CARTESIAN_POINT('Ctrl Pts',(2.34537492442379,7.88809097054327,25.863055335318));
#59076=CARTESIAN_POINT('Ctrl Pts',(2.49643931797058,7.90664055205604,25.8563543239282));
#59077=CARTESIAN_POINT('Ctrl Pts',(2.65146457128827,7.9275790342485,25.8488159962454));
#59078=CARTESIAN_POINT('Ctrl Pts',(2.72897719794712,7.93804827534472,25.845046832404));
#59079=CARTESIAN_POINT('Ctrl Pts',(2.80748002846577,7.94911480280078,25.8410682634669));
#59080=CARTESIAN_POINT('Ctrl Pts',(2.88696074174985,7.96081263315031,25.8368685087714));
#59081=CARTESIAN_POINT('Ctrl Pts',(2.9267010983919,7.96666154832508,25.8347686314237));
#59082=CARTESIAN_POINT('Ctrl Pts',(2.96668592478411,7.97266829189018,25.8326134542077));
#59083=CARTESIAN_POINT('Ctrl Pts',(3.00691356216396,7.97883714334385,25.8304015173849));
#59084=CARTESIAN_POINT('Ctrl Pts',(3.02702738085389,7.98192156907068,25.8292955489735));
#59085=CARTESIAN_POINT('Ctrl Pts',(3.04720190226842,7.98504652189608,25.828175390503));
#59086=CARTESIAN_POINT('Ctrl Pts',(3.06743691470062,7.98821253678811,25.8270408588531));
#59087=CARTESIAN_POINT('Ctrl Pts',(3.07755442091672,7.98979554423412,25.8264735930282));
#59088=CARTESIAN_POINT('Ctrl Pts',(3.08768704988573,7.9913888172036,25.8259027338999));
#59089=CARTESIAN_POINT('Ctrl Pts',(3.09783477468347,7.99299242260474,25.8253282586107));
#59090=CARTESIAN_POINT('Ctrl Pts',(3.1079824994812,7.99459602800587,25.8247537833214));
#59091=CARTESIAN_POINT('Ctrl Pts',(3.11649259020815,7.99594619889963,25.8242701557867));
#59092=CARTESIAN_POINT('Ctrl Pts',(3.12832320949474,7.99783430303326,25.8235939613969));
#59093=CARTESIAN_POINT('Ctrl Pts',(3.31761311808016,8.02804396917128,25.8127748511597));
#59094=CARTESIAN_POINT('Ctrl Pts',(3.49939719834751,8.05986842387775,25.8014674996312));
#59095=CARTESIAN_POINT('Ctrl Pts',(3.67375234747637,8.09268657565345,25.789880031812));
#59096=CARTESIAN_POINT('Ctrl Pts',(3.84164845972872,8.12428896951435,25.7787218250862));
#59097=CARTESIAN_POINT('Ctrl Pts',(4.00265585952441,8.15681325436566,25.7673037128964));
#59098=CARTESIAN_POINT('Ctrl Pts',(4.15684321068927,8.18975608782384,25.7557927511104));
#59099=CARTESIAN_POINT('Ctrl Pts',(4.31992804411597,8.22459990910065,25.7436175417222));
#59100=CARTESIAN_POINT('Ctrl Pts',(4.47538300777857,8.25991157362596,25.7313386112449));
#59101=CARTESIAN_POINT('Ctrl Pts',(4.62328935151025,8.29515455818551,25.7191318794806));
#59102=CARTESIAN_POINT('Ctrl Pts',(4.77119569524193,8.33039754274507,25.7069251477163));
#59103=CARTESIAN_POINT('Ctrl Pts',(4.91155341904269,8.36557198094537,25.6947905665999));
#59104=CARTESIAN_POINT('Ctrl Pts',(5.04444377274572,8.40020003885417,25.6828823980407));
#59105=CARTESIAN_POINT('Ctrl Pts',(5.17491740965991,8.43419835798525,25.6711907889991));
#59106=CARTESIAN_POINT('Ctrl Pts',(5.29821637053551,8.46768019613915,25.6597182023876));
#59107=CARTESIAN_POINT('Ctrl Pts',(5.4144320887901,8.50026217361815,25.6485965003309));
#59108=CARTESIAN_POINT('Ctrl Pts',(5.52974605649533,8.53259133834057,25.6375610946986));
#59109=CARTESIAN_POINT('Ctrl Pts',(5.6380862768788,8.56403474748396,25.626871076913));
#59110=CARTESIAN_POINT('Ctrl Pts',(5.73954207145701,8.59426848248594,25.6166368019706));
#59111=CARTESIAN_POINT('Ctrl Pts',(5.84223096597527,8.62486968015452,25.6062781390239));
#59112=CARTESIAN_POINT('Ctrl Pts',(5.93786707024696,8.65423164742993,25.5963863521321));
#59113=CARTESIAN_POINT('Ctrl Pts',(6.02654300239053,8.68206912588511,25.5870574344231));
#59114=CARTESIAN_POINT('Ctrl Pts',(6.11514461892748,8.70988327490863,25.5777363348915));
#59115=CARTESIAN_POINT('Ctrl Pts',(6.19679772450881,8.73617562297342,25.5689771098566));
#59116=CARTESIAN_POINT('Ctrl Pts',(6.27159470458989,8.76071047653694,25.5608577605037));
#59117=CARTESIAN_POINT('Ctrl Pts',(-6.27159552384839,8.76070944182917,25.5608567088099));
#59118=CARTESIAN_POINT('Ctrl Pts',(-6.27195777361699,8.56459406830873,25.4158727684));
#59119=CARTESIAN_POINT('Ctrl Pts',(-6.2722903133114,8.37478235054355,25.2662940221908));
#59120=CARTESIAN_POINT('Ctrl Pts',(-6.27259314317768,8.1913536795449,25.1127468866755));
#59121=CARTESIAN_POINT('Ctrl Pts',(-6.2728986358801,8.00631208806859,24.9578495842652));
#59122=CARTESIAN_POINT('Ctrl Pts',(-6.27317389396976,7.82776621191305,24.7989137498099));
#59123=CARTESIAN_POINT('Ctrl Pts',(-6.2734189176993,7.65576229132537,24.636542046575));
#59124=CARTESIAN_POINT('Ctrl Pts',(-6.27366754287355,7.4812301967884,24.4717837470997));
#59125=CARTESIAN_POINT('Ctrl Pts',(-6.27388503836533,7.31343373081403,24.3034878218648));
#59126=CARTESIAN_POINT('Ctrl Pts',(-6.27407140443858,7.1523860062935,24.1322428455118));
#59127=CARTESIAN_POINT('Ctrl Pts',(-6.2742180449349,7.02566702872147,23.99750025053));
#59128=CARTESIAN_POINT('Ctrl Pts',(-6.27434541261665,6.90312560578793,23.8609310108925));
#59129=CARTESIAN_POINT('Ctrl Pts',(-6.27445350761239,6.78475354200027,23.7228045339272));
#59130=CARTESIAN_POINT('Ctrl Pts',(-6.27450262993924,6.73096093886088,23.6600348016045));
#59131=CARTESIAN_POINT('Ctrl Pts',(-6.27454777221241,6.67802917492449,23.596943288945));
#59132=CARTESIAN_POINT('Ctrl Pts',(-6.27458893444397,6.62595269073056,23.5335577352352));
#59133=CARTESIAN_POINT('Ctrl Pts',(-6.27470712624797,6.47642208026929,23.3515546548168));
#59134=CARTESIAN_POINT('Ctrl Pts',(-6.2747925032677,6.33394460102529,23.1671310836941));
#59135=CARTESIAN_POINT('Ctrl Pts',(-6.27484506550317,6.19837397944143,22.9809084183222));
#59136=CARTESIAN_POINT('Ctrl Pts',(-6.27489762773865,6.06280335785757,22.7946857529503));
#59137=CARTESIAN_POINT('Ctrl Pts',(-6.27491737518986,5.93413948700878,22.6066638313622));
#59138=CARTESIAN_POINT('Ctrl Pts',(-6.2749043078568,5.8122156331048,22.4174136415825));
#59139=CARTESIAN_POINT('Ctrl Pts',(-6.27489476774449,5.72320227013048,22.2792471114374));
#59140=CARTESIAN_POINT('Ctrl Pts',(-6.27486753879387,5.63762486509131,22.1401744339752));
#59141=CARTESIAN_POINT('Ctrl Pts',(-6.27482283819033,5.55559553449373,22.0006684995205));
#59142=CARTESIAN_POINT('Ctrl Pts',(-6.27477792069608,5.47316819138009,21.8604856717208));
#59143=CARTESIAN_POINT('Ctrl Pts',(-6.27471536159001,5.39432351602081,21.719865714071));
#59144=CARTESIAN_POINT('Ctrl Pts',(-6.27463538123425,5.31912418999798,21.579301685377));
#59145=CARTESIAN_POINT('Ctrl Pts',(-6.27457691148509,5.26414961920891,21.476542158736));
#59146=CARTESIAN_POINT('Ctrl Pts',(-6.27450913119094,5.21112218524964,21.3738128162492));
#59147=CARTESIAN_POINT('Ctrl Pts',(-6.27443212644733,5.16004899754176,21.2713091693909));
#59148=CARTESIAN_POINT('Ctrl Pts',(-6.27435635475634,5.10979362863869,21.1704468810169));
#59149=CARTESIAN_POINT('Ctrl Pts',(-6.27427024761671,5.06062331622896,21.0681861191557));
#59150=CARTESIAN_POINT('Ctrl Pts',(-6.27417380502847,5.01262251510087,20.9645377933533));
#59151=CARTESIAN_POINT('Ctrl Pts',(-6.27399075539136,4.92151619592085,20.7678115464762));
#59152=CARTESIAN_POINT('Ctrl Pts',(-6.27377047264002,4.83462175639446,20.5660838236771));
#59153=CARTESIAN_POINT('Ctrl Pts',(-6.27351295677444,4.75246063087173,20.359496943365));
#59154=CARTESIAN_POINT('Ctrl Pts',(-6.27325823305762,4.67119034787724,20.1551500077663));
#59155=CARTESIAN_POINT('Ctrl Pts',(-6.27296707925897,4.59455128074756,19.9460486010722));
#59156=CARTESIAN_POINT('Ctrl Pts',(-6.27263949537848,4.52307269166766,19.7323746340451));
#59157=CARTESIAN_POINT('Ctrl Pts',(-6.27231699866829,4.45270411982966,19.5220188884686));
#59158=CARTESIAN_POINT('Ctrl Pts',(-6.27195919456296,4.38733700196248,19.3072314291763));
#59159=CARTESIAN_POINT('Ctrl Pts',(-6.27156608306249,4.32750028726097,19.0882301610031));
#59160=CARTESIAN_POINT('Ctrl Pts',(-6.27136275163803,4.29655058362445,18.9749548186019));
#59161=CARTESIAN_POINT('Ctrl Pts',(-6.271149974317,4.2670808390044,18.8605528781773));
#59162=CARTESIAN_POINT('Ctrl Pts',(-6.2709277510994,4.23916681564939,18.7450593575327));
#59163=CARTESIAN_POINT('Ctrl Pts',(-6.27050608302727,4.18620001703831,18.5259106532752));
#59164=CARTESIAN_POINT('Ctrl Pts',(-6.27005040565995,4.13883316994885,18.3028289465057));
#59165=CARTESIAN_POINT('Ctrl Pts',(-6.26956071854046,4.09760165659947,18.0760878674739));
#59166=CARTESIAN_POINT('Ctrl Pts',(-6.26938505201858,4.08281058643722,17.9947485486814));
#59167=CARTESIAN_POINT('Ctrl Pts',(-6.26920500882359,4.06880928510534,17.9129387397966));
#59168=CARTESIAN_POINT('Ctrl Pts',(-6.26902058893439,4.05562321457744,17.8306725394457));
#59169=CARTESIAN_POINT('Ctrl Pts',(-6.26850854166759,4.01901170047753,17.6022580055087));
#59170=CARTESIAN_POINT('Ctrl Pts',(-6.26796275395663,3.98868443887669,17.3703213887534));
#59171=CARTESIAN_POINT('Ctrl Pts',(-6.26738322534997,3.96507786816877,17.1352143265461));
#59172=CARTESIAN_POINT('Ctrl Pts',(-6.26681231314397,3.94182227870524,16.9036028237013));
#59173=CARTESIAN_POINT('Ctrl Pts',(-6.26620865589936,3.92508904508753,16.6689144045329));
#59174=CARTESIAN_POINT('Ctrl Pts',(-6.26557225318442,3.91530350242448,16.4315347899381));
#59175=CARTESIAN_POINT('Ctrl Pts',(-6.26502584174864,3.90690169600378,16.2277221207056));
#59176=CARTESIAN_POINT('Ctrl Pts',(-6.26445529089762,3.90362174274592,16.02192627987));
#59177=CARTESIAN_POINT('Ctrl Pts',(-6.26386060035812,3.90573752918775,15.8144217504419));
#59178=CARTESIAN_POINT('Ctrl Pts',(-6.09387055512539,9.75736361516117,25.6953077691695));
#59179=CARTESIAN_POINT('Ctrl Pts',(-6.05578069227928,9.74451714524749,25.6998076991855));
#59180=CARTESIAN_POINT('Ctrl Pts',(-5.7118011452561,9.62959716207432,25.7401664910213));
#59181=CARTESIAN_POINT('Ctrl Pts',(-5.02575508002472,9.41991852694549,25.8155531544346));
#59182=CARTESIAN_POINT('Ctrl Pts',(-3.98545756790916,9.15752992500609,25.9125296973922));
#59183=CARTESIAN_POINT('Ctrl Pts',(-2.81199940005833,8.93210922179495,25.9977998207745));
#59184=CARTESIAN_POINT('Ctrl Pts',(-1.52033800454874,8.77271519431179,26.0595632938288));
#59185=CARTESIAN_POINT('Ctrl Pts',(-0.189364146702586,8.70902521570103,
26.0852161182419));
#59186=CARTESIAN_POINT('Ctrl Pts',(1.08600948443229,8.74409647810586,26.0709736512751));
#59187=CARTESIAN_POINT('Ctrl Pts',(2.24105687247373,8.85467761705376,26.0276782166891));
#59188=CARTESIAN_POINT('Ctrl Pts',(3.2726709241743,9.01596244605114,25.9659557725239));
#59189=CARTESIAN_POINT('Ctrl Pts',(4.19957173728585,9.2102230477197,25.8929883674436));
#59190=CARTESIAN_POINT('Ctrl Pts',(5.05653935127232,9.43093766095788,25.8116628442957));
#59191=CARTESIAN_POINT('Ctrl Pts',(5.67993901992691,9.61982782716416,25.7436848816572));
#59192=CARTESIAN_POINT('Ctrl Pts',(6.0218052874218,9.73305033543495,25.7038225890372));
#59193=CARTESIAN_POINT('Ctrl Pts',(6.09373583888459,9.75730938060936,25.6953260385087));
#59194=CARTESIAN_POINT('Ctrl Pts',(-6.21813195904801,9.42872268326465,25.8362993824541));
#59195=CARTESIAN_POINT('Ctrl Pts',(-6.17931198320937,9.41558743764238,25.8407694982643));
#59196=CARTESIAN_POINT('Ctrl Pts',(-5.82873515267428,9.29807096860313,25.8808306633429));
#59197=CARTESIAN_POINT('Ctrl Pts',(-5.12944745498144,9.08342540207168,25.9551345139311));
#59198=CARTESIAN_POINT('Ctrl Pts',(-4.06852260420401,8.8143072231865,26.0496506589018));
#59199=CARTESIAN_POINT('Ctrl Pts',(-2.87108324194528,8.58268008383095,26.1318474967083));
#59200=CARTESIAN_POINT('Ctrl Pts',(-1.55234198144858,8.41859936175768,26.1906370912154));
#59201=CARTESIAN_POINT('Ctrl Pts',(-0.193311005377795,8.35288471919688,
26.2145712771427));
#59202=CARTESIAN_POINT('Ctrl Pts',(1.10882136147559,8.38908730322682,26.2013369838684));
#59203=CARTESIAN_POINT('Ctrl Pts',(2.28821900828739,8.50299476126,26.160351622698));
#59204=CARTESIAN_POINT('Ctrl Pts',(3.34121045601103,8.66886917024187,26.1012117007145));
#59205=CARTESIAN_POINT('Ctrl Pts',(4.2868974775528,8.86836587472699,26.0306330877797));
#59206=CARTESIAN_POINT('Ctrl Pts',(5.16080887717921,9.09469004474556,25.9512681740581));
#59207=CARTESIAN_POINT('Ctrl Pts',(5.79625990804498,9.28807268518097,25.8843031567456));
#59208=CARTESIAN_POINT('Ctrl Pts',(6.144685049683,9.40386174784378,25.8447556017848));
#59209=CARTESIAN_POINT('Ctrl Pts',(6.21799459468972,9.42866605228754,25.836314917434));
#59210=CARTESIAN_POINT('Ctrl Pts',(-6.32901962278943,9.07127866903577,25.7779388186334));
#59211=CARTESIAN_POINT('Ctrl Pts',(-6.28949395526499,9.05793150332501,25.7823663832484));
#59212=CARTESIAN_POINT('Ctrl Pts',(-5.93255281589158,8.93852936550552,25.822012056803));
#59213=CARTESIAN_POINT('Ctrl Pts',(-5.22070660987746,8.72061347463833,25.8949526569753));
#59214=CARTESIAN_POINT('Ctrl Pts',(-4.14072872696723,8.44768011879346,25.9865501773639));
#59215=CARTESIAN_POINT('Ctrl Pts',(-2.92175304970983,8.21303070472776,26.0652056115562));
#59216=CARTESIAN_POINT('Ctrl Pts',(-1.57937527961094,8.04705905770207,26.1206423805555));
#59217=CARTESIAN_POINT('Ctrl Pts',(-0.196590777430159,7.98076752197201,
26.1426783013704));
#59218=CARTESIAN_POINT('Ctrl Pts',(1.12799798891678,8.01726693809018,26.1305544980894));
#59219=CARTESIAN_POINT('Ctrl Pts',(2.32844022148747,8.13240355674583,26.0921550930378));
#59220=CARTESIAN_POINT('Ctrl Pts',(3.40033110933316,8.30032567273698,26.0359566715004));
#59221=CARTESIAN_POINT('Ctrl Pts',(4.36302821848509,8.50249774507351,25.9681511314834));
#59222=CARTESIAN_POINT('Ctrl Pts',(5.25262945577457,8.73205768537551,25.8911219437363));
#59223=CARTESIAN_POINT('Ctrl Pts',(5.89949730737536,8.92837895799797,25.8254258028569));
#59224=CARTESIAN_POINT('Ctrl Pts',(6.25423659942717,9.04601668254853,25.7863121700845));
#59225=CARTESIAN_POINT('Ctrl Pts',(6.32887899044518,9.07122133557283,25.7779513691211));
#59226=CARTESIAN_POINT('Ctrl Pts',(-6.39488356451668,8.78685862461965,25.5363210871781));
#59227=CARTESIAN_POINT('Ctrl Pts',(-6.35487788243824,8.77343702129268,25.5407054600534));
#59228=CARTESIAN_POINT('Ctrl Pts',(-5.99362047734077,8.65339956398283,25.5799359106881));
#59229=CARTESIAN_POINT('Ctrl Pts',(-5.27348111855406,8.43484693326501,25.6516207146261));
#59230=CARTESIAN_POINT('Ctrl Pts',(-4.18146072739243,8.16210843159642,25.740672220695));
#59231=CARTESIAN_POINT('Ctrl Pts',(-2.94954017637816,7.92849121802153,25.8163264943927));
#59232=CARTESIAN_POINT('Ctrl Pts',(-1.59371729035546,7.76397112863256,25.8689863324045));
#59233=CARTESIAN_POINT('Ctrl Pts',(-0.198266597753138,7.69871888560939,
25.8894850580979));
#59234=CARTESIAN_POINT('Ctrl Pts',(1.13806229620182,7.73459374464174,25.8782577446869));
#59235=CARTESIAN_POINT('Ctrl Pts',(2.35023472334337,7.84850622225583,25.8419836867962));
#59236=CARTESIAN_POINT('Ctrl Pts',(3.43315220364043,8.01534345346998,25.7882481148275));
#59237=CARTESIAN_POINT('Ctrl Pts',(4.40622894576758,8.21686044545929,25.7228103861928));
#59238=CARTESIAN_POINT('Ctrl Pts',(5.30578955887226,8.44635339776932,25.6478271591733));
#59239=CARTESIAN_POINT('Ctrl Pts',(5.96018308030503,8.64321743602772,25.5832947728205));
#59240=CARTESIAN_POINT('Ctrl Pts',(6.31919099850295,8.76145692896501,25.5446108624864));
#59241=CARTESIAN_POINT('Ctrl Pts',(6.3947399743137,8.78680248751152,25.5363312532158));
#59242=CARTESIAN_POINT('',(5.98852581355243,9.69456736137294,25.7188095578805));
#59243=CARTESIAN_POINT('Origin',(5.99999764423362,9.33250908123741,24.7867226423621));
#59244=CARTESIAN_POINT('',(-5.98852245733777,9.69456809190998,25.7188096065452));
#59245=CARTESIAN_POINT('Ctrl Pts',(-5.98852261949133,9.69456765143689,25.7188097472679));
#59246=CARTESIAN_POINT('Ctrl Pts',(-5.87209162705512,9.65602993335219,25.7323460956292));
#59247=CARTESIAN_POINT('Ctrl Pts',(-5.74896424736322,9.6164051610127,25.7463642488386));
#59248=CARTESIAN_POINT('Ctrl Pts',(-5.61913822764799,9.57607812122987,25.7607354226545));
#59249=CARTESIAN_POINT('Ctrl Pts',(-5.51166398174339,9.54269407233328,25.7726323526536));
#59250=CARTESIAN_POINT('Ctrl Pts',(-5.39959907267352,9.50882946946539,25.7847708339679));
#59251=CARTESIAN_POINT('Ctrl Pts',(-5.28294523335611,9.47472488475404,25.7970626699146));
#59252=CARTESIAN_POINT('Ctrl Pts',(-5.21062717308089,9.45358218231708,25.8046828368811));
#59253=CARTESIAN_POINT('Ctrl Pts',(-5.13654508001346,9.43235034959351,25.8123606216791));
#59254=CARTESIAN_POINT('Ctrl Pts',(-5.06069907855041,9.41109782338285,25.8200693992105));
#59255=CARTESIAN_POINT('Ctrl Pts',(-5.00147803450858,9.39450371470942,25.8260884621128));
#59256=CARTESIAN_POINT('Ctrl Pts',(-4.9411816374162,9.37789704478032,25.8321263597675));
#59257=CARTESIAN_POINT('Ctrl Pts',(-4.87980975520643,9.36131224719765,25.8381705190934));
#59258=CARTESIAN_POINT('Ctrl Pts',(-4.80982349490603,9.34239954778453,25.8450630583581));
#59259=CARTESIAN_POINT('Ctrl Pts',(-4.73843872583953,9.32351554899608,25.8519636512814));
#59260=CARTESIAN_POINT('Ctrl Pts',(-4.66565544719248,9.30471492867056,25.8588519543252));
#59261=CARTESIAN_POINT('Ctrl Pts',(-4.62926380786896,9.2953146185078,25.8622961058471));
#59262=CARTESIAN_POINT('Ctrl Pts',(-4.5925225411935,9.28593515099749,25.8657371798275));
#59263=CARTESIAN_POINT('Ctrl Pts',(-4.55543164722946,9.276583697005,25.8691724714731));
#59264=CARTESIAN_POINT('Ctrl Pts',(-4.53688620024744,9.27190797000876,25.8708901172959));
#59265=CARTESIAN_POINT('Ctrl Pts',(-4.5182533464447,9.2672392462662,25.8726063172043));
#59266=CARTESIAN_POINT('Ctrl Pts',(-4.49953308583469,9.26257842951481,25.8743207280067));
#59267=CARTESIAN_POINT('Ctrl Pts',(-4.49017295552969,9.26024802113911,25.8751779334078));
#59268=CARTESIAN_POINT('Ctrl Pts',(-4.48079097352291,9.257919589503,25.8760346915106));
#59269=CARTESIAN_POINT('Ctrl Pts',(-4.47138713981614,9.25559324869522,25.8768909588464));
#59270=CARTESIAN_POINT('Ctrl Pts',(-4.46198330610937,9.25326690788744,25.8777472261823));
#59271=CARTESIAN_POINT('Ctrl Pts',(-4.45131619556557,9.25063753651448,25.8787153833017));
#59272=CARTESIAN_POINT('Ctrl Pts',(-4.44311008359767,9.24862061315132,25.879458244869));
#59273=CARTESIAN_POINT('Ctrl Pts',(-4.30892004448045,9.21563897384911,25.8916058518184));
#59274=CARTESIAN_POINT('Ctrl Pts',(-4.17039904010703,9.1830097895467,25.9036805413857));
#59275=CARTESIAN_POINT('Ctrl Pts',(-4.02753916638022,9.15105780377832,25.9155540151468));
#59276=CARTESIAN_POINT('Ctrl Pts',(-3.89083751623016,9.12048316398505,25.9269156621496));
#59277=CARTESIAN_POINT('Ctrl Pts',(-3.7501627969802,9.09052877936022,25.9380928402357));
#59278=CARTESIAN_POINT('Ctrl Pts',(-3.60552271823339,9.06149687437662,25.9489689143327));
#59279=CARTESIAN_POINT('Ctrl Pts',(-3.45762471998779,9.03181104545884,25.9600899646091));
#59280=CARTESIAN_POINT('Ctrl Pts',(-3.30557667061893,9.00309070988402,25.9708958864366));
#59281=CARTESIAN_POINT('Ctrl Pts',(-3.14937857027222,8.97567617574966,25.9812526344922));
#59282=CARTESIAN_POINT('Ctrl Pts',(-3.07127952009887,8.96196890868248,25.98643100852));
#59283=CARTESIAN_POINT('Ctrl Pts',(-2.99214295707096,8.94858831228371,25.9914969566742));
#59284=CARTESIAN_POINT('Ctrl Pts',(-2.91196888033323,8.93557803426197,25.9964329681702));
#59285=CARTESIAN_POINT('Ctrl Pts',(-2.89544646589152,8.93289685333387,25.9974501900822));
#59286=CARTESIAN_POINT('Ctrl Pts',(-2.87887999163314,8.93023139589497,25.9984618940561));
#59287=CARTESIAN_POINT('Ctrl Pts',(-2.86226945200005,8.9275820550892,25.99946792148));
#59288=CARTESIAN_POINT('Ctrl Pts',(-2.83857914202376,8.9238035080758,26.0009027394959));
#59289=CARTESIAN_POINT('Ctrl Pts',(-2.81479919798029,8.92005774359815,26.002326011));
#59290=CARTESIAN_POINT('Ctrl Pts',(-2.79092962977707,8.91634587600413,26.003737295366));
#59291=CARTESIAN_POINT('Ctrl Pts',(-2.7706267321079,8.91318864805257,26.0049377009124));
#59292=CARTESIAN_POINT('Ctrl Pts',(-2.75025898982132,8.91005594735042,26.0061294327482));
#59293=CARTESIAN_POINT('Ctrl Pts',(-2.7298264029262,8.90694846685246,26.0073122162978));
#59294=CARTESIAN_POINT('Ctrl Pts',(-2.71961010947864,8.90539472660348,26.0079036080727));
#59295=CARTESIAN_POINT('Ctrl Pts',(-2.70937760487891,8.9038472914013,26.0084927627642));
#59296=CARTESIAN_POINT('Ctrl Pts',(-2.69912888912821,8.90230624805375,26.0090796459032));
#59297=CARTESIAN_POINT('Ctrl Pts',(-2.68888017337751,8.9007652047062,26.0096665290422));
#59298=CARTESIAN_POINT('Ctrl Pts',(-2.67721604462066,8.89902257795092,26.010330388956));
#59299=CARTESIAN_POINT('Ctrl Pts',(-2.6683341084243,8.89770238042146,26.0108334461247));
#59300=CARTESIAN_POINT('Ctrl Pts',(-2.48253474165827,8.87008544425381,26.0213567938855));
#59301=CARTESIAN_POINT('Ctrl Pts',(-2.2918411092769,8.84458851855033,26.0311242682293));
#59302=CARTESIAN_POINT('Ctrl Pts',(-2.09624736712906,8.8216845816214,26.0399422366958));
#59303=CARTESIAN_POINT('Ctrl Pts',(-1.99263644895492,8.80955179092498,26.0446133360839));
#59304=CARTESIAN_POINT('Ctrl Pts',(-1.88765086776274,8.79814730437633,26.0490176494173));
#59305=CARTESIAN_POINT('Ctrl Pts',(-1.78129230367924,8.78754624690616,26.0531239528998));
#59306=CARTESIAN_POINT('Ctrl Pts',(-1.70032438874362,8.77947594690853,26.0562499713256));
#59307=CARTESIAN_POINT('Ctrl Pts',(-1.61856086797209,8.77187004290322,26.059203690954));
#59308=CARTESIAN_POINT('Ctrl Pts',(-1.53600027727007,8.76475978009922,26.0619717492177));
#59309=CARTESIAN_POINT('Ctrl Pts',(-1.46197046667242,8.75838420303267,26.0644537909187));
#59310=CARTESIAN_POINT('Ctrl Pts',(-1.38729978418251,8.7524071578645,26.0667865511724));
#59311=CARTESIAN_POINT('Ctrl Pts',(-1.31198948711474,8.74685080292186,26.0689596020403));
#59312=CARTESIAN_POINT('Ctrl Pts',(-1.23234002195582,8.74097430639156,26.0712578580043));
#59313=CARTESIAN_POINT('Ctrl Pts',(-1.15197439044148,8.73556841058776,26.073377465122));
#59314=CARTESIAN_POINT('Ctrl Pts',(-1.07089259101654,8.73065879334457,26.0753059915675));
#59315=CARTESIAN_POINT('Ctrl Pts',(-1.03035169130407,8.72820398472298,26.0762702547902));
#59316=CARTESIAN_POINT('Ctrl Pts',(-0.989631749612645,8.72587324436221,
26.0771867436368));
#59317=CARTESIAN_POINT('Ctrl Pts',(-0.948732765844986,8.72366974188885,
26.0780538888504));
#59318=CARTESIAN_POINT('Ctrl Pts',(-0.928283273961157,8.72256799065217,
26.0784874614572));
#59319=CARTESIAN_POINT('Ctrl Pts',(-0.907789021558714,8.72149804879681,
26.0789086978804));
#59320=CARTESIAN_POINT('Ctrl Pts',(-0.887250008635169,8.7204603094842,26.0793174011297));
#59321=CARTESIAN_POINT('Ctrl Pts',(-0.876980502173397,8.7199414398279,26.0795217527544));
#59322=CARTESIAN_POINT('Ctrl Pts',(-0.866699805581386,8.71943062080149,
26.0797229710681));
#59323=CARTESIAN_POINT('Ctrl Pts',(-0.856407918859501,8.71892790132903,
26.0799210314036));
#59324=CARTESIAN_POINT('Ctrl Pts',(-0.846116032137616,8.71842518185657,
26.0801190917392));
#59325=CARTESIAN_POINT('Ctrl Pts',(-0.834124913337858,8.7178509455999,26.0803453710984));
#59326=CARTESIAN_POINT('Ctrl Pts',(-0.825498688304884,8.71744409041346,
26.0805057137582));
#59327=CARTESIAN_POINT('Ctrl Pts',(-0.603586179648995,8.70697760539389,
26.084630582023));
#59328=CARTESIAN_POINT('Ctrl Pts',(-0.379552796555947,8.70066335356724,
26.0871469150606));
#59329=CARTESIAN_POINT('Ctrl Pts',(-0.153393845956384,8.698714469009,26.0879160669694));
#59330=CARTESIAN_POINT('Ctrl Pts',(-0.0982314036651066,8.69823911646739,
26.0881036708545));
#59331=CARTESIAN_POINT('Ctrl Pts',(-0.042942542021569,8.69802366194984,
26.0881872185615));
#59332=CARTESIAN_POINT('Ctrl Pts',(0.0124721856994969,8.69806975931062,
26.0881665546718));
#59333=CARTESIAN_POINT('Ctrl Pts',(0.153776193840033,8.69818730462956,26.0881138630759));
#59334=CARTESIAN_POINT('Ctrl Pts',(0.295901299624064,8.70001019720623,26.087381983723));
#59335=CARTESIAN_POINT('Ctrl Pts',(0.438847517233882,8.70357851179769,26.0859643099591));
#59336=CARTESIAN_POINT('Ctrl Pts',(0.510320626038792,8.70536266909342,26.0852554730772));
#59337=CARTESIAN_POINT('Ctrl Pts',(0.581999012323971,8.70758318342142,26.0843751914009));
#59338=CARTESIAN_POINT('Ctrl Pts',(0.653882676053584,8.71024373540388,26.0833231229802));
#59339=CARTESIAN_POINT('Ctrl Pts',(0.689824507918391,8.71157401139511,26.0827970887698));
#59340=CARTESIAN_POINT('Ctrl Pts',(0.725817659130263,8.71301429695668,26.0822281083633));
#59341=CARTESIAN_POINT('Ctrl Pts',(0.761862129614743,8.71456501226555,26.0816161561889));
#59342=CARTESIAN_POINT('Ctrl Pts',(0.779884364856982,8.71534036991999,26.0813101801018));
#59343=CARTESIAN_POINT('Ctrl Pts',(0.797919429916728,8.71614333502365,26.0809934611126));
#59344=CARTESIAN_POINT('Ctrl Pts',(0.815967324782474,8.71697395525709,26.0806659979335));
#59345=CARTESIAN_POINT('Ctrl Pts',(0.83401521964822,8.71780457549052,26.0803385347544));
#59346=CARTESIAN_POINT('Ctrl Pts',(0.853700655374708,8.71874249564784,26.0799689583905));
#59347=CARTESIAN_POINT('Ctrl Pts',(0.870149498784838,8.71954882757381,26.0796513752337));
#59348=CARTESIAN_POINT('Ctrl Pts',(0.954975880144235,8.72370706640852,26.0780136047657));
#59349=CARTESIAN_POINT('Ctrl Pts',(1.03918186933026,8.7284368786165,26.0761547094014));
#59350=CARTESIAN_POINT('Ctrl Pts',(1.12276164329517,8.73371220957732,26.0740868617806));
#59351=CARTESIAN_POINT('Ctrl Pts',(1.34023325878723,8.74743843413957,26.0687063954145));
#59352=CARTESIAN_POINT('Ctrl Pts',(1.55346394526637,8.76485473917061,26.0619130100553));
#59353=CARTESIAN_POINT('Ctrl Pts',(1.76245348567662,8.78548898909608,26.0539195188657));
#59354=CARTESIAN_POINT('Ctrl Pts',(1.93914916545501,8.80293475604758,26.0471612124127));
#59355=CARTESIAN_POINT('Ctrl Pts',(2.11281359860282,8.82268164254982,26.0395445710804));
#59356=CARTESIAN_POINT('Ctrl Pts',(2.28345799976991,8.84446770250537,26.0311854117516));
#59357=CARTESIAN_POINT('Ctrl Pts',(2.31474293705894,8.84846183014638,26.0296528928199));
#59358=CARTESIAN_POINT('Ctrl Pts',(2.34592639292191,8.85252455266215,26.0280953865591));
#59359=CARTESIAN_POINT('Ctrl Pts',(2.37700846453754,8.85665426172438,26.0265135770043));
#59360=CARTESIAN_POINT('Ctrl Pts',(2.47789359773873,8.87005833124641,26.0213793932338));
#59361=CARTESIAN_POINT('Ctrl Pts',(2.57857877971435,8.88427984309705,26.0159461893127));
#59362=CARTESIAN_POINT('Ctrl Pts',(2.67829454913604,8.89918228045029,26.010268885374));
#59363=CARTESIAN_POINT('Ctrl Pts',(2.78016201893597,8.91440628760413,26.0044690746633));
#59364=CARTESIAN_POINT('Ctrl Pts',(2.88101763983595,8.93034084026915,25.9984145814764));
#59365=CARTESIAN_POINT('Ctrl Pts',(2.9800513379607,8.94678980911212,25.9921818732103));
#59366=CARTESIAN_POINT('Ctrl Pts',(3.01383476948858,8.95240105683015,25.9900557052804));
#59367=CARTESIAN_POINT('Ctrl Pts',(3.04740628009826,8.95807174850422,25.9879089442522));
#59368=CARTESIAN_POINT('Ctrl Pts',(3.08073402057498,8.96379283741397,25.9857450608471));
#59369=CARTESIAN_POINT('Ctrl Pts',(3.15917419640476,8.97725799327511,25.9806521444854));
#59370=CARTESIAN_POINT('Ctrl Pts',(3.23647655748982,8.99103650927858,25.9754514131821));
#59371=CARTESIAN_POINT('Ctrl Pts',(3.31263963066391,9.00508372882959,25.9701602706044));
#59372=CARTESIAN_POINT('Ctrl Pts',(3.45655652485398,9.03162719832913,25.9601621865625));
#59373=CARTESIAN_POINT('Ctrl Pts',(3.59640516989599,9.05912869720995,25.9498420248917));
#59374=CARTESIAN_POINT('Ctrl Pts',(3.73218981795613,9.08729847637573,25.9393136497869));
#59375=CARTESIAN_POINT('Ctrl Pts',(3.83601182259918,9.10883731000034,25.9312635717801));
#59376=CARTESIAN_POINT('Ctrl Pts',(3.93745684683485,9.13076709674976,25.923091594256));
#59377=CARTESIAN_POINT('Ctrl Pts',(4.03652489001273,9.15296524319345,25.9148447710799));
#59378=CARTESIAN_POINT('Ctrl Pts',(4.0612919008072,9.15851477980437,25.9127830652858));
#59379=CARTESIAN_POINT('Ctrl Pts',(4.08692151241491,9.16430499799161,25.9106334161247));
#59380=CARTESIAN_POINT('Ctrl Pts',(4.11487271596183,9.17068852739269,25.9082656521577));
#59381=CARTESIAN_POINT('Ctrl Pts',(4.14282391950875,9.17707205679377,25.9058978881908));
#59382=CARTESIAN_POINT('Ctrl Pts',(4.17059661622636,9.1834801016058,25.9035230642124));
#59383=CARTESIAN_POINT('Ctrl Pts',(4.19819080613438,9.18990996456923,25.9011421988763));
#59384=CARTESIAN_POINT('Ctrl Pts',(4.20585187599977,9.19169510954185,25.9004811910431));
#59385=CARTESIAN_POINT('Ctrl Pts',(4.21349918708703,9.19348193687302,25.8998197172862));
#59386=CARTESIAN_POINT('Ctrl Pts',(4.22113273884194,9.1952703903218,25.8991577987902));
#59387=CARTESIAN_POINT('Ctrl Pts',(4.26848933350235,9.20636549621251,25.8950514264333));
#59388=CARTESIAN_POINT('Ctrl Pts',(4.31531637062675,9.21752315728304,25.8909279539873));
#59389=CARTESIAN_POINT('Ctrl Pts',(4.36161386414175,9.22873008213421,25.8867925860485));
#59390=CARTESIAN_POINT('Ctrl Pts',(4.51956603546999,9.26696450866056,25.8726840394387));
#59391=CARTESIAN_POINT('Ctrl Pts',(4.67135538159587,9.30576725556285,25.8584396044212));
#59392=CARTESIAN_POINT('Ctrl Pts',(4.81697964948199,9.34464732854181,25.8442463695933));
#59393=CARTESIAN_POINT('Ctrl Pts',(4.86961306902873,9.35869987090179,25.8391164658055));
#59394=CARTESIAN_POINT('Ctrl Pts',(4.92144124545563,9.37276293483443,25.8339930114225));
#59395=CARTESIAN_POINT('Ctrl Pts',(4.97246446091363,9.38681474486927,25.8288840498562));
#59396=CARTESIAN_POINT('Ctrl Pts',(5.00468126036627,9.39568726185541,25.8256581773055));
#59397=CARTESIAN_POINT('Ctrl Pts',(5.03657708832332,9.4045544425085,25.8224384021553));
#59398=CARTESIAN_POINT('Ctrl Pts',(5.06815190938425,9.41341154727271,25.8192264433304));
#59399=CARTESIAN_POINT('Ctrl Pts',(5.21039246414893,9.45331167822954,25.8047569771611));
#59400=CARTESIAN_POINT('Ctrl Pts',(5.34611826469743,9.49300395844047,25.7904485750103));
#59401=CARTESIAN_POINT('Ctrl Pts',(5.47532885619636,9.53208557266711,25.7764520422943));
#59402=CARTESIAN_POINT('Ctrl Pts',(5.60705590595806,9.57192832613088,25.762182918222));
#59403=CARTESIAN_POINT('Ctrl Pts',(5.73201169332115,9.61113637645999,25.7482377381105));
#59404=CARTESIAN_POINT('Ctrl Pts',(5.85019776510156,9.64932746814793,25.734746207583));
#59405=CARTESIAN_POINT('Ctrl Pts',(5.86233276528394,9.65324881774198,25.7333609366881));
#59406=CARTESIAN_POINT('Ctrl Pts',(5.87439639539093,9.65715948412718,25.7319804242722));
#59407=CARTESIAN_POINT('Ctrl Pts',(5.88638865699179,9.6610590795782,25.7306047944961));
#59408=CARTESIAN_POINT('Ctrl Pts',(5.92103004145991,9.67232362581519,25.7266310886558));
#59409=CARTESIAN_POINT('Ctrl Pts',(5.95507590117461,9.68349577951184,25.7226981412014));
#59410=CARTESIAN_POINT('Ctrl Pts',(5.98852582160936,9.69456702970002,25.7188089328355));
#59411=CARTESIAN_POINT('Origin',(-5.999994980806,9.33250914740904,24.7867195890732));
#59412=CARTESIAN_POINT('Origin',(5.999999877386,9.33250977407517,24.7867246592848));
#59413=CARTESIAN_POINT('Origin',(6.,9.33250981977681,24.7867247762149));
#59414=CARTESIAN_POINT('Ctrl Pts',(6.9999999999895,10.9278021978942,24.1259274561224));
#59415=CARTESIAN_POINT('Ctrl Pts',(6.9999999999895,10.9277942569348,24.1259309538583));
#59416=CARTESIAN_POINT('Ctrl Pts',(6.9999999999895,10.6629101446723,24.2426037363051));
#59417=CARTESIAN_POINT('Ctrl Pts',(6.9999999999895,10.1335216816106,24.468757012286));
#59418=CARTESIAN_POINT('Ctrl Pts',(6.9999999999895,9.5992651391747,24.6831018468203));
#59419=CARTESIAN_POINT('Ctrl Pts',(6.9999999999895,9.3325057408578,24.7867214499759));
#59420=CARTESIAN_POINT('Ctrl Pts',(7.00000270561806,11.1660644378675,24.6668575635543));
#59421=CARTESIAN_POINT('Ctrl Pts',(7.00000270561806,11.1660563761497,24.6668611144804));
#59422=CARTESIAN_POINT('Ctrl Pts',(7.00000270561806,10.8971441621799,24.7853081441803));
#59423=CARTESIAN_POINT('Ctrl Pts',(7.00000270561804,10.3597134220153,25.0148970046547));
#59424=CARTESIAN_POINT('Ctrl Pts',(7.00000270561804,9.8173405913843,25.2324981642003));
#59425=CARTESIAN_POINT('Ctrl Pts',(7.00000270561804,9.54652457492641,25.3376935135328));
#59426=CARTESIAN_POINT('Ctrl Pts',(6.57967197773943,11.3336093881527,25.0472372157089));
#59427=CARTESIAN_POINT('Ctrl Pts',(6.57967197773943,11.333601241518,25.0472408040382));
#59428=CARTESIAN_POINT('Ctrl Pts',(6.57967197773943,11.0618564842979,25.1669354765322));
#59429=CARTESIAN_POINT('Ctrl Pts',(6.57967197773943,10.5187704505481,25.3989402247821));
#59430=CARTESIAN_POINT('Ctrl Pts',(6.57967197773943,9.97069028206527,25.6188312176277));
#59431=CARTESIAN_POINT('Ctrl Pts',(6.57967197773943,9.69702166972346,25.7251346246858));
#59432=CARTESIAN_POINT('Ctrl Pts',(5.98852435812654,11.3308746780979,25.0410285650898));
#59433=CARTESIAN_POINT('Ctrl Pts',(5.98852435812654,11.3308665328493,25.0410321528085));
#59434=CARTESIAN_POINT('Ctrl Pts',(5.98852435812654,11.0591680090977,25.1607064609686));
#59435=CARTESIAN_POINT('Ctrl Pts',(5.98852435812654,10.5161742824468,25.3926717765052));
#59436=CARTESIAN_POINT('Ctrl Pts',(5.98852435812654,9.96818727053848,25.6125253941221));
#59437=CARTESIAN_POINT('Ctrl Pts',(5.98852435812654,9.69456521897248,25.7188107151854));
#59438=CARTESIAN_POINT('',(6.9999999999401,10.9277762175509,24.1259366383994));
#59439=CARTESIAN_POINT('',(5.98852583813019,11.3308502415552,25.0410393194074));
#59440=CARTESIAN_POINT('Origin',(5.99999999906,10.9277802195584,24.1259421376201));
#59441=CARTESIAN_POINT('Origin',(5.98846854897676,-4.75314842173399,-11.4751152994772));
#59442=CARTESIAN_POINT('Origin',(6.99999997874015,-4.74964876082222,-11.4663999132518));
#59443=CARTESIAN_POINT('Ctrl Pts',(-6.05497710532883,11.6468330260664,24.9009950262097));
#59444=CARTESIAN_POINT('Ctrl Pts',(-4.03665140355255,12.1728066175418,24.6398170408189));
#59445=CARTESIAN_POINT('Ctrl Pts',(7.59695908486568E-7,12.7121751393787,
24.4084894089112));
#59446=CARTESIAN_POINT('Ctrl Pts',(4.0366529229439,12.1728064145219,24.6398171278867));
#59447=CARTESIAN_POINT('Ctrl Pts',(6.05497938441634,11.646832432147,24.9009953211277));
#59448=CARTESIAN_POINT('Ctrl Pts',(-6.05497710532883,10.8985073422741,25.2386054571744));
#59449=CARTESIAN_POINT('Ctrl Pts',(-4.03665140355255,11.070715415319,25.1429517412782));
#59450=CARTESIAN_POINT('Ctrl Pts',(7.59695908486568E-7,11.3017723854694,
25.1799926939185));
#59451=CARTESIAN_POINT('Ctrl Pts',(4.0366529229439,11.0707153283507,25.1429517273329));
#59452=CARTESIAN_POINT('Ctrl Pts',(6.05497938441634,10.8985071478217,25.2386055651884));
#59453=CARTESIAN_POINT('Ctrl Pts',(-6.05497710532883,10.1393897253838,25.5530351225277));
#59454=CARTESIAN_POINT('Ctrl Pts',(-4.03665140355255,9.94970084961926,25.6072791213988));
#59455=CARTESIAN_POINT('Ctrl Pts',(7.59695908486568E-7,9.81221489841592,
25.796939183938));
#59456=CARTESIAN_POINT('Ctrl Pts',(4.0366529229439,9.9497009013654,25.6072790500129));
#59457=CARTESIAN_POINT('Ctrl Pts',(6.05497938441634,10.1393899395764,25.5530350612747));
#59458=CARTESIAN_POINT('Ctrl Pts',(-6.05497710532883,9.37151240627548,25.8434422446624));
#59459=CARTESIAN_POINT('Ctrl Pts',(-4.03665140355255,8.81462746052429,26.0307842227122));
#59460=CARTESIAN_POINT('Ctrl Pts',(7.59695908486568E-7,8.2693467820933,
26.2486239006384));
#59461=CARTESIAN_POINT('Ctrl Pts',(4.0366529229439,8.8146276657733,26.0307841407194));
#59462=CARTESIAN_POINT('Ctrl Pts',(6.05497938441634,9.37151303510997,25.8434420331122));
#59463=CARTESIAN_POINT('',(-5.98852246661619,11.3308498387676,25.041039515264));
#59464=CARTESIAN_POINT('Ctrl Pts',(-5.98852262876941,11.3308502497312,25.0410393033033));
#59465=CARTESIAN_POINT('Ctrl Pts',(-5.94977386272025,11.3431047501248,25.0351557412125));
#59466=CARTESIAN_POINT('Ctrl Pts',(-5.90273483017515,11.357905868771,25.0280623795449));
#59467=CARTESIAN_POINT('Ctrl Pts',(-5.84730745884751,11.3750868173769,25.0198539645138));
#59468=CARTESIAN_POINT('Ctrl Pts',(-5.7980099252371,11.3903676862162,25.0125533365715));
#59469=CARTESIAN_POINT('Ctrl Pts',(-5.74207682856626,11.4075322478359,25.0043703278146));
#59470=CARTESIAN_POINT('Ctrl Pts',(-5.67943916884476,11.4264328448299,24.995387473731));
#59471=CARTESIAN_POINT('Ctrl Pts',(-5.62099151837065,11.4440691277269,24.9870055080244));
#59472=CARTESIAN_POINT('Ctrl Pts',(-5.55670627844591,11.4632175893215,24.9779269258027));
#59473=CARTESIAN_POINT('Ctrl Pts',(-5.48652739029172,11.4837185193206,24.9682369644011));
#59474=CARTESIAN_POINT('Ctrl Pts',(-5.4207988987062,11.5029193821497,24.95916149223));
#59475=CARTESIAN_POINT('Ctrl Pts',(-5.34990054958627,11.5233068590478,24.9495496451382));
#59476=CARTESIAN_POINT('Ctrl Pts',(-5.27378628704188,11.5447078507216,24.9394898133861));
#59477=CARTESIAN_POINT('Ctrl Pts',(-5.23117480484552,11.5566888900854,24.9338579603368));
#59478=CARTESIAN_POINT('Ctrl Pts',(-5.18692857181283,11.5689867928501,24.9280860442334));
#59479=CARTESIAN_POINT('Ctrl Pts',(-5.14103950690912,11.5815645387794,24.9221924626799));
#59480=CARTESIAN_POINT('Ctrl Pts',(-5.08921127757209,11.5957701518582,24.9155361079032));
#59481=CARTESIAN_POINT('Ctrl Pts',(-5.03528346648521,11.6103415053243,24.9087206071008));
#59482=CARTESIAN_POINT('Ctrl Pts',(-4.97924174038057,11.625228677746,24.901770743559));
#59483=CARTESIAN_POINT('Ctrl Pts',(-4.97223652461749,11.6270895742988,24.9009020106163));
#59484=CARTESIAN_POINT('Ctrl Pts',(-4.96519827893489,11.6289554054276,24.9000311780376));
#59485=CARTESIAN_POINT('Ctrl Pts',(-4.9581269707769,11.6308260577858,24.8991583011216));
#59486=CARTESIAN_POINT('Ctrl Pts',(-4.95105566261891,11.6326967101439,24.8982854242056));
#59487=CARTESIAN_POINT('Ctrl Pts',(-4.95002336600476,11.6329683362338,24.8981587538712));
#59488=CARTESIAN_POINT('Ctrl Pts',(-4.9467512886278,11.6338319100799,24.8977558964836));
#59489=CARTESIAN_POINT('Ctrl Pts',(-4.94020713387388,11.635559057772,24.8969501817086));
#59490=CARTESIAN_POINT('Ctrl Pts',(-4.93353444378895,11.6373165853176,24.8961304666749));
#59491=CARTESIAN_POINT('Ctrl Pts',(-4.92673308920624,11.639104084663,24.8952969595343));
#59492=CARTESIAN_POINT('Ctrl Pts',(-4.91313038004081,11.6426790833538,24.8936299452533));
#59493=CARTESIAN_POINT('Ctrl Pts',(-4.89901301288448,11.6463739691115,24.8919077622549));
#59494=CARTESIAN_POINT('Ctrl Pts',(-4.88438006285243,11.6501860013663,24.8901318453057));
#59495=CARTESIAN_POINT('Ctrl Pts',(-4.829421636142,11.6645032302801,24.8834618572798));
#59496=CARTESIAN_POINT('Ctrl Pts',(-4.76719038225856,11.6804723613988,24.8760340871454));
#59497=CARTESIAN_POINT('Ctrl Pts',(-4.69762431072455,11.6978935667144,24.8679498539363));
#59498=CARTESIAN_POINT('Ctrl Pts',(-4.69310115448302,11.6990262860389,24.8674242205479));
#59499=CARTESIAN_POINT('Ctrl Pts',(-4.68854698997108,11.700165127177,24.8668958197986));
#59500=CARTESIAN_POINT('Ctrl Pts',(-4.6839618001492,11.7013100279032,24.8663646829141));
#59501=CARTESIAN_POINT('Ctrl Pts',(-4.61785866763921,11.7178156748562,24.8587074618991));
#59502=CARTESIAN_POINT('Ctrl Pts',(-4.54530722999598,11.7355836340615,24.8504802696492));
#59503=CARTESIAN_POINT('Ctrl Pts',(-4.46624869967402,11.7544058575354,24.8417863906958));
#59504=CARTESIAN_POINT('Ctrl Pts',(-4.45548217444166,11.7569691475831,24.8406024214677));
#59505=CARTESIAN_POINT('Ctrl Pts',(-4.44459496772472,11.7595519176375,24.8394098294196));
#59506=CARTESIAN_POINT('Ctrl Pts',(-4.43358693104393,11.7621535716983,24.8382089068316));
#59507=CARTESIAN_POINT('Ctrl Pts',(-4.38766693898259,11.7730063638249,24.8331992618504));
#59508=CARTESIAN_POINT('Ctrl Pts',(-4.33964418259454,11.7841883687306,24.8280443854871));
#59509=CARTESIAN_POINT('Ctrl Pts',(-4.28950715573058,11.7956542720061,24.8227663700682));
#59510=CARTESIAN_POINT('Ctrl Pts',(-4.26443864229859,11.8013872236439,24.8201273623587));
#59511=CARTESIAN_POINT('Ctrl Pts',(-4.23884156124774,11.8071911491883,24.817457568396));
#59512=CARTESIAN_POINT('Ctrl Pts',(-4.21271443784642,11.8130598792849,24.8147599693042));
#59513=CARTESIAN_POINT('Ctrl Pts',(-4.19965087614576,11.8159942443332,24.8134111697584));
#59514=CARTESIAN_POINT('Ctrl Pts',(-4.18645480385771,11.8189448104674,24.8120554188158));
#59515=CARTESIAN_POINT('Ctrl Pts',(-4.17312603658067,11.821910791555,24.8106930950912));
#59516=CARTESIAN_POINT('Ctrl Pts',(-4.16646165294215,11.8233937820988,24.8100119332289));
#59517=CARTESIAN_POINT('Ctrl Pts',(-4.15976409555639,11.8248806263771,24.8093291281626));
#59518=CARTESIAN_POINT('Ctrl Pts',(-4.15303334128542,11.8263712242906,24.8086447280003));
#59519=CARTESIAN_POINT('Ctrl Pts',(-4.14630258701445,11.827861822204,24.807960327838));
#59520=CARTESIAN_POINT('Ctrl Pts',(-4.13831907940943,11.8296249476383,24.8071509729098));
#59521=CARTESIAN_POINT('Ctrl Pts',(-4.13274146466081,11.8308541782705,24.8065867905511));
#59522=CARTESIAN_POINT('Ctrl Pts',(-4.01469641459156,11.8568697060672,24.7946463934847));
#59523=CARTESIAN_POINT('Ctrl Pts',(-3.89907535590093,11.8813165391594,24.7834646730415));
#59524=CARTESIAN_POINT('Ctrl Pts',(-3.7859303789415,11.9043055522377,24.7729779011038));
#59525=CARTESIAN_POINT('Ctrl Pts',(-3.72800057606713,11.9160758405147,24.767608713293));
#59526=CARTESIAN_POINT('Ctrl Pts',(-3.67071985363078,11.9274648234898,24.7624213665553));
#59527=CARTESIAN_POINT('Ctrl Pts',(-3.61409520292724,11.9384921739262,24.7574053705903));
#59528=CARTESIAN_POINT('Ctrl Pts',(-3.53048496112061,11.9547748251218,24.7499989030834));
#59529=CARTESIAN_POINT('Ctrl Pts',(-3.44830456978397,11.9702644006063,24.7429681554761));
#59530=CARTESIAN_POINT('Ctrl Pts',(-3.36757331113062,11.9850131712523,24.7362852046435));
#59531=CARTESIAN_POINT('Ctrl Pts',(-3.32720768180394,11.9923875565753,24.7329437292272));
#59532=CARTESIAN_POINT('Ctrl Pts',(-3.28720433568016,11.999576745109,24.7296892123884));
#59533=CARTESIAN_POINT('Ctrl Pts',(-3.2475654491488,12.0065871586355,24.7265182809435));
#59534=CARTESIAN_POINT('Ctrl Pts',(-3.2124930980483,12.0127899485237,24.7237126516567));
#59535=CARTESIAN_POINT('Ctrl Pts',(-3.17911908413293,12.0186098553888,24.7210821798983));
#59536=CARTESIAN_POINT('Ctrl Pts',(-3.14369422059917,12.0246963262419,24.71833322792));
#59537=CARTESIAN_POINT('Ctrl Pts',(-3.13908178689044,12.0254888047592,24.7179753053339));
#59538=CARTESIAN_POINT('Ctrl Pts',(-3.13443458534099,12.0262857371774,24.7176154050858));
#59539=CARTESIAN_POINT('Ctrl Pts',(-3.12974434028523,12.0270884968926,24.7172529074598));
#59540=CARTESIAN_POINT('Ctrl Pts',(-2.96689344872027,12.0549612698035,24.7046665583719));
#59541=CARTESIAN_POINT('Ctrl Pts',(-2.80360512101477,12.0808137172381,24.6930389394681));
#59542=CARTESIAN_POINT('Ctrl Pts',(-2.63993695717176,12.1046081287205,24.6823718917912));
#59543=CARTESIAN_POINT('Ctrl Pts',(-2.55810287525025,12.1165053344617,24.6770383679527));
#59544=CARTESIAN_POINT('Ctrl Pts',(-2.47617400265685,12.1278883711933,24.6719448369763));
#59545=CARTESIAN_POINT('Ctrl Pts',(-2.39415787710936,12.1387531871149,24.6670912522717));
#59546=CARTESIAN_POINT('Ctrl Pts',(-2.35314981433562,12.1441855950756,24.6646644599195));
#59547=CARTESIAN_POINT('Ctrl Pts',(-2.31211993832262,12.1494884478784,24.6622976542637));
#59548=CARTESIAN_POINT('Ctrl Pts',(-2.27106919241763,12.1546612385219,24.6599908297852));
#59549=CARTESIAN_POINT('Ctrl Pts',(-2.23514978975077,12.159187430335,24.6579723583666));
#59550=CARTESIAN_POINT('Ctrl Pts',(-2.19921440857278,12.1636140433123,24.6559998100488));
#59551=CARTESIAN_POINT('Ctrl Pts',(-2.16326368103987,12.1679407375121,24.6540731808108));
#59552=CARTESIAN_POINT('Ctrl Pts',(-2.15812786282088,12.1685588366835,24.6537979480625));
#59553=CARTESIAN_POINT('Ctrl Pts',(-2.15095354419729,12.1694185453608,24.653415181293));
#59554=CARTESIAN_POINT('Ctrl Pts',(-2.14785528866281,12.1697889165532,24.6532502939249));
#59555=CARTESIAN_POINT('Ctrl Pts',(-2.07187460693358,12.1788717876642,24.6492066459772));
#59556=CARTESIAN_POINT('Ctrl Pts',(-1.98856296642531,12.1882955082351,24.6450211910771));
#59557=CARTESIAN_POINT('Ctrl Pts',(-1.89789453975114,12.1977714412891,24.6408247447902));
#59558=CARTESIAN_POINT('Ctrl Pts',(-1.80764463495196,12.2072036338106,24.6366476691336));
#59559=CARTESIAN_POINT('Ctrl Pts',(-1.71010570450369,12.2166876251517,24.6324597596906));
#59560=CARTESIAN_POINT('Ctrl Pts',(-1.60525227702567,12.2258907031711,24.6284092714104));
#59561=CARTESIAN_POINT('Ctrl Pts',(-1.54053826031317,12.2315707096246,24.6259093687123));
#59562=CARTESIAN_POINT('Ctrl Pts',(-1.47303802030777,12.2371427568608,24.6234621923046));
#59563=CARTESIAN_POINT('Ctrl Pts',(-1.40274556876306,12.2425193369782,24.6211060655178));
#59564=CARTESIAN_POINT('Ctrl Pts',(-1.28716646499202,12.2513598354625,24.617231979234));
#59565=CARTESIAN_POINT('Ctrl Pts',(-1.16403957039885,12.2596745372903,24.613603241472));
#59566=CARTESIAN_POINT('Ctrl Pts',(-1.0333545078798,12.2670275652562,24.6104067966571));
#59567=CARTESIAN_POINT('Ctrl Pts',(-0.995223826797064,12.2691729976335,
24.6094741528225));
#59568=CARTESIAN_POINT('Ctrl Pts',(-0.956449697259837,12.2712362342796,
24.6085784122977));
#59569=CARTESIAN_POINT('Ctrl Pts',(-0.917031861504277,12.273205652951,24.6077244509902));
#59570=CARTESIAN_POINT('Ctrl Pts',(-0.829774683487843,12.277565250892,24.6058340820138));
#59571=CARTESIAN_POINT('Ctrl Pts',(-0.739363747682051,12.2814654079063,
24.6041484487088));
#59572=CARTESIAN_POINT('Ctrl Pts',(-0.645800341501278,12.2847716669504,
24.6027230440238));
#59573=CARTESIAN_POINT('Ctrl Pts',(-0.599018638410892,12.2864247964724,
24.6020103416812));
#59574=CARTESIAN_POINT('Ctrl Pts',(-0.551448817581928,12.2879294374135,
24.6013626681618));
#59575=CARTESIAN_POINT('Ctrl Pts',(-0.503092201724354,12.2892678057657,
24.6007872112589));
#59576=CARTESIAN_POINT('Ctrl Pts',(-0.478913893795567,12.2899369899417,
24.6004994828075));
#59577=CARTESIAN_POINT('Ctrl Pts',(-0.454538887106797,12.2905646049275,
24.6002298064347));
#59578=CARTESIAN_POINT('Ctrl Pts',(-0.429967428839181,12.291148405519,24.5999790751891));
#59579=CARTESIAN_POINT('Ctrl Pts',(-0.417681699705374,12.2914403058147,
24.5998537095663));
#59580=CARTESIAN_POINT('Ctrl Pts',(-0.405346857677343,12.2917212524407,
24.5997330800844));
#59581=CARTESIAN_POINT('Ctrl Pts',(-0.39296293297194,12.291990960342,24.5996172994885));
#59582=CARTESIAN_POINT('Ctrl Pts',(-0.386770970619239,12.2921258142927,
24.5995594091905));
#59583=CARTESIAN_POINT('Ctrl Pts',(-0.380566737597225,12.2922578585576,
24.5995027311048));
#59584=CARTESIAN_POINT('Ctrl Pts',(-0.374350237930138,12.292387057274,24.5994472793692));
#59585=CARTESIAN_POINT('Ctrl Pts',(-0.36813373826305,12.2925162559905,24.5993918276337));
#59586=CARTESIAN_POINT('Ctrl Pts',(-0.359901584797702,12.2926822439143,
24.5993205939438));
#59587=CARTESIAN_POINT('Ctrl Pts',(-0.355663943074357,12.2927660808317,
24.5992846173454));
#59588=CARTESIAN_POINT('Ctrl Pts',(-0.236599314602959,12.2951216389641,
24.5982737861797));
#59589=CARTESIAN_POINT('Ctrl Pts',(-0.118032132646121,12.2962965905457,
24.5977734526346));
#59590=CARTESIAN_POINT('Ctrl Pts',(-6.22613072209788E-13,12.2963134975005,
24.5977650017124));
#59591=CARTESIAN_POINT('Ctrl Pts',(0.150825086921002,12.2963351017271,24.5977542028642));
#59592=CARTESIAN_POINT('Ctrl Pts',(0.300776517831056,12.2944653694354,24.5985470676585));
#59593=CARTESIAN_POINT('Ctrl Pts',(0.449775834204791,12.2907821275701,24.6001284130191));
#59594=CARTESIAN_POINT('Ctrl Pts',(0.582577156369656,12.287499297813,24.6015378473695));
#59595=CARTESIAN_POINT('Ctrl Pts',(0.714626434474783,12.2827727566975,24.6035750839994));
#59596=CARTESIAN_POINT('Ctrl Pts',(0.845889638816335,12.2766488845794,24.6062309232188));
#59597=CARTESIAN_POINT('Ctrl Pts',(0.911521240987111,12.2735869485203,24.6075588428285));
#59598=CARTESIAN_POINT('Ctrl Pts',(0.976956324341615,12.270175664687,24.6090413829613));
#59599=CARTESIAN_POINT('Ctrl Pts',(1.04219086193149,12.2664207372365,24.6106772326368));
#59600=CARTESIAN_POINT('Ctrl Pts',(1.07480813072642,12.2645432735113,24.6114951574745));
#59601=CARTESIAN_POINT('Ctrl Pts',(1.1073752630609,12.2625798981021,24.6123514080813));
#59602=CARTESIAN_POINT('Ctrl Pts',(1.13989176180785,12.2605313191956,24.613245811462));
#59603=CARTESIAN_POINT('Ctrl Pts',(1.15615001118132,12.2595070297423,24.6136930131524));
#59604=CARTESIAN_POINT('Ctrl Pts',(1.17239560215684,12.2584614393706,24.6141497529425));
#59605=CARTESIAN_POINT('Ctrl Pts',(1.18862847336251,12.2573946363024,24.6146160086764));
#59606=CARTESIAN_POINT('Ctrl Pts',(1.19674490896535,12.2568612347683,24.6148491365434));
#59607=CARTESIAN_POINT('Ctrl Pts',(1.20485816462567,12.2563225300575,24.6150846433906));
#59608=CARTESIAN_POINT('Ctrl Pts',(1.21296823271956,12.2557785331572,24.6153225264273));
#59609=CARTESIAN_POINT('Ctrl Pts',(1.2170232667665,12.2555065347071,24.6154414679457));
#59610=CARTESIAN_POINT('Ctrl Pts',(1.22107750392184,12.2552332132094,24.615561003511));
#59611=CARTESIAN_POINT('Ctrl Pts',(1.22513094323861,12.2549585701678,24.6156811327076));
#59612=CARTESIAN_POINT('Ctrl Pts',(1.22715766289699,12.254821248647,24.6157411973059));
#59613=CARTESIAN_POINT('Ctrl Pts',(1.22918418309573,12.2546835967402,24.6158014103119));
#59614=CARTESIAN_POINT('Ctrl Pts',(1.23121050371738,12.2545456146664,24.6158617716582));
#59615=CARTESIAN_POINT('Ctrl Pts',(1.23323682433902,12.2544076325926,24.6159221330045));
#59616=CARTESIAN_POINT('Ctrl Pts',(1.23664151732613,12.2541749789446,24.6160239184199));
#59617=CARTESIAN_POINT('Ctrl Pts',(1.23728886673302,12.2541306781364,24.6160433006635));
#59618=CARTESIAN_POINT('Ctrl Pts',(1.27899082428633,12.2512768400026,24.6172918960758));
#59619=CARTESIAN_POINT('Ctrl Pts',(1.329632197791,12.2476963537022,24.6188585341755));
#59620=CARTESIAN_POINT('Ctrl Pts',(1.3891670989942,12.243136392662,24.6208588486595));
#59621=CARTESIAN_POINT('Ctrl Pts',(1.45035959118757,12.238449471634,24.6229148565803));
#59622=CARTESIAN_POINT('Ctrl Pts',(1.52094773855851,12.23272755589,24.625429066743));
#59623=CARTESIAN_POINT('Ctrl Pts',(1.60088171223753,12.2256437990597,24.6285505871955));
#59624=CARTESIAN_POINT('Ctrl Pts',(1.68763810646718,12.2179554386303,24.6319385316014));
#59625=CARTESIAN_POINT('Ctrl Pts',(1.78540375455881,12.2086627108728,24.6360417972231));
#59626=CARTESIAN_POINT('Ctrl Pts',(1.89411494890352,12.1972887482862,24.641079110611));
#59627=CARTESIAN_POINT('Ctrl Pts',(1.97505001713986,12.1888208766599,24.6448293711544));
#59628=CARTESIAN_POINT('Ctrl Pts',(2.06205192313041,12.1791979832714,24.6490980028743));
#59629=CARTESIAN_POINT('Ctrl Pts',(2.15509437759377,12.1682070553229,24.6539839983181));
#59630=CARTESIAN_POINT('Ctrl Pts',(2.28390882697447,12.1529904497419,24.6607485104582));
#59631=CARTESIAN_POINT('Ctrl Pts',(2.42428242791866,12.1351252395717,24.6687090764788));
#59632=CARTESIAN_POINT('Ctrl Pts',(2.57602975677601,12.1138166138051,24.6782447930643));
#59633=CARTESIAN_POINT('Ctrl Pts',(2.68650546919738,12.0983034207228,24.6851870245432));
#59634=CARTESIAN_POINT('Ctrl Pts',(2.80300947452861,12.0809646523758,24.6929643411522));
#59635=CARTESIAN_POINT('Ctrl Pts',(2.92547022396319,12.0615113539224,24.7017176516046));
#59636=CARTESIAN_POINT('Ctrl Pts',(3.04051821297009,12.0432355971843,24.7099411090744));
#59637=CARTESIAN_POINT('Ctrl Pts',(3.16081857299903,12.0230822496991,24.71903140512));
#59638=CARTESIAN_POINT('Ctrl Pts',(3.28628241049585,12.0007593860875,24.7291338183826));
#59639=CARTESIAN_POINT('Ctrl Pts',(3.31931172104303,11.9948827222676,24.7317933555973));
#59640=CARTESIAN_POINT('Ctrl Pts',(3.35269888418365,11.98885595359,24.7345229380971));
#59641=CARTESIAN_POINT('Ctrl Pts',(3.38644227805871,11.9826743497142,24.7373249864784));
#59642=CARTESIAN_POINT('Ctrl Pts',(3.46740213813978,11.9678429493306,24.7440478859512));
#59643=CARTESIAN_POINT('Ctrl Pts',(3.55041195750174,11.952116979161,24.7511894115549));
#59644=CARTESIAN_POINT('Ctrl Pts',(3.6354448591658,11.9354211828935,24.7587882878275));
#59645=CARTESIAN_POINT('Ctrl Pts',(3.67796130999782,11.9270732847597,24.7625877259637));
#59646=CARTESIAN_POINT('Ctrl Pts',(3.72098353143885,11.9184829356168,24.7665015135186));
#59647=CARTESIAN_POINT('Ctrl Pts',(3.7645077837846,11.9096404763391,24.7705347060947));
#59648=CARTESIAN_POINT('Ctrl Pts',(3.78626990995747,11.9052192467003,24.7725513023827));
#59649=CARTESIAN_POINT('Ctrl Pts',(3.80815754385888,11.900734989943,24.7745977508124));
#59650=CARTESIAN_POINT('Ctrl Pts',(3.8301702057321,11.8961864945343,24.7766746921987));
#59651=CARTESIAN_POINT('Ctrl Pts',(3.84117653666871,11.8939122468299,24.7777131628918));
#59652=CARTESIAN_POINT('Ctrl Pts',(3.85221412459836,11.8916219394916,24.7787592568861));
#59653=CARTESIAN_POINT('Ctrl Pts',(3.86328290819419,11.889315420327,24.7798130551019));
#59654=CARTESIAN_POINT('Ctrl Pts',(3.86881729999211,11.8881621607447,24.7803399542098));
#59655=CARTESIAN_POINT('Ctrl Pts',(3.87435949070658,11.8870048482077,24.7808687793772));
#59656=CARTESIAN_POINT('Ctrl Pts',(3.87990947258041,11.8858434636443,24.7813995407716));
#59657=CARTESIAN_POINT('Ctrl Pts',(3.88545945445423,11.8846820790809,24.7819303021661));
#59658=CARTESIAN_POINT('Ctrl Pts',(3.89320613467674,11.8830566448808,24.7826732727751));
#59659=CARTESIAN_POINT('Ctrl Pts',(3.89658278389481,11.8823470747937,24.7829976438288));
#59660=CARTESIAN_POINT('Ctrl Pts',(4.05478128241934,11.8491031945051,24.7981946661861));
#59661=CARTESIAN_POINT('Ctrl Pts',(4.20725187154444,11.8150833635526,24.813808149887));
#59662=CARTESIAN_POINT('Ctrl Pts',(4.35406646400287,11.7807204817787,24.829644840975));
#59663=CARTESIAN_POINT('Ctrl Pts',(4.49799162540886,11.7470338895751,24.8451698530518));
#59664=CARTESIAN_POINT('Ctrl Pts',(4.63648122865026,11.7130177567802,24.8609093236835));
#59665=CARTESIAN_POINT('Ctrl Pts',(4.7696030235706,11.6790336138896,24.876700411352));
#59666=CARTESIAN_POINT('Ctrl Pts',(4.9002562079937,11.6456796729275,24.8921986690988));
#59667=CARTESIAN_POINT('Ctrl Pts',(5.02573881948381,11.6123566061781,24.9077466533623));
#59668=CARTESIAN_POINT('Ctrl Pts',(5.14611490828662,11.5793596951519,24.9232094066191));
#59669=CARTESIAN_POINT('Ctrl Pts',(5.26571077368129,11.5465766551913,24.938571937297));
#59670=CARTESIAN_POINT('Ctrl Pts',(5.380266098206,11.5141156414518,24.9538503395685));
#59671=CARTESIAN_POINT('Ctrl Pts',(5.48984369472711,11.4822186912238,24.9689311707428));
#59672=CARTESIAN_POINT('Ctrl Pts',(5.59891528315245,11.4504690349279,24.9839423615626));
#59673=CARTESIAN_POINT('Ctrl Pts',(5.70305500979413,11.4192782828121,24.9987578168915));
#59674=CARTESIAN_POINT('Ctrl Pts',(5.80232482135773,11.3888369471314,25.0132843278572));
#59675=CARTESIAN_POINT('Ctrl Pts',(5.86641621843993,11.3691831601231,25.0226630540566));
#59676=CARTESIAN_POINT('Ctrl Pts',(5.92847766024371,11.3498407748922,25.0319217160901));
#59677=CARTESIAN_POINT('Ctrl Pts',(5.98852581792974,11.3308502649382,25.0410393365944));
#59678=CARTESIAN_POINT('Origin',(-5.98852353411075,-4.75229019515312,-11.473043446859));
#59679=CARTESIAN_POINT('Ctrl Pts',(-6.39567215186926,11.8440001009078,24.265774917167));
#59680=CARTESIAN_POINT('Ctrl Pts',(-6.35564925265182,11.85659016276,24.2594187697523));
#59681=CARTESIAN_POINT('Ctrl Pts',(-5.98524772032908,11.9719915346492,24.201263545813));
#59682=CARTESIAN_POINT('Ctrl Pts',(-5.25616196134156,12.1789688183688,24.0987560784236));
#59683=CARTESIAN_POINT('Ctrl Pts',(-4.17575456655968,12.4300259295094,23.9769539472116));
#59684=CARTESIAN_POINT('Ctrl Pts',(-3.01936369311187,12.6350416910811,23.8792984905102));
#59685=CARTESIAN_POINT('Ctrl Pts',(-1.83578568452794,12.7756187374379,23.8136687753784));
#59686=CARTESIAN_POINT('Ctrl Pts',(-0.697928666899182,12.8441379077251,
23.7825584029238));
#59687=CARTESIAN_POINT('Ctrl Pts',(0.331398824709615,12.8512035850883,23.7794557664846));
#59688=CARTESIAN_POINT('Ctrl Pts',(1.24579451141582,12.8144580444262,23.7959563368043));
#59689=CARTESIAN_POINT('Ctrl Pts',(2.07028251458803,12.7465829770363,23.8272311099001));
#59690=CARTESIAN_POINT('Ctrl Pts',(2.81704923736738,12.6564423117063,23.8693916417645));
#59691=CARTESIAN_POINT('Ctrl Pts',(3.49016613607229,12.5517067197984,23.9189795923457));
#59692=CARTESIAN_POINT('Ctrl Pts',(4.0949553302766,12.4387818440348,23.9729931464066));
#59693=CARTESIAN_POINT('Ctrl Pts',(4.65003900301249,12.3195562907933,24.0305528564122));
#59694=CARTESIAN_POINT('Ctrl Pts',(5.180490898606,12.1916432061588,24.092883824788));
#59695=CARTESIAN_POINT('Ctrl Pts',(5.70541362588262,12.0514986413341,24.1618778453152));
#59696=CARTESIAN_POINT('Ctrl Pts',(6.10977777422788,11.9329745555922,24.2209465726705));
#59697=CARTESIAN_POINT('Ctrl Pts',(6.34031405438408,11.8614134775702,24.2569833946951));
#59698=CARTESIAN_POINT('Ctrl Pts',(6.39541676810711,11.8440802193301,24.2657356932574));
#59699=CARTESIAN_POINT('Ctrl Pts',(-6.33011224179481,11.8152698388501,24.6389123673273));
#59700=CARTESIAN_POINT('Ctrl Pts',(-6.29056405060346,11.8278254058075,24.6326369136256));
#59701=CARTESIAN_POINT('Ctrl Pts',(-5.92452851936487,11.9429205323235,24.5752163287446));
#59702=CARTESIAN_POINT('Ctrl Pts',(-5.20357136152678,12.1495103384449,24.4739420826815));
#59703=CARTESIAN_POINT('Ctrl Pts',(-4.13460886818725,12.4003002415022,24.3535497596591));
#59704=CARTESIAN_POINT('Ctrl Pts',(-2.9900914803837,12.6052169620649,24.2569987045062));
#59705=CARTESIAN_POINT('Ctrl Pts',(-1.81832885962656,12.745786877442,24.1920958956842));
#59706=CARTESIAN_POINT('Ctrl Pts',(-0.691524096675534,12.8143243855958,
24.1613192188688));
#59707=CARTESIAN_POINT('Ctrl Pts',(0.32839667136552,12.8213935876436,24.1582483778528));
#59708=CARTESIAN_POINT('Ctrl Pts',(1.23407752119641,12.7846352465759,24.1745745145462));
#59709=CARTESIAN_POINT('Ctrl Pts',(2.05048413456686,12.7167522286949,24.2055078846837));
#59710=CARTESIAN_POINT('Ctrl Pts',(2.78978431718345,12.6266205777662,24.2472006090323));
#59711=CARTESIAN_POINT('Ctrl Pts',(3.45605929775469,12.5219212851974,24.2962312061184));
#59712=CARTESIAN_POINT('Ctrl Pts',(4.05460643170645,12.4090658151592,24.3496307103682));
#59713=CARTESIAN_POINT('Ctrl Pts',(4.60386797000098,12.2899482805146,24.4065282055716));
#59714=CARTESIAN_POINT('Ctrl Pts',(5.12864846123703,12.1621933780158,24.4681316577684));
#59715=CARTESIAN_POINT('Ctrl Pts',(5.64781590092389,12.0222780918086,24.5363045861396));
#59716=CARTESIAN_POINT('Ctrl Pts',(6.04758532775613,11.9040090244283,24.5946499786562));
#59717=CARTESIAN_POINT('Ctrl Pts',(6.27541087928418,11.8326354722664,24.6302324927227));
#59718=CARTESIAN_POINT('Ctrl Pts',(6.32985956424417,11.8153497944645,24.6388735577287));
#59719=CARTESIAN_POINT('Ctrl Pts',(-6.21909721196556,11.6041667995241,24.9345589552791));
#59720=CARTESIAN_POINT('Ctrl Pts',(-6.18025379385954,11.6165919593275,24.9284549741306));
#59721=CARTESIAN_POINT('Ctrl Pts',(-5.82072765592081,11.7304974169554,24.8726034547386));
#59722=CARTESIAN_POINT('Ctrl Pts',(-5.11236921789459,11.9350420954516,24.7741000987782));
#59723=CARTESIAN_POINT('Ctrl Pts',(-4.06203918887106,12.1834236616043,24.6570690059104));
#59724=CARTESIAN_POINT('Ctrl Pts',(-2.93761905916863,12.3863982267026,24.5632789748405));
#59725=CARTESIAN_POINT('Ctrl Pts',(-1.78654249655019,12.5256445065243,24.5002681039227));
#59726=CARTESIAN_POINT('Ctrl Pts',(-0.679607685364788,12.5935428444393,
24.4703931528392));
#59727=CARTESIAN_POINT('Ctrl Pts',(0.322770033085937,12.6005472441068,24.4674113481417));
#59728=CARTESIAN_POINT('Ctrl Pts',(1.21259297328069,12.5641298285676,24.483260547359));
#59729=CARTESIAN_POINT('Ctrl Pts',(2.01460081624777,12.4968834095009,24.5132884775637));
#59730=CARTESIAN_POINT('Ctrl Pts',(2.74085389058468,12.4076008364804,24.5537690843015));
#59731=CARTESIAN_POINT('Ctrl Pts',(3.39540207428237,12.3038918865634,24.6013888811208));
#59732=CARTESIAN_POINT('Ctrl Pts',(3.98345489728963,12.1921091082277,24.6532698675774));
#59733=CARTESIAN_POINT('Ctrl Pts',(4.52311935809495,12.0741314785244,24.7085682944355));
#59734=CARTESIAN_POINT('Ctrl Pts',(5.03874789287724,11.9476113810817,24.7684595170186));
#59735=CARTESIAN_POINT('Ctrl Pts',(5.54885110815234,11.8090692255007,24.8347559275283));
#59736=CARTESIAN_POINT('Ctrl Pts',(5.94159338885824,11.6919892200842,24.8915060754566));
#59737=CARTESIAN_POINT('Ctrl Pts',(6.16537079301529,11.6213520344321,24.9261162878907));
#59738=CARTESIAN_POINT('Ctrl Pts',(6.21884874455077,11.6042459796829,24.9345211260386));
#59739=CARTESIAN_POINT('Ctrl Pts',(-6.09442747551374,11.2712687731348,25.068247785561));
#59740=CARTESIAN_POINT('Ctrl Pts',(-6.05631707756792,11.2835050162748,25.0623569142849));
#59741=CARTESIAN_POINT('Ctrl Pts',(-5.70357968237373,11.3956786059711,25.0084592116254));
#59742=CARTESIAN_POINT('Ctrl Pts',(-5.00868192961402,11.5971072515952,24.9134702394146));
#59743=CARTESIAN_POINT('Ctrl Pts',(-3.9788351244146,11.8416305120833,24.8007883278658));
#59744=CARTESIAN_POINT('Ctrl Pts',(-2.87697914274819,12.0413773094681,24.7106244572076));
#59745=CARTESIAN_POINT('Ctrl Pts',(-1.74953331073714,12.1783634704876,24.6501281720072));
#59746=CARTESIAN_POINT('Ctrl Pts',(-0.665593611714366,12.2451486628473,
24.6214644543181));
#59747=CARTESIAN_POINT('Ctrl Pts',(0.316131026122826,12.2520385424126,24.6186033990537));
#59748=CARTESIAN_POINT('Ctrl Pts',(1.18749622986108,12.2162178808641,24.6338098959915));
#59749=CARTESIAN_POINT('Ctrl Pts',(1.97291294062881,12.1500698270089,24.6626279294911));
#59750=CARTESIAN_POINT('Ctrl Pts',(2.68427596727038,12.0622326265172,24.7014995980027));
#59751=CARTESIAN_POINT('Ctrl Pts',(3.32557172596527,11.9601837655491,24.747259581196));
#59752=CARTESIAN_POINT('Ctrl Pts',(3.90188404781945,11.8501690615632,24.7971528788433));
#59753=CARTESIAN_POINT('Ctrl Pts',(4.43092541213141,11.7340360652914,24.8503737539427));
#59754=CARTESIAN_POINT('Ctrl Pts',(4.93654273176015,11.6094730471387,24.9080588205053));
#59755=CARTESIAN_POINT('Ctrl Pts',(5.43686879684977,11.4730538901245,24.9719611389093));
#59756=CARTESIAN_POINT('Ctrl Pts',(5.8221639465597,11.3577558829121,25.0267013366178));
#59757=CARTESIAN_POINT('Ctrl Pts',(6.04171502508226,11.2881926952705,25.0600999046611));
#59758=CARTESIAN_POINT('Ctrl Pts',(6.09418351640657,11.271346787654,25.0682112217091));
#59759=CARTESIAN_POINT('',(6.27159454904393,11.8794923467406,24.2690137147172));
#59760=CARTESIAN_POINT('Origin',(5.999999949012,10.9277802669415,24.1259420051707));
#59761=CARTESIAN_POINT('',(-6.27159362679375,11.8794975540956,24.2690120913865));
#59762=CARTESIAN_POINT('Ctrl Pts',(-6.27159387327999,11.8794984953294,24.2690123753742));
#59763=CARTESIAN_POINT('Ctrl Pts',(-6.13239665975347,11.9224692155082,24.2474082746545));
#59764=CARTESIAN_POINT('Ctrl Pts',(-5.98564494831062,11.9663158668838,24.2255025468638));
#59765=CARTESIAN_POINT('Ctrl Pts',(-5.83132868240695,12.0105538899393,24.203534985663));
#59766=CARTESIAN_POINT('Ctrl Pts',(-5.67907415991493,12.0542008706181,24.1818609221977));
#59767=CARTESIAN_POINT('Ctrl Pts',(-5.51945557022787,12.0982288673079,24.1601268955012));
#59768=CARTESIAN_POINT('Ctrl Pts',(-5.35247255846345,12.1421228213731,24.1385690083634));
#59769=CARTESIAN_POINT('Ctrl Pts',(-5.32566531741069,12.1491695011218,24.1351081324875));
#59770=CARTESIAN_POINT('Ctrl Pts',(-5.29866830053705,12.1562126203553,24.1316518043049));
#59771=CARTESIAN_POINT('Ctrl Pts',(-5.27148153698936,12.1632499256716,24.128201008766));
#59772=CARTESIAN_POINT('Ctrl Pts',(-5.14595062003312,12.1957436569577,24.1122674634778));
#59773=CARTESIAN_POINT('Ctrl Pts',(-5.01637391730844,12.2281146709243,24.0964515384637));
#59774=CARTESIAN_POINT('Ctrl Pts',(-4.88275740018152,12.2601325340667,24.0808623975426));
#59775=CARTESIAN_POINT('Ctrl Pts',(-4.71106411325276,12.3012745446621,24.0608308108594));
#59776=CARTESIAN_POINT('Ctrl Pts',(-4.53269557213984,12.3418362253296,24.0411729460729));
#59777=CARTESIAN_POINT('Ctrl Pts',(-4.34764559027276,12.3812950570725,24.0221340647503));
#59778=CARTESIAN_POINT('Ctrl Pts',(-4.2958379438806,12.3923421762419,24.016803831149));
#59779=CARTESIAN_POINT('Ctrl Pts',(-4.2435067021697,12.4033025668906,24.0115221856858));
#59780=CARTESIAN_POINT('Ctrl Pts',(-4.19065197808048,12.4141640869762,24.0062946755803));
#59781=CARTESIAN_POINT('Ctrl Pts',(-4.14337959060077,12.4238784501661,24.0016192773539));
#59782=CARTESIAN_POINT('Ctrl Pts',(-4.09568845748379,12.4335137197591,23.9969871831794));
#59783=CARTESIAN_POINT('Ctrl Pts',(-4.04757900720712,12.4430611393021,23.9924025369345));
#59784=CARTESIAN_POINT('Ctrl Pts',(-3.90056248959711,12.4722368701677,23.9783924262074));
#59785=CARTESIAN_POINT('Ctrl Pts',(-3.74963598878708,12.5005941082547,23.9648249569629));
#59786=CARTESIAN_POINT('Ctrl Pts',(-3.59479968040675,12.5278747688691,23.951821468078));
#59787=CARTESIAN_POINT('Ctrl Pts',(-3.51738152621659,12.5415150991762,23.9453197236355));
#59788=CARTESIAN_POINT('Ctrl Pts',(-3.43898591152213,12.5548860349274,23.93895906991));
#59789=CARTESIAN_POINT('Ctrl Pts',(-3.35961280896348,12.5679537407706,23.9327552496512));
#59790=CARTESIAN_POINT('Ctrl Pts',(-3.31992625768416,12.5744875936921,23.9296533395218));
#59791=CARTESIAN_POINT('Ctrl Pts',(-3.2799953320476,12.5809456233232,23.9265906359475));
#59792=CARTESIAN_POINT('Ctrl Pts',(-3.23982002808293,12.5873234942267,23.9235691515302));
#59793=CARTESIAN_POINT('Ctrl Pts',(-3.2197323761006,12.5905124296784,23.9220584093215));
#59794=CARTESIAN_POINT('Ctrl Pts',(-3.19958362938644,12.5936813244136,23.9205579717845));
#59795=CARTESIAN_POINT('Ctrl Pts',(-3.17937378695259,12.5968296299603,23.9190680913502));
#59796=CARTESIAN_POINT('Ctrl Pts',(-3.16169017482297,12.5995843973137,23.9177644459701));
#59797=CARTESIAN_POINT('Ctrl Pts',(-3.14395978627424,12.6023234010082,23.9164688833649));
#59798=CARTESIAN_POINT('Ctrl Pts',(-3.12618262055138,12.6050462707541,23.9151815734085));
#59799=CARTESIAN_POINT('Ctrl Pts',(-3.12364302544811,12.6054352521464,23.9149976719862));
#59800=CARTESIAN_POINT('Ctrl Pts',(-3.11986205084656,12.6060134313777,23.9147243474001));
#59801=CARTESIAN_POINT('Ctrl Pts',(-3.11856097133547,12.6062122260373,23.9146303749287));
#59802=CARTESIAN_POINT('Ctrl Pts',(-3.09161078795331,12.6103300009199,23.9126838564297));
#59803=CARTESIAN_POINT('Ctrl Pts',(-3.06343524023067,12.6145814696381,23.9106763719954));
#59804=CARTESIAN_POINT('Ctrl Pts',(-3.03403435500432,12.6189513764305,23.9086151433588));
#59805=CARTESIAN_POINT('Ctrl Pts',(-2.9619677253846,12.6296627700452,23.9035627172304));
#59806=CARTESIAN_POINT('Ctrl Pts',(-2.88253900653253,12.6410890424655,23.898185873917));
#59807=CARTESIAN_POINT('Ctrl Pts',(-2.79574783276679,12.6529730518689,23.892606171807));
#59808=CARTESIAN_POINT('Ctrl Pts',(-2.70928691593848,12.6648118403543,23.8870477015258));
#59809=CARTESIAN_POINT('Ctrl Pts',(-2.61551922198365,12.6771049175497,23.8812879491854));
#59810=CARTESIAN_POINT('Ctrl Pts',(-2.51444548334207,12.689550941705,23.8754684237424));
#59811=CARTESIAN_POINT('Ctrl Pts',(-2.50258801369576,12.6910110475211,23.8747857058848));
#59812=CARTESIAN_POINT('Ctrl Pts',(-2.49062999607805,12.6924732044915,23.8741021892436));
#59813=CARTESIAN_POINT('Ctrl Pts',(-2.47857143521673,12.6939368830162,23.8734181212848));
#59814=CARTESIAN_POINT('Ctrl Pts',(-2.37688557180676,12.7062796008792,23.8676496019884));
#59815=CARTESIAN_POINT('Ctrl Pts',(-2.26804971895943,12.7187343238039,23.8618405702272));
#59816=CARTESIAN_POINT('Ctrl Pts',(-2.1520626700025,12.7309579651534,23.8561524935622));
#59817=CARTESIAN_POINT('Ctrl Pts',(-2.11969727196408,12.7343688892291,23.8545652744115));
#59818=CARTESIAN_POINT('Ctrl Pts',(-2.08677509095584,12.7377615371318,23.8529875939479));
#59819=CARTESIAN_POINT('Ctrl Pts',(-2.05329622092775,12.7411277927086,23.8514232396551));
#59820=CARTESIAN_POINT('Ctrl Pts',(-1.97656810089333,12.7488427024934,23.8478379942793));
#59821=CARTESIAN_POINT('Ctrl Pts',(-1.8969155054141,12.7564195734445,23.8443225602372));
#59822=CARTESIAN_POINT('Ctrl Pts',(-1.81433838927152,12.7637550206789,23.8409252157065));
#59823=CARTESIAN_POINT('Ctrl Pts',(-1.81240102804,12.7639271193396,23.8408455098038));
#59824=CARTESIAN_POINT('Ctrl Pts',(-1.81046205708854,12.7640990847574,23.8407658688772));
#59825=CARTESIAN_POINT('Ctrl Pts',(-1.80852147639801,12.7642709155407,23.8406862936122));
#59826=CARTESIAN_POINT('Ctrl Pts',(-1.76910488671214,12.7677610994404,23.83906998073));
#59827=CARTESIAN_POINT('Ctrl Pts',(-1.72902415885956,12.7711957707857,23.8374807465779));
#59828=CARTESIAN_POINT('Ctrl Pts',(-1.6882793161297,12.7745632609372,23.8359241922724));
#59829=CARTESIAN_POINT('Ctrl Pts',(-1.66690390775258,12.7763299011392,23.8351075985218));
#59830=CARTESIAN_POINT('Ctrl Pts',(-1.64534571912912,12.7780780455687,23.8342999980866));
#59831=CARTESIAN_POINT('Ctrl Pts',(-1.62360475111848,12.7798059673452,23.8335022084597));
#59832=CARTESIAN_POINT('Ctrl Pts',(-1.61273426711316,12.7806699282335,23.8331033136463));
#59833=CARTESIAN_POINT('Ctrl Pts',(-1.60181808822608,12.7815288330184,23.8327068714887));
#59834=CARTESIAN_POINT('Ctrl Pts',(-1.59085621455979,12.7823824630006,23.8323129855334));
#59835=CARTESIAN_POINT('Ctrl Pts',(-1.58537527772664,12.7828092779917,23.8321160425557));
#59836=CARTESIAN_POINT('Ctrl Pts',(-1.57988291719653,12.7832347742544,23.8319197386257));
#59837=CARTESIAN_POINT('Ctrl Pts',(-1.5743791329824,12.7836589242724,23.8317240867766));
#59838=CARTESIAN_POINT('Ctrl Pts',(-1.56887534876828,12.7840830742904,23.8315284349275));
#59839=CARTESIAN_POINT('Ctrl Pts',(-1.56205962342448,12.7846050482238,23.831287704659));
#59840=CARTESIAN_POINT('Ctrl Pts',(-1.55783350929622,12.7849273079608,23.8311391005259));
#59841=CARTESIAN_POINT('Ctrl Pts',(-1.33210029545101,12.8021404555285,23.8232015750512));
#59842=CARTESIAN_POINT('Ctrl Pts',(-1.11005370632018,12.8153351626569,23.817122034248));
#59843=CARTESIAN_POINT('Ctrl Pts',(-0.891696800345942,12.8248709230765,
23.8127291041508));
#59844=CARTESIAN_POINT('Ctrl Pts',(-0.84842062124671,12.8267608164779,23.811858468854));
#59845=CARTESIAN_POINT('Ctrl Pts',(-0.805289264854227,12.8285068913263,
23.8110541618022));
#59846=CARTESIAN_POINT('Ctrl Pts',(-0.762302602899293,12.8301118023318,
23.8103149645275));
#59847=CARTESIAN_POINT('Ctrl Pts',(-0.724718063253752,12.8315150246005,
23.8096686619766));
#59848=CARTESIAN_POINT('Ctrl Pts',(-0.687244120817588,12.8328103362796,
23.8090721006341));
#59849=CARTESIAN_POINT('Ctrl Pts',(-0.649880973381661,12.8339994885111,
23.8085243488097));
#59850=CARTESIAN_POINT('Ctrl Pts',(-0.558068160819892,12.8369216034407,
23.8071783531151));
#59851=CARTESIAN_POINT('Ctrl Pts',(-0.466924415806544,12.8392027555537,
23.8061270509237));
#59852=CARTESIAN_POINT('Ctrl Pts',(-0.376448972902625,12.8408704266499,
23.8053581698283));
#59853=CARTESIAN_POINT('Ctrl Pts',(-0.312801798465681,12.8420435908783,
23.8048172815206));
#59854=CARTESIAN_POINT('Ctrl Pts',(-0.249485511111982,12.8429131416853,
23.8044160900822));
#59855=CARTESIAN_POINT('Ctrl Pts',(-0.18650011116102,12.8434883988289,23.8041502792515));
#59856=CARTESIAN_POINT('Ctrl Pts',(-0.155007411185538,12.8437760274007,
23.8040173738361));
#59857=CARTESIAN_POINT('Ctrl Pts',(-0.123597432937689,12.8439900795162,
23.8039183132638));
#59858=CARTESIAN_POINT('Ctrl Pts',(-0.0922701760386044,12.8441317020175,
23.8038525590397));
#59859=CARTESIAN_POINT('Ctrl Pts',(-0.0647193034850948,12.8442562524528,
23.8037947312428));
#59860=CARTESIAN_POINT('Ctrl Pts',(-0.0383382064328693,12.8443236938424,
23.8037631762405));
#59861=CARTESIAN_POINT('Ctrl Pts',(-0.0102093966394934,12.8443378683841,
23.8037560877189));
#59862=CARTESIAN_POINT('Ctrl Pts',(-0.00635379472499661,12.8443398112815,
23.8037551160988));
#59863=CARTESIAN_POINT('Ctrl Pts',(-0.0024653565932188,12.844340680764,
23.803754636878));
#59864=CARTESIAN_POINT('Ctrl Pts',(0.00146343106551837,12.8443404157949,
23.8037546773412));
#59865=CARTESIAN_POINT('Ctrl Pts',(0.123994138919106,12.8443321519592,23.8037559393069));
#59866=CARTESIAN_POINT('Ctrl Pts',(0.24652145032575,12.8432200851129,23.8042791685664));
#59867=CARTESIAN_POINT('Ctrl Pts',(0.36905046775366,12.8410042079906,23.8053127231307));
#59868=CARTESIAN_POINT('Ctrl Pts',(0.644865199825655,12.8360162339772,23.8076392705984));
#59869=CARTESIAN_POINT('Ctrl Pts',(0.920688389422045,12.8254382930282,23.8125501318452));
#59870=CARTESIAN_POINT('Ctrl Pts',(1.19650944973774,12.8092731224474,23.8200734126678));
#59871=CARTESIAN_POINT('Ctrl Pts',(1.22210575983819,12.8077729878364,23.820771576284));
#59872=CARTESIAN_POINT('Ctrl Pts',(1.24770205338369,12.8062247032809,23.8214922543273));
#59873=CARTESIAN_POINT('Ctrl Pts',(1.27329832267905,12.8046282506351,23.8222354795427));
#59874=CARTESIAN_POINT('Ctrl Pts',(1.37081820380044,12.798545884864,23.8250671123017));
#59875=CARTESIAN_POINT('Ctrl Pts',(1.46833773422664,12.7917643882597,23.8282260014275));
#59876=CARTESIAN_POINT('Ctrl Pts',(1.56585686708111,12.7842847837547,23.8317101403452));
#59877=CARTESIAN_POINT('Ctrl Pts',(1.7401743530888,12.7709148345407,23.8379381114033));
#59878=CARTESIAN_POINT('Ctrl Pts',(1.91449222409226,12.7553144041715,23.8452066434151));
#59879=CARTESIAN_POINT('Ctrl Pts',(2.08880964225459,12.737482741405,23.8535154632649));
#59880=CARTESIAN_POINT('Ctrl Pts',(2.17522432420784,12.7286430196898,23.8576344092216));
#59881=CARTESIAN_POINT('Ctrl Pts',(2.26163887766306,12.7192548608822,23.8620090644269));
#59882=CARTESIAN_POINT('Ctrl Pts',(2.3480535937233,12.7093187481637,23.8666392624854));
#59883=CARTESIAN_POINT('Ctrl Pts',(2.47841969523524,12.6943290295331,23.8736244254025));
#59884=CARTESIAN_POINT('Ctrl Pts',(2.60878583587792,12.6780923252995,23.8811913884638));
#59885=CARTESIAN_POINT('Ctrl Pts',(2.73915198832477,12.6606086880375,23.8893399954516));
#59886=CARTESIAN_POINT('Ctrl Pts',(2.77253967456891,12.6561310058757,23.8914269108689));
#59887=CARTESIAN_POINT('Ctrl Pts',(2.80592736751217,12.6515715264161,23.8935519669626));
#59888=CARTESIAN_POINT('Ctrl Pts',(2.83931504872826,12.6469302299745,23.8957151760613));
#59889=CARTESIAN_POINT('Ctrl Pts',(2.87111043391928,12.6425102821742,23.8977752192879));
#59890=CARTESIAN_POINT('Ctrl Pts',(2.90290580844884,12.6380161351086,23.8998698632239));
#59891=CARTESIAN_POINT('Ctrl Pts',(2.93470118833342,12.6334478142511,23.901999091622));
#59892=CARTESIAN_POINT('Ctrl Pts',(2.98358847997979,12.626423748651,23.9052729071906));
#59893=CARTESIAN_POINT('Ctrl Pts',(3.03247576815835,12.6192243312319,23.9086285033686));
#59894=CARTESIAN_POINT('Ctrl Pts',(3.08136305876389,12.6118496254351,23.9120658773373));
#59895=CARTESIAN_POINT('Ctrl Pts',(3.09765882229907,12.6093913901695,23.9132116686601));
#59896=CARTESIAN_POINT('Ctrl Pts',(3.11203761249439,12.6072074380347,23.9142296219463));
#59897=CARTESIAN_POINT('Ctrl Pts',(3.13025035019709,12.6044164907937,23.9155305102362));
#59898=CARTESIAN_POINT('Ctrl Pts',(3.25876627310765,12.5847225180193,23.924710066979));
#59899=CARTESIAN_POINT('Ctrl Pts',(3.38586269051035,12.56402720794,23.934421740979));
#59900=CARTESIAN_POINT('Ctrl Pts',(3.51152584085004,12.542411839432,23.9446264834151));
#59901=CARTESIAN_POINT('Ctrl Pts',(3.71378615759454,12.5076209618424,23.9610514610783));
#59902=CARTESIAN_POINT('Ctrl Pts',(3.91233263338801,12.4704476520642,23.9787535291653));
#59903=CARTESIAN_POINT('Ctrl Pts',(4.10713150515215,12.4312229146291,23.9975737301052));
#59904=CARTESIAN_POINT('Ctrl Pts',(4.29248338111171,12.3939004260449,24.015481223709));
#59905=CARTESIAN_POINT('Ctrl Pts',(4.4744426089921,12.3547205225641,24.0344011133741));
#59906=CARTESIAN_POINT('Ctrl Pts',(4.65299936796426,12.3139554246983,24.0542036567935));
#59907=CARTESIAN_POINT('Ctrl Pts',(4.83064040150767,12.2733993899727,24.0739046431917));
#59908=CARTESIAN_POINT('Ctrl Pts',(5.0049139245582,12.2312743461914,24.0944793585985));
#59909=CARTESIAN_POINT('Ctrl Pts',(5.17582589534808,12.1878340421094,24.1158100264904));
#59910=CARTESIAN_POINT('Ctrl Pts',(5.35319905371138,12.1427515127834,24.1379470828739));
#59911=CARTESIAN_POINT('Ctrl Pts',(5.52695177479932,12.0962524555958,24.1608985086487));
#59912=CARTESIAN_POINT('Ctrl Pts',(5.69710560176435,12.0486025329149,24.1845471907116));
#59913=CARTESIAN_POINT('Ctrl Pts',(5.87743847974876,11.9981020660959,24.2096105993519));
#59914=CARTESIAN_POINT('Ctrl Pts',(6.05372901480326,11.9463090227909,24.2354575530271));
#59915=CARTESIAN_POINT('Ctrl Pts',(6.22601604554166,11.8935163209721,24.2619703523821));
#59916=CARTESIAN_POINT('Ctrl Pts',(6.24124062221443,11.8888511611329,24.2643132225614));
#59917=CARTESIAN_POINT('Ctrl Pts',(6.25643394241564,11.8841781814134,24.2666612898628));
#59918=CARTESIAN_POINT('Ctrl Pts',(6.27159604047703,11.8794975711571,24.2690144967149));
#59919=CARTESIAN_POINT('Origin',(-5.999994993362,10.9277770074801,24.1259380195517));
#59920=CARTESIAN_POINT('Origin',(5.99999999906,10.9277802195584,24.1259421376201));
#59921=CARTESIAN_POINT('Origin',(5.99996968668208,10.9277552850209,24.1259230381653));
#59922=CARTESIAN_POINT('Ctrl Pts',(6.25331147241795,8.42894521849349,13.948377678764));
#59923=CARTESIAN_POINT('Ctrl Pts',(6.30255402214553,8.40744222105348,13.9453310478153));
#59924=CARTESIAN_POINT('Ctrl Pts',(6.44286889530678,8.33601401238666,13.9419588806518));
#59925=CARTESIAN_POINT('Ctrl Pts',(6.65934670592776,8.1750683081117,13.9631279626853));
#59926=CARTESIAN_POINT('Ctrl Pts',(6.87326007648327,7.92769689971508,14.0292863828931));
#59927=CARTESIAN_POINT('Ctrl Pts',(7.02774581839624,7.63652467033211,14.1338750541619));
#59928=CARTESIAN_POINT('Ctrl Pts',(7.09502298419993,7.37242077306597,14.2481499818927));
#59929=CARTESIAN_POINT('Ctrl Pts',(7.10386618336956,7.21380101513048,14.3251097596679));
#59930=CARTESIAN_POINT('Ctrl Pts',(7.10318236346192,7.16033603230201,14.352035876389));
#59931=CARTESIAN_POINT('Ctrl Pts',(6.05603900145848,8.02832546593723,13.4854857122089));
#59932=CARTESIAN_POINT('Ctrl Pts',(6.09977809654048,8.00942840821252,13.48252913969));
#59933=CARTESIAN_POINT('Ctrl Pts',(6.22466181234398,7.94659667061775,13.4786408662298));
#59934=CARTESIAN_POINT('Ctrl Pts',(6.41837418436726,7.80451142267422,13.4954440662563));
#59935=CARTESIAN_POINT('Ctrl Pts',(6.61083155733378,7.58521226783456,13.5518110042824));
#59936=CARTESIAN_POINT('Ctrl Pts',(6.7503372588355,7.32644368001614,13.6428774049336));
#59937=CARTESIAN_POINT('Ctrl Pts',(6.81114777276548,7.09176064198665,13.7435290137315));
#59938=CARTESIAN_POINT('Ctrl Pts',(6.81910616842577,6.95129282556063,13.8115623985171));
#59939=CARTESIAN_POINT('Ctrl Pts',(6.81849079330802,6.90404543882402,13.8353666299144));
#59940=CARTESIAN_POINT('Ctrl Pts',(6.04665680408591,8.08800353272693,12.8453843521092));
#59941=CARTESIAN_POINT('Ctrl Pts',(6.10683798511585,8.0623848792519,12.841560624492));
#59942=CARTESIAN_POINT('Ctrl Pts',(6.27752443201705,7.97777606934776,12.837110603505));
#59943=CARTESIAN_POINT('Ctrl Pts',(6.53754543161355,7.78998742220227,12.8615274272874));
#59944=CARTESIAN_POINT('Ctrl Pts',(6.79117844125654,7.5057761358831,12.9376338739102));
#59945=CARTESIAN_POINT('Ctrl Pts',(6.9727101644675,7.17465351943412,13.0568546025352));
#59946=CARTESIAN_POINT('Ctrl Pts',(7.05158421179892,6.87547066530062,13.1864794295886));
#59947=CARTESIAN_POINT('Ctrl Pts',(7.06206245935511,6.69496529079826,13.2740717028483));
#59948=CARTESIAN_POINT('Ctrl Pts',(7.06125212490234,6.63390802281003,13.304820049174));
#59949=CARTESIAN_POINT('Ctrl Pts',(6.23115653270046,8.56708401712786,12.4587093936205));
#59950=CARTESIAN_POINT('Ctrl Pts',(6.31863448173896,8.52995082214717,12.4536458922549));
#59951=CARTESIAN_POINT('Ctrl Pts',(6.56546156683406,8.40788311970759,12.4489662200631));
#59952=CARTESIAN_POINT('Ctrl Pts',(6.93613642272148,8.14066201853445,12.4878374168353));
#59953=CARTESIAN_POINT('Ctrl Pts',(7.29230959064227,7.74235076973145,12.5998939031533));
#59954=CARTESIAN_POINT('Ctrl Pts',(7.54452359386327,7.28293596703667,12.7699474219303));
#59955=CARTESIAN_POINT('Ctrl Pts',(7.65380606172403,6.86885355188191,12.9515917840878));
#59956=CARTESIAN_POINT('Ctrl Pts',(7.66850900399649,6.61713607686126,13.0740309563524));
#59957=CARTESIAN_POINT('Ctrl Pts',(7.66737181947984,6.5315594617666,13.1171039874949));
#59958=CARTESIAN_POINT('',(6.9999916354347,6.97709969495907,13.9487325181045));
#59959=CARTESIAN_POINT('',(7.00000025951341,8.04447732699761,12.5220641950641));
#59960=CARTESIAN_POINT('Ctrl Pts',(7.,6.97709969493429,13.94873251817));
#59961=CARTESIAN_POINT('Ctrl Pts',(7.,7.02062865649979,13.8481984403386));
#59962=CARTESIAN_POINT('Ctrl Pts',(7.,7.06182311179943,13.7584316945066));
#59963=CARTESIAN_POINT('Ctrl Pts',(7.,7.09986953085516,13.6808089002891));
#59964=CARTESIAN_POINT('Ctrl Pts',(7.,7.11889274038302,13.6419975031804));
#59965=CARTESIAN_POINT('Ctrl Pts',(7.,7.13709521427333,13.6061961582339));
#59966=CARTESIAN_POINT('Ctrl Pts',(7.,7.15421673583155,13.5734556202725));
#59967=CARTESIAN_POINT('Ctrl Pts',(7.,7.16277749661066,13.5570853512918));
#59968=CARTESIAN_POINT('Ctrl Pts',(7.,7.17106680179347,13.5414792765318));
#59969=CARTESIAN_POINT('Ctrl Pts',(7.,7.17904737612002,13.5266383750259));
#59970=CARTESIAN_POINT('Ctrl Pts',(7.,7.1830376632833,13.5192179242729));
#59971=CARTESIAN_POINT('Ctrl Pts',(7.,7.18695076773252,13.5119887668335));
#59972=CARTESIAN_POINT('Ctrl Pts',(7.,7.1907818958336,13.5049506945816));
#59973=CARTESIAN_POINT('Ctrl Pts',(7.,7.19269745988415,13.5014316584557));
#59974=CARTESIAN_POINT('Ctrl Pts',(7.,7.19459252984766,13.4979603936266));
#59975=CARTESIAN_POINT('Ctrl Pts',(7.,7.19646651204854,13.4945368678279));
#59976=CARTESIAN_POINT('Ctrl Pts',(7.,7.19834049424942,13.4911133420292));
#59977=CARTESIAN_POINT('Ctrl Pts',(7.,7.19942602526282,13.4891321804845));
#59978=CARTESIAN_POINT('Ctrl Pts',(7.,7.20202460170296,13.4844094706777));
#59979=CARTESIAN_POINT('Ctrl Pts',(7.,7.24360182474522,13.408846113769));
#59980=CARTESIAN_POINT('Ctrl Pts',(7.,7.28586258548639,13.3375859005503));
#59981=CARTESIAN_POINT('Ctrl Pts',(7.,7.328413443107,13.2711285919118));
#59982=CARTESIAN_POINT('Ctrl Pts',(7.,7.37096430072761,13.2046712832734));
#59983=CARTESIAN_POINT('Ctrl Pts',(7.,7.41282803400312,13.144309635631));
#59984=CARTESIAN_POINT('Ctrl Pts',(7.,7.45598818177928,13.0863402094606));
#59985=CARTESIAN_POINT('Ctrl Pts',(7.,7.5423084773316,12.9704013571197));
#59986=CARTESIAN_POINT('Ctrl Pts',(7.,7.63586174972797,12.8624663289328));
#59987=CARTESIAN_POINT('Ctrl Pts',(7.,7.73521543344203,12.7672008088884));
#59988=CARTESIAN_POINT('Ctrl Pts',(7.,7.83456911715609,12.6719352888439));
#59989=CARTESIAN_POINT('Ctrl Pts',(7.,7.93954239456337,12.5894748091373));
#59990=CARTESIAN_POINT('Ctrl Pts',(7.,8.04447653888369,12.5220644911691));
#59991=CARTESIAN_POINT('',(6.24994452403135,8.55169657613351,12.4626509071323));
#59992=CARTESIAN_POINT('Ctrl Pts',(6.24994457521983,8.55169667629553,12.4626510531007));
#59993=CARTESIAN_POINT('Ctrl Pts',(6.29978446790311,8.52998434340969,12.4600718849041));
#59994=CARTESIAN_POINT('Ctrl Pts',(6.34860942389968,8.50674633505747,12.458637151969));
#59995=CARTESIAN_POINT('Ctrl Pts',(6.39644290451949,8.48204920681093,12.45829327108));
#59996=CARTESIAN_POINT('Ctrl Pts',(6.425658215371,8.46696491293324,12.4580832385477));
#59997=CARTESIAN_POINT('Ctrl Pts',(6.454503509566,8.45133541296467,12.4582806915151));
#59998=CARTESIAN_POINT('Ctrl Pts',(6.48298161554681,8.43516819850334,12.458878450293));
#59999=CARTESIAN_POINT('Ctrl Pts',(6.53032984027627,8.40828828928185,12.4598722950721));
#60000=CARTESIAN_POINT('Ctrl Pts',(6.57666452439768,8.3799238482972,12.4619712726638));
#60001=CARTESIAN_POINT('Ctrl Pts',(6.62201867977745,8.3500909877409,12.4651442021191));
#60002=CARTESIAN_POINT('Ctrl Pts',(6.63083239554454,8.34429353982768,12.465760800491));
#60003=CARTESIAN_POINT('Ctrl Pts',(6.63960900365929,8.33844052794818,12.466418038111));
#60004=CARTESIAN_POINT('Ctrl Pts',(6.64834862719593,8.33253191639426,12.4671158030968));
#60005=CARTESIAN_POINT('Ctrl Pts',(6.69477098455228,8.30114707746084,12.470822129277));
#60006=CARTESIAN_POINT('Ctrl Pts',(6.74013197243143,8.26820234249192,12.475673311407));
#60007=CARTESIAN_POINT('Ctrl Pts',(6.78442186677646,8.23368098850016,12.481666533661));
#60008=CARTESIAN_POINT('Ctrl Pts',(6.82871176112148,8.1991596345084,12.487659755915));
#60009=CARTESIAN_POINT('Ctrl Pts',(6.87193117326179,8.16306120631539,12.4947951523366));
#60010=CARTESIAN_POINT('Ctrl Pts',(6.91402897842334,8.12534103701035,12.5030954937722));
#60011=CARTESIAN_POINT('Ctrl Pts',(6.94323288792411,8.09917396234908,12.5088535711632));
#60012=CARTESIAN_POINT('Ctrl Pts',(6.97189609944987,8.07222583883693,12.5151728308876));
#60013=CARTESIAN_POINT('Ctrl Pts',(7.00000077683936,8.04447756164977,12.5220630299184));
#60014=CARTESIAN_POINT('',(6.26385807711555,8.42072586779743,13.9442710283615));
#60015=CARTESIAN_POINT('Origin',(6.52772556344856,9.09520187390111,13.2547574611158));
#60016=CARTESIAN_POINT('Ctrl Pts',(6.26385545879972,8.42071917467894,13.9442778706664));
#60017=CARTESIAN_POINT('Ctrl Pts',(6.30496680145664,8.39385467933137,13.9337310194281));
#60018=CARTESIAN_POINT('Ctrl Pts',(6.34565967410041,8.36408702383874,13.9242414338528));
#60019=CARTESIAN_POINT('Ctrl Pts',(6.38553796953683,8.3314258597232,13.9158860764687));
#60020=CARTESIAN_POINT('Ctrl Pts',(6.43022288687479,8.29482797100472,13.9065236288025));
#60021=CARTESIAN_POINT('Ctrl Pts',(6.47388545279323,8.25459587635117,13.8985855268188));
#60022=CARTESIAN_POINT('Ctrl Pts',(6.51600797558017,8.21087401920264,13.8921009540601));
#60023=CARTESIAN_POINT('Ctrl Pts',(6.52844998279364,8.1979596060565,13.8901855630601));
#60024=CARTESIAN_POINT('Ctrl Pts',(6.54075731479757,8.18474082982893,13.888397071652));
#60025=CARTESIAN_POINT('Ctrl Pts',(6.55291581058607,8.1712216559871,13.8867364803161));
#60026=CARTESIAN_POINT('Ctrl Pts',(6.57257265518867,8.14936498029407,13.8840517743783));
#60027=CARTESIAN_POINT('Ctrl Pts',(6.59184067821734,8.12672309019558,13.8817013219084));
#60028=CARTESIAN_POINT('Ctrl Pts',(6.61065772423113,8.10331314446322,13.8796902373481));
#60029=CARTESIAN_POINT('Ctrl Pts',(6.63494501282913,8.07309776912488,13.8770945169));
#60030=CARTESIAN_POINT('Ctrl Pts',(6.65848117657335,8.04160268323559,13.8750641472367));
#60031=CARTESIAN_POINT('Ctrl Pts',(6.68115250257791,8.00889137467638,13.8735913556586));
#60032=CARTESIAN_POINT('Ctrl Pts',(6.70127068946919,7.97986386129141,13.8722844230066));
#60033=CARTESIAN_POINT('Ctrl Pts',(6.72070781417969,7.9498786944054,13.8714165516457));
#60034=CARTESIAN_POINT('Ctrl Pts',(6.73937916399641,7.91898200451403,13.8709840640806));
#60035=CARTESIAN_POINT('Ctrl Pts',(6.74871483890477,7.90353365956835,13.870767820298));
#60036=CARTESIAN_POINT('Ctrl Pts',(6.75785902080652,7.8878574044475,13.8706604547887));
#60037=CARTESIAN_POINT('Ctrl Pts',(6.76680054007733,7.87195919711844,13.8706617016596));
#60038=CARTESIAN_POINT('Ctrl Pts',(6.77127129971274,7.8640100934539,13.870662325095));
#60039=CARTESIAN_POINT('Ctrl Pts',(6.7756913901382,7.85600549948828,13.8706901040865));
#60040=CARTESIAN_POINT('Ctrl Pts',(6.78005938330691,7.84794615914813,13.870745019926));
#60041=CARTESIAN_POINT('Ctrl Pts',(6.78279756125055,7.84289397451614,13.8707794451952));
#60042=CARTESIAN_POINT('Ctrl Pts',(6.78584184729762,7.83720799132701,13.8708299285122));
#60043=CARTESIAN_POINT('Ctrl Pts',(6.78857536488141,7.83203835562467,13.8708875817803));
#60044=CARTESIAN_POINT('Ctrl Pts',(6.7902024061723,7.82896129082126,13.8709218980943));
#60045=CARTESIAN_POINT('Ctrl Pts',(6.7917202829825,7.82606777959187,13.8709582453095));
#60046=CARTESIAN_POINT('Ctrl Pts',(6.79300562079399,7.8236046403435,13.8709911695315));
#60047=CARTESIAN_POINT('Ctrl Pts',(6.79345272558942,7.82274783728371,13.8710026222231));
#60048=CARTESIAN_POINT('Ctrl Pts',(6.79389954821732,7.82188983815143,13.8710143691982));
#60049=CARTESIAN_POINT('Ctrl Pts',(6.79434608427298,7.82103064210005,13.8710264118769));
#60050=CARTESIAN_POINT('Ctrl Pts',(6.81252333387961,7.78605514372952,13.8715166360683));
#60051=CARTESIAN_POINT('Ctrl Pts',(6.83022894062228,7.74909367512641,13.8724970484977));
#60052=CARTESIAN_POINT('Ctrl Pts',(6.84717623523151,7.71012612079511,13.8740440457161));
#60053=CARTESIAN_POINT('Ctrl Pts',(6.86323327632808,7.67320555997651,13.8755097780637));
#60054=CARTESIAN_POINT('Ctrl Pts',(6.87860976086485,7.63448416891028,13.877484028969));
#60055=CARTESIAN_POINT('Ctrl Pts',(6.89302553076019,7.59397247530125,13.8800306971348));
#60056=CARTESIAN_POINT('Ctrl Pts',(6.90424943002053,7.56243068660491,13.8820134942487));
#60057=CARTESIAN_POINT('Ctrl Pts',(6.91489035793338,7.52980412810098,13.8843432466388));
#60058=CARTESIAN_POINT('Ctrl Pts',(6.92479798906295,7.49611033022436,13.8870502692081));
#60059=CARTESIAN_POINT('Ctrl Pts',(6.92907683310261,7.48155886940268,13.8882193607129));
#60060=CARTESIAN_POINT('Ctrl Pts',(6.93321866944701,7.46680848796475,13.8894588320564));
#60061=CARTESIAN_POINT('Ctrl Pts',(6.93721230138223,7.4518625562698,13.8907701671218));
#60062=CARTESIAN_POINT('Ctrl Pts',(6.9484442045095,7.40982782205596,13.8944582356921));
#60063=CARTESIAN_POINT('Ctrl Pts',(6.95850648009574,7.36624350871026,13.8987151208828));
#60064=CARTESIAN_POINT('Ctrl Pts',(6.96712753753733,7.32120898892648,13.9035711092745));
#60065=CARTESIAN_POINT('Ctrl Pts',(6.97532946869924,7.27836389321998,13.9081910161458));
#60066=CARTESIAN_POINT('Ctrl Pts',(6.9822272334274,7.2342062429364,13.9133530784423));
#60067=CARTESIAN_POINT('Ctrl Pts',(6.98755254580326,7.18885404781863,13.9190811460232));
#60068=CARTESIAN_POINT('Ctrl Pts',(6.98923555651714,7.1745209486699,13.9208914434157));
#60069=CARTESIAN_POINT('Ctrl Pts',(6.99076122017395,7.1600687861646,13.9227582632191));
#60070=CARTESIAN_POINT('Ctrl Pts',(6.99212021289044,7.14550199364052,13.9246823352425));
#60071=CARTESIAN_POINT('Ctrl Pts',(6.99623922944679,7.10135101413096,13.9305140696029));
#60072=CARTESIAN_POINT('Ctrl Pts',(6.99882923224073,7.05614391289398,13.9368721862835));
#60073=CARTESIAN_POINT('Ctrl Pts',(6.99967290755981,7.0100657634129,13.9437477057266));
#60074=CARTESIAN_POINT('Ctrl Pts',(6.99987322812676,6.9991250604913,13.9453802152024));
#60075=CARTESIAN_POINT('Ctrl Pts',(6.99997495712425,6.98813543089333,13.9470418721719));
#60076=CARTESIAN_POINT('Ctrl Pts',(6.99997490630447,6.97709969502297,13.9487325180188));
#60077=CARTESIAN_POINT('Ctrl Pts',(6.99990207204853,6.87914589968496,13.8881633252755));
#60078=CARTESIAN_POINT('Ctrl Pts',(6.99990207204853,7.13651903111862,14.0922344622602));
#60079=CARTESIAN_POINT('Ctrl Pts',(6.99990207204853,7.80837747144884,14.6760282815914));
#60080=CARTESIAN_POINT('Ctrl Pts',(6.99990207204853,8.78348339483348,15.7555617435629));
#60081=CARTESIAN_POINT('Ctrl Pts',(6.99990207204853,9.70999136997589,17.1681316968964));
#60082=CARTESIAN_POINT('Ctrl Pts',(6.99990207204853,10.4111900158817,18.7078358093743));
#60083=CARTESIAN_POINT('Ctrl Pts',(6.99990207204853,10.8675506644196,20.3372588457581));
#60084=CARTESIAN_POINT('Ctrl Pts',(6.99990207204853,11.0696787430501,22.0150965875122));
#60085=CARTESIAN_POINT('Ctrl Pts',(6.99990207204853,11.0250235947296,23.3220448130867));
#60086=CARTESIAN_POINT('Ctrl Pts',(6.99990207204853,10.9251663319762,24.0577252196839));
#60087=CARTESIAN_POINT('Ctrl Pts',(6.99990207204853,10.8963460242105,24.2367460192875));
#60088=CARTESIAN_POINT('Ctrl Pts',(7.00660351962175,7.17662270770088,13.5129633937184));
#60089=CARTESIAN_POINT('Ctrl Pts',(7.00660351962175,7.44526632069181,13.7259689543078));
#60090=CARTESIAN_POINT('Ctrl Pts',(7.00660351962175,8.14635256616599,14.3351781181045));
#60091=CARTESIAN_POINT('Ctrl Pts',(7.00660351962175,9.16384720170705,15.4616262299551));
#60092=CARTESIAN_POINT('Ctrl Pts',(7.00660351962175,10.1310075548848,16.9361119525886));
#60093=CARTESIAN_POINT('Ctrl Pts',(7.00660351962175,10.8627090938492,18.5429270809962));
#60094=CARTESIAN_POINT('Ctrl Pts',(7.00660351962175,11.3389908857068,20.2432827124676));
#60095=CARTESIAN_POINT('Ctrl Pts',(7.00660351962175,11.5499472237732,21.9946879765234));
#60096=CARTESIAN_POINT('Ctrl Pts',(7.00660351962175,11.5033434054452,23.3583635329505));
#60097=CARTESIAN_POINT('Ctrl Pts',(7.00660351962175,11.39915283926,24.1260290318526));
#60098=CARTESIAN_POINT('Ctrl Pts',(7.00660351962175,11.3690777000579,24.3128491557423));
#60099=CARTESIAN_POINT('Ctrl Pts',(6.71669448330701,7.4134869680442,13.214212526843));
#60100=CARTESIAN_POINT('Ctrl Pts',(6.71669448330701,7.69110463953127,13.4343320727304));
#60101=CARTESIAN_POINT('Ctrl Pts',(6.71669448330701,8.4154633629351,14.0637780637606));
#60102=CARTESIAN_POINT('Ctrl Pts',(6.71669448330701,9.46670977568878,15.2275817056569));
#60103=CARTESIAN_POINT('Ctrl Pts',(6.71669448330701,10.4662393596655,16.7513675165855));
#60104=CARTESIAN_POINT('Ctrl Pts',(6.71669448330701,11.2222286582395,18.4116194196232));
#60105=CARTESIAN_POINT('Ctrl Pts',(6.71669448330701,11.714372550101,20.1684547369726));
#60106=CARTESIAN_POINT('Ctrl Pts',(6.71669448330701,11.932358340829,21.9784377330904));
#60107=CARTESIAN_POINT('Ctrl Pts',(6.71669448330701,11.8842029048076,23.3872821124319));
#60108=CARTESIAN_POINT('Ctrl Pts',(6.71669448330701,11.7765619697793,24.1804155638817));
#60109=CARTESIAN_POINT('Ctrl Pts',(6.71669448330701,11.7454876779928,24.3734458565265));
#60110=CARTESIAN_POINT('Ctrl Pts',(6.25325583820154,7.48886254419364,13.1191432298515));
#60111=CARTESIAN_POINT('Ctrl Pts',(6.25325583820154,7.76933596448606,13.3415266070968));
#60112=CARTESIAN_POINT('Ctrl Pts',(6.25325583820154,8.50110051783243,13.977412415217));
#60113=CARTESIAN_POINT('Ctrl Pts',(6.25325583820154,9.56308751107701,15.1531034334399));
#60114=CARTESIAN_POINT('Ctrl Pts',(6.25325583820154,10.5729177179411,16.6925776498335));
#60115=CARTESIAN_POINT('Ctrl Pts',(6.25325583820154,11.3366359320959,18.3698343457033));
#60116=CARTESIAN_POINT('Ctrl Pts',(6.25325583820154,11.8338275036932,20.1446427791995));
#60117=CARTESIAN_POINT('Ctrl Pts',(6.25325583820154,12.0540502255857,21.9732665373202));
#60118=CARTESIAN_POINT('Ctrl Pts',(6.25325583820154,12.0054010296428,23.3964846598617));
#60119=CARTESIAN_POINT('Ctrl Pts',(6.25325583820154,11.8966621090471,24.197722591042));
#60120=CARTESIAN_POINT('Ctrl Pts',(6.25325583820154,11.8652698642546,24.3927291001344));
#60121=CARTESIAN_POINT('Ctrl Pts',(6.99999999999964,6.9770996949353,13.9487325181688));
#60122=CARTESIAN_POINT('Ctrl Pts',(6.99999999999964,7.10630919510342,14.0533969802629));
#60123=CARTESIAN_POINT('Ctrl Pts',(6.9999999999822,7.23276302591308,14.1606658502628));
#60124=CARTESIAN_POINT('Ctrl Pts',(6.99999999939354,7.35656040710902,14.2705574401669));
#60125=CARTESIAN_POINT('Ctrl Pts',(6.99999999894868,7.45011564810677,14.3536038994521));
#60126=CARTESIAN_POINT('Ctrl Pts',(6.99999999821258,7.54215320932168,14.4381491461423));
#60127=CARTESIAN_POINT('Ctrl Pts',(6.99999999796688,7.63270310594372,14.5242160801555));
#60128=CARTESIAN_POINT('Ctrl Pts',(6.99999999764081,7.75286913175653,14.6384329020413));
#60129=CARTESIAN_POINT('Ctrl Pts',(6.99999999919465,7.87041678058885,14.7553285309957));
#60130=CARTESIAN_POINT('Ctrl Pts',(6.99999999987621,7.98540560911135,14.8750121804876));
#60131=CARTESIAN_POINT('Ctrl Pts',(6.99999999995187,7.99817037168945,14.8882981091284));
#60132=CARTESIAN_POINT('Ctrl Pts',(6.99999999999966,8.0109035611319,14.9016184278241));
#60133=CARTESIAN_POINT('Ctrl Pts',(6.99999999999966,8.02360522778826,14.9149733106003));
#60134=CARTESIAN_POINT('Ctrl Pts',(6.99999999999966,8.16383226758317,15.0624118892664));
#60135=CARTESIAN_POINT('Ctrl Pts',(6.99999999555676,8.30026050838411,15.2139928575566));
#60136=CARTESIAN_POINT('Ctrl Pts',(6.9999999949331,8.43247331547347,15.3693638375008));
#60137=CARTESIAN_POINT('Ctrl Pts',(6.9999999944045,8.54453604154188,15.5010552821329));
#60138=CARTESIAN_POINT('Ctrl Pts',(6.99999999611176,8.65357075339724,15.6354687272598));
#60139=CARTESIAN_POINT('Ctrl Pts',(6.99999999794596,8.75934445476941,15.7723688164645));
#60140=CARTESIAN_POINT('Ctrl Pts',(6.99999999900076,8.82017273892882,15.8510972472518));
#60141=CARTESIAN_POINT('Ctrl Pts',(6.99999999999966,8.87992292103336,15.9306477113447));
#60142=CARTESIAN_POINT('Ctrl Pts',(6.99999999999966,8.93856128342716,16.0109662939737));
#60143=CARTESIAN_POINT('Ctrl Pts',(6.99999999999966,9.09304441859853,16.2225661059487));
#60144=CARTESIAN_POINT('Ctrl Pts',(6.99999999747658,9.23974414863281,16.4395584290727));
#60145=CARTESIAN_POINT('Ctrl Pts',(6.99999999839567,9.37848092351118,16.6614642208066));
#60146=CARTESIAN_POINT('Ctrl Pts',(6.99999999910204,9.48510581806906,16.832007911664));
#60147=CARTESIAN_POINT('Ctrl Pts',(6.9999999999434,9.58702683609379,17.0054547377811));
#60148=CARTESIAN_POINT('Ctrl Pts',(6.99999999999483,9.6841487530217,17.1816030217134));
#60149=CARTESIAN_POINT('Ctrl Pts',(6.99999999999816,9.69044305714598,17.1930188885446));
#60150=CARTESIAN_POINT('Ctrl Pts',(6.99999999999966,9.69671719993505,17.204446106161));
#60151=CARTESIAN_POINT('Ctrl Pts',(6.99999999999966,9.70297115744669,17.2158846182766));
#60152=CARTESIAN_POINT('Ctrl Pts',(6.99999999999966,9.87483116551721,17.5302172278029));
#60153=CARTESIAN_POINT('Ctrl Pts',(7.00000000000773,10.0314645880133,17.8530584345459));
#60154=CARTESIAN_POINT('Ctrl Pts',(6.99999999997817,10.1719515132473,18.18283371903));
#60155=CARTESIAN_POINT('Ctrl Pts',(6.99999999996847,10.2181007081393,18.291163115868));
#60156=CARTESIAN_POINT('Ctrl Pts',(6.99999999999966,10.2625076901965,18.4002403628134));
#60157=CARTESIAN_POINT('Ctrl Pts',(6.99999999999966,10.3051403168605,18.5100085133683));
#60158=CARTESIAN_POINT('Ctrl Pts',(6.99999999999966,10.3319503563143,18.5790375335677));
#60159=CARTESIAN_POINT('Ctrl Pts',(6.99999999997182,10.358061234196,18.6483391264715));
#60160=CARTESIAN_POINT('Ctrl Pts',(6.99999999993242,10.3834658664667,18.7178989075883));
#60161=CARTESIAN_POINT('Ctrl Pts',(6.99999999971846,10.5214375580093,19.0956757067867));
#60162=CARTESIAN_POINT('Ctrl Pts',(6.99999999999966,10.6385735736358,19.481068218458));
#60163=CARTESIAN_POINT('Ctrl Pts',(6.99999999999966,10.7343189353094,19.8715618853161));
#60164=CARTESIAN_POINT('Ctrl Pts',(6.99999999999966,10.7726975056961,20.0280873651628));
#60165=CARTESIAN_POINT('Ctrl Pts',(6.99999999962326,10.8076377716897,20.185433198903));
#60166=CARTESIAN_POINT('Ctrl Pts',(6.99999999912715,10.8391033444699,20.3434768176547));
#60167=CARTESIAN_POINT('Ctrl Pts',(6.99999999825489,10.8944266540483,20.6213518179981));
#60168=CARTESIAN_POINT('Ctrl Pts',(6.99999999886813,10.9390114311113,20.901384532212));
#60169=CARTESIAN_POINT('Ctrl Pts',(6.99999999981999,10.9726752761601,21.1829081638845));
#60170=CARTESIAN_POINT('Ctrl Pts',(6.99999999992605,10.9764261391342,21.2142758393488));
#60171=CARTESIAN_POINT('Ctrl Pts',(6.99999999999966,10.9800413701157,21.2456620137402));
#60172=CARTESIAN_POINT('Ctrl Pts',(6.99999999999966,10.9835206775455,21.2770657559186));
#60173=CARTESIAN_POINT('Ctrl Pts',(6.99999999999966,11.0078800144039,21.4969297230345));
#60174=CARTESIAN_POINT('Ctrl Pts',(6.99999999634613,11.0256232012553,21.7176567471409));
#60175=CARTESIAN_POINT('Ctrl Pts',(6.99999999542162,11.0366759629532,21.9386384483813));
#60176=CARTESIAN_POINT('Ctrl Pts',(6.99999999531135,11.0379943367139,21.9649971526099));
#60177=CARTESIAN_POINT('Ctrl Pts',(6.99999999523594,11.0392175818929,21.991359479604));
#60178=CARTESIAN_POINT('Ctrl Pts',(6.99999999520043,11.0403456220732,22.017724397347));
#60179=CARTESIAN_POINT('Ctrl Pts',(6.99999999489237,11.0501296267264,22.2463992995019));
#60180=CARTESIAN_POINT('Ctrl Pts',(6.99999999999966,11.0527466422052,22.4752684797614));
#60181=CARTESIAN_POINT('Ctrl Pts',(6.99999999999966,11.0482982700561,22.7036632710443));
#60182=CARTESIAN_POINT('Ctrl Pts',(6.99999999999966,11.04498338064,22.8738611436468));
#60183=CARTESIAN_POINT('Ctrl Pts',(6.99999999741397,11.0376887143849,23.0437872743491));
#60184=CARTESIAN_POINT('Ctrl Pts',(6.999999997457,11.0264496314453,23.2135421338117));
#60185=CARTESIAN_POINT('Ctrl Pts',(6.99999999749808,11.015721453047,23.3755803024133));
#60186=CARTESIAN_POINT('Ctrl Pts',(6.999999998651,11.0013989616562,23.5374627543917));
#60187=CARTESIAN_POINT('Ctrl Pts',(6.99999999924032,10.9834686167949,23.6992764926476));
#60188=CARTESIAN_POINT('Ctrl Pts',(6.99999999975843,10.9677048395953,23.8415378789977));
#60189=CARTESIAN_POINT('Ctrl Pts',(6.99999999990829,10.9491517993076,23.9837463392033));
#60190=CARTESIAN_POINT('Ctrl Pts',(6.99999999989363,10.927773309634,24.1259362011891));
#60191=CARTESIAN_POINT('Ctrl Pts',(6.26386081937142,8.42073287750616,13.9442638621487));
#60192=CARTESIAN_POINT('Ctrl Pts',(6.26460715755161,8.6058952350089,14.1256648827888));
#60193=CARTESIAN_POINT('Ctrl Pts',(6.26531568582214,8.78358439506317,14.3114857095034));
#60194=CARTESIAN_POINT('Ctrl Pts',(6.26598638726736,8.95374370287065,14.501085754477));
#60195=CARTESIAN_POINT('Ctrl Pts',(6.26666473794233,9.12584364707761,14.6928481539722));
#60196=CARTESIAN_POINT('Ctrl Pts',(6.26730439407986,9.29024105734324,14.8884764945959));
#60197=CARTESIAN_POINT('Ctrl Pts',(6.26790534152617,9.44691000884794,15.0873499596924));
#60198=CARTESIAN_POINT('Ctrl Pts',(6.26800176663185,9.47204834714509,15.1192602290592));
#60199=CARTESIAN_POINT('Ctrl Pts',(6.26809719515578,9.49698777632441,15.1512541330831));
#60200=CARTESIAN_POINT('Ctrl Pts',(6.26819162704677,9.52172826504943,15.1833292053216));
#60201=CARTESIAN_POINT('Ctrl Pts',(6.26876871480417,9.67292118308826,15.3793448872247));
#60202=CARTESIAN_POINT('Ctrl Pts',(6.26930858191222,9.81668277327996,15.5783878909095));
#60203=CARTESIAN_POINT('Ctrl Pts',(6.26981121816768,9.95308962999951,15.7798039214011));
#60204=CARTESIAN_POINT('Ctrl Pts',(6.27017912420821,10.0529330177616,15.9272309592898));
#60205=CARTESIAN_POINT('Ctrl Pts',(6.27052708368989,10.1488365136903,16.0759303990776));
#60206=CARTESIAN_POINT('Ctrl Pts',(6.27085509339984,10.2408369655875,16.2256619541204));
#60207=CARTESIAN_POINT('Ctrl Pts',(6.2712113779156,10.3407679598827,16.3883005375646));
#60208=CARTESIAN_POINT('Ctrl Pts',(6.27154412378864,10.4360939213311,16.5521566168677));
#60209=CARTESIAN_POINT('Ctrl Pts',(6.2718533269388,10.5268693884646,16.7169400098764));
#60210=CARTESIAN_POINT('Ctrl Pts',(6.27227096849388,10.6494800644449,16.9395133972145));
#60211=CARTESIAN_POINT('Ctrl Pts',(6.27264565867609,10.7637884966596,17.1637765277338));
#60212=CARTESIAN_POINT('Ctrl Pts',(6.27297738955254,10.8699989601779,17.3890723859027));
#60213=CARTESIAN_POINT('Ctrl Pts',(6.27330912042898,10.9762094236961,17.6143682440716));
#60214=CARTESIAN_POINT('Ctrl Pts',(6.27359789201885,11.0743220034987,17.8406970067989));
#60215=CARTESIAN_POINT('Ctrl Pts',(6.27384369853182,11.1645577069347,18.067457721897));
#60216=CARTESIAN_POINT('Ctrl Pts',(6.27395596472971,11.2057706887037,18.1710252108335));
#60217=CARTESIAN_POINT('Ctrl Pts',(6.27405926854011,11.2453407879993,18.2746835591084));
#60218=CARTESIAN_POINT('Ctrl Pts',(6.27415361658734,11.2832901518629,18.3783792666538));
#60219=CARTESIAN_POINT('Ctrl Pts',(6.27415652014011,11.2844580401626,18.3815704928362));
#60220=CARTESIAN_POINT('Ctrl Pts',(6.27415941515016,11.2856243934921,18.3847617544467));
#60221=CARTESIAN_POINT('Ctrl Pts',(6.2741623016233,11.28678921251,18.3879530499727));
#60222=CARTESIAN_POINT('Ctrl Pts',(6.27420631168118,11.3045492088017,18.436610734845));
#60223=CARTESIAN_POINT('Ctrl Pts',(6.27424833715608,11.3219525216513,18.4852762942839));
#60224=CARTESIAN_POINT('Ctrl Pts',(6.27428839865745,11.339002369061,18.5339441294818));
#60225=CARTESIAN_POINT('Ctrl Pts',(6.2743178505947,11.3515368727312,18.5697231686864));
#60226=CARTESIAN_POINT('Ctrl Pts',(6.27434670178379,11.3640966427874,18.6061341459457));
#60227=CARTESIAN_POINT('Ctrl Pts',(6.27437398807154,11.3762335233597,18.6418700169536));
#60228=CARTESIAN_POINT('Ctrl Pts',(6.27438625179296,11.3816883995814,18.6579313724119));
#60229=CARTESIAN_POINT('Ctrl Pts',(6.27439819940099,11.3870585284997,18.6738561212743));
#60230=CARTESIAN_POINT('Ctrl Pts',(6.27440974336018,11.3923064605535,18.6895245117215));
#60231=CARTESIAN_POINT('Ctrl Pts',(6.274560647478,11.4609081026565,18.8943437248441));
#60232=CARTESIAN_POINT('Ctrl Pts',(6.27467736549451,11.5248696283609,19.1037519752928));
#60233=CARTESIAN_POINT('Ctrl Pts',(6.27475989567,11.5836612122644,19.3175737252288));
#60234=CARTESIAN_POINT('Ctrl Pts',(6.27484107236027,11.6414886210769,19.5278888235064));
#60235=CARTESIAN_POINT('Ctrl Pts',(6.27488917337323,11.6943142587797,19.7424739301517));
#60236=CARTESIAN_POINT('Ctrl Pts',(6.27490419802558,11.7416106438955,19.9611171627007));
#60237=CARTESIAN_POINT('Ctrl Pts',(6.27490863189467,11.7555681036062,20.025640151125));
#60238=CARTESIAN_POINT('Ctrl Pts',(6.27491018522552,11.7690438774239,20.0905162465538));
#60239=CARTESIAN_POINT('Ctrl Pts',(6.27490885801623,11.7820240141381,20.1557392229126));
#60240=CARTESIAN_POINT('Ctrl Pts',(6.27490450962152,11.8245514121042,20.3694321549065));
#60241=CARTESIAN_POINT('Ctrl Pts',(6.27486924020097,11.8617597650821,20.5868522809959));
#60242=CARTESIAN_POINT('Ctrl Pts',(6.27480305022229,11.8931690681274,20.8077236719151));
#60243=CARTESIAN_POINT('Ctrl Pts',(6.27475277155223,11.9170279364352,20.9755001240474));
#60244=CARTESIAN_POINT('Ctrl Pts',(6.2746846514378,11.9375403381901,21.1452670712505));
#60245=CARTESIAN_POINT('Ctrl Pts',(6.27459869040533,11.9544888397465,21.3168846885222));
#60246=CARTESIAN_POINT('Ctrl Pts',(6.27448994587059,11.9759294490948,21.5339886181507));
#60247=CARTESIAN_POINT('Ctrl Pts',(6.27435264873577,11.9916671385014,21.7540557993486));
#60248=CARTESIAN_POINT('Ctrl Pts',(6.27418680148104,12.0012474181871,21.9767636838325));
#60249=CARTESIAN_POINT('Ctrl Pts',(6.27401315166475,12.0112784181575,22.2099492333138));
#60250=CARTESIAN_POINT('Ctrl Pts',(6.27380820214771,12.0145579386257,22.4460299249337));
#60251=CARTESIAN_POINT('Ctrl Pts',(6.27357195670799,12.0106606480893,22.6846258656287));
#60252=CARTESIAN_POINT('Ctrl Pts',(6.27333930431345,12.0068226312514,22.9195930124892));
#60253=CARTESIAN_POINT('Ctrl Pts',(6.27307630070905,11.9960244157004,23.1569995372925));
#60254=CARTESIAN_POINT('Ctrl Pts',(6.27278295049408,11.9778553213893,23.3964324270879));
#60255=CARTESIAN_POINT('Ctrl Pts',(6.27261681839334,11.9675656755929,23.5320296993485));
#60256=CARTESIAN_POINT('Ctrl Pts',(6.27244095336116,11.9549119178812,23.6682759604467));
#60257=CARTESIAN_POINT('Ctrl Pts',(6.27225535638668,11.9398188605389,23.8050887673585));
#60258=CARTESIAN_POINT('Ctrl Pts',(6.27204648360782,11.9228329757344,23.9590593331134));
#60259=CARTESIAN_POINT('Ctrl Pts',(6.27182528484552,11.9027576373191,24.1137477342554));
#60260=CARTESIAN_POINT('Ctrl Pts',(6.27159176169286,11.8794807213832,24.2690119676737));
#60261=CARTESIAN_POINT('Ctrl Pts',(-6.390310997221,8.13937950336677,13.724966055094));
#60262=CARTESIAN_POINT('Ctrl Pts',(-4.26020733148,9.11426650158535,13.8221738588783));
#60263=CARTESIAN_POINT('Ctrl Pts',(0.0001535202090341,10.090263157491,13.9182984617449));
#60264=CARTESIAN_POINT('Ctrl Pts',(4.260514371898,9.11419615983807,13.8221669310127));
#60265=CARTESIAN_POINT('Ctrl Pts',(6.390771557848,8.13916871046851,13.7249450365314));
#60266=CARTESIAN_POINT('Ctrl Pts',(-6.390310997221,8.71309690457886,14.2543287817288));
#60267=CARTESIAN_POINT('Ctrl Pts',(-4.26020733148,9.62713419180251,14.3567676707055));
#60268=CARTESIAN_POINT('Ctrl Pts',(0.0001535202090341,10.5425537312226,
14.4578350530826));
#60269=CARTESIAN_POINT('Ctrl Pts',(4.260514371898,9.62706821595377,14.3567603866072));
#60270=CARTESIAN_POINT('Ctrl Pts',(6.390771557848,8.71289926878235,14.2543066320824));
#60271=CARTESIAN_POINT('Ctrl Pts',(-6.390310997221,9.96973300996386,15.6641218054972));
#60272=CARTESIAN_POINT('Ctrl Pts',(-4.26020733148,10.7489906364333,15.7526919792829));
#60273=CARTESIAN_POINT('Ctrl Pts',(0.0001535202090341,11.5273040839031,
15.8421753984647));
#60274=CARTESIAN_POINT('Ctrl Pts',(4.260514371898,10.7489345420516,15.7526855300649));
#60275=CARTESIAN_POINT('Ctrl Pts',(6.390771557848,9.96956451660001,15.6641026546034));
#60276=CARTESIAN_POINT('Ctrl Pts',(-6.390310997221,11.387980958516,18.3168609124995));
#60277=CARTESIAN_POINT('Ctrl Pts',(-4.26020733148,12.0191857141961,18.305065900394));
#60278=CARTESIAN_POINT('Ctrl Pts',(0.0001535202090341,12.6510838649606,
18.2929947853334));
#60279=CARTESIAN_POINT('Ctrl Pts',(4.260514371898,12.0191401722118,18.3050667703745));
#60280=CARTESIAN_POINT('Ctrl Pts',(6.390771557848,11.3878444775859,18.3168634628528));
#60281=CARTESIAN_POINT('Ctrl Pts',(-6.390310997221,12.0713618431303,21.4528914163341));
#60282=CARTESIAN_POINT('Ctrl Pts',(-4.26020733148,12.6592425324047,21.2792389757137));
#60283=CARTESIAN_POINT('Ctrl Pts',(0.0001535202090341,13.2456889758127,
21.1056340488841));
#60284=CARTESIAN_POINT('Ctrl Pts',(4.260514371898,12.6592002662047,21.2792514877189));
#60285=CARTESIAN_POINT('Ctrl Pts',(6.390771557848,12.07123472984,21.4529289639673));
#60286=CARTESIAN_POINT('Ctrl Pts',(-6.390310997221,11.9720502124569,23.5458951845851));
#60287=CARTESIAN_POINT('Ctrl Pts',(-4.26020733148,12.6077625569466,23.2652553028773));
#60288=CARTESIAN_POINT('Ctrl Pts',(0.0001535202090341,13.2461450660892,
22.9846380445134));
#60289=CARTESIAN_POINT('Ctrl Pts',(4.260514371898,12.6077165476319,23.2652755274378));
#60290=CARTESIAN_POINT('Ctrl Pts',(6.390771557848,11.9719127569025,23.5459558653499));
#60291=CARTESIAN_POINT('Ctrl Pts',(-6.390310997221,11.8061936875927,24.5118462831628));
#60292=CARTESIAN_POINT('Ctrl Pts',(-4.26020733148,12.4817978962268,24.1870546128076));
#60293=CARTESIAN_POINT('Ctrl Pts',(0.0001535202090341,13.1582606881552,
23.8622603664262));
#60294=CARTESIAN_POINT('Ctrl Pts',(4.260514371898,12.4817491423946,24.1870780212883));
#60295=CARTESIAN_POINT('Ctrl Pts',(6.390771557848,11.8060476064905,24.5119165105573));
#60296=CARTESIAN_POINT('',(-6.26385899039824,8.42070725657994,13.944262563225));
#60297=CARTESIAN_POINT('Ctrl Pts',(-6.26386059994869,8.4207113711049,13.9442583573388));
#60298=CARTESIAN_POINT('Ctrl Pts',(-6.26455152048013,8.59292042455144,14.1129910531294));
#60299=CARTESIAN_POINT('Ctrl Pts',(-6.26520985692811,8.75834812375439,14.2852422441848));
#60300=CARTESIAN_POINT('Ctrl Pts',(-6.26583560983094,8.91699593500101,14.4604068244786));
#60301=CARTESIAN_POINT('Ctrl Pts',(-6.26647066381859,9.07800186035863,14.6381750213322));
#60302=CARTESIAN_POINT('Ctrl Pts',(-6.26707215842975,9.23202489931598,14.8189438733917));
#60303=CARTESIAN_POINT('Ctrl Pts',(-6.26764009422708,9.37909856275395,15.0021245936472));
#60304=CARTESIAN_POINT('Ctrl Pts',(-6.26812468345807,9.50458865124676,15.1584229019757));
#60305=CARTESIAN_POINT('Ctrl Pts',(-6.26858484087964,9.62501996429814,15.3164778898243));
#60306=CARTESIAN_POINT('Ctrl Pts',(-6.2690205668413,9.7404307958954,15.4759481442773));
#60307=CARTESIAN_POINT('Ctrl Pts',(-6.26953467307883,9.87660222845387,15.6641045997745));
#60308=CARTESIAN_POINT('Ctrl Pts',(-6.27001476762018,10.005784944435,15.8542296366687));
#60309=CARTESIAN_POINT('Ctrl Pts',(-6.27046085103946,10.1281582269328,16.0457333774502));
#60310=CARTESIAN_POINT('Ctrl Pts',(-6.27062083324975,10.1720458662577,16.1144137865495));
#60311=CARTESIAN_POINT('Ctrl Pts',(-6.27077644092214,10.215057822839,16.1832719922629));
#60312=CARTESIAN_POINT('Ctrl Pts',(-6.27092767408311,10.2572028653329,16.2522823290061));
#60313=CARTESIAN_POINT('Ctrl Pts',(-6.27136815432473,10.3799541083887,16.4532811681964));
#60314=CARTESIAN_POINT('Ctrl Pts',(-6.27177152391562,10.4953498718875,16.6555664402298));
#60315=CARTESIAN_POINT('Ctrl Pts',(-6.27213778285578,10.6036187611275,16.8585419856448));
#60316=CARTESIAN_POINT('Ctrl Pts',(-6.27250404179594,10.7118876503675,17.0615175310597));
#60317=CARTESIAN_POINT('Ctrl Pts',(-6.27283319008536,10.8130297690453,17.2651835383498));
#60318=CARTESIAN_POINT('Ctrl Pts',(-6.27312522772406,10.9072902654271,17.4689981447037));
#60319=CARTESIAN_POINT('Ctrl Pts',(-6.27334042077645,10.9767477642208,17.6191825095052));
#60320=CARTESIAN_POINT('Ctrl Pts',(-6.27353526317237,11.0423479808087,17.769176079745));
#60321=CARTESIAN_POINT('Ctrl Pts',(-6.27370997657693,11.1043415438198,17.919075764095));
#60322=CARTESIAN_POINT('Ctrl Pts',(-6.27388468998149,11.1663351068308,18.068975448445));
#60323=CARTESIAN_POINT('Ctrl Pts',(-6.2740392743947,11.2247220604115,18.2187816725573));
#60324=CARTESIAN_POINT('Ctrl Pts',(-6.27417395148167,11.2797074208758,18.3686262123368));
#60325=CARTESIAN_POINT('Ctrl Pts',(-6.27427013678984,11.3189775295513,18.4756439951042));
#60326=CARTESIAN_POINT('Ctrl Pts',(-6.27435616796176,11.3565116921192,18.5826820367218));
#60327=CARTESIAN_POINT('Ctrl Pts',(-6.27443212574741,11.3923815531531,18.6897932929545));
#60328=CARTESIAN_POINT('Ctrl Pts',(-6.27457884479819,11.4616673007278,18.8966879741109));
#60329=CARTESIAN_POINT('Ctrl Pts',(-6.27469165460118,11.5261460216362,19.1080571548633));
#60330=CARTESIAN_POINT('Ctrl Pts',(-6.27477055515638,11.5853122037843,19.3236966635228));
#60331=CARTESIAN_POINT('Ctrl Pts',(-6.27484862828138,11.643857910118,19.5370747604283));
#60332=CARTESIAN_POINT('Ctrl Pts',(-6.27489349964197,11.6972019214643,19.754634199829));
#60333=CARTESIAN_POINT('Ctrl Pts',(-6.27490516923817,11.7448338369295,19.9761313157618));
#60334=CARTESIAN_POINT('Ctrl Pts',(-6.27491664524404,11.7916755726868,20.1939539515765));
#60335=CARTESIAN_POINT('Ctrl Pts',(-6.2748960119357,11.8329931410015,20.4155847540337));
#60336=CARTESIAN_POINT('Ctrl Pts',(-6.27484326931315,11.8682812208486,20.6407462755647));
#60337=CARTESIAN_POINT('Ctrl Pts',(-6.27479056675521,11.9035424949843,20.8657367587512));
#60338=CARTESIAN_POINT('Ctrl Pts',(-6.27470580364662,11.9327834716963,21.0942527726353));
#60339=CARTESIAN_POINT('Ctrl Pts',(-6.27458897998737,11.9554797474119,21.3259696114708));
#60340=CARTESIAN_POINT('Ctrl Pts',(-6.2745478138118,11.9634774327867,21.4076217026017));
#60341=CARTESIAN_POINT('Ctrl Pts',(-6.27450266669875,11.9706622713164,21.4896707935314));
#60342=CARTESIAN_POINT('Ctrl Pts',(-6.27445353863612,11.9770107062091,21.5721011963808));
#60343=CARTESIAN_POINT('Ctrl Pts',(-6.27431624106106,11.9947525968845,21.8024684003303));
#60344=CARTESIAN_POINT('Ctrl Pts',(-6.27414785116559,12.0059621132111,22.0358174529015));
#60345=CARTESIAN_POINT('Ctrl Pts',(-6.27394836868557,12.0102364706698,22.2717644772196));
#60346=CARTESIAN_POINT('Ctrl Pts',(-6.27375072726245,12.0144713793746,22.5055339073128));
#60347=CARTESIAN_POINT('Ctrl Pts',(-6.27352256452363,12.0118985251308,22.7418536687606));
#60348=CARTESIAN_POINT('Ctrl Pts',(-6.27326388021221,12.0021219229472,22.9802999805628));
#60349=CARTESIAN_POINT('Ctrl Pts',(-6.27300884387037,11.9924831905364,23.2153837193321));
#60350=CARTESIAN_POINT('Ctrl Pts',(-6.27272414071743,11.975842425797,23.4525344972157));
#60351=CARTESIAN_POINT('Ctrl Pts',(-6.27240977050724,11.9518163952354,23.6912960224347));
#60352=CARTESIAN_POINT('Ctrl Pts',(-6.27215746727189,11.9325338899391,23.8829182033343));
#60353=CARTESIAN_POINT('Ctrl Pts',(-6.27188605506393,11.9084943551137,24.0755769702775));
#60354=CARTESIAN_POINT('Ctrl Pts',(-6.27159553375607,11.879498052505,24.2690121689631));
#60355=CARTESIAN_POINT('Ctrl Pts',(-6.26386059994846,8.42071137104667,13.9442583572817));
#60356=CARTESIAN_POINT('Ctrl Pts',(-5.93717696836598,8.56158840445482,13.9570575565163));
#60357=CARTESIAN_POINT('Ctrl Pts',(-5.60632732377181,8.69216934607849,13.9678446821751));
#60358=CARTESIAN_POINT('Ctrl Pts',(-5.27194469098664,8.81191899897469,13.9769587750825));
#60359=CARTESIAN_POINT('Ctrl Pts',(-4.97209615130009,8.91930124622187,13.9851315902377));
#60360=CARTESIAN_POINT('Ctrl Pts',(-4.66940669402091,9.01797284387651,13.991959419582));
#60361=CARTESIAN_POINT('Ctrl Pts',(-4.36433277146454,9.10758639984849,13.9977003959948));
#60362=CARTESIAN_POINT('Ctrl Pts',(-4.0887152634072,9.18854731836354,14.0028870523943));
#60363=CARTESIAN_POINT('Ctrl Pts',(-3.81115152413417,9.26211453872501,14.0071867723874));
#60364=CARTESIAN_POINT('Ctrl Pts',(-3.53197814314358,9.32807438052413,14.0107986489402));
#60365=CARTESIAN_POINT('Ctrl Pts',(-3.4190946039569,9.35474519118688,14.0122591084114));
#60366=CARTESIAN_POINT('Ctrl Pts',(-3.30594789109754,9.3801727576117,14.013607200518));
#60367=CARTESIAN_POINT('Ctrl Pts',(-3.19256025663433,9.40434542805185,14.0148564684661));
#60368=CARTESIAN_POINT('Ctrl Pts',(-2.94892827982676,9.45628438516944,14.0175407260678));
#60369=CARTESIAN_POINT('Ctrl Pts',(-2.70418858676455,9.50244713954166,14.019792523974));
#60370=CARTESIAN_POINT('Ctrl Pts',(-2.45859671448438,9.54266471038575,14.0216629006831));
#60371=CARTESIAN_POINT('Ctrl Pts',(-2.21908138008969,9.58188720109698,14.0234869997413));
#60372=CARTESIAN_POINT('Ctrl Pts',(-1.97875551474025,9.61545500774489,14.0249483422051));
#60373=CARTESIAN_POINT('Ctrl Pts',(-1.73785615309579,9.64326071165928,14.0260991718243));
#60374=CARTESIAN_POINT('Ctrl Pts',(-1.49989746871486,9.67072698918109,14.0272359531768));
#60375=CARTESIAN_POINT('Ctrl Pts',(-1.2613792040085,9.69257085714106,14.0280697696858));
#60376=CARTESIAN_POINT('Ctrl Pts',(-1.0225298186672,9.7087390174652,14.0286555606451));
#60377=CARTESIAN_POINT('Ctrl Pts',(-0.787286942176469,9.72466304647947,
14.0292325064476));
#60378=CARTESIAN_POINT('Ctrl Pts',(-0.551722869076018,9.73508141111193,
14.0295688746588));
#60379=CARTESIAN_POINT('Ctrl Pts',(-0.316055865644371,9.73999356983431,
14.0297214195832));
#60380=CARTESIAN_POINT('Ctrl Pts',(-0.21080646463155,9.74218735070173,14.0297895464813));
#60381=CARTESIAN_POINT('Ctrl Pts',(-0.105536533801802,9.74328358190328,
14.0298210651924));
#60382=CARTESIAN_POINT('Ctrl Pts',(-0.000265515525107667,9.74328558134228,
14.0298213016319));
#60383=CARTESIAN_POINT('Ctrl Pts',(-0.000177010350108755,9.74328558302328,
14.0298213018307));
#60384=CARTESIAN_POINT('Ctrl Pts',(-8.8505175545061E-5,9.74328558393097,
14.0298213020073));
#60385=CARTESIAN_POINT('Ctrl Pts',(-1.42996123777008E-12,9.74328558406533,
14.0298213021619));
#60386=CARTESIAN_POINT('Ctrl Pts',(0.235250051412205,9.74328594120638,14.0298217130422));
#60387=CARTESIAN_POINT('Ctrl Pts',(0.470496939858318,9.73781829803784,14.0296656159884));
#60388=CARTESIAN_POINT('Ctrl Pts',(0.705523626716445,9.72685975003266,14.029294704648));
#60389=CARTESIAN_POINT('Ctrl Pts',(0.944752984767102,9.7157052448167,14.028917160791));
#60390=CARTESIAN_POINT('Ctrl Pts',(1.18375419567222,9.69886173425948,14.0283170354621));
#60391=CARTESIAN_POINT('Ctrl Pts',(1.42229836833,9.67635915367304,14.0274372869502));
#60392=CARTESIAN_POINT('Ctrl Pts',(1.66374043057524,9.6535832065514,14.0265468510506));
#60393=CARTESIAN_POINT('Ctrl Pts',(1.90471428271175,9.6250099765416,14.0253699432079));
#60394=CARTESIAN_POINT('Ctrl Pts',(2.14498259002289,9.5907242399444,14.0238521563959));
#60395=CARTESIAN_POINT('Ctrl Pts',(2.39034044630107,9.55571223637827,14.0223022186507));
#60396=CARTESIAN_POINT('Ctrl Pts',(2.63496255037747,9.51474323025704,14.0203967857286));
#60397=CARTESIAN_POINT('Ctrl Pts',(2.87859616357419,9.46796179871245,14.0180831143291));
#60398=CARTESIAN_POINT('Ctrl Pts',(2.9833098709974,9.44785514318441,14.017088698547));
#60399=CARTESIAN_POINT('Ctrl Pts',(3.08784097650595,9.4266754343928,14.0160189359209));
#60400=CARTESIAN_POINT('Ctrl Pts',(3.1921694136428,9.40443706680239,14.0148699389744));
#60401=CARTESIAN_POINT('Ctrl Pts',(3.47744261700037,9.34362900205935,14.0117281489836));
#60402=CARTESIAN_POINT('Ctrl Pts',(3.7611942824795,9.27487280401547,14.0079602275019));
#60403=CARTESIAN_POINT('Ctrl Pts',(4.04306981736332,9.19837143643058,14.0033530332897));
#60404=CARTESIAN_POINT('Ctrl Pts',(4.3441061229289,9.11666981206661,13.9984326604549));
#60405=CARTESIAN_POINT('Ctrl Pts',(4.64300256509685,9.02613498942633,13.9925549084651));
#60406=CARTESIAN_POINT('Ctrl Pts',(4.93932721295378,8.92707680407218,13.9854712892336));
#60407=CARTESIAN_POINT('Ctrl Pts',(5.28135521912764,8.81274047101008,13.9772951345338));
#60408=CARTESIAN_POINT('Ctrl Pts',(5.6199569361215,8.6870497021254,13.9675119701404));
#60409=CARTESIAN_POINT('Ctrl Pts',(5.95446816838324,8.55054995909253,13.9557592260817));
#60410=CARTESIAN_POINT('Ctrl Pts',(6.05799647460643,8.50830448021714,13.9521218543928));
#60411=CARTESIAN_POINT('Ctrl Pts',(6.16113297437773,8.4650240396021,13.9482959819136));
#60412=CARTESIAN_POINT('Ctrl Pts',(6.26385797790307,8.4207256142375,13.944271287676));
#60413=CARTESIAN_POINT('Ctrl Pts',(-6.38404538826909,8.37116243072582,13.9421882754888));
#60414=CARTESIAN_POINT('Ctrl Pts',(-5.83050262796989,8.62265888536472,13.9723470810333));
#60415=CARTESIAN_POINT('Ctrl Pts',(-4.53016629286474,9.12937227622254,14.0254998662653));
#60416=CARTESIAN_POINT('Ctrl Pts',(-2.39024486123905,9.65381240370912,14.0662444267208));
#60417=CARTESIAN_POINT('Ctrl Pts',(0.000832361431650141,9.85055455252627,
14.0780418370757));
#60418=CARTESIAN_POINT('Ctrl Pts',(2.39185021568528,9.65354673660712,14.0662272090006));
#60419=CARTESIAN_POINT('Ctrl Pts',(4.53118408442122,9.12901549215188,14.0254666479336));
#60420=CARTESIAN_POINT('Ctrl Pts',(5.83097915587935,8.62244285400822,13.972321193994));
#60421=CARTESIAN_POINT('Ctrl Pts',(6.38405559839713,8.37115779336739,13.9421877126995));
#60422=CARTESIAN_POINT('Ctrl Pts',(-6.17704425963179,7.96381194474042,13.469457267312));
#60423=CARTESIAN_POINT('Ctrl Pts',(-5.64115395945954,8.20569173180422,13.5001727964708));
#60424=CARTESIAN_POINT('Ctrl Pts',(-4.38244641924109,8.6930773017877,13.5546902039183));
#60425=CARTESIAN_POINT('Ctrl Pts',(-2.31188356464167,9.19745367496022,13.5973133398307));
#60426=CARTESIAN_POINT('Ctrl Pts',(0.000805005365969324,9.38662212148953,
13.6099340037559));
#60427=CARTESIAN_POINT('Ctrl Pts',(2.31343653166433,9.19719821279148,13.597295055307));
#60428=CARTESIAN_POINT('Ctrl Pts',(4.38343153533807,8.69273412120314,13.554655889156));
#60429=CARTESIAN_POINT('Ctrl Pts',(5.64161529098573,8.20548395793609,13.5001464313595));
#60430=CARTESIAN_POINT('Ctrl Pts',(6.17705414513472,7.96380748312364,13.4694566948018));
#60431=CARTESIAN_POINT('Ctrl Pts',(-6.17529619645408,8.03269332841907,12.8173794683781));
#60432=CARTESIAN_POINT('Ctrl Pts',(-5.64080537297811,8.27163446441592,12.8477800372787));
#60433=CARTESIAN_POINT('Ctrl Pts',(-4.38470620031409,8.75357501952359,12.9017719820197));
#60434=CARTESIAN_POINT('Ctrl Pts',(-2.31484672892392,9.25351908787722,12.9440117423692));
#60435=CARTESIAN_POINT('Ctrl Pts',(0.000806324308182919,9.4413973955616,
12.9565148963448));
#60436=CARTESIAN_POINT('Ctrl Pts',(2.31640066515831,9.25326551722142,12.9439936229367));
#60437=CARTESIAN_POINT('Ctrl Pts',(4.38568966269628,8.75323537235754,12.901737984911));
#60438=CARTESIAN_POINT('Ctrl Pts',(5.64126549941951,8.27142921664869,12.8477539377952));
#60439=CARTESIAN_POINT('Ctrl Pts',(6.17530605203147,8.03268892390896,12.8173789001941));
#60440=CARTESIAN_POINT('Ctrl Pts',(-6.3774727247386,8.52454337342127,12.4367962200776));
#60441=CARTESIAN_POINT('Ctrl Pts',(-5.82736598295725,8.7691633154091,12.4662375870123));
#60442=CARTESIAN_POINT('Ctrl Pts',(-4.53354138556052,9.26311663296809,12.5181988107581));
#60443=CARTESIAN_POINT('Ctrl Pts',(-2.39609281858094,9.77711650863112,12.558084900948));
#60444=CARTESIAN_POINT('Ctrl Pts',(0.000835057210998115,9.97079836899108,
12.5696222296354));
#60445=CARTESIAN_POINT('Ctrl Pts',(2.39769975586005,9.7768553172162,12.5580680497235));
#60446=CARTESIAN_POINT('Ctrl Pts',(4.5345549711749,9.26276814234134,12.5181663094043));
#60447=CARTESIAN_POINT('Ctrl Pts',(5.82783955217292,8.76895319507773,12.4662123049363));
#60448=CARTESIAN_POINT('Ctrl Pts',(6.37748286204222,8.52453886954492,12.4367956671127));
#60449=CARTESIAN_POINT('',(-6.249945884441,8.55169184623365,12.462653724233));
#60450=CARTESIAN_POINT('Ctrl Pts',(-6.24994577295826,8.55169162808957,12.4626534063286));
#60451=CARTESIAN_POINT('Ctrl Pts',(-5.97414683512782,8.67183837135021,12.476926751268));
#60452=CARTESIAN_POINT('Ctrl Pts',(-5.69345325622611,8.7852362693789,12.4896158765507));
#60453=CARTESIAN_POINT('Ctrl Pts',(-5.40803913489735,8.8912995328883,12.5009061876321));
#60454=CARTESIAN_POINT('Ctrl Pts',(-5.2203826970391,8.96103488489237,12.508329434772));
#60455=CARTESIAN_POINT('Ctrl Pts',(-5.03068593865463,9.0275986149699,12.5151481565809));
#60456=CARTESIAN_POINT('Ctrl Pts',(-4.83900279328378,9.09081292957561,12.5214173229241));
#60457=CARTESIAN_POINT('Ctrl Pts',(-4.78610405895494,9.10825816310221,12.5231474226896));
#60458=CARTESIAN_POINT('Ctrl Pts',(-4.73305460290303,9.12544877501386,12.5248351566563));
#60459=CARTESIAN_POINT('Ctrl Pts',(-4.67985525062854,9.14238145556753,12.5264814015791));
#60460=CARTESIAN_POINT('Ctrl Pts',(-4.4900707310435,9.20278746629457,12.5323542513119));
#60461=CARTESIAN_POINT('Ctrl Pts',(-4.29837839943429,9.25991178170323,12.537698995585));
#60462=CARTESIAN_POINT('Ctrl Pts',(-4.10484844319214,9.31360787682988,12.5425507056659));
#60463=CARTESIAN_POINT('Ctrl Pts',(-3.98095883883625,9.34798182135955,12.5456565630435));
#60464=CARTESIAN_POINT('Ctrl Pts',(-3.85631586549759,9.38095127312882,12.5485600232877));
#60465=CARTESIAN_POINT('Ctrl Pts',(-3.7309389117039,9.41247972892901,12.5512670848039));
#60466=CARTESIAN_POINT('Ctrl Pts',(-3.66825043480706,9.42824395682911,12.552620615562));
#60467=CARTESIAN_POINT('Ctrl Pts',(-3.60537845978922,9.44364792669368,12.5539250344385));
#60468=CARTESIAN_POINT('Ctrl Pts',(-3.54232557106459,9.45868722349521,12.555180829398));
#60469=CARTESIAN_POINT('Ctrl Pts',(-3.51079912670227,9.46620687189598,12.5558087268778));
#60470=CARTESIAN_POINT('Ctrl Pts',(-3.47922745375773,9.47363535146565,12.5564244676311));
#60471=CARTESIAN_POINT('Ctrl Pts',(-3.44761087944285,9.48097211313099,12.5570281024581));
#60472=CARTESIAN_POINT('Ctrl Pts',(-3.43180259228541,9.48464049396366,12.5573299198716));
#60473=CARTESIAN_POINT('Ctrl Pts',(-3.41598307977717,9.48828594528422,12.5576287107566));
#60474=CARTESIAN_POINT('Ctrl Pts',(-3.40015238340376,9.49190839899051,12.5579244804943));
#60475=CARTESIAN_POINT('Ctrl Pts',(-3.38432168703035,9.49553085269679,12.558220250232));
#60476=CARTESIAN_POINT('Ctrl Pts',(-3.36983043489144,9.49882561136923,12.5584883145983));
#60477=CARTESIAN_POINT('Ctrl Pts',(-3.35262678433449,9.5027066992511,12.5588027312502));
#60478=CARTESIAN_POINT('Ctrl Pts',(-3.03782920764183,9.57372401363455,12.5645560217955));
#60479=CARTESIAN_POINT('Ctrl Pts',(-2.72122916966243,9.63497186079253,12.5691453737108));
#60480=CARTESIAN_POINT('Ctrl Pts',(-2.40317289992791,9.68615982574975,12.5728383075911));
#60481=CARTESIAN_POINT('Ctrl Pts',(-2.09865862325337,9.73516834281624,12.5763740061337));
#60482=CARTESIAN_POINT('Ctrl Pts',(-1.79280890371693,9.77495539237363,12.5790876950664));
#60483=CARTESIAN_POINT('Ctrl Pts',(-1.48603152505855,9.80541199434123,12.5810916990609));
#60484=CARTESIAN_POINT('Ctrl Pts',(-1.18132021538454,9.83566347870542,12.5830822065893));
#60485=CARTESIAN_POINT('Ctrl Pts',(-0.875693114117407,9.85670979197821,
12.5843724777896));
#60486=CARTESIAN_POINT('Ctrl Pts',(-0.569548332777583,9.86839321701482,
12.585068453806));
#60487=CARTESIAN_POINT('Ctrl Pts',(-0.379870270103967,9.87563191439401,
12.5854996595312));
#60488=CARTESIAN_POINT('Ctrl Pts',(-0.189993493543507,9.87927550563717,
12.5857026581081));
#60489=CARTESIAN_POINT('Ctrl Pts',(-1.38566163258134E-5,9.87927649678122,
12.5857020423665));
#60490=CARTESIAN_POINT('Ctrl Pts',(0.000267316804323126,9.87927649824813,
12.5857020414552));
#60491=CARTESIAN_POINT('Ctrl Pts',(0.000548489975148814,9.87927649178495,
12.5857020400583));
#60492=CARTESIAN_POINT('Ctrl Pts',(0.000829662895873392,9.87927647739157,
12.5857020381761));
#60493=CARTESIAN_POINT('Ctrl Pts',(0.298695167394001,9.87926122951397,12.5857000441388));
#60494=CARTESIAN_POINT('Ctrl Pts',(0.596280588157101,9.87035061745305,12.5851534870738));
#60495=CARTESIAN_POINT('Ctrl Pts',(0.893243902548241,9.8526544670475,12.5840196522909));
#60496=CARTESIAN_POINT('Ctrl Pts',(1.15817186246262,9.83686731490417,12.5830081316035));
#60497=CARTESIAN_POINT('Ctrl Pts',(1.4226048826074,9.81408706026283,12.5815292139631));
#60498=CARTESIAN_POINT('Ctrl Pts',(1.6862923402662,9.78435764326541,12.5795502474415));
#60499=CARTESIAN_POINT('Ctrl Pts',(1.92647727742504,9.7572780156764,12.5777476666366));
#60500=CARTESIAN_POINT('Ctrl Pts',(2.16604769956152,9.72445009753053,12.5755159664622));
#60501=CARTESIAN_POINT('Ctrl Pts',(2.40481940572151,9.68596137852757,12.5727677736108));
#60502=CARTESIAN_POINT('Ctrl Pts',(2.44417119287767,9.67961808139879,12.5723148459926));
#60503=CARTESIAN_POINT('Ctrl Pts',(2.48350129415924,9.67312097694517,12.5718478849593));
#60504=CARTESIAN_POINT('Ctrl Pts',(2.52280914060445,9.66647082366531,12.571366243551));
#60505=CARTESIAN_POINT('Ctrl Pts',(2.66171560913018,9.64297044420424,12.5696642142317));
#60506=CARTESIAN_POINT('Ctrl Pts',(2.80034190062008,9.61755692273634,12.5677807463362));
#60507=CARTESIAN_POINT('Ctrl Pts',(2.93865339111066,9.59025489483843,12.5656945718778));
#60508=CARTESIAN_POINT('Ctrl Pts',(3.00780913635596,9.57660388088948,12.5646514846486));
#60509=CARTESIAN_POINT('Ctrl Pts',(3.07688618068542,9.56248072941162,12.5635577069064));
#60510=CARTESIAN_POINT('Ctrl Pts',(3.14588026881465,9.54788887725495,12.5624101605141));
#60511=CARTESIAN_POINT('Ctrl Pts',(3.18037731287926,9.54059295117661,12.5618363873179));
#60512=CARTESIAN_POINT('Ctrl Pts',(3.2148536178259,9.53317984924622,12.5612491710932));
#60513=CARTESIAN_POINT('Ctrl Pts',(3.24930865362242,9.52565000838149,12.5606481127858));
#60514=CARTESIAN_POINT('Ctrl Pts',(3.26653617152068,9.52188508794913,12.5603475836321));
#60515=CARTESIAN_POINT('Ctrl Pts',(3.28375837212493,9.51809098274095,12.5600435939036));
#60516=CARTESIAN_POINT('Ctrl Pts',(3.30097518943068,9.51426774860628,12.5597360922117));
#60517=CARTESIAN_POINT('Ctrl Pts',(3.31819200673643,9.51044451447161,12.5594285905199));
#60518=CARTESIAN_POINT('Ctrl Pts',(3.3367571155512,9.50628678066224,12.5590928276944));
#60519=CARTESIAN_POINT('Ctrl Pts',(3.3526094255081,9.50271071554887,12.5588029992888));
#60520=CARTESIAN_POINT('Ctrl Pts',(3.64533816404849,9.43667510102825,12.5534510282646));
#60521=CARTESIAN_POINT('Ctrl Pts',(3.93428895180789,9.36270676548869,12.5471205564749));
#60522=CARTESIAN_POINT('Ctrl Pts',(4.21919428495158,9.28133608325902,12.5396851351043));
#60523=CARTESIAN_POINT('Ctrl Pts',(4.37443882435552,9.23699730607876,12.5356335838285));
#60524=CARTESIAN_POINT('Ctrl Pts',(4.52848250685322,9.19045977823743,12.5312541178136));
#60525=CARTESIAN_POINT('Ctrl Pts',(4.68128396609355,9.14180323426352,12.5265273067055));
#60526=CARTESIAN_POINT('Ctrl Pts',(4.9729361761219,9.04893246815381,12.5175052403395));
#60527=CARTESIAN_POINT('Ctrl Pts',(5.26006262434337,8.94834508993225,12.5072172317331));
#60528=CARTESIAN_POINT('Ctrl Pts',(5.54249832830085,8.84059374815403,12.4955147618435));
#60529=CARTESIAN_POINT('Ctrl Pts',(5.78171086995658,8.74933236734269,12.4856032048883));
#60530=CARTESIAN_POINT('Ctrl Pts',(6.01755870886431,8.65293089162241,12.4746771936492));
#60531=CARTESIAN_POINT('Ctrl Pts',(6.24994442165545,8.55169637580964,12.4626506151949));
#60532=CARTESIAN_POINT('Origin',(-6.52772161867356,9.09517583526925,13.2547520177953));
#60533=CARTESIAN_POINT('Ctrl Pts',(-7.10353236946292,7.16066185286935,14.3526205195542));
#60534=CARTESIAN_POINT('Ctrl Pts',(-7.10420293835514,7.21308870857396,14.3262172775605));
#60535=CARTESIAN_POINT('Ctrl Pts',(-7.09563107978587,7.3705695395524,14.2497542901758));
#60536=CARTESIAN_POINT('Ctrl Pts',(-7.02933623228066,7.63362087193247,14.1357461990317));
#60537=CARTESIAN_POINT('Ctrl Pts',(-6.87564852386692,7.92504962172612,14.0308126426424));
#60538=CARTESIAN_POINT('Ctrl Pts',(-6.66239699291616,8.17291221316709,13.9642188305442));
#60539=CARTESIAN_POINT('Ctrl Pts',(-6.44555610564831,8.33500242562356,13.9425618528397));
#60540=CARTESIAN_POINT('Ctrl Pts',(-6.30450358810212,8.40710732731462,13.9457940739706));
#60541=CARTESIAN_POINT('Ctrl Pts',(-6.25443531412204,8.42901391761335,13.9488692087856));
#60542=CARTESIAN_POINT('Ctrl Pts',(-6.81826428076322,6.90434192273487,13.8358832847937));
#60543=CARTESIAN_POINT('Ctrl Pts',(-6.81886755214442,6.95065173710113,13.8125514270221));
#60544=CARTESIAN_POINT('Ctrl Pts',(-6.81115710634597,7.09004574570647,13.7449862263706));
#60545=CARTESIAN_POINT('Ctrl Pts',(-6.75126038426607,7.32369230474132,13.6446049998666));
#60546=CARTESIAN_POINT('Ctrl Pts',(-6.61252933785919,7.58258619595588,13.5532653427725));
#60547=CARTESIAN_POINT('Ctrl Pts',(-6.42074067344956,7.80223546862304,13.4965368481301));
#60548=CARTESIAN_POINT('Ctrl Pts',(-6.22677981154663,7.94527355841214,13.4793227929944));
#60549=CARTESIAN_POINT('Ctrl Pts',(-6.10129479490154,8.00867147432692,13.483096339267));
#60550=CARTESIAN_POINT('Ctrl Pts',(-6.05684383053052,8.02791388513029,13.4860821707956));
#60551=CARTESIAN_POINT('Ctrl Pts',(-7.060874166321,6.6340016482441,13.304922676125));
#60552=CARTESIAN_POINT('Ctrl Pts',(-7.06166823277956,6.69385033520045,13.2747830501599));
#60553=CARTESIAN_POINT('Ctrl Pts',(-7.05151407295871,6.87300456587821,13.187783681333));
#60554=CARTESIAN_POINT('Ctrl Pts',(-6.97381583014319,7.17088697666304,13.058513067576));
#60555=CARTESIAN_POINT('Ctrl Pts',(-6.79329978326933,7.50214854137371,12.9389604953336));
#60556=CARTESIAN_POINT('Ctrl Pts',(-6.54058076329436,7.78676910420727,12.8623986671141));
#60557=CARTESIAN_POINT('Ctrl Pts',(-6.28027246344682,7.97577465832861,12.837429458236));
#60558=CARTESIAN_POINT('Ctrl Pts',(-6.10878315575702,8.06113488688539,12.841713067788));
#60559=CARTESIAN_POINT('Ctrl Pts',(-6.04762212113882,8.08722094161854,12.845572584902));
#60560=CARTESIAN_POINT('Ctrl Pts',(-7.66738794438976,6.53159212007938,13.1170811767575));
#60561=CARTESIAN_POINT('Ctrl Pts',(-7.66850215410177,6.6154980655897,13.0748492588303));
#60562=CARTESIAN_POINT('Ctrl Pts',(-7.65424811838746,6.86542480593276,12.9532002482573));
#60563=CARTESIAN_POINT('Ctrl Pts',(-7.54656095063027,7.27782973006081,12.7720225130049));
#60564=CARTESIAN_POINT('Ctrl Pts',(-7.29571415084507,7.73752000958537,12.6014925340904));
#60565=CARTESIAN_POINT('Ctrl Pts',(-6.94078600799892,8.1364481836985,12.488785652677));
#60566=CARTESIAN_POINT('Ctrl Pts',(-6.56967193451163,8.40541915029099,12.4490985003834));
#60567=CARTESIAN_POINT('Ctrl Pts',(-6.32164837097176,8.52859001388426,12.4535176928861));
#60568=CARTESIAN_POINT('Ctrl Pts',(-6.23272511332852,8.56640925874193,12.4586246319277));
#60569=CARTESIAN_POINT('',(-6.99999992462727,8.04448113171624,12.522061793522));
#60570=CARTESIAN_POINT('Ctrl Pts',(-6.99999977388181,8.04448088283872,12.522061406121));
#60571=CARTESIAN_POINT('Ctrl Pts',(-6.97337631313135,8.07076607346233,12.5155347659721));
#60572=CARTESIAN_POINT('Ctrl Pts',(-6.94625148402719,8.09633310306438,12.5095205719456));
#60573=CARTESIAN_POINT('Ctrl Pts',(-6.91864059243224,8.12119833195497,12.5040104271219));
#60574=CARTESIAN_POINT('Ctrl Pts',(-6.87585521537613,8.15972907588304,12.4954719986143));
#60575=CARTESIAN_POINT('Ctrl Pts',(-6.83190509173913,8.19657608428999,12.488142519529));
#60576=CARTESIAN_POINT('Ctrl Pts',(-6.78684501309333,8.23178719521259,12.4819974151937));
#60577=CARTESIAN_POINT('Ctrl Pts',(-6.74178493444752,8.26699830613518,12.4758523108585));
#60578=CARTESIAN_POINT('Ctrl Pts',(-6.69561423203128,8.30057401877221,12.4708914337041));
#60579=CARTESIAN_POINT('Ctrl Pts',(-6.64834300893827,8.33253226428265,12.4671176743163));
#60580=CARTESIAN_POINT('Ctrl Pts',(-6.60338098943086,8.36292934656748,12.4635282634208));
#60581=CARTESIAN_POINT('Ctrl Pts',(-6.55744285298859,8.39185759134211,12.4610091938602));
#60582=CARTESIAN_POINT('Ctrl Pts',(-6.5104998360318,8.41930782318824,12.4595867219062));
#60583=CARTESIAN_POINT('Ctrl Pts',(-6.5032227285201,8.42356315872726,12.4593662102729));
#60584=CARTESIAN_POINT('Ctrl Pts',(-6.49592142164987,8.4277829051022,12.4591721040651));
#60585=CARTESIAN_POINT('Ctrl Pts',(-6.48859575470359,8.43196694805737,12.4590045600572));
#60586=CARTESIAN_POINT('Ctrl Pts',(-6.44205415411054,8.45854910876866,12.4579401155015));
#60587=CARTESIAN_POINT('Ctrl Pts',(-6.3945306542809,8.48369338771844,12.4579456234358));
#60588=CARTESIAN_POINT('Ctrl Pts',(-6.34600963025918,8.50736035805974,12.4590572591614));
#60589=CARTESIAN_POINT('Ctrl Pts',(-6.31441415112375,8.5227716005612,12.4597811240031));
#60590=CARTESIAN_POINT('Ctrl Pts',(-6.2823953056962,8.53755565881508,12.4609745518824));
#60591=CARTESIAN_POINT('Ctrl Pts',(-6.2499459205233,8.55169191683731,12.4626538271208));
#60592=CARTESIAN_POINT('',(-6.9999915801407,6.97712494714797,13.9487134680504));
#60593=CARTESIAN_POINT('Ctrl Pts',(-6.99999158015451,6.9771362153215,13.9487146197636));
#60594=CARTESIAN_POINT('Ctrl Pts',(-6.99999158015451,6.98139583880415,13.9388762305162));
#60595=CARTESIAN_POINT('Ctrl Pts',(-7.,6.98228449209442,13.9352913921393));
#60596=CARTESIAN_POINT('Ctrl Pts',(-7.,6.9971931901372,13.9030475786216));
#60597=CARTESIAN_POINT('Ctrl Pts',(-7.00000000000326,7.03259754383002,13.8211717575672));
#60598=CARTESIAN_POINT('Ctrl Pts',(-7.00000000000326,7.11638182264416,13.6465448627553));
#60599=CARTESIAN_POINT('Ctrl Pts',(-7.,7.15192570282134,13.5765007476151));
#60600=CARTESIAN_POINT('Ctrl Pts',(-7.,7.26853858730711,13.3617723992316));
#60601=CARTESIAN_POINT('Ctrl Pts',(-7.,7.35673215220611,13.2193982896567));
#60602=CARTESIAN_POINT('Ctrl Pts',(-7.,7.66322934186235,12.8078043924259));
#60603=CARTESIAN_POINT('Ctrl Pts',(-7.,7.86763429655534,12.6356713199051));
#60604=CARTESIAN_POINT('Ctrl Pts',(-7.,8.04448084282976,12.5220613438382));
#60605=CARTESIAN_POINT('Ctrl Pts',(-6.9999915801407,6.97712494714797,13.9487134680504));
#60606=CARTESIAN_POINT('Ctrl Pts',(-6.99999179357842,7.02345511516882,13.9416137324713));
#60607=CARTESIAN_POINT('Ctrl Pts',(-6.99820050635823,7.06895925542468,13.9350275981178));
#60608=CARTESIAN_POINT('Ctrl Pts',(-6.99484214212171,7.11344412994376,13.9289647197009));
#60609=CARTESIAN_POINT('Ctrl Pts',(-6.99412245220856,7.12297713864213,13.9276654584731));
#60610=CARTESIAN_POINT('Ctrl Pts',(-6.99333067941413,7.13246348909142,13.9263902088819));
#60611=CARTESIAN_POINT('Ctrl Pts',(-6.99246885265765,7.14190152098239,13.925139034573));
#60612=CARTESIAN_POINT('Ctrl Pts',(-6.98828270432694,7.18774484291289,13.9190617096289));
#60613=CARTESIAN_POINT('Ctrl Pts',(-6.98244713497531,7.23244547821124,13.9135524609592));
#60614=CARTESIAN_POINT('Ctrl Pts',(-6.97524064834229,7.27587635862952,13.908587731437));
#60615=CARTESIAN_POINT('Ctrl Pts',(-6.96767039519366,7.3214995278626,13.9033723940317));
#60616=CARTESIAN_POINT('Ctrl Pts',(-6.95858694743669,7.3657214505831,13.8987580531846));
#60617=CARTESIAN_POINT('Ctrl Pts',(-6.9482703839507,7.40843320711306,13.8947152622816));
#60618=CARTESIAN_POINT('Ctrl Pts',(-6.94468364742794,7.42328270785089,13.8933097142223));
#60619=CARTESIAN_POINT('Ctrl Pts',(-6.9409475238705,7.43795000162698,13.8919732243342));
#60620=CARTESIAN_POINT('Ctrl Pts',(-6.93707278116213,7.45243154331358,13.8907044581386));
#60621=CARTESIAN_POINT('Ctrl Pts',(-6.93345734647906,7.46594394194718,13.8895206011308));
#60622=CARTESIAN_POINT('Ctrl Pts',(-6.92972121451281,7.47929463244384,13.8883956974777));
#60623=CARTESIAN_POINT('Ctrl Pts',(-6.92587277883775,7.49248113455884,13.8873286131981));
#60624=CARTESIAN_POINT('Ctrl Pts',(-6.91348381119123,7.53493140834987,13.8838934323268));
#60625=CARTESIAN_POINT('Ctrl Pts',(-6.89993442942445,7.57567800006318,13.8810573272698));
#60626=CARTESIAN_POINT('Ctrl Pts',(-6.88552314565712,7.61468928798206,13.8787588902026));
#60627=CARTESIAN_POINT('Ctrl Pts',(-6.87043421251612,7.65553497006394,13.8763523757105));
#60628=CARTESIAN_POINT('Ctrl Pts',(-6.8544001109962,7.69447831442104,13.8745353972937));
#60629=CARTESIAN_POINT('Ctrl Pts',(-6.83771752002407,7.73151542393473,13.8732375782579));
#60630=CARTESIAN_POINT('Ctrl Pts',(-6.83626070142977,7.73474971469382,13.8731242453285));
#60631=CARTESIAN_POINT('Ctrl Pts',(-6.83479891154535,7.73796948843846,13.8730148708164));
#60632=CARTESIAN_POINT('Ctrl Pts',(-6.83333233337493,7.74117475359548,13.8729094074551));
#60633=CARTESIAN_POINT('Ctrl Pts',(-6.82678505896167,7.75548408328111,13.8724385852504));
#60634=CARTESIAN_POINT('Ctrl Pts',(-6.82014241935267,7.76950420249532,13.8720457161995));
#60635=CARTESIAN_POINT('Ctrl Pts',(-6.81342017547794,7.78323627338698,13.8717265688566));
#60636=CARTESIAN_POINT('Ctrl Pts',(-6.81005905354057,7.79010230883282,13.8715669951852));
#60637=CARTESIAN_POINT('Ctrl Pts',(-6.80667802550112,7.7968963297535,13.8714258546653));
#60638=CARTESIAN_POINT('Ctrl Pts',(-6.80327897382311,7.80361856091292,13.8713026089469));
#60639=CARTESIAN_POINT('Ctrl Pts',(-6.8010541405342,7.80801856570131,13.8712219390415));
#60640=CARTESIAN_POINT('Ctrl Pts',(-6.79917315425435,7.81170206754556,13.8711605766567));
#60641=CARTESIAN_POINT('Ctrl Pts',(-6.79694806932509,7.81601686256903,13.8710945194426));
#60642=CARTESIAN_POINT('Ctrl Pts',(-6.79667926136544,7.81653812413135,13.8710865392056));
#60643=CARTESIAN_POINT('Ctrl Pts',(-6.79640538380907,7.81706856956299,13.8710785155005));
#60644=CARTESIAN_POINT('Ctrl Pts',(-6.79612518284729,7.81761054962054,13.8710704276006));
#60645=CARTESIAN_POINT('Ctrl Pts',(-6.79518125958311,7.81943633773277,13.8710431815956));
#60646=CARTESIAN_POINT('Ctrl Pts',(-6.79416569539586,7.82139310245855,13.8710151428786));
#60647=CARTESIAN_POINT('Ctrl Pts',(-6.79302961569968,7.8235701075631,13.8709860233455));
#60648=CARTESIAN_POINT('Ctrl Pts',(-6.76368963094169,7.87979265673828,13.8702339927812));
#60649=CARTESIAN_POINT('Ctrl Pts',(-6.73182093305379,7.93345140989508,13.8707651590374));
#60650=CARTESIAN_POINT('Ctrl Pts',(-6.69787436544692,7.98430705174562,13.8725913407545));
#60651=CARTESIAN_POINT('Ctrl Pts',(-6.67085582426605,8.02478375824305,13.8740448239607));
#60652=CARTESIAN_POINT('Ctrl Pts',(-6.64251966059964,8.06348488349544,13.8763192220685));
#60653=CARTESIAN_POINT('Ctrl Pts',(-6.6130719875628,8.10029601588777,13.8794277946745));
#60654=CARTESIAN_POINT('Ctrl Pts',(-6.57434521287239,8.14870651095385,13.8835158932748));
#60655=CARTESIAN_POINT('Ctrl Pts',(-6.53369822918461,8.19384839995991,13.8890457406106));
#60656=CARTESIAN_POINT('Ctrl Pts',(-6.49166404576566,8.23557412981306,13.8959769055419));
#60657=CARTESIAN_POINT('Ctrl Pts',(-6.45807128302675,8.26892038348224,13.9015161348096));
#60658=CARTESIAN_POINT('Ctrl Pts',(-6.42359132347886,8.30008482318858,13.9079509341316));
#60659=CARTESIAN_POINT('Ctrl Pts',(-6.38847438568453,8.32899839343566,13.9152673758578));
#60660=CARTESIAN_POINT('Ctrl Pts',(-6.3476522735808,8.36260932536996,13.9237724626651));
#60661=CARTESIAN_POINT('Ctrl Pts',(-6.30597044168472,8.39317911113965,13.9334683683526));
#60662=CARTESIAN_POINT('Ctrl Pts',(-6.26385540534517,8.42069809212293,13.9442719314227));
#60663=CARTESIAN_POINT('Ctrl Pts',(-6.22266933631966,7.49367505102186,13.1134072735229));
#60664=CARTESIAN_POINT('Ctrl Pts',(-6.22400486673781,7.81349730664259,13.3673816679581));
#60665=CARTESIAN_POINT('Ctrl Pts',(-6.22726445118346,8.61699336812186,14.0755188055406));
#60666=CARTESIAN_POINT('Ctrl Pts',(-6.23205297895451,9.75631511884638,15.3875857998101));
#60667=CARTESIAN_POINT('Ctrl Pts',(-6.23570680591364,10.7961444652413,17.0892590921569));
#60668=CARTESIAN_POINT('Ctrl Pts',(-6.23759597390816,11.541637417471,18.9411614085076));
#60669=CARTESIAN_POINT('Ctrl Pts',(-6.23804316716047,11.9701365581257,20.8893410093233));
#60670=CARTESIAN_POINT('Ctrl Pts',(-6.23649631643492,12.0627638071392,22.7260240074032));
#60671=CARTESIAN_POINT('Ctrl Pts',(-6.23490853076659,11.9504777429291,23.892461951891));
#60672=CARTESIAN_POINT('Ctrl Pts',(-6.23413323858226,11.8700330549955,24.3933787302679));
#60673=CARTESIAN_POINT('Ctrl Pts',(-6.71589075887148,7.42368503417367,13.2016810446589));
#60674=CARTESIAN_POINT('Ctrl Pts',(-6.71707947563242,7.74006436636922,13.453789394194));
#60675=CARTESIAN_POINT('Ctrl Pts',(-6.71993400051002,8.53485728885363,14.1564673243464));
#60676=CARTESIAN_POINT('Ctrl Pts',(-6.72416485221413,9.66125417255672,15.4573970130228));
#60677=CARTESIAN_POINT('Ctrl Pts',(-6.72736852339175,10.689155926356,17.143170277743));
#60678=CARTESIAN_POINT('Ctrl Pts',(-6.72902457707724,11.426258395907,18.9767998262514));
#60679=CARTESIAN_POINT('Ctrl Pts',(-6.72941957129847,11.8502298588172,20.9054834886988));
#60680=CARTESIAN_POINT('Ctrl Pts',(-6.72805203821864,11.9427120051071,22.7235306556374));
#60681=CARTESIAN_POINT('Ctrl Pts',(-6.72668376548171,11.8323442369596,23.8785262234885));
#60682=CARTESIAN_POINT('Ctrl Pts',(-6.72599062030542,11.7530859526059,24.3745538120327));
#60683=CARTESIAN_POINT('Ctrl Pts',(-7.02184862101457,7.17355760292472,13.5171491223171));
#60684=CARTESIAN_POINT('Ctrl Pts',(-7.02249157348648,7.478872844128,13.7610241429803));
#60685=CARTESIAN_POINT('Ctrl Pts',(-7.02397823406739,8.24599459896698,14.440704212245));
#60686=CARTESIAN_POINT('Ctrl Pts',(-7.0262282722894,9.33267229285362,15.6982356777953));
#60687=CARTESIAN_POINT('Ctrl Pts',(-7.02790162445773,10.3242143997312,17.3268265378416));
#60688=CARTESIAN_POINT('Ctrl Pts',(-7.0287661637212,11.0353397613724,19.0974453756984));
#60689=CARTESIAN_POINT('Ctrl Pts',(-7.028976081938,11.4446321919501,20.9601377844438));
#60690=CARTESIAN_POINT('Ctrl Pts',(-7.02824777989815,11.5344315703546,22.71520034539));
#60691=CARTESIAN_POINT('Ctrl Pts',(-7.02756283605818,11.4283603739875,23.8309174838911));
#60692=CARTESIAN_POINT('Ctrl Pts',(-7.02718415215858,11.3520777791479,24.3100040794306));
#60693=CARTESIAN_POINT('Ctrl Pts',(-6.99898915856098,6.85988137547321,13.9127665107488));
#60694=CARTESIAN_POINT('Ctrl Pts',(-6.99894180138027,7.1516676167299,14.1458797488553));
#60695=CARTESIAN_POINT('Ctrl Pts',(-6.99873531965576,7.88504568030388,14.7957455291437));
#60696=CARTESIAN_POINT('Ctrl Pts',(-6.99850468872881,8.92371894485393,15.9978491112633));
#60697=CARTESIAN_POINT('Ctrl Pts',(-6.99828080920108,9.87141264267925,17.5546291349416));
#60698=CARTESIAN_POINT('Ctrl Pts',(-6.99816434195365,10.5510797273584,19.2468680102348));
#60699=CARTESIAN_POINT('Ctrl Pts',(-6.99814257317328,10.9423828246477,21.0278308117662));
#60700=CARTESIAN_POINT('Ctrl Pts',(-6.99821546035646,11.0282138258093,22.7049155532659));
#60701=CARTESIAN_POINT('Ctrl Pts',(-6.99835922374124,10.9268166315182,23.7718253761471));
#60702=CARTESIAN_POINT('Ctrl Pts',(-6.99838072450059,10.8539129115264,24.2298152719421));
#60703=CARTESIAN_POINT('',(-7.00000355776417,10.9277699389974,24.1259406808918));
#60704=CARTESIAN_POINT('Ctrl Pts',(-7.00001601640884,6.97712293922472,13.9487170608442));
#60705=CARTESIAN_POINT('Ctrl Pts',(-7.00002088952752,7.14853164172674,14.0875671114257));
#60706=CARTESIAN_POINT('Ctrl Pts',(-7.000015982516,7.31421700914964,14.2303325311141));
#60707=CARTESIAN_POINT('Ctrl Pts',(-7.00000988103554,7.47407638767217,14.376420366171));
#60708=CARTESIAN_POINT('Ctrl Pts',(-7.00000652429656,7.56202327378949,14.4567908161979));
#60709=CARTESIAN_POINT('Ctrl Pts',(-7.00000279079959,7.64820743489774,14.5381675622895));
#60710=CARTESIAN_POINT('Ctrl Pts',(-6.99999999965548,7.73261611072525,14.6204569781481));
#60711=CARTESIAN_POINT('Ctrl Pts',(-6.99999455428923,7.89729272255631,14.7809990321527));
#60712=CARTESIAN_POINT('Ctrl Pts',(-6.99999266088549,8.05521000034952,14.9450123533677));
#60713=CARTESIAN_POINT('Ctrl Pts',(-6.99999257352085,8.20639703738741,15.1118865720018));
#60714=CARTESIAN_POINT('Ctrl Pts',(-6.99999248489117,8.35977324988939,15.281177115158));
#60715=CARTESIAN_POINT('Ctrl Pts',(-6.99999425322672,8.50622295743612,15.4534120257722));
#60716=CARTESIAN_POINT('Ctrl Pts',(-6.99999619758808,8.64580647529293,15.6279989379776));
#60717=CARTESIAN_POINT('Ctrl Pts',(-6.9999975442515,8.74248192916988,15.7489177200629));
#60718=CARTESIAN_POINT('Ctrl Pts',(-6.99999897835711,8.83586434207461,15.870965684437));
#60719=CARTESIAN_POINT('Ctrl Pts',(-6.99999998662364,8.92598174885412,15.9939582552016));
#60720=CARTESIAN_POINT('Ctrl Pts',(-7.0000014370777,9.05562123868325,16.1708907113886));
#60721=CARTESIAN_POINT('Ctrl Pts',(-7.00000201440511,9.17850354164596,16.3497755201176));
#60722=CARTESIAN_POINT('Ctrl Pts',(-7.0000021087437,9.29479363545964,16.5300313754151));
#60723=CARTESIAN_POINT('Ctrl Pts',(-7.00000220459648,9.41295025611371,16.7131804469875));
#60724=CARTESIAN_POINT('Ctrl Pts',(-7.00000180216161,9.52430140158153,16.8977449605128));
#60725=CARTESIAN_POINT('Ctrl Pts',(-7.00000129011683,9.62903794576636,17.0831664637562));
#60726=CARTESIAN_POINT('Ctrl Pts',(-7.00000086166955,9.71667498162649,17.2383156626862));
#60727=CARTESIAN_POINT('Ctrl Pts',(-7.00000035619204,9.79968127750393,17.3940658191389));
#60728=CARTESIAN_POINT('Ctrl Pts',(-6.99999998816694,9.87817756458936,17.5501163157672));
#60729=CARTESIAN_POINT('Ctrl Pts',(-6.99999970373616,9.93884396874961,17.6707210328739));
#60730=CARTESIAN_POINT('Ctrl Pts',(-6.99999950020192,9.99681674665053,17.7915056337493));
#60731=CARTESIAN_POINT('Ctrl Pts',(-6.99999936067802,10.0521635248232,17.9123401859273));
#60732=CARTESIAN_POINT('Ctrl Pts',(-6.99999924479307,10.0981331255442,18.0127022359021));
#60733=CARTESIAN_POINT('Ctrl Pts',(-6.99999917321886,10.142291206268,18.1130988977463));
#60734=CARTESIAN_POINT('Ctrl Pts',(-6.99999913936912,10.1846774087402,18.2134599710767));
#60735=CARTESIAN_POINT('Ctrl Pts',(-6.99999912244425,10.2058705099763,18.2636405077418));
#60736=CARTESIAN_POINT('Ctrl Pts',(-6.99999911499185,10.2266206416495,18.3138121472786));
#60737=CARTESIAN_POINT('Ctrl Pts',(-6.99999911640488,10.246932844701,18.3639665348978));
#60738=CARTESIAN_POINT('Ctrl Pts',(-6.9999991171114,10.2570889462268,18.3890437287075));
#60739=CARTESIAN_POINT('Ctrl Pts',(-6.99999912003648,10.2671355655972,18.4141166095378));
#60740=CARTESIAN_POINT('Ctrl Pts',(-6.99999912511644,10.2770733350148,18.4391841440791));
#60741=CARTESIAN_POINT('Ctrl Pts',(-6.99999912765642,10.2820422197236,18.4517179113498));
#60742=CARTESIAN_POINT('Ctrl Pts',(-6.99999913073525,10.2869838919442,18.4642503420482));
#60743=CARTESIAN_POINT('Ctrl Pts',(-6.99999913434566,10.291898430994,18.4767813084774));
#60744=CARTESIAN_POINT('Ctrl Pts',(-6.99999913750188,10.296194727389,18.48773589554));
#60745=CARTESIAN_POINT('Ctrl Pts',(-6.99999914057233,10.2999248874935,18.4972873011398));
#60746=CARTESIAN_POINT('Ctrl Pts',(-6.99999914483751,10.3045195539668,18.5091124088053));
#60747=CARTESIAN_POINT('Ctrl Pts',(-6.99999914545128,10.3051807324653,18.5108140572221));
#60748=CARTESIAN_POINT('Ctrl Pts',(-6.99999914609173,10.305859732172,18.5125628199288));
#60749=CARTESIAN_POINT('Ctrl Pts',(-6.9999991467648,10.3065607280344,18.514369687696));
#60750=CARTESIAN_POINT('Ctrl Pts',(-6.99999923697471,10.4005130113583,18.7565385241931));
#60751=CARTESIAN_POINT('Ctrl Pts',(-6.99999952144554,10.4851674501396,19.00016538121));
#60752=CARTESIAN_POINT('Ctrl Pts',(-6.99999999018483,10.5606734143179,19.2445368434734));
#60753=CARTESIAN_POINT('Ctrl Pts',(-7.0000004436457,10.6337182819468,19.4809430837961));
#60754=CARTESIAN_POINT('Ctrl Pts',(-7.00000106797418,10.698202212125,19.7180460706751));
#60755=CARTESIAN_POINT('Ctrl Pts',(-7.00000142593608,10.7543697313658,19.9551865164325));
#60756=CARTESIAN_POINT('Ctrl Pts',(-7.00000178766141,10.8111277673616,20.19482013633));
#60757=CARTESIAN_POINT('Ctrl Pts',(-7.00000187627638,10.8593936259894,20.4344920434748));
#60758=CARTESIAN_POINT('Ctrl Pts',(-7.00000131558951,10.8994259328862,20.6735748933678));
#60759=CARTESIAN_POINT('Ctrl Pts',(-7.0000010387301,10.9191933315174,20.7916306929476));
#60760=CARTESIAN_POINT('Ctrl Pts',(-7.00000060480743,10.9369532806506,20.9095436715295));
#60761=CARTESIAN_POINT('Ctrl Pts',(-6.99999997635849,10.9527374502756,21.0272429376326));
#60762=CARTESIAN_POINT('Ctrl Pts',(-6.99999887928608,10.980291601027,21.2327085020917));
#60763=CARTESIAN_POINT('Ctrl Pts',(-6.99999719588076,11.0018249275505,21.4375214622287));
#60764=CARTESIAN_POINT('Ctrl Pts',(-6.99999590265571,11.0175572494836,21.6413537925878));
#60765=CARTESIAN_POINT('Ctrl Pts',(-6.99999568173169,11.0202448310013,21.6761748448211));
#60766=CARTESIAN_POINT('Ctrl Pts',(-6.99999546003708,11.0229065683484,21.7128796154196));
#60767=CARTESIAN_POINT('Ctrl Pts',(-6.99999525389955,11.0254108669411,21.75013794005));
#60768=CARTESIAN_POINT('Ctrl Pts',(-6.99999512031371,11.0270337583356,21.7742829100596));
#60769=CARTESIAN_POINT('Ctrl Pts',(-6.99999499325482,11.0285915187921,21.7986602554154));
#60770=CARTESIAN_POINT('Ctrl Pts',(-6.99999487632675,11.0300601216929,21.8229070746112));
#60771=CARTESIAN_POINT('Ctrl Pts',(-6.9999945789659,11.0337949391971,21.8845693828506));
#60772=CARTESIAN_POINT('Ctrl Pts',(-6.99999434329384,11.0369990612,21.9460662528043));
#60773=CARTESIAN_POINT('Ctrl Pts',(-6.9999941942213,11.0396820511593,22.0073884345677));
#60774=CARTESIAN_POINT('Ctrl Pts',(-6.99999365475384,11.0493913227684,22.229302689719));
#60775=CARTESIAN_POINT('Ctrl Pts',(-6.9999942620196,11.0522757640116,22.4489301954425));
#60776=CARTESIAN_POINT('Ctrl Pts',(-6.99999708882545,11.0487792507388,22.6658974333243));
#60777=CARTESIAN_POINT('Ctrl Pts',(-6.99999738657601,11.0484109591607,22.6887508304715));
#60778=CARTESIAN_POINT('Ctrl Pts',(-6.99999770879879,11.0479718662955,22.7115747599508));
#60779=CARTESIAN_POINT('Ctrl Pts',(-6.99999805663954,11.0474624859708,22.7343688182385));
#60780=CARTESIAN_POINT('Ctrl Pts',(-6.9999986310883,11.0466212593786,22.7720125336482));
#60781=CARTESIAN_POINT('Ctrl Pts',(-6.9999992754144,11.0455883341832,22.809574777292));
#60782=CARTESIAN_POINT('Ctrl Pts',(-6.99999999465564,11.0443660188271,22.8470537692267));
#60783=CARTESIAN_POINT('Ctrl Pts',(-7.00000393353128,11.0376720921033,23.052304913658));
#60784=CARTESIAN_POINT('Ctrl Pts',(-7.00001006487307,11.025299318151,23.2550551439592));
#60785=CARTESIAN_POINT('Ctrl Pts',(-7.00001375756393,11.0076804835671,23.4549606777513));
#60786=CARTESIAN_POINT('Ctrl Pts',(-7.000017504741,10.9898016804802,23.6578158471807));
#60787=CARTESIAN_POINT('Ctrl Pts',(-7.00001874207249,10.9665208779502,23.8577418328988));
#60788=CARTESIAN_POINT('Ctrl Pts',(-7.00001328549311,10.938274975984,24.0544306054433));
#60789=CARTESIAN_POINT('Ctrl Pts',(-7.00001262288882,10.9348450147417,24.0783149504158));
#60790=CARTESIAN_POINT('Ctrl Pts',(-7.00001186234527,10.9313418208076,24.1021516203976));
#60791=CARTESIAN_POINT('Ctrl Pts',(-7.00001099700083,10.9277661612326,24.1259401133248));
#60792=CARTESIAN_POINT('Origin',(-5.99998362341993,10.9277594518961,24.125947303705));
#60793=CARTESIAN_POINT('Origin',(-5.999994993362,10.9277770074801,24.1259380195517));
#60794=CARTESIAN_POINT('Origin',(-6.,10.9277790634077,24.125942705097));
#60795=CARTESIAN_POINT('Ctrl Pts',(-5.9884183442854,11.3313022292381,25.0408390360803));
#60796=CARTESIAN_POINT('Ctrl Pts',(-5.98810619593714,11.2108096660665,25.0939098183863));
#60797=CARTESIAN_POINT('Ctrl Pts',(-5.98726411407663,10.7897530180886,25.2768810270768));
#60798=CARTESIAN_POINT('Ctrl Pts',(-5.98726411407568,10.2439464472041,25.5029615111316));
#60799=CARTESIAN_POINT('Ctrl Pts',(-5.98810619595882,9.81683424998038,25.6713133410833));
#60800=CARTESIAN_POINT('Ctrl Pts',(-5.98841834432643,9.69410642640033,25.7189877414102));
#60801=CARTESIAN_POINT('Ctrl Pts',(-6.58019637256003,11.3340652231778,25.047111700226));
#60802=CARTESIAN_POINT('Ctrl Pts',(-6.5798820750521,11.2136264141743,25.1003606676502));
#60803=CARTESIAN_POINT('Ctrl Pts',(-6.57903382472758,10.7926924751956,25.2838219693725));
#60804=CARTESIAN_POINT('Ctrl Pts',(-6.57903382472674,10.2467759245194,25.5099480085486));
#60805=CARTESIAN_POINT('Ctrl Pts',(-6.57988207507353,9.81940394754026,25.6778665220155));
#60806=CARTESIAN_POINT('Ctrl Pts',(-6.58019637260084,9.69658813799417,25.7253769164937));
#60807=CARTESIAN_POINT('Ctrl Pts',(-7.00079676143853,11.1662377150805,24.6661026672652));
#60808=CARTESIAN_POINT('Ctrl Pts',(-7.00061242393279,11.0471100806974,24.7189175646936));
#60809=CARTESIAN_POINT('Ctrl Pts',(-7.00011450599634,10.6307098582429,24.9007951477761));
#60810=CARTESIAN_POINT('Ctrl Pts',(-7.0001145059963,10.0904740685619,25.1245681387042));
#60811=CARTESIAN_POINT('Ctrl Pts',(-7.00061242394545,9.66742777151116,25.290400688646));
#60812=CARTESIAN_POINT('Ctrl Pts',(-7.00079676146261,9.54584603631305,25.3372908764602));
#60813=CARTESIAN_POINT('Ctrl Pts',(-6.99999917328613,10.927678046055,24.1245145225457));
#60814=CARTESIAN_POINT('Ctrl Pts',(-6.99999957798843,10.8103388551858,24.1765413802751));
#60815=CARTESIAN_POINT('Ctrl Pts',(-7.00000004346175,10.4001857821127,24.3557037853022));
#60816=CARTESIAN_POINT('Ctrl Pts',(-7.00000004346256,9.86804140738225,24.576125202425));
#60817=CARTESIAN_POINT('Ctrl Pts',(-6.99999957798869,9.45133243288797,24.7394602714692));
#60818=CARTESIAN_POINT('Ctrl Pts',(-6.99999917328596,9.33157254651437,24.7856430669351));
#60819=CARTESIAN_POINT('',(-7.00000356386834,9.33251602085003,24.7867164879855));
#60820=CARTESIAN_POINT('Origin',(-6.,9.33251101143585,24.7867243678371));
#60821=CARTESIAN_POINT('Origin',(-7.0002107682112,-4.74293616361314,-11.4504608650742));
#60822=CARTESIAN_POINT('Origin',(-5.999994980806,9.33250914740904,24.7867195890732));
#60823=CARTESIAN_POINT('Origin',(-5.99998370354292,9.33252808467289,24.7867138043456));
#60824=CARTESIAN_POINT('Ctrl Pts',(-6.23412989340402,8.85535213519231,25.6421122842036));
#60825=CARTESIAN_POINT('Ctrl Pts',(-6.23490519370591,8.44426394556272,25.3447917122089));
#60826=CARTESIAN_POINT('Ctrl Pts',(-6.23649298896613,7.54006566407591,24.5993912594835));
#60827=CARTESIAN_POINT('Ctrl Pts',(-6.23803984395223,6.30682932830241,23.2351599451));
#60828=CARTESIAN_POINT('Ctrl Pts',(-6.2375926509193,5.23225286032833,21.5545941421788));
#60829=CARTESIAN_POINT('Ctrl Pts',(-6.23570347947279,4.44990325945585,19.7179581728001));
#60830=CARTESIAN_POINT('Ctrl Pts',(-6.23204965637528,3.98190889009471,17.7794230915657));
#60831=CARTESIAN_POINT('Ctrl Pts',(-6.22726110625498,3.8597596825099,16.0460302370417));
#60832=CARTESIAN_POINT('Ctrl Pts',(-6.22400156292249,3.92718833567129,14.9771464147955));
#60833=CARTESIAN_POINT('Ctrl Pts',(-6.22266603698934,3.9737495101578,14.5714122610983));
#60834=CARTESIAN_POINT('Ctrl Pts',(-6.72598994962541,8.92473422419825,25.5461078251555));
#60835=CARTESIAN_POINT('Ctrl Pts',(-6.7266831066965,8.51794212602247,25.2514055028052));
#60836=CARTESIAN_POINT('Ctrl Pts',(-6.7280513688563,7.62319122749838,24.5127395435205));
#60837=CARTESIAN_POINT('Ctrl Pts',(-6.72941891797283,6.40302972279236,23.1617882479885));
#60838=CARTESIAN_POINT('Ctrl Pts',(-6.72902392012398,5.33903731288351,21.4982095508128));
#60839=CARTESIAN_POINT('Ctrl Pts',(-6.7273678628286,4.56367546252717,19.6804271754057));
#60840=CARTESIAN_POINT('Ctrl Pts',(-6.72416418641298,4.09848997856963,17.7615690069914));
#60841=CARTESIAN_POINT('Ctrl Pts',(-6.71993332126113,3.97507673802481,16.0451905115539));
#60842=CARTESIAN_POINT('Ctrl Pts',(-6.71707880685382,4.04021160935505,14.9863208404887));
#60843=CARTESIAN_POINT('Ctrl Pts',(-6.71589008825079,4.08565776872657,14.5843406421682));
#60844=CARTESIAN_POINT('Ctrl Pts',(-7.02718522642081,9.16264689799124,25.2169070753993));
#60845=CARTESIAN_POINT('Ctrl Pts',(-7.02756392064403,8.76993819821337,24.9320798125953));
#60846=CARTESIAN_POINT('Ctrl Pts',(-7.02824883165012,7.90599974588617,24.2181499613082));
#60847=CARTESIAN_POINT('Ctrl Pts',(-7.02897715373606,6.7284783391173,22.9136327893854));
#60848=CARTESIAN_POINT('Ctrl Pts',(-7.02876722992311,5.70076930069521,21.3070968357706));
#60849=CARTESIAN_POINT('Ctrl Pts',(-7.02790269246911,4.95159426737389,19.5522386119276));
#60850=CARTESIAN_POINT('Ctrl Pts',(-7.02622933538481,4.50113275642416,17.6995249184679));
#60851=CARTESIAN_POINT('Ctrl Pts',(-7.02397930905116,4.38032098780939,16.0419195542338));
#60852=CARTESIAN_POINT('Ctrl Pts',(-7.02249262973376,4.44215133384606,15.0188783064057));
#60853=CARTESIAN_POINT('Ctrl Pts',(-7.02184967226858,4.48559584516257,14.6305434540714));
#60854=CARTESIAN_POINT('Ctrl Pts',(-6.99838062538608,9.45820155481245,24.8079470509315));
#60855=CARTESIAN_POINT('Ctrl Pts',(-6.99835912980461,9.08279992667889,24.5356483167704));
#60856=CARTESIAN_POINT('Ctrl Pts',(-6.99821532184398,8.2566788241358,23.8529257033659));
#60857=CARTESIAN_POINT('Ctrl Pts',(-6.99814245121138,7.1314903406498,22.6063536230413));
#60858=CARTESIAN_POINT('Ctrl Pts',(-6.9981642146033,6.1488526955293,21.0703299396964));
#60859=CARTESIAN_POINT('Ctrl Pts',(-6.9982806895177,5.43285646000756,19.3931394441194));
#60860=CARTESIAN_POINT('Ctrl Pts',(-6.99850456865247,5.00216746505037,17.6222095472215));
#60861=CARTESIAN_POINT('Ctrl Pts',(-6.9987352349114,4.88660490348886,16.0377422203896));
#60862=CARTESIAN_POINT('Ctrl Pts',(-6.99894167917053,4.94565673237532,15.0596432877823));
#60863=CARTESIAN_POINT('Ctrl Pts',(-6.99898903104342,4.98714453063266,14.6884846342227));
#60864=CARTESIAN_POINT('',(-7.,4.92966193692261,14.7967990234135));
#60865=CARTESIAN_POINT('Ctrl Pts',(-7.00001101651645,9.33251828728899,24.7867134201296));
#60866=CARTESIAN_POINT('Ctrl Pts',(-7.00001786894295,9.17931983979782,24.6735516965421));
#60867=CARTESIAN_POINT('Ctrl Pts',(-7.00001802523628,9.03120918194217,24.5580124632972));
#60868=CARTESIAN_POINT('Ctrl Pts',(-7.00001556833393,8.88816179628229,24.4406082397738));
#60869=CARTESIAN_POINT('Ctrl Pts',(-7.00001306404844,8.74235563775587,24.3209397904152));
#60870=CARTESIAN_POINT('Ctrl Pts',(-7.0000078433619,8.60180983017618,24.1993336963811));
#60871=CARTESIAN_POINT('Ctrl Pts',(-7.00000354817398,8.4664648926225,24.0762902302008));
#60872=CARTESIAN_POINT('Ctrl Pts',(-7.00000225617386,8.42575289619948,24.0392785381084));
#60873=CARTESIAN_POINT('Ctrl Pts',(-7.00000104339817,8.38551126318123,24.0021365051628));
#60874=CARTESIAN_POINT('Ctrl Pts',(-6.99999999753967,8.34573781976912,23.964877022));
#60875=CARTESIAN_POINT('Ctrl Pts',(-6.99999887667098,8.30311177925403,23.9249452458545));
#60876=CARTESIAN_POINT('Ctrl Pts',(-6.99999794691815,8.26102348599585,23.8848785705131));
#60877=CARTESIAN_POINT('Ctrl Pts',(-6.99999718088437,8.21946771151489,23.8446921506738));
#60878=CARTESIAN_POINT('Ctrl Pts',(-6.99999462213106,8.08066055039311,23.7104589923891));
#60879=CARTESIAN_POINT('Ctrl Pts',(-6.99999387749955,7.94779642121724,23.5748934964743));
#60880=CARTESIAN_POINT('Ctrl Pts',(-6.99999403436534,7.82066688325193,23.4385283478739));
#60881=CARTESIAN_POINT('Ctrl Pts',(-6.99999406718762,7.79406655336375,23.409995577315));
#60882=CARTESIAN_POINT('Ctrl Pts',(-6.99999414005197,7.76771721764197,23.3814276290268));
#60883=CARTESIAN_POINT('Ctrl Pts',(-6.99999424550222,7.74161685943437,23.352829118262));
#60884=CARTESIAN_POINT('Ctrl Pts',(-6.99999432423845,7.72212858259807,23.3314755532857));
#60885=CARTESIAN_POINT('Ctrl Pts',(-6.99999441864875,7.70323903377222,23.3106151007504));
#60886=CARTESIAN_POINT('Ctrl Pts',(-6.9999945314086,7.68388235950719,23.2890695977729));
#60887=CARTESIAN_POINT('Ctrl Pts',(-6.99999463684072,7.66578358463525,23.2689242358912));
#60888=CARTESIAN_POINT('Ctrl Pts',(-6.99999475849199,7.64727647773833,23.2481798529943));
#60889=CARTESIAN_POINT('Ctrl Pts',(-6.99999490352853,7.62752043826751,23.2258462258222));
#60890=CARTESIAN_POINT('Ctrl Pts',(-6.99999520368191,7.58663527688044,23.1796267417684));
#60891=CARTESIAN_POINT('Ctrl Pts',(-6.99999556267868,7.54621521311681,23.1331494749869));
#60892=CARTESIAN_POINT('Ctrl Pts',(-6.99999595372411,7.50626134984804,23.0864242861152));
#60893=CARTESIAN_POINT('Ctrl Pts',(-6.99999673581497,7.42635362331049,22.992973908372));
#60894=CARTESIAN_POINT('Ctrl Pts',(-6.99999764539642,7.34831069875224,22.8985318422683));
#60895=CARTESIAN_POINT('Ctrl Pts',(-6.99999847634406,7.27213982922329,22.8031748296488));
#60896=CARTESIAN_POINT('Ctrl Pts',(-6.99999902467282,7.22187591795764,22.7402502962871));
#60897=CARTESIAN_POINT('Ctrl Pts',(-6.99999953898546,7.17242715196673,22.6769273058003));
#60898=CARTESIAN_POINT('Ctrl Pts',(-6.99999996276665,7.12379521756591,22.6132273646642));
#60899=CARTESIAN_POINT('Ctrl Pts',(-7.000001267365,6.97408319067755,22.4171289075978));
#60900=CARTESIAN_POINT('Ctrl Pts',(-7.00000171384827,6.83211409570069,22.2174616157779));
#60901=CARTESIAN_POINT('Ctrl Pts',(-7.00000170643154,6.69789322077232,22.0149182197186));
#60902=CARTESIAN_POINT('Ctrl Pts',(-7.00000169893551,6.56223720785845,21.8102091566455));
#60903=CARTESIAN_POINT('Ctrl Pts',(-7.00000122941501,6.43449595912778,21.6025621300187));
#60904=CARTESIAN_POINT('Ctrl Pts',(-7.00000072342875,6.31464981325747,21.3926452566123));
#60905=CARTESIAN_POINT('Ctrl Pts',(-7.00000046988977,6.25459745267091,21.2874603657385));
#60906=CARTESIAN_POINT('Ctrl Pts',(-7.00000020716712,6.19652700585555,21.1817048306048));
#60907=CARTESIAN_POINT('Ctrl Pts',(-6.9999999876651,6.14043371090483,21.0754583709577));
#60908=CARTESIAN_POINT('Ctrl Pts',(-6.99999993928858,6.12807119021431,21.0520424875293));
#60909=CARTESIAN_POINT('Ctrl Pts',(-6.99999989300536,6.11580469922885,21.0286027476278));
#60910=CARTESIAN_POINT('Ctrl Pts',(-6.99999984878286,6.10363403754539,21.0051400153112));
#60911=CARTESIAN_POINT('Ctrl Pts',(-6.99999965374465,6.0499567448507,20.901660353915));
#60912=CARTESIAN_POINT('Ctrl Pts',(-6.99999949863664,5.99814353340517,20.7977336628826));
#60913=CARTESIAN_POINT('Ctrl Pts',(-6.99999938184581,5.94817674612069,20.6934324333637));
#60914=CARTESIAN_POINT('Ctrl Pts',(-6.99999932345039,5.92319335247844,20.6412818186042));
#60915=CARTESIAN_POINT('Ctrl Pts',(-6.99999927466558,5.89867156487647,20.589037569223));
#60916=CARTESIAN_POINT('Ctrl Pts',(-6.99999923547373,5.87460909341309,20.5367084539057));
#60917=CARTESIAN_POINT('Ctrl Pts',(-6.9999992158778,5.86257785768141,20.510543896247));
#60918=CARTESIAN_POINT('Ctrl Pts',(-6.99999919868214,5.85066145098437,20.4843581221043));
#60919=CARTESIAN_POINT('Ctrl Pts',(-6.9999991838965,5.83885958468295,20.4581522189196));
#60920=CARTESIAN_POINT('Ctrl Pts',(-6.99999917283138,5.83002742864498,20.4385405219106));
#60921=CARTESIAN_POINT('Ctrl Pts',(-6.99999916268834,5.82084768949662,20.417992321048));
#60922=CARTESIAN_POINT('Ctrl Pts',(-6.99999915445987,5.81224564769479,20.3985848619336));
#60923=CARTESIAN_POINT('Ctrl Pts',(-6.99999915169314,5.80935331068039,20.3920593283864));
#60924=CARTESIAN_POINT('Ctrl Pts',(-6.99999914913284,5.80652587403082,20.3856629460377));
#60925=CARTESIAN_POINT('Ctrl Pts',(-6.99999914678746,5.80379731694203,20.3794752047448));
#60926=CARTESIAN_POINT('Ctrl Pts',(-6.99999907529424,5.72062370058133,20.1908565305928));
#60927=CARTESIAN_POINT('Ctrl Pts',(-6.99999912491859,5.64168481543872,19.9974674673488));
#60928=CARTESIAN_POINT('Ctrl Pts',(-6.99999933315959,5.56752048182436,19.7994484879038));
#60929=CARTESIAN_POINT('Ctrl Pts',(-6.99999947285733,5.5177675985959,19.6666081496818));
#60930=CARTESIAN_POINT('Ctrl Pts',(-6.99999968443233,5.47016400472382,19.5316850389696));
#60931=CARTESIAN_POINT('Ctrl Pts',(-6.9999999881677,5.42487991144661,19.3947326004997));
#60932=CARTESIAN_POINT('Ctrl Pts',(-7.00000042903665,5.35915048847276,19.1959474619658));
#60933=CARTESIAN_POINT('Ctrl Pts',(-7.00000106780692,5.2983069601726,18.9928846798482));
#60934=CARTESIAN_POINT('Ctrl Pts',(-7.00000153331199,5.24286429356814,18.7857670926481));
#60935=CARTESIAN_POINT('Ctrl Pts',(-7.00000199134801,5.18831120660947,18.5819727148307));
#60936=CARTESIAN_POINT('Ctrl Pts',(-7.0000022813202,5.13898707176438,18.3742525496783));
#60937=CARTESIAN_POINT('Ctrl Pts',(-7.00000202662856,5.0954046904489,18.1628637274833));
#60938=CARTESIAN_POINT('Ctrl Pts',(-7.00000181209397,5.05869391263252,17.9848044326435));
#60939=CARTESIAN_POINT('Ctrl Pts',(-7.00000121063182,5.02605739395554,17.8041428574034));
#60940=CARTESIAN_POINT('Ctrl Pts',(-6.99999998662441,4.99781410946024,17.6210585612637));
#60941=CARTESIAN_POINT('Ctrl Pts',(-6.99999852881493,4.96417597344145,17.4030026741207));
#60942=CARTESIAN_POINT('Ctrl Pts',(-6.9999961728693,4.93677017808673,17.1815088206562));
#60943=CARTESIAN_POINT('Ctrl Pts',(-6.99999449845864,4.91605392436374,16.9569202229915));
#60944=CARTESIAN_POINT('Ctrl Pts',(-6.99999284827044,4.8956373574151,16.7355805830434));
#60945=CARTESIAN_POINT('Ctrl Pts',(-6.99999186158996,4.88171821086046,16.5112350383155));
#60946=CARTESIAN_POINT('Ctrl Pts',(-6.99999320068044,4.87474433973957,16.2842614502171));
#60947=CARTESIAN_POINT('Ctrl Pts',(-6.99999413396,4.86988389785898,16.1260721297867));
#60948=CARTESIAN_POINT('Ctrl Pts',(-6.99999620011843,4.86839726354882,15.9666072810556));
#60949=CARTESIAN_POINT('Ctrl Pts',(-6.99999999965507,4.87043896665418,15.8060095551962));
#60950=CARTESIAN_POINT('Ctrl Pts',(-7.0000050688351,4.87316292001774,15.5917469063387));
#60951=CARTESIAN_POINT('Ctrl Pts',(-7.00001329848799,4.88216722682931,15.3754653522329));
#60952=CARTESIAN_POINT('Ctrl Pts',(-7.00001657716596,4.89779630351165,15.1576281480176));
#60953=CARTESIAN_POINT('Ctrl Pts',(-7.00001838079985,4.90639401651905,15.0377937008366));
#60954=CARTESIAN_POINT('Ctrl Pts',(-7.00001867122039,4.91699660060305,14.9174893752695));
#60955=CARTESIAN_POINT('Ctrl Pts',(-7.0000159872059,4.92966193666588,14.796799023232));
#60956=CARTESIAN_POINT('Ctrl Pts',(-6.26386075990253,3.90573694599532,15.8144217439117));
#60957=CARTESIAN_POINT('Ctrl Pts',(-6.27437424078817,3.90868760274242,15.8076587396846));
#60958=CARTESIAN_POINT('Ctrl Pts',(-6.28486073450179,3.91182238565663,15.8008093299079));
#60959=CARTESIAN_POINT('Ctrl Pts',(-6.29531386314359,3.91514200828217,15.7938746164386));
#60960=CARTESIAN_POINT('Ctrl Pts',(-6.33637970203193,3.92818337537731,15.766631114916));
#60961=CARTESIAN_POINT('Ctrl Pts',(-6.37693083405109,3.94408145526261,15.7380701969033));
#60962=CARTESIAN_POINT('Ctrl Pts',(-6.41657832582218,3.96284753712821,15.7082659326139));
#60963=CARTESIAN_POINT('Ctrl Pts',(-6.45584412580718,3.98143295537587,15.6787485980233));
#60964=CARTESIAN_POINT('Ctrl Pts',(-6.49422354029561,4.00283147356113,15.6480118989296));
#60965=CARTESIAN_POINT('Ctrl Pts',(-6.53133639222252,4.02700421041334,15.6161374338063));
#60966=CARTESIAN_POINT('Ctrl Pts',(-6.53913743592629,4.03208526904487,15.6094374880314));
#60967=CARTESIAN_POINT('Ctrl Pts',(-6.54688251210572,4.03728872113799,15.6026873013788));
#60968=CARTESIAN_POINT('Ctrl Pts',(-6.55456808012088,4.04261391242737,15.5958876755575));
#60969=CARTESIAN_POINT('Ctrl Pts',(-6.59048110957155,4.06749740200537,15.5641144660964));
#60970=CARTESIAN_POINT('Ctrl Pts',(-6.62509401715786,4.09504226037126,15.5312624561904));
#60971=CARTESIAN_POINT('Ctrl Pts',(-6.65805353180285,4.12515734110993,15.4974380911881));
#60972=CARTESIAN_POINT('Ctrl Pts',(-6.66665268310277,4.1330143784016,15.4886133000645));
#60973=CARTESIAN_POINT('Ctrl Pts',(-6.67513927108329,4.14104609822003,15.4797223433999));
#60974=CARTESIAN_POINT('Ctrl Pts',(-6.6835069874228,4.14925028383301,15.4707671487047));
#60975=CARTESIAN_POINT('Ctrl Pts',(-6.70372707170477,4.16907520592987,15.4491274582383));
#60976=CARTESIAN_POINT('Ctrl Pts',(-6.72325280714651,4.18990753989218,15.427113219735));
#60977=CARTESIAN_POINT('Ctrl Pts',(-6.74199680599635,4.2117111890082,15.404754774594));
#60978=CARTESIAN_POINT('Ctrl Pts',(-6.75136880542126,4.22261301356621,15.3935755520236));
#60979=CARTESIAN_POINT('Ctrl Pts',(-6.76054545271633,4.23375761324951,15.3823102742471));
#60980=CARTESIAN_POINT('Ctrl Pts',(-6.76951613170011,4.24514000632777,15.3709629941128));
#60981=CARTESIAN_POINT('Ctrl Pts',(-6.774001471192,4.2508312028669,15.3652893540456));
#60982=CARTESIAN_POINT('Ctrl Pts',(-6.77843532773899,4.25658185105849,15.3595952131745));
#60983=CARTESIAN_POINT('Ctrl Pts',(-6.78281636744521,4.26239126853153,15.3538811340133));
#60984=CARTESIAN_POINT('Ctrl Pts',(-6.78500688729832,4.26529597726805,15.3510240944326));
#60985=CARTESIAN_POINT('Ctrl Pts',(-6.78718420291574,4.2682153777334,15.3481620702732));
#60986=CARTESIAN_POINT('Ctrl Pts',(-6.78934814805164,4.27114938188087,15.3452951314681));
#60987=CARTESIAN_POINT('Ctrl Pts',(-6.79114832908272,4.27359017325018,15.3429101316044));
#60988=CARTESIAN_POINT('Ctrl Pts',(-6.79330664708345,4.27654724408184,15.3400288633611));
#60989=CARTESIAN_POINT('Ctrl Pts',(-6.79490577325515,4.27875757383909,15.3378814778922));
#60990=CARTESIAN_POINT('Ctrl Pts',(-6.79522891003434,4.2792042170442,15.3374475538928));
#60991=CARTESIAN_POINT('Ctrl Pts',(-6.79552935127015,4.27962025354817,15.3370435698547));
#60992=CARTESIAN_POINT('Ctrl Pts',(-6.79579970571376,4.27999511491821,15.336679641855));
#60993=CARTESIAN_POINT('Ctrl Pts',(-6.8103038065088,4.30010585185524,15.3171554634471));
#60994=CARTESIAN_POINT('Ctrl Pts',(-6.82466112344216,4.32154660532228,15.2967066172978));
#60995=CARTESIAN_POINT('Ctrl Pts',(-6.83868683916184,4.34442059427056,15.2753634668361));
#60996=CARTESIAN_POINT('Ctrl Pts',(-6.8523579833504,4.36671632643349,15.2545598734058));
#60997=CARTESIAN_POINT('Ctrl Pts',(-6.86571378715539,4.39037451869574,15.2329067157737));
#60998=CARTESIAN_POINT('Ctrl Pts',(-6.87854492101801,4.41546138438675,15.2104366111897));
#60999=CARTESIAN_POINT('Ctrl Pts',(-6.89092336821551,4.43966317712243,15.1887592593599));
#61000=CARTESIAN_POINT('Ctrl Pts',(-6.9028129530209,4.46519521373549,15.1663217176226));
#61001=CARTESIAN_POINT('Ctrl Pts',(-6.91399605182675,4.49207938040125,15.1431558653217));
#61002=CARTESIAN_POINT('Ctrl Pts',(-6.92152697963795,4.51018372893101,15.1275555058515));
#61003=CARTESIAN_POINT('Ctrl Pts',(-6.928736887252,4.52890048186552,15.1116249176021));
#61004=CARTESIAN_POINT('Ctrl Pts',(-6.93555357905215,4.54822416775344,15.0953740358282));
#61005=CARTESIAN_POINT('Ctrl Pts',(-6.94510274554621,4.5752937638614,15.0726089790698));
#61006=CARTESIAN_POINT('Ctrl Pts',(-6.95387447251374,4.60353495328979,15.0491954413136));
#61007=CARTESIAN_POINT('Ctrl Pts',(-6.96168682153978,4.63298567227641,15.0252248664936));
#61008=CARTESIAN_POINT('Ctrl Pts',(-6.96890749341195,4.6602059075082,15.0030697304666));
#61009=CARTESIAN_POINT('Ctrl Pts',(-6.97530773605332,4.68845969100606,14.9804388867761));
#61010=CARTESIAN_POINT('Ctrl Pts',(-6.98071683853119,4.71773610714928,14.957402693869));
#61011=CARTESIAN_POINT('Ctrl Pts',(-6.98600813822278,4.74637492335643,14.9348681974487));
#61012=CARTESIAN_POINT('Ctrl Pts',(-6.99035024736982,4.77599276568247,14.911945979747));
#61013=CARTESIAN_POINT('Ctrl Pts',(-6.99356765821133,4.80653286408542,14.8886977956708));
#61014=CARTESIAN_POINT('Ctrl Pts',(-6.99669733437195,4.83624017304388,14.8660835598566));
#61015=CARTESIAN_POINT('Ctrl Pts',(-6.99876194175778,4.86682028043261,14.8431610402342));
#61016=CARTESIAN_POINT('Ctrl Pts',(-6.99959682204669,4.89817205285958,14.8199808716854));
#61017=CARTESIAN_POINT('Ctrl Pts',(-6.99987412951937,4.90858561860223,14.8122815235968));
#61018=CARTESIAN_POINT('Ctrl Pts',(-7.0000157989355,4.91908390180451,14.8045536889217));
#61019=CARTESIAN_POINT('Ctrl Pts',(-7.0000159872059,4.92966193655724,14.7967990233117));
#61020=CARTESIAN_POINT('Ctrl Pts',(-6.24907873965842,3.90163420221723,15.8312168444344));
#61021=CARTESIAN_POINT('Ctrl Pts',(-6.29175678648451,3.91267140088817,15.8162585233033));
#61022=CARTESIAN_POINT('Ctrl Pts',(-6.42266965978749,3.95530760846479,15.7676241602702));
#61023=CARTESIAN_POINT('Ctrl Pts',(-6.62983849714768,4.0702747377564,15.6756774243267));
#61024=CARTESIAN_POINT('Ctrl Pts',(-6.84319911297757,4.2747492473435,15.553294548616));
#61025=CARTESIAN_POINT('Ctrl Pts',(-7.00357104976123,4.53497041307359,15.4263581296174));
#61026=CARTESIAN_POINT('Ctrl Pts',(-7.09151802900392,4.81587189318471,15.3108183618548));
#61027=CARTESIAN_POINT('Ctrl Pts',(-7.10724350840679,5.00645768800968,15.2433526903401));
#61028=CARTESIAN_POINT('Ctrl Pts',(-7.10592746249851,5.09162974565076,15.2153112980894));
#61029=CARTESIAN_POINT('Ctrl Pts',(-6.05068860243976,3.86152988210803,15.2178949522498));
#61030=CARTESIAN_POINT('Ctrl Pts',(-6.08843043831061,3.87101767241173,15.2046346505576));
#61031=CARTESIAN_POINT('Ctrl Pts',(-6.20441284673364,3.90776438456602,15.1614401205735));
#61032=CARTESIAN_POINT('Ctrl Pts',(-6.38893740513147,4.00756197392119,15.0793702464572));
#61033=CARTESIAN_POINT('Ctrl Pts',(-6.58005579450863,4.18649249103738,14.9697285938614));
#61034=CARTESIAN_POINT('Ctrl Pts',(-6.72429241821602,4.41551556330386,14.8559648014311));
#61035=CARTESIAN_POINT('Ctrl Pts',(-6.80352362709971,4.66352886406962,14.7527862461739));
#61036=CARTESIAN_POINT('Ctrl Pts',(-6.81764215739556,4.83172244359836,14.6930400233625));
#61037=CARTESIAN_POINT('Ctrl Pts',(-6.81646301824315,4.90672397733544,14.6683643944402));
#61038=CARTESIAN_POINT('Ctrl Pts',(-6.03817570823002,3.3653742336236,14.8043699886451));
#61039=CARTESIAN_POINT('Ctrl Pts',(-6.09017057840755,3.37836166406013,14.7864796423558));
#61040=CARTESIAN_POINT('Ctrl Pts',(-6.24902820060427,3.42842032220146,14.7286780918748));
#61041=CARTESIAN_POINT('Ctrl Pts',(-6.49746651777635,3.56211616729947,14.6212903640043));
#61042=CARTESIAN_POINT('Ctrl Pts',(-6.75008955648423,3.79671603666322,14.4808560682429));
#61043=CARTESIAN_POINT('Ctrl Pts',(-6.938221838207,4.09228824662061,14.3368904112171));
#61044=CARTESIAN_POINT('Ctrl Pts',(-7.04099372055609,4.40971738199054,14.2065130934989));
#61045=CARTESIAN_POINT('Ctrl Pts',(-7.05951570838809,4.62558997385974,14.1301183926698));
#61046=CARTESIAN_POINT('Ctrl Pts',(-7.05795834765348,4.7225588847146,14.0981910611585));
#61047=CARTESIAN_POINT('Ctrl Pts',(-6.22023196797387,2.74899963093355,14.8711973556313));
#61048=CARTESIAN_POINT('Ctrl Pts',(-6.29602853838421,2.76816901593314,14.8454805002066));
#61049=CARTESIAN_POINT('Ctrl Pts',(-6.52656687096162,2.84173846370411,14.7629046578067));
#61050=CARTESIAN_POINT('Ctrl Pts',(-6.88224706785488,3.03547585470201,14.6121278007695));
#61051=CARTESIAN_POINT('Ctrl Pts',(-7.2385216941781,3.36931140292561,14.4181924261346));
#61052=CARTESIAN_POINT('Ctrl Pts',(-7.50089116590327,3.78417613333916,14.2210755321012));
#61053=CARTESIAN_POINT('Ctrl Pts',(-7.64353817399801,4.22638305526497,14.0423330763607));
#61054=CARTESIAN_POINT('Ctrl Pts',(-7.66949567306553,4.52776300479599,13.9361805986748));
#61055=CARTESIAN_POINT('Ctrl Pts',(-7.66730078022939,4.66398161311348,13.8912880999727));
#61056=CARTESIAN_POINT('',(-7.00000002017424,3.16613029753958,14.5427413090324));
#61057=CARTESIAN_POINT('Ctrl Pts',(-7.,4.92966193692261,14.7967990234135));
#61058=CARTESIAN_POINT('Ctrl Pts',(-7.,4.82595068015789,14.7556187999394));
#61059=CARTESIAN_POINT('Ctrl Pts',(-7.,4.73230467693603,14.7209082500355));
#61060=CARTESIAN_POINT('Ctrl Pts',(-7.,4.65045299426906,14.6929800881805));
#61061=CARTESIAN_POINT('Ctrl Pts',(-7.,4.60952715293557,14.679016007253));
#61062=CARTESIAN_POINT('Ctrl Pts',(-7.,4.57156438471307,14.6666986894123));
#61063=CARTESIAN_POINT('Ctrl Pts',(-7.,4.536804100054,14.6558533229263));
#61064=CARTESIAN_POINT('Ctrl Pts',(-7.,4.51942395772447,14.6504306396834));
#61065=CARTESIAN_POINT('Ctrl Pts',(-7.,4.5028443894743,14.6453743550468));
#61066=CARTESIAN_POINT('Ctrl Pts',(-7.,4.48709423463723,14.6406556616635));
#61067=CARTESIAN_POINT('Ctrl Pts',(-7.,4.47921915721869,14.6382963149719));
#61068=CARTESIAN_POINT('Ctrl Pts',(-7.,4.47155143315342,14.6360213660936));
#61069=CARTESIAN_POINT('Ctrl Pts',(-7.,4.46409448566477,14.6338269308933));
#61070=CARTESIAN_POINT('Ctrl Pts',(-7.,4.46036601192044,14.6327297132932));
#61071=CARTESIAN_POINT('Ctrl Pts',(-7.,4.45669023232026,14.6316526241125));
#61072=CARTESIAN_POINT('Ctrl Pts',(-7.,4.45306756465829,14.6305951801213));
#61073=CARTESIAN_POINT('Ctrl Pts',(-7.,4.44944489699631,14.6295377361301));
#61074=CARTESIAN_POINT('Ctrl Pts',(-7.,4.44753558080656,14.6289809309358));
#61075=CARTESIAN_POINT('Ctrl Pts',(-7.,4.44235931122075,14.6274812983564));
#61076=CARTESIAN_POINT('Ctrl Pts',(-7.,4.35953899784779,14.603487177086));
#61077=CARTESIAN_POINT('Ctrl Pts',(-7.,4.27926853216976,14.5830032990511));
#61078=CARTESIAN_POINT('Ctrl Pts',(-7.,4.20217774711042,14.5661085517943));
#61079=CARTESIAN_POINT('Ctrl Pts',(-7.,4.12508696205109,14.5492138045375));
#61080=CARTESIAN_POINT('Ctrl Pts',(-7.,4.0527845638725,14.5361291043884));
#61081=CARTESIAN_POINT('Ctrl Pts',(-7.,3.98126344323272,14.5256474164678));
#61082=CARTESIAN_POINT('Ctrl Pts',(-7.,3.83822120195318,14.5046840406266));
#61083=CARTESIAN_POINT('Ctrl Pts',(-7.,3.69572435361907,14.4945099507662));
#61084=CARTESIAN_POINT('Ctrl Pts',(-7.,3.55810486077357,14.4974003670815));
#61085=CARTESIAN_POINT('Ctrl Pts',(-7.,3.42048536792807,14.5002907833969));
#61086=CARTESIAN_POINT('Ctrl Pts',(-7.,3.28796856453053,14.5162141391388));
#61087=CARTESIAN_POINT('Ctrl Pts',(-7.,3.16613072517763,14.542741284242));
#61088=CARTESIAN_POINT('Ctrl Pts',(-6.2499459998768,2.76546773691422,14.8593866472137));
#61089=CARTESIAN_POINT('Ctrl Pts',(-6.29701743055659,2.77824199061018,14.8431647544954));
#61090=CARTESIAN_POINT('Ctrl Pts',(-6.34322178177099,2.792709947018,14.8266893964536));
#61091=CARTESIAN_POINT('Ctrl Pts',(-6.38860511461875,2.80882516992212,14.8099544424063));
#61092=CARTESIAN_POINT('Ctrl Pts',(-6.40556261896127,2.81484663078076,14.8037014187053));
#61093=CARTESIAN_POINT('Ctrl Pts',(-6.4224053522873,2.82109856990858,14.7974120498922));
#61094=CARTESIAN_POINT('Ctrl Pts',(-6.43913510817571,2.82758028715883,14.7910856860475));
#61095=CARTESIAN_POINT('Ctrl Pts',(-6.46648688592921,2.83817736286468,14.7807426004089));
#61096=CARTESIAN_POINT('Ctrl Pts',(-6.49353686265284,2.84938831338855,14.7703006731512));
#61097=CARTESIAN_POINT('Ctrl Pts',(-6.52029720529596,2.86121064762762,14.7597553008202));
#61098=CARTESIAN_POINT('Ctrl Pts',(-6.59365016089588,2.89361692770002,14.7308493096417));
#61099=CARTESIAN_POINT('Ctrl Pts',(-6.66481622967055,2.93059441007357,14.7011737610307));
#61100=CARTESIAN_POINT('Ctrl Pts',(-6.73336338682278,2.97189481715064,14.6708725711793));
#61101=CARTESIAN_POINT('Ctrl Pts',(-6.7460546543055,2.9795414437233,14.6652624113795));
#61102=CARTESIAN_POINT('Ctrl Pts',(-6.75865601417981,2.987336308447,14.6596308188776));
#61103=CARTESIAN_POINT('Ctrl Pts',(-6.77116453647933,2.99527789980353,14.6539787286651));
#61104=CARTESIAN_POINT('Ctrl Pts',(-6.80197425854347,3.01483882127632,14.6400570739439));
#61105=CARTESIAN_POINT('Ctrl Pts',(-6.83222110171795,3.03529283448632,14.6260105120857));
#61106=CARTESIAN_POINT('Ctrl Pts',(-6.86190703099567,3.05665271147598,14.6118299629835));
#61107=CARTESIAN_POINT('Ctrl Pts',(-6.90200296541259,3.08550288554055,14.5926767014676));
#61108=CARTESIAN_POINT('Ctrl Pts',(-6.9410772764051,3.11600461962484,14.5732789530564));
#61109=CARTESIAN_POINT('Ctrl Pts',(-6.97913132965225,3.14820836614017,14.5536087616453));
#61110=CARTESIAN_POINT('Ctrl Pts',(-6.98612216659513,3.15412445448368,14.5499951886076));
#61111=CARTESIAN_POINT('Ctrl Pts',(-6.99307845882553,3.16009806955511,14.5463724203771));
#61112=CARTESIAN_POINT('Ctrl Pts',(-7.00000005853886,3.16612963662624,14.5427402846217));
#61113=CARTESIAN_POINT('Ctrl Pts',(7.10691982128491,-7.16634812687415,14.3573277946041));
#61114=CARTESIAN_POINT('Ctrl Pts',(7.10723242798241,-7.19552103167944,14.3426529330767));
#61115=CARTESIAN_POINT('Ctrl Pts',(7.1039242705972,-7.3187564684501,14.2819048781017));
#61116=CARTESIAN_POINT('Ctrl Pts',(7.06369615611098,-7.53922760006879,14.1823067263407));
#61117=CARTESIAN_POINT('Ctrl Pts',(6.94787920664715,-7.8127689334572,14.0761819460459));
#61118=CARTESIAN_POINT('Ctrl Pts',(6.77787455319756,-8.05682754693778,13.9995481841559));
#61119=CARTESIAN_POINT('Ctrl Pts',(6.56638861545542,-8.25893233176591,13.9558001011829));
#61120=CARTESIAN_POINT('Ctrl Pts',(6.38249370354767,-8.37571921190027,13.9481326205135));
#61121=CARTESIAN_POINT('Ctrl Pts',(6.27483013576736,-8.42598304509719,13.9530906703659));
#61122=CARTESIAN_POINT('Ctrl Pts',(6.25029140148474,-8.43656339435967,13.9546787322473));
#61123=CARTESIAN_POINT('Ctrl Pts',(6.81469559418484,-6.90842566153106,13.8380339234899));
#61124=CARTESIAN_POINT('Ctrl Pts',(6.81497660549222,-6.93407149048773,13.8251286161839));
#61125=CARTESIAN_POINT('Ctrl Pts',(6.81201885386562,-7.04253689015183,13.7717073504501));
#61126=CARTESIAN_POINT('Ctrl Pts',(6.77586367536613,-7.23730205240579,13.6842786040574));
#61127=CARTESIAN_POINT('Ctrl Pts',(6.6717314805588,-7.47924373358209,13.5919128736868));
#61128=CARTESIAN_POINT('Ctrl Pts',(6.5192820021909,-7.69478794234902,13.5262200739852));
#61129=CARTESIAN_POINT('Ctrl Pts',(6.33046962900436,-7.87269576845227,13.4898403370137));
#61130=CARTESIAN_POINT('Ctrl Pts',(6.16723164439068,-7.97503474134159,13.4846001443658));
#61131=CARTESIAN_POINT('Ctrl Pts',(6.07210359157714,-8.01895822338946,13.4895950828663));
#61132=CARTESIAN_POINT('Ctrl Pts',(6.05044504509845,-8.02819857653725,13.4911219087981));
#61133=CARTESIAN_POINT('Ctrl Pts',(7.05841184590234,-6.63607078428829,13.3013650836311));
#61134=CARTESIAN_POINT('Ctrl Pts',(7.0587777866451,-6.66928177922984,13.2846602023184));
#61135=CARTESIAN_POINT('Ctrl Pts',(7.05485772682236,-6.80931320231469,13.2156289903415));
#61136=CARTESIAN_POINT('Ctrl Pts',(7.00774539855559,-7.05851473581658,13.1029646382612));
#61137=CARTESIAN_POINT('Ctrl Pts',(6.87223084342461,-7.36801504029715,12.9826820888225));
#61138=CARTESIAN_POINT('Ctrl Pts',(6.67211859264277,-7.64608395178626,12.8952410504026));
#61139=CARTESIAN_POINT('Ctrl Pts',(6.42070776244213,-7.8789865058943,12.8449652134551));
#61140=CARTESIAN_POINT('Ctrl Pts',(6.19931043638224,-8.01568553558642,12.8364055904847));
#61141=CARTESIAN_POINT('Ctrl Pts',(6.06838347156874,-8.07522561979308,12.8426925700324));
#61142=CARTESIAN_POINT('Ctrl Pts',(6.03847420372112,-8.08779776067679,12.8446797960011));
#61143=CARTESIAN_POINT('Ctrl Pts',(7.67172816874031,-6.5351689148283,13.1136040700797));
#61144=CARTESIAN_POINT('Ctrl Pts',(7.67223759814686,-6.58187397818695,13.0901237528483));
#61145=CARTESIAN_POINT('Ctrl Pts',(7.66669930574663,-6.77826320004743,12.9931998819998));
#61146=CARTESIAN_POINT('Ctrl Pts',(7.60107815888014,-7.12488980375239,12.835118593979));
#61147=CARTESIAN_POINT('Ctrl Pts',(7.4125330539824,-7.55499723180348,12.6642970064452));
#61148=CARTESIAN_POINT('Ctrl Pts',(7.13207063067744,-7.94395590627747,12.5372620297768));
#61149=CARTESIAN_POINT('Ctrl Pts',(6.77551369413477,-8.27351015060811,12.4613099458292));
#61150=CARTESIAN_POINT('Ctrl Pts',(6.45683536720761,-8.46992594992077,12.4459497372264));
#61151=CARTESIAN_POINT('Ctrl Pts',(6.26620834906591,-8.55638102622129,12.4539020742517));
#61152=CARTESIAN_POINT('Ctrl Pts',(6.22254868972825,-8.57468274401025,12.4565571066556));
#61153=CARTESIAN_POINT('',(6.26385989014072,-8.4207183952526,13.9442649556632));
#61154=CARTESIAN_POINT('',(6.24999925108292,-8.5516700679197,12.4626498445719));
#61155=CARTESIAN_POINT('Origin',(6.527902330383,-9.095144289412,13.2547395928924));
#61156=CARTESIAN_POINT('',(6.99999925693877,-8.04450726878133,12.5220453001149));
#61157=CARTESIAN_POINT('Ctrl Pts',(6.99999932345931,-8.04450779086442,12.5220461127869));
#61158=CARTESIAN_POINT('Ctrl Pts',(6.93523191518207,-8.10843582533326,12.5061772190589));
#61159=CARTESIAN_POINT('Ctrl Pts',(6.86743938004946,-8.1682348981219,12.493290097609));
#61160=CARTESIAN_POINT('Ctrl Pts',(6.79657680503947,-8.22416384023962,12.483332862315));
#61161=CARTESIAN_POINT('Ctrl Pts',(6.78822731619943,-8.23075375145836,12.4821596361805));
#61162=CARTESIAN_POINT('Ctrl Pts',(6.77983520416841,-8.23728990558737,12.4810270335501));
#61163=CARTESIAN_POINT('Ctrl Pts',(6.77140039427982,-8.24377270394801,12.4799349282528));
#61164=CARTESIAN_POINT('Ctrl Pts',(6.69137888490863,-8.30527537165709,12.469574064708));
#61165=CARTESIAN_POINT('Ctrl Pts',(6.60751263574372,-8.36197566386238,12.4628589954802));
#61166=CARTESIAN_POINT('Ctrl Pts',(6.52054032183533,-8.41339421877647,12.459915588264));
#61167=CARTESIAN_POINT('Ctrl Pts',(6.44077171921804,-8.4605538962621,12.4572159765137));
#61168=CARTESIAN_POINT('Ctrl Pts',(6.35839158720097,-8.50327266058605,12.4576922431241));
#61169=CARTESIAN_POINT('Ctrl Pts',(6.27311920727313,-8.5414595618975,12.4615310781794));
#61170=CARTESIAN_POINT('Ctrl Pts',(6.26544704768595,-8.54489532856954,12.4618764673336));
#61171=CARTESIAN_POINT('Ctrl Pts',(6.25775147218604,-8.54829438959152,12.4622490480023));
#61172=CARTESIAN_POINT('Ctrl Pts',(6.25003227450165,-8.55165666657415,12.4626489390251));
#61173=CARTESIAN_POINT('',(6.99999053791474,-6.97711506405584,13.9486981655111));
#61174=CARTESIAN_POINT('Ctrl Pts',(6.999992895158,-6.97711506288399,13.9486981661339));
#61175=CARTESIAN_POINT('Ctrl Pts',(7.,-7.01455702470623,13.862138053422));
#61176=CARTESIAN_POINT('Ctrl Pts',(7.,-7.0801064098619,13.7187009838892));
#61177=CARTESIAN_POINT('Ctrl Pts',(7.,-7.1457012109594,13.5893393878538));
#61178=CARTESIAN_POINT('Ctrl Pts',(7.,-7.18319507671516,13.5188655305678));
#61179=CARTESIAN_POINT('Ctrl Pts',(7.,-7.19198611824022,13.5025948308775));
#61180=CARTESIAN_POINT('Ctrl Pts',(7.,-7.28161416552635,13.3396546434541));
#61181=CARTESIAN_POINT('Ctrl Pts',(7.,-7.36734370955451,13.2056023658641));
#61182=CARTESIAN_POINT('Ctrl Pts',(7.,-7.63342635361862,12.8482671475625));
#61183=CARTESIAN_POINT('Ctrl Pts',(7.,-7.82958249364545,12.660118225788));
#61184=CARTESIAN_POINT('Ctrl Pts',(6.999998447357,-8.04450634432302,12.5220438611068));
#61185=CARTESIAN_POINT('Ctrl Pts',(6.99997871935865,-6.97711506623554,13.9486981642574));
#61186=CARTESIAN_POINT('Ctrl Pts',(6.99998461169886,-7.00647256572936,13.944192975335));
#61187=CARTESIAN_POINT('Ctrl Pts',(6.99926918215788,-7.03549390394242,13.9398952854494));
#61188=CARTESIAN_POINT('Ctrl Pts',(6.9978867243848,-7.06412133653092,13.9358116282601));
#61189=CARTESIAN_POINT('Ctrl Pts',(6.99565943477728,-7.11024323937347,13.9292324130424));
#61190=CARTESIAN_POINT('Ctrl Pts',(6.99170320771225,-7.15534155737423,13.9232085050283));
#61191=CARTESIAN_POINT('Ctrl Pts',(6.98629128447007,-7.19927391203044,13.9177213839171));
#61192=CARTESIAN_POINT('Ctrl Pts',(6.98059873556339,-7.24548430088387,13.9119497378896));
#61193=CARTESIAN_POINT('Ctrl Pts',(6.9732952011298,-7.29040458299394,13.9067721201308));
#61194=CARTESIAN_POINT('Ctrl Pts',(6.96465598626061,-7.33390797762943,13.9021650165857));
#61195=CARTESIAN_POINT('Ctrl Pts',(6.96131166253051,-7.35074856293986,13.9003815621924));
#61196=CARTESIAN_POINT('Ctrl Pts',(6.95776677933511,-7.3673772269038,13.8986835707991));
#61197=CARTESIAN_POINT('Ctrl Pts',(6.95403590762787,-7.38378810741358,13.8970695411509));
#61198=CARTESIAN_POINT('Ctrl Pts',(6.94867965578311,-7.40734850184747,13.8947523482911));
#61199=CARTESIAN_POINT('Ctrl Pts',(6.94294025497593,-7.4304599269881,13.8926081951853));
#61200=CARTESIAN_POINT('Ctrl Pts',(6.93686495180243,-7.45311123350962,13.8906295633292));
#61201=CARTESIAN_POINT('Ctrl Pts',(6.92508574188899,-7.49702912315409,13.8867932576653));
#61202=CARTESIAN_POINT('Ctrl Pts',(6.91204633189904,-7.53921528441703,13.8835791656713));
#61203=CARTESIAN_POINT('Ctrl Pts',(6.89805485559285,-7.57961678769472,13.8809316931373));
#61204=CARTESIAN_POINT('Ctrl Pts',(6.8849547097132,-7.61744450330617,13.8784528784899));
#61205=CARTESIAN_POINT('Ctrl Pts',(6.87101910746412,-7.65370821014627,13.8764708448023));
#61206=CARTESIAN_POINT('Ctrl Pts',(6.85646977033409,-7.68839143484718,13.8749381971813));
#61207=CARTESIAN_POINT('Ctrl Pts',(6.84887976069648,-7.70648476840533,13.874138654899));
#61208=CARTESIAN_POINT('Ctrl Pts',(6.84112232443655,-7.72414843240078,13.8734613457473));
#61209=CARTESIAN_POINT('Ctrl Pts',(6.83322939388326,-7.74138491679247,13.8728974458017));
#61210=CARTESIAN_POINT('Ctrl Pts',(6.82669899579392,-7.7556459195947,13.8724308901792));
#61211=CARTESIAN_POINT('Ctrl Pts',(6.82007579813622,-7.76961452281618,13.8720419720816));
#61212=CARTESIAN_POINT('Ctrl Pts',(6.81337672309828,-7.78329277122056,13.8717257571408));
#61213=CARTESIAN_POINT('Ctrl Pts',(6.81002718557931,-7.79013189542275,13.8715676496704));
#61214=CARTESIAN_POINT('Ctrl Pts',(6.80665867083591,-7.79689842709432,13.871427722253));
#61215=CARTESIAN_POINT('Ctrl Pts',(6.80327319043602,-7.80359269140715,13.8713053571058));
#61216=CARTESIAN_POINT('Ctrl Pts',(6.80113746306185,-7.80781576224322,13.8712281631589));
#61217=CARTESIAN_POINT('Ctrl Pts',(6.79934549967287,-7.81132577461448,13.8711696878805));
#61218=CARTESIAN_POINT('Ctrl Pts',(6.79723646122255,-7.81541914235799,13.8711065106));
#61219=CARTESIAN_POINT('Ctrl Pts',(6.79600232562242,-7.8178144381175,13.8710695414633));
#61220=CARTESIAN_POINT('Ctrl Pts',(6.79465906404181,-7.82040915241095,13.8710312483486));
#61221=CARTESIAN_POINT('Ctrl Pts',(6.79306783305638,-7.82345899582193,13.8709903453484));
#61222=CARTESIAN_POINT('Ctrl Pts',(6.76770433410507,-7.87207211413368,13.8703383701076));
#61223=CARTESIAN_POINT('Ctrl Pts',(6.74051264580759,-7.91869839077715,13.8706400530389));
#61224=CARTESIAN_POINT('Ctrl Pts',(6.71177143962633,-7.9631738516196,13.8719116731427));
#61225=CARTESIAN_POINT('Ctrl Pts',(6.67920446635632,-8.01356947994824,13.8733525597104));
#61226=CARTESIAN_POINT('Ctrl Pts',(6.64464924538837,-8.06120381413504,13.8760382416814));
#61227=CARTESIAN_POINT('Ctrl Pts',(6.60855631925091,-8.10592857893428,13.8799422685215));
#61228=CARTESIAN_POINT('Ctrl Pts',(6.58247964648337,-8.13824164360055,13.8827628774685));
#61229=CARTESIAN_POINT('Ctrl Pts',(6.55559909698159,-8.16903621853364,13.8862198555525));
#61230=CARTESIAN_POINT('Ctrl Pts',(6.52806938950912,-8.19826223787322,13.8903070009252));
#61231=CARTESIAN_POINT('Ctrl Pts',(6.48890293382725,-8.23984203280442,13.896121773867));
#61232=CARTESIAN_POINT('Ctrl Pts',(6.44842494734317,-8.27824683059856,13.9032112200784));
#61233=CARTESIAN_POINT('Ctrl Pts',(6.40711341512205,-8.31342797164745,13.9115007136302));
#61234=CARTESIAN_POINT('Ctrl Pts',(6.37671580707502,-8.33931475140976,13.9176002398968));
#61235=CARTESIAN_POINT('Ctrl Pts',(6.34586575073266,-8.36345636015453,13.9243498879396));
#61236=CARTESIAN_POINT('Ctrl Pts',(6.31473704059775,-8.38583898722829,13.9317234455883));
#61237=CARTESIAN_POINT('Ctrl Pts',(6.29786789628842,-8.39796848968737,13.9357192940353));
#61238=CARTESIAN_POINT('Ctrl Pts',(6.28091670191048,-8.40958155320845,13.9398983834985));
#61239=CARTESIAN_POINT('Ctrl Pts',(6.26391275766735,-8.42068213410475,13.9442527024039));
#61240=CARTESIAN_POINT('Ctrl Pts',(6.99933866940308,-10.874321861748,24.2330493766441));
#61241=CARTESIAN_POINT('Ctrl Pts',(6.99933866940308,-10.8803485967835,24.1955798273128));
#61242=CARTESIAN_POINT('Ctrl Pts',(6.99933866940308,-10.9752955965243,23.5851351122749));
#61243=CARTESIAN_POINT('Ctrl Pts',(6.99933866940308,-11.0599204354475,22.3847684638779));
#61244=CARTESIAN_POINT('Ctrl Pts',(6.99933866940308,-10.904731832472,20.6450473295634));
#61245=CARTESIAN_POINT('Ctrl Pts',(6.99933866940308,-10.4757466585894,18.9490871086045));
#61246=CARTESIAN_POINT('Ctrl Pts',(6.99933866940308,-9.78232713548459,17.3424622371035));
#61247=CARTESIAN_POINT('Ctrl Pts',(6.99933866940308,-8.84436745984052,15.8669670641752));
#61248=CARTESIAN_POINT('Ctrl Pts',(6.99933866940308,-7.8388982304481,14.7344891895317));
#61249=CARTESIAN_POINT('Ctrl Pts',(6.99933866940308,-7.1385959671508,14.1224323391862));
#61250=CARTESIAN_POINT('Ctrl Pts',(6.99933866940308,-6.8652637212831,13.9057057530616));
#61251=CARTESIAN_POINT('Ctrl Pts',(7.01707119673726,-11.3554689991295,24.3104931498652));
#61252=CARTESIAN_POINT('Ctrl Pts',(7.01707119673726,-11.3617630889567,24.2713590868946));
#61253=CARTESIAN_POINT('Ctrl Pts',(7.01707119673726,-11.4609222058883,23.6338095273083));
#61254=CARTESIAN_POINT('Ctrl Pts',(7.01707119673726,-11.5493039149732,22.3805007967095));
#61255=CARTESIAN_POINT('Ctrl Pts',(7.01707119673726,-11.3871776978523,20.5627917354021));
#61256=CARTESIAN_POINT('Ctrl Pts',(7.01707119673726,-10.9391538957696,18.7917526334238));
#61257=CARTESIAN_POINT('Ctrl Pts',(7.01707119673726,-10.2148922939487,17.1135088397462));
#61258=CARTESIAN_POINT('Ctrl Pts',(7.01707119673726,-9.23504398166122,15.5722064363879));
#61259=CARTESIAN_POINT('Ctrl Pts',(7.01707119673726,-8.18492837750478,14.3894430108701));
#61260=CARTESIAN_POINT('Ctrl Pts',(7.01707119673726,-7.45357513988494,13.7502283468605));
#61261=CARTESIAN_POINT('Ctrl Pts',(7.01707119673726,-7.16803669166219,13.5238268590662));
#61262=CARTESIAN_POINT('Ctrl Pts',(6.72645657496606,-11.7431402439294,24.3728913678652));
#61263=CARTESIAN_POINT('Ctrl Pts',(6.72645657496606,-11.7496497476197,24.3324161682093));
#61264=CARTESIAN_POINT('Ctrl Pts',(6.72645657496606,-11.8522026636346,23.6730276159059));
#61265=CARTESIAN_POINT('Ctrl Pts',(6.72645657496606,-11.9436113688706,22.377062239736));
#61266=CARTESIAN_POINT('Ctrl Pts',(6.72645657496606,-11.7758953574806,20.4965165233067));
#61267=CARTESIAN_POINT('Ctrl Pts',(6.72645657496606,-11.3125316975443,18.664984651021));
#61268=CARTESIAN_POINT('Ctrl Pts',(6.72645657496606,-10.5634199280358,16.9290358549664));
#61269=CARTESIAN_POINT('Ctrl Pts',(6.72645657496606,-9.54982098387161,15.3347110620732));
#61270=CARTESIAN_POINT('Ctrl Pts',(6.72645657496606,-8.46373277521302,14.1114314189815));
#61271=CARTESIAN_POINT('Ctrl Pts',(6.72645657496606,-7.70736105793842,13.4503350838351));
#61272=CARTESIAN_POINT('Ctrl Pts',(6.72645657496606,-7.41198779351563,13.2161383066535));
#61273=CARTESIAN_POINT('Ctrl Pts',(6.2530336072437,-11.8653885094301,24.3925680243669));
#61274=CARTESIAN_POINT('Ctrl Pts',(6.2530336072437,-11.871965941738,24.3516699106168));
#61275=CARTESIAN_POINT('Ctrl Pts',(6.2530336072437,-11.9755890584896,23.6853946494987));
#61276=CARTESIAN_POINT('Ctrl Pts',(6.2530336072437,-12.0679522968085,22.3759779250414));
#61277=CARTESIAN_POINT('Ctrl Pts',(6.2530336072437,-11.8984735994768,20.4756172953318));
#61278=CARTESIAN_POINT('Ctrl Pts',(6.2530336072437,-11.4302726681641,18.6250096304905));
#61279=CARTESIAN_POINT('Ctrl Pts',(6.2530336072437,-10.6733246458032,16.8708641367243));
#61280=CARTESIAN_POINT('Ctrl Pts',(6.2530336072437,-9.64908277606497,15.2598192614479));
#61281=CARTESIAN_POINT('Ctrl Pts',(6.2530336072437,-8.55165096489382,14.023763232717));
#61282=CARTESIAN_POINT('Ctrl Pts',(6.2530336072437,-7.78738991926524,13.3557667305361));
#61283=CARTESIAN_POINT('Ctrl Pts',(6.2530336072437,-7.48891534351923,13.1191117864997));
#61284=CARTESIAN_POINT('',(6.99999999999999,-10.9277801898196,24.1259420764689));
#61285=CARTESIAN_POINT('Ctrl Pts',(6.99999999999999,-10.9277802009504,24.1259420781412));
#61286=CARTESIAN_POINT('Ctrl Pts',(6.99999999999999,-10.9521697295792,23.9636071725245));
#61287=CARTESIAN_POINT('Ctrl Pts',(7.00000000006069,-10.9728907817461,23.8012468908599));
#61288=CARTESIAN_POINT('Ctrl Pts',(6.9999999986734,-10.9899916559804,23.6387646053103));
#61289=CARTESIAN_POINT('Ctrl Pts',(6.99999999728326,-11.007127638005,23.4759487465215));
#61290=CARTESIAN_POINT('Ctrl Pts',(6.99999999422988,-11.0206285810772,23.3130099248014));
#61291=CARTESIAN_POINT('Ctrl Pts',(6.99999999314799,-11.0304911277933,23.1498445645567));
#61292=CARTESIAN_POINT('Ctrl Pts',(6.99999999206991,-11.0403189654241,22.9872534292619));
#61293=CARTESIAN_POINT('Ctrl Pts',(6.99999999472212,-11.0465339705917,22.8244368952001));
#61294=CARTESIAN_POINT('Ctrl Pts',(6.99999999803537,-11.0490812192129,22.6612929825452));
#61295=CARTESIAN_POINT('Ctrl Pts',(6.9999999990723,-11.0498784125077,22.6102350558974));
#61296=CARTESIAN_POINT('Ctrl Pts',(6.99999999999999,-11.050315984112,22.5591450947523));
#61297=CARTESIAN_POINT('Ctrl Pts',(6.99999999999999,-11.0503912041555,22.5080200916307));
#61298=CARTESIAN_POINT('Ctrl Pts',(6.99999999999999,-11.0504514191662,22.4670935982913));
#61299=CARTESIAN_POINT('Ctrl Pts',(6.99999999938395,-11.050284473563,22.4261442171503));
#61300=CARTESIAN_POINT('Ctrl Pts',(6.99999999847198,-11.0498891036841,22.3851771719374));
#61301=CARTESIAN_POINT('Ctrl Pts',(6.99999999416106,-11.0480201762815,22.1915245001614));
#61302=CARTESIAN_POINT('Ctrl Pts',(6.99999998574661,-11.0410429983283,21.9974766397485));
#61303=CARTESIAN_POINT('Ctrl Pts',(6.99999998500516,-11.0289287826382,21.8035275616802));
#61304=CARTESIAN_POINT('Ctrl Pts',(6.99999998426214,-11.0167889585745,21.6091684925233));
#61305=CARTESIAN_POINT('Ctrl Pts',(6.9999999898422,-10.9994903474747,21.4149090420219));
#61306=CARTESIAN_POINT('Ctrl Pts',(6.99999999472998,-10.9770562251435,21.2212489722765));
#61307=CARTESIAN_POINT('Ctrl Pts',(6.99999999759807,-10.9638921791236,21.107611806859));
#61308=CARTESIAN_POINT('Ctrl Pts',(6.99999999999999,-10.9489608647286,20.9941810381186));
#61309=CARTESIAN_POINT('Ctrl Pts',(6.99999999999999,-10.932275327311,20.8810571714478));
#61310=CARTESIAN_POINT('Ctrl Pts',(6.99999999999999,-10.9207674511519,20.8030365829761));
#61311=CARTESIAN_POINT('Ctrl Pts',(6.99999999890217,-10.9084190204695,20.7251635518545));
#61312=CARTESIAN_POINT('Ctrl Pts',(6.99999999758209,-10.8952326698626,20.6474486195686));
#61313=CARTESIAN_POINT('Ctrl Pts',(6.99999999346273,-10.8540842340522,20.4049366465432));
#61314=CARTESIAN_POINT('Ctrl Pts',(6.99999998925867,-10.8047802507612,20.1639637182118));
#61315=CARTESIAN_POINT('Ctrl Pts',(6.99999999152157,-10.7474287547034,19.9248987552727));
#61316=CARTESIAN_POINT('Ctrl Pts',(6.99999999354312,-10.6961940769102,19.7113312428321));
#61317=CARTESIAN_POINT('Ctrl Pts',(6.99999999999999,-10.638536191055,19.4992861507973));
#61318=CARTESIAN_POINT('Ctrl Pts',(6.99999999999999,-10.5744977406333,19.2890339660142));
#61319=CARTESIAN_POINT('Ctrl Pts',(6.99999999999999,-10.5402382199967,19.176552495647));
#61320=CARTESIAN_POINT('Ctrl Pts',(6.99999999803026,-10.5041671068588,19.064577502989));
#61321=CARTESIAN_POINT('Ctrl Pts',(6.9999999963631,-10.4662992290647,18.953187918004));
#61322=CARTESIAN_POINT('Ctrl Pts',(6.99999999271524,-10.383442022048,18.7094607687616));
#61323=CARTESIAN_POINT('Ctrl Pts',(6.9999999920498,-10.2919792980796,18.4685373660799));
#61324=CARTESIAN_POINT('Ctrl Pts',(6.99999999506633,-10.192229900311,18.2311614364419));
#61325=CARTESIAN_POINT('Ctrl Pts',(6.99999999705715,-10.126398300433,18.0745004683543));
#61326=CARTESIAN_POINT('Ctrl Pts',(6.99999999999999,-10.0569584112504,17.9193843975432));
#61327=CARTESIAN_POINT('Ctrl Pts',(6.99999999999999,-9.98401350683041,17.7660225963322));
#61328=CARTESIAN_POINT('Ctrl Pts',(6.99999999999999,-9.91676134047503,17.6246293975939));
#61329=CARTESIAN_POINT('Ctrl Pts',(6.99999999722473,-9.84651938466177,17.4847350710404));
#61330=CARTESIAN_POINT('Ctrl Pts',(6.99999999446462,-9.77332652212723,17.3464252545198));
#61331=CARTESIAN_POINT('Ctrl Pts',(6.99999999008266,-9.65712508822082,17.126843748257));
#61332=CARTESIAN_POINT('Ctrl Pts',(6.9999999878424,-9.53348786437254,16.9112542269386));
#61333=CARTESIAN_POINT('Ctrl Pts',(6.9999999926269,-9.40257758585834,16.7000150351235));
#61334=CARTESIAN_POINT('Ctrl Pts',(6.99999999531398,-9.32905545431275,16.5813783946359));
#61335=CARTESIAN_POINT('Ctrl Pts',(6.99999999999999,-9.25323851341331,16.464114496737));
#61336=CARTESIAN_POINT('Ctrl Pts',(6.99999999999999,-9.17515027025553,16.3482917014736));
#61337=CARTESIAN_POINT('Ctrl Pts',(6.99999999999999,-9.06614443700028,16.1866110207835));
#61338=CARTESIAN_POINT('Ctrl Pts',(6.99999999014829,-8.95275813323968,16.0276937647234));
#61339=CARTESIAN_POINT('Ctrl Pts',(6.99999998525269,-8.83523425972555,15.8719395760796));
#61340=CARTESIAN_POINT('Ctrl Pts',(6.9999999800339,-8.70995173852396,15.7059028649202));
#61341=CARTESIAN_POINT('Ctrl Pts',(6.99999998144993,-8.57996719499021,15.5434613062878));
#61342=CARTESIAN_POINT('Ctrl Pts',(6.99999998835927,-8.44567949375304,15.3850002973565));
#61343=CARTESIAN_POINT('Ctrl Pts',(6.99999999308627,-8.35380681241871,15.2765894924701));
#61344=CARTESIAN_POINT('Ctrl Pts',(6.99999999999999,-8.25992084841546,15.1700411226945));
#61345=CARTESIAN_POINT('Ctrl Pts',(6.99999999999999,-8.16415901451128,15.0654684229204));
#61346=CARTESIAN_POINT('Ctrl Pts',(6.99999999999999,-8.0515313796965,14.9424781316783));
#61347=CARTESIAN_POINT('Ctrl Pts',(6.99999999283346,-7.93626854432952,14.8222826805839));
#61348=CARTESIAN_POINT('Ctrl Pts',(6.99999999157248,-7.81832399166569,14.704766066323));
#61349=CARTESIAN_POINT('Ctrl Pts',(6.99999999107886,-7.77215394478804,14.6587635382978));
#61350=CARTESIAN_POINT('Ctrl Pts',(6.99999999110859,-7.72557250945403,14.6131718504097));
#61351=CARTESIAN_POINT('Ctrl Pts',(6.99999999149962,-7.67857521415048,14.5679854218538));
#61352=CARTESIAN_POINT('Ctrl Pts',(6.99999999249427,-7.55902957501349,14.4530460312539));
#61353=CARTESIAN_POINT('Ctrl Pts',(6.99999999550996,-7.43679567896384,14.3407261100692));
#61354=CARTESIAN_POINT('Ctrl Pts',(6.9999999971702,-7.31180057699937,14.2309835488546));
#61355=CARTESIAN_POINT('Ctrl Pts',(6.99999999862359,-7.2023786773616,14.1349138682792));
#61356=CARTESIAN_POINT('Ctrl Pts',(6.99999999923208,-7.09084007712802,14.0408196924531));
#61357=CARTESIAN_POINT('Ctrl Pts',(6.99999999922763,-6.97711506346271,13.9486981662434));
#61358=CARTESIAN_POINT('',(6.27159471697349,-11.879498130607,24.2690139179281));
#61359=CARTESIAN_POINT('Origin',(5.999999877384,-10.9277801432444,24.1259420367214));
#61360=CARTESIAN_POINT('Ctrl Pts',(6.27159470457059,-11.8794980693497,24.2690136413476));
#61361=CARTESIAN_POINT('Ctrl Pts',(6.27193966902461,-11.9138782752637,24.0395180963159));
#61362=CARTESIAN_POINT('Ctrl Pts',(6.27225782570503,-11.9412741979417,23.8113318898144));
#61363=CARTESIAN_POINT('Ctrl Pts',(6.2725491703234,-11.9620370299863,23.5849163366204));
#61364=CARTESIAN_POINT('Ctrl Pts',(6.27284515823024,-11.9831307684991,23.3548922982783));
#61365=CARTESIAN_POINT('Ctrl Pts',(6.27311347263771,-11.9973783339202,23.1266957546801));
#61366=CARTESIAN_POINT('Ctrl Pts',(6.27335410998336,-12.0051465975195,22.9007562103819));
#61367=CARTESIAN_POINT('Ctrl Pts',(6.27354178919894,-12.0112052648252,22.7245401857032));
#61368=CARTESIAN_POINT('Ctrl Pts',(6.27371263292358,-12.0133226538049,22.5496959438336));
#61369=CARTESIAN_POINT('Ctrl Pts',(6.27386663982658,-12.0116720606791,22.3764053057318));
#61370=CARTESIAN_POINT('Ctrl Pts',(6.27406868985895,-12.0095065577829,22.1490558924583));
#61371=CARTESIAN_POINT('Ctrl Pts',(6.27424175991821,-12.0008567741586,21.924382128493));
#61372=CARTESIAN_POINT('Ctrl Pts',(6.27438584775141,-11.9862080268575,21.702730216841));
#61373=CARTESIAN_POINT('Ctrl Pts',(6.27447251988024,-11.9773964701482,21.5694015199156));
#61374=CARTESIAN_POINT('Ctrl Pts',(6.27454870539273,-11.9664139927013,21.4371652340053));
#61375=CARTESIAN_POINT('Ctrl Pts',(6.27461440393747,-11.9533633920536,21.3060881202131));
#61376=CARTESIAN_POINT('Ctrl Pts',(6.27472591298159,-11.9312128252649,21.0836131214071));
#61377=CARTESIAN_POINT('Ctrl Pts',(6.27480721144035,-11.9031053991405,20.8644800898332));
#61378=CARTESIAN_POINT('Ctrl Pts',(6.27485829825228,-11.8695299765572,20.6489750513824));
#61379=CARTESIAN_POINT('Ctrl Pts',(6.27487121253493,-11.861042414286,20.5944973324769));
#61380=CARTESIAN_POINT('Ctrl Pts',(6.27488219619905,-11.852205343758,20.5402512077538));
#61381=CARTESIAN_POINT('Ctrl Pts',(6.27489124923553,-11.8430264894263,20.4862408043289));
#61382=CARTESIAN_POINT('Ctrl Pts',(6.2749281265656,-11.8056366433318,20.266230703004));
#61383=CARTESIAN_POINT('Ctrl Pts',(6.27493296851791,-11.7625774362594,20.0501357110777));
#61384=CARTESIAN_POINT('Ctrl Pts',(6.27490577502609,-11.7143927225912,19.8381799883121));
#61385=CARTESIAN_POINT('Ctrl Pts',(6.27488257562516,-11.6732852216319,19.6573556269408));
#61386=CARTESIAN_POINT('Ctrl Pts',(6.27483606022284,-11.6284468537051,19.4795430164125));
#61387=CARTESIAN_POINT('Ctrl Pts',(6.27476622928505,-11.580201581638,19.3048547409607));
#61388=CARTESIAN_POINT('Ctrl Pts',(6.27472435130897,-11.5512686414021,19.2000932748732));
#61389=CARTESIAN_POINT('Ctrl Pts',(6.27467408806462,-11.5211101803306,19.0964550027122));
#61390=CARTESIAN_POINT('Ctrl Pts',(6.27461544106535,-11.4897939376987,18.9939601886112));
#61391=CARTESIAN_POINT('Ctrl Pts',(6.27458611756572,-11.4741358163827,18.9427127815608));
#61392=CARTESIAN_POINT('Ctrl Pts',(6.27455469549538,-11.4581882408752,18.8917512417613));
#61393=CARTESIAN_POINT('Ctrl Pts',(6.27452117829932,-11.4419595134016,18.8410777748231));
#61394=CARTESIAN_POINT('Ctrl Pts',(6.27450441970129,-11.4338451496648,18.815741041354));
#61395=CARTESIAN_POINT('Ctrl Pts',(6.27448713714406,-11.42566049734,18.7904763262773));
#61396=CARTESIAN_POINT('Ctrl Pts',(6.27446933062821,-11.417406587565,18.7652838965214));
#61397=CARTESIAN_POINT('Ctrl Pts',(6.27445391884753,-11.410262716844,18.7434795073012));
#61398=CARTESIAN_POINT('Ctrl Pts',(6.27443872924805,-11.4033391852076,18.7225464152243));
#61399=CARTESIAN_POINT('Ctrl Pts',(6.27442216557726,-11.3959300847421,18.7003629482844));
#61400=CARTESIAN_POINT('Ctrl Pts',(6.27441959185747,-11.3947788333836,18.6969160053567));
#61401=CARTESIAN_POINT('Ctrl Pts',(6.27441698496212,-11.3936157619352,18.6934389053631));
#61402=CARTESIAN_POINT('Ctrl Pts',(6.27441433890278,-11.3924381130524,18.6899237251114));
#61403=CARTESIAN_POINT('Ctrl Pts',(6.27440279536136,-11.3873005719312,18.674588608375));
#61404=CARTESIAN_POINT('Ctrl Pts',(6.27439106194386,-11.3821286345952,18.659254378921));
#61405=CARTESIAN_POINT('Ctrl Pts',(6.27437913865126,-11.3769222139522,18.6439212020826));
#61406=CARTESIAN_POINT('Ctrl Pts',(6.27420010485628,-11.298745381651,18.4136864061409));
#61407=CARTESIAN_POINT('Ctrl Pts',(6.27397826087162,-11.2127926337038,18.1836848208436));
#61408=CARTESIAN_POINT('Ctrl Pts',(6.27371361097497,-11.1188661132799,17.954486037609));
#61409=CARTESIAN_POINT('Ctrl Pts',(6.27345238303172,-11.0261540734958,17.7282508208268));
#61410=CARTESIAN_POINT('Ctrl Pts',(6.27314944898001,-10.9256730981749,17.5027977428166));
#61411=CARTESIAN_POINT('Ctrl Pts',(6.27280481477215,-10.8172468333938,17.2787232728831));
#61412=CARTESIAN_POINT('Ctrl Pts',(6.27260797344829,-10.7553180723634,17.1507408663181));
#61413=CARTESIAN_POINT('Ctrl Pts',(6.27239752857088,-10.6907976264797,17.0232090921316));
#61414=CARTESIAN_POINT('Ctrl Pts',(6.27217348154728,-10.6236547832016,16.8962464403836));
#61415=CARTESIAN_POINT('Ctrl Pts',(6.27177013422557,-10.5027788814663,16.6676781482547));
#61416=CARTESIAN_POINT('Ctrl Pts',(6.27132270209057,-10.3734022583509,16.4409510714598));
#61417=CARTESIAN_POINT('Ctrl Pts',(6.27083119534451,-10.2354141323912,16.2167885889214));
#61418=CARTESIAN_POINT('Ctrl Pts',(6.27036732298328,-10.1051842254242,16.005229376537));
#61419=CARTESIAN_POINT('Ctrl Pts',(6.26986419337307,-9.9672840646058,15.7959548398425));
#61420=CARTESIAN_POINT('Ctrl Pts',(6.26932181699206,-9.82164027902969,15.5896211743922));
#61421=CARTESIAN_POINT('Ctrl Pts',(6.26905884654146,-9.7510250876935,15.4895805773476));
#61422=CARTESIAN_POINT('Ctrl Pts',(6.26878665006723,-9.67858983338576,15.3902320272094));
#61423=CARTESIAN_POINT('Ctrl Pts',(6.26850522898499,-9.60432785523052,15.2916544052724));
#61424=CARTESIAN_POINT('Ctrl Pts',(6.26791730417586,-9.44918503869204,15.0857130838198));
#61425=CARTESIAN_POINT('Ctrl Pts',(6.26728911874199,-9.28606733530127,14.8831340243101));
#61426=CARTESIAN_POINT('Ctrl Pts',(6.2666206878755,-9.11502762540494,14.6845502371122));
#61427=CARTESIAN_POINT('Ctrl Pts',(6.26595956710941,-8.94585844171389,14.4881382039364));
#61428=CARTESIAN_POINT('Ctrl Pts',(6.26525907633653,-8.76893953451425,14.2956345095279));
#61429=CARTESIAN_POINT('Ctrl Pts',(6.26451923361523,-8.58435346620896,14.1076918850216));
#61430=CARTESIAN_POINT('Ctrl Pts',(6.26430323028774,-8.5304620054781,14.0528204493752));
#61431=CARTESIAN_POINT('Ctrl Pts',(6.26408387263419,-8.47591720627682,13.9983380635825));
#61432=CARTESIAN_POINT('Ctrl Pts',(6.26386116116393,-8.42072164431578,13.9442616342516));
#61433=CARTESIAN_POINT('Ctrl Pts',(6.99999999998952,-9.33248386897495,24.7867299440625));
#61434=CARTESIAN_POINT('Ctrl Pts',(6.99999999998952,-9.33249195735398,24.786726802229));
#61435=CARTESIAN_POINT('Ctrl Pts',(6.99999999998952,-9.6023398658611,24.6819075264287));
#61436=CARTESIAN_POINT('Ctrl Pts',(6.99999999998952,-10.1365881548782,24.4674868371929));
#61437=CARTESIAN_POINT('Ctrl Pts',(6.99999999998952,-10.6659288230028,24.2412740854125));
#61438=CARTESIAN_POINT('Ctrl Pts',(6.99999999998952,-10.9277807259463,24.1259369152881));
#61439=CARTESIAN_POINT('Ctrl Pts',(7.00000270572501,-9.54650236979056,25.3377021349181));
#61440=CARTESIAN_POINT('Ctrl Pts',(7.00000270572501,-9.54651058116988,25.3376989453067));
#61441=CARTESIAN_POINT('Ctrl Pts',(7.00000270572501,-9.82046207618911,25.2312856794191));
#61442=CARTESIAN_POINT('Ctrl Pts',(7.00000270572501,-10.3628264314778,25.0136075514825));
#61443=CARTESIAN_POINT('Ctrl Pts',(7.00000270572501,-10.9002087461763,24.7839582708241));
#61444=CARTESIAN_POINT('Ctrl Pts',(7.00000270572501,-11.1660426386622,24.6668671647262));
#61445=CARTESIAN_POINT('Ctrl Pts',(6.57967198017911,-9.69699923069142,25.725143336737));
#61446=CARTESIAN_POINT('Ctrl Pts',(6.57967198017911,-9.69700752856398,25.7251401135283));
#61447=CARTESIAN_POINT('Ctrl Pts',(6.57967198017911,-9.97384464742507,25.617605960879));
#61448=CARTESIAN_POINT('Ctrl Pts',(6.57967198017911,-10.5219161845321,25.3976372164886));
#61449=CARTESIAN_POINT('Ctrl Pts',(6.57967198017911,-11.0649533494474,25.1655713839582));
#61450=CARTESIAN_POINT('Ctrl Pts',(6.57967198017911,-11.3335873593288,25.0472469178692));
#61451=CARTESIAN_POINT('Ctrl Pts',(5.98852436209622,-9.69454278461808,25.7188194279643));
#61452=CARTESIAN_POINT('Ctrl Pts',(5.98852436209622,-9.69455108107887,25.718816205304));
#61453=CARTESIAN_POINT('Ctrl Pts',(5.98852436209622,-9.97134110008892,25.6113003480331));
#61454=CARTESIAN_POINT('Ctrl Pts',(5.98852436209622,-10.519319483198,25.3913689916389));
#61455=CARTESIAN_POINT('Ctrl Pts',(5.98852436209622,-11.0622643482839,25.1593426026514));
#61456=CARTESIAN_POINT('Ctrl Pts',(5.98852436209622,-11.3308526539734,25.0410382677614));
#61457=CARTESIAN_POINT('',(6.99999999994033,-9.33250873275173,24.7867180660544));
#61458=CARTESIAN_POINT('',(5.98852583803188,-9.69456766153457,25.7188097331067));
#61459=CARTESIAN_POINT('Origin',(5.999999999061,-9.33250979146063,24.7867247845918));
#61460=CARTESIAN_POINT('',(5.98852581752181,-11.3308503373093,25.0410389569969));
#61461=CARTESIAN_POINT('Origin',(5.98846855648545,4.75314843273632,-11.4751154999728));
#61462=CARTESIAN_POINT('Origin',(6.,-10.9277801936245,24.1259421517584));
#61463=CARTESIAN_POINT('Origin',(6.99999997873566,4.74946019458188,-11.4664777699154));
#61464=CARTESIAN_POINT('Origin',(5.999999877384,-10.9277801432444,24.1259420367214));
#61465=CARTESIAN_POINT('Origin',(5.99999763271771,-10.927779210435,24.1259401188868));
#61466=CARTESIAN_POINT('Ctrl Pts',(-6.09474589299296,-11.2721661211721,
25.0678864406018));
#61467=CARTESIAN_POINT('Ctrl Pts',(-6.05665088594491,-11.2844331672992,
25.0619829591023));
#61468=CARTESIAN_POINT('Ctrl Pts',(-5.71262397471385,-11.3942435667727,
25.0092456877338));
#61469=CARTESIAN_POINT('Ctrl Pts',(-5.02648233484312,-11.5958351263256,
24.9142565089414));
#61470=CARTESIAN_POINT('Ctrl Pts',(-3.98603640523322,-11.8499663881965,
24.7972465440184));
#61471=CARTESIAN_POINT('Ctrl Pts',(-2.81241127776029,-12.0696726758818,
24.6980993235061));
#61472=CARTESIAN_POINT('Ctrl Pts',(-1.52058000263906,-12.2260603896697,
24.6290271692427));
#61473=CARTESIAN_POINT('Ctrl Pts',(-0.18943338566882,-12.2892377815174,
24.6021117442546));
#61474=CARTESIAN_POINT('Ctrl Pts',(1.08611700923628,-12.2543717429925,24.6168486008321));
#61475=CARTESIAN_POINT('Ctrl Pts',(2.24134999476999,-12.1455614154255,24.6644539540119));
#61476=CARTESIAN_POINT('Ctrl Pts',(3.27313427271148,-11.9878599489094,24.7348915555515));
#61477=CARTESIAN_POINT('Ctrl Pts',(4.20017951060728,-11.7988850751499,24.8206976463489));
#61478=CARTESIAN_POINT('Ctrl Pts',(5.05727095054733,-11.5852913554165,24.9192987376905));
#61479=CARTESIAN_POINT('Ctrl Pts',(5.68075726226311,-11.403640393652,25.004824199225));
#61480=CARTESIAN_POINT('Ctrl Pts',(6.02267051912257,-11.2953816471556,25.0567121658076));
#61481=CARTESIAN_POINT('Ctrl Pts',(6.09461115805388,-11.2722173874739,25.0678609837662));
#61482=CARTESIAN_POINT('Ctrl Pts',(-6.21870783125079,-11.6030071289173,
24.9346094928434));
#61483=CARTESIAN_POINT('Ctrl Pts',(-6.17988419054913,-11.6154566213683,
24.9284813863121));
#61484=CARTESIAN_POINT('Ctrl Pts',(-5.82927340985939,-11.7268865197749,
24.8737036247638));
#61485=CARTESIAN_POINT('Ctrl Pts',(-5.12991816585638,-11.9312122509951,
24.7744497244118));
#61486=CARTESIAN_POINT('Ctrl Pts',(-4.06889120378561,-12.1883443489005,
24.6509624758045));
#61487=CARTESIAN_POINT('Ctrl Pts',(-2.8713420059513,-12.4102486289105,24.5452756161874));
#61488=CARTESIAN_POINT('Ctrl Pts',(-1.55249930391971,-12.5678336068868,
24.4708055953072));
#61489=CARTESIAN_POINT('Ctrl Pts',(-0.193370339803287,-12.631221050945,
24.4412527778677));
#61490=CARTESIAN_POINT('Ctrl Pts',(1.10886668231814,-12.5962715383566,24.4574968110138));
#61491=CARTESIAN_POINT('Ctrl Pts',(2.28838800899833,-12.4867526600937,24.5090736087206));
#61492=CARTESIAN_POINT('Ctrl Pts',(3.34149766488906,-12.3276452266319,24.5845653347974));
#61493=CARTESIAN_POINT('Ctrl Pts',(4.28728535808482,-12.1366714881359,24.6757451511196));
#61494=CARTESIAN_POINT('Ctrl Pts',(5.16128278679853,-11.9205124015365,24.7796819536751));
#61495=CARTESIAN_POINT('Ctrl Pts',(5.79679487909143,-11.7364122164643,24.8690883834396));
#61496=CARTESIAN_POINT('Ctrl Pts',(6.14525360451488,-11.6265672049225,24.9230077699474));
#61497=CARTESIAN_POINT('Ctrl Pts',(6.21857044990854,-11.6030581495952,24.934580419999));
#61498=CARTESIAN_POINT('Ctrl Pts',(-6.32920995303496,-11.8134825706664,
24.6410481436331));
#61499=CARTESIAN_POINT('Ctrl Pts',(-6.28968289989913,-11.8260512681113,
24.6347407922777));
#61500=CARTESIAN_POINT('Ctrl Pts',(-5.93272838617964,-11.9385158037939,
24.5783421587689));
#61501=CARTESIAN_POINT('Ctrl Pts',(-5.22085586767563,-12.1441818047848,
24.4758249486542));
#61502=CARTESIAN_POINT('Ctrl Pts',(-4.14083998302221,-12.4019390210003,
24.3475960658914));
#61503=CARTESIAN_POINT('Ctrl Pts',(-2.92182894542457,-12.6234699451084,
24.2372880454582));
#61504=CARTESIAN_POINT('Ctrl Pts',(-1.57943400594235,-12.7800180096094,
24.1591267156643));
#61505=CARTESIAN_POINT('Ctrl Pts',(-0.19663864163009,-12.8424707279084,
24.1278317350971));
#61506=CARTESIAN_POINT('Ctrl Pts',(1.12797187797457,-12.8080965926766,24.1450661652523));
#61507=CARTESIAN_POINT('Ctrl Pts',(2.32846266169234,-12.6995389486587,24.1993284835348));
#61508=CARTESIAN_POINT('Ctrl Pts',(3.4004058329485,-12.5410674609128,24.2783326775672));
#61509=CARTESIAN_POINT('Ctrl Pts',(4.36314548455404,-12.3501685854821,24.3733486865178));
#61510=CARTESIAN_POINT('Ctrl Pts',(5.25278011477892,-12.1333806487397,24.4812087583929));
#61511=CARTESIAN_POINT('Ctrl Pts',(5.89967149746468,-11.948107139288,24.573578404262));
#61512=CARTESIAN_POINT('Ctrl Pts',(6.25442391879544,-11.8372665858876,24.6291055563114));
#61513=CARTESIAN_POINT('Ctrl Pts',(6.32906931217782,-11.8135319788164,24.6410164748022));
#61514=CARTESIAN_POINT('Ctrl Pts',(-6.39488492041273,-11.8436591114854,
24.2701454690196));
#61515=CARTESIAN_POINT('Ctrl Pts',(-6.35487922842965,-11.8562498384674,
24.2637551803992));
#61516=CARTESIAN_POINT('Ctrl Pts',(-5.99362080848964,-11.9688695480746,
24.2066158363988));
#61517=CARTESIAN_POINT('Ctrl Pts',(-5.27347888337443,-12.1740990310879,
24.1027642521193));
#61518=CARTESIAN_POINT('Ctrl Pts',(-4.18145499098206,-12.4299236517987,
23.972877644657));
#61519=CARTESIAN_POINT('Ctrl Pts',(-2.94953624141899,-12.6486106768879,
23.8611813945531));
#61520=CARTESIAN_POINT('Ctrl Pts',(-1.5937350037576,-12.8021773211153,23.7820856217206));
#61521=CARTESIAN_POINT('Ctrl Pts',(-0.198310009722217,-12.8628133789537,
23.7504395921336));
#61522=CARTESIAN_POINT('Ctrl Pts',(1.13800675393286,-12.8295115867388,23.7678657201884));
#61523=CARTESIAN_POINT('Ctrl Pts',(2.35019416885011,-12.7233156388094,23.8227634215804));
#61524=CARTESIAN_POINT('Ctrl Pts',(3.43313248483788,-12.5673456810811,23.9027391680116));
#61525=CARTESIAN_POINT('Ctrl Pts',(4.40622212620569,-12.3785782658713,23.9989627708025));
#61526=CARTESIAN_POINT('Ctrl Pts',(5.30578762347871,-12.1632801814373,24.1082181549124));
#61527=CARTESIAN_POINT('Ctrl Pts',(5.9601831227946,-11.9784445497445,24.2017910192575));
#61528=CARTESIAN_POINT('Ctrl Pts',(6.31919194555327,-11.8674827026873,24.2580454484966));
#61529=CARTESIAN_POINT('Ctrl Pts',(6.39474133018431,-11.8437059948412,24.270112962504));
#61530=CARTESIAN_POINT('',(-5.98852245733355,-11.3308498383553,25.041039515272));
#61531=CARTESIAN_POINT('Ctrl Pts',(-5.98852261948756,-11.3308502493362,
25.0410393033413));
#61532=CARTESIAN_POINT('Ctrl Pts',(-5.87203729212264,-11.3676893585621,
25.0233524151582));
#61533=CARTESIAN_POINT('Ctrl Pts',(-5.74885694585024,-11.4056370269848,
25.0052380517102));
#61534=CARTESIAN_POINT('Ctrl Pts',(-5.61897930285015,-11.4443295356622,
24.9868774560996));
#61535=CARTESIAN_POINT('Ctrl Pts',(-5.51139836494418,-11.4763795196109,
24.9716689101892));
#61536=CARTESIAN_POINT('Ctrl Pts',(-5.39922222271884,-11.5089397853205,
24.95629165793));
#61537=CARTESIAN_POINT('Ctrl Pts',(-5.28245262905368,-11.5417771151824,
24.9408537610589));
#61538=CARTESIAN_POINT('Ctrl Pts',(-5.21028892635494,-11.5620706114189,
24.9313131283897));
#61539=CARTESIAN_POINT('Ctrl Pts',(-5.13637046322292,-11.5824668107469,
24.9217505880393));
#61540=CARTESIAN_POINT('Ctrl Pts',(-5.06069736322921,-11.6028989291272,
24.9121955101112));
#61541=CARTESIAN_POINT('Ctrl Pts',(-5.00123303445601,-11.618954597588,24.9046870785098));
#61542=CARTESIAN_POINT('Ctrl Pts',(-4.94068526356721,-11.6350323657382,
24.8971832504966));
#61543=CARTESIAN_POINT('Ctrl Pts',(-4.87905391860342,-11.6510985731773,
24.8896996784921));
#61544=CARTESIAN_POINT('Ctrl Pts',(-4.80902284567548,-11.6693544419322,
24.8811961714355));
#61545=CARTESIAN_POINT('Ctrl Pts',(-4.73759279368948,-11.6875951379917,
24.8727189371375));
#61546=CARTESIAN_POINT('Ctrl Pts',(-4.66476376183948,-11.7057675159946,
24.8642922961047));
#61547=CARTESIAN_POINT('Ctrl Pts',(-4.62834924591448,-11.7148537049961,
24.8600789755884));
#61548=CARTESIAN_POINT('Ctrl Pts',(-4.59158498506663,-11.7239228122847,
24.8558782984125));
#61549=CARTESIAN_POINT('Ctrl Pts',(-4.55447097936004,-11.7329678424902,
24.8516934278991));
#61550=CARTESIAN_POINT('Ctrl Pts',(-4.53591397650673,-11.737490357593,24.8496009926424));
#61551=CARTESIAN_POINT('Ctrl Pts',(-4.51726953744016,-11.74200685328,24.8475125087285));
#61552=CARTESIAN_POINT('Ctrl Pts',(-4.49853766217382,-11.7465164463142,
24.8454283731866));
#61553=CARTESIAN_POINT('Ctrl Pts',(-4.48917172454064,-11.7487712428313,
24.8443863054157));
#61554=CARTESIAN_POINT('Ctrl Pts',(-4.47978392785757,-11.7510243136755,
24.8433453247165));
#61555=CARTESIAN_POINT('Ctrl Pts',(-4.47037427212638,-11.7532755472464,
24.842305481108));
#61556=CARTESIAN_POINT('Ctrl Pts',(-4.46096461639519,-11.7555267808173,
24.8412656374995));
#61557=CARTESIAN_POINT('Ctrl Pts',(-4.45028767571464,-11.7580722650254,
24.8400902439203));
#61558=CARTESIAN_POINT('Ctrl Pts',(-4.44207972779027,-11.7600236241699,
24.839189411637));
#61559=CARTESIAN_POINT('Ctrl Pts',(-4.3082138427399,-11.7918489258584,24.8244974676823));
#61560=CARTESIAN_POINT('Ctrl Pts',(-4.17003358662756,-11.8233757417418,
24.8100018159802));
#61561=CARTESIAN_POINT('Ctrl Pts',(-4.02753109711927,-11.8542860450678,
24.7958403638104));
#61562=CARTESIAN_POINT('Ctrl Pts',(-3.89043362431304,-11.8840239428708,
24.782216045313));
#61563=CARTESIAN_POINT('Ctrl Pts',(-3.74933536252293,-11.9131909388871,
24.768901016943));
#61564=CARTESIAN_POINT('Ctrl Pts',(-3.60424405611465,-11.9414881581407,
24.7560277004985));
#61565=CARTESIAN_POINT('Ctrl Pts',(-3.45629266440207,-11.9703431810486,
24.7429006212057));
#61566=CARTESIAN_POINT('Ctrl Pts',(-3.30418521703504,-11.9982928718332,
24.7302333253027));
#61567=CARTESIAN_POINT('Ctrl Pts',(-3.14792171413729,-12.0250014601485,
24.7181717967167));
#61568=CARTESIAN_POINT('Ctrl Pts',(-3.06978996268842,-12.0383557543061,
24.7121410324237));
#61569=CARTESIAN_POINT('Ctrl Pts',(-2.99061919724623,-12.0513995223159,
24.706261772375));
#61570=CARTESIAN_POINT('Ctrl Pts',(-2.91040941695071,-12.0640894680238,
24.7005525165982));
#61571=CARTESIAN_POINT('Ctrl Pts',(-2.8944008951393,-12.0666221675512,24.6994130452607));
#61572=CARTESIAN_POINT('Ctrl Pts',(-2.87835098870976,-12.0691407759745,
24.698280343509));
#61573=CARTESIAN_POINT('Ctrl Pts',(-2.86225969246319,-12.0716449382825,
24.6971545622365));
#61574=CARTESIAN_POINT('Ctrl Pts',(-2.83803873028227,-12.0754142567779,
24.6954600122631));
#61575=CARTESIAN_POINT('Ctrl Pts',(-2.81372399115987,-12.0791508453967,
24.6937811417577));
#61576=CARTESIAN_POINT('Ctrl Pts',(-2.7893154852027,-12.0828535279687,24.6921184602829));
#61577=CARTESIAN_POINT('Ctrl Pts',(-2.76900328635972,-12.0859348154834,
24.6907348148935));
#61578=CARTESIAN_POINT('Ctrl Pts',(-2.74862614907856,-12.0889926192221,
24.6893623822283));
#61579=CARTESIAN_POINT('Ctrl Pts',(-2.72818407336812,-12.0920262541816,
24.6880014584464));
#61580=CARTESIAN_POINT('Ctrl Pts',(-2.7179630355129,-12.0935430716613,24.6873209965555));
#61581=CARTESIAN_POINT('Ctrl Pts',(-2.70772576305032,-12.0950538469408,
24.686643411874));
#61582=CARTESIAN_POINT('Ctrl Pts',(-2.69747225598158,-12.0965584941556,
24.6859687414516));
#61583=CARTESIAN_POINT('Ctrl Pts',(-2.68721874891285,-12.0980631413704,
24.6852940710292));
#61584=CARTESIAN_POINT('Ctrl Pts',(-2.6755394896848,-12.0997661554961,24.6845306665604));
#61585=CARTESIAN_POINT('Ctrl Pts',(-2.66666303095805,-12.1010539656649,
24.6839535099897));
#61586=CARTESIAN_POINT('Ctrl Pts',(-2.48101466815436,-12.1279881132578,
24.6718824605159));
#61587=CARTESIAN_POINT('Ctrl Pts',(-2.29046761447812,-12.152891870862,24.6607744723008));
#61588=CARTESIAN_POINT('Ctrl Pts',(-2.09501603487607,-12.1752942100462,
24.6508269772436));
#61589=CARTESIAN_POINT('Ctrl Pts',(-1.9914217661717,-12.187168015056,24.6455545538742));
#61590=CARTESIAN_POINT('Ctrl Pts',(-1.88645003482912,-12.198338371781,24.6406083864231));
#61591=CARTESIAN_POINT('Ctrl Pts',(-1.78010252029589,-12.2087299989047,
24.6360195566438));
#61592=CARTESIAN_POINT('Ctrl Pts',(-1.69952665156399,-12.2166033788018,
24.6325427575146));
#61593=CARTESIAN_POINT('Ctrl Pts',(-1.61816109532668,-12.224030864184,24.6292705220193));
#61594=CARTESIAN_POINT('Ctrl Pts',(-1.53600439826816,-12.2309813192398,
24.6262153348566));
#61595=CARTESIAN_POINT('Ctrl Pts',(-1.46165279623633,-12.2372714634003,
24.6234503982393));
#61596=CARTESIAN_POINT('Ctrl Pts',(-1.38665322243647,-12.2431708891406,
24.6208632424687));
#61597=CARTESIAN_POINT('Ctrl Pts',(-1.31100694342468,-12.2486562098158,
24.6184622894281));
#61598=CARTESIAN_POINT('Ctrl Pts',(-1.23139016223158,-12.2544294425732,
24.61593531579));
#61599=CARTESIAN_POINT('Ctrl Pts',(-1.15105628669057,-12.2597439305082,
24.6136146255172));
#61600=CARTESIAN_POINT('Ctrl Pts',(-1.07000531525417,-12.2645727179209,
24.6115095904989));
#61601=CARTESIAN_POINT('Ctrl Pts',(-1.02947982953596,-12.2669871116273,
24.6104570729898));
#61602=CARTESIAN_POINT('Ctrl Pts',(-0.988775069842594,-12.2692800782001,
24.6094584653373));
#61603=CARTESIAN_POINT('Ctrl Pts',(-0.947891036077653,-12.2714482656201,
24.6085148998782));
#61604=CARTESIAN_POINT('Ctrl Pts',(-0.927449019195181,-12.2725323593301,
24.6080431171487));
#61605=CARTESIAN_POINT('Ctrl Pts',(-0.906962183795259,-12.273585258121,
24.6075850947084));
#61606=CARTESIAN_POINT('Ctrl Pts',(-0.886430529875502,-12.2746065445393,
24.6071409713632));
#61607=CARTESIAN_POINT('Ctrl Pts',(-0.876164702915622,-12.2751171877484,
24.6069189096906));
#61608=CARTESIAN_POINT('Ctrl Pts',(-0.865887671325822,-12.2756199278561,
24.6067003227752));
#61609=CARTESIAN_POINT('Ctrl Pts',(-0.855599435106474,-12.2761147128055,
24.6064852277811));
#61610=CARTESIAN_POINT('Ctrl Pts',(-0.845311198887126,-12.2766094977549,
24.6062701327869));
#61611=CARTESIAN_POINT('Ctrl Pts',(-0.833325131026369,-12.277174653871,
24.6060244894571));
#61612=CARTESIAN_POINT('Ctrl Pts',(-0.824701112560467,-12.2775751501454,
24.6058504356311));
#61613=CARTESIAN_POINT('Ctrl Pts',(-0.603040005567242,-12.2878690111678,
24.6013767713046));
#61614=CARTESIAN_POINT('Ctrl Pts',(-0.379291206361343,-12.2940987664784,
24.5986974694608));
#61615=CARTESIAN_POINT('Ctrl Pts',(-0.153450032143192,-12.2960189027172,
24.5978640448336));
#61616=CARTESIAN_POINT('Ctrl Pts',(-0.0981184220889285,-12.296489340537,
24.5976598538723));
#61617=CARTESIAN_POINT('Ctrl Pts',(-0.0426612493675976,-12.2967008729678,
24.5975665207692));
#61618=CARTESIAN_POINT('Ctrl Pts',(0.0129209291749937,-12.2966522430943,
24.5975851009201));
#61619=CARTESIAN_POINT('Ctrl Pts',(0.154143964989606,-12.2965286844546,
24.5976323093129));
#61620=CARTESIAN_POINT('Ctrl Pts',(0.296176681680763,-12.2947211521966,
24.5984041962327));
#61621=CARTESIAN_POINT('Ctrl Pts',(0.439019093386752,-12.2911972488102,
24.5999241571628));
#61622=CARTESIAN_POINT('Ctrl Pts',(0.510440299239747,-12.289435297117,24.6006841376278));
#61623=CARTESIAN_POINT('Ctrl Pts',(0.582063928371205,-12.2872442541996,
24.6016311402581));
#61624=CARTESIAN_POINT('Ctrl Pts',(0.653889980745084,-12.284621348819,24.6027674927322));
#61625=CARTESIAN_POINT('Ctrl Pts',(0.689803006932021,-12.2833098961286,
24.6033356689693));
#61626=CARTESIAN_POINT('Ctrl Pts',(0.72576663891555,-12.2818904780535,24.6039511831153));
#61627=CARTESIAN_POINT('Ctrl Pts',(0.761780876621343,-12.2803627883741,
24.6046143100682));
#61628=CARTESIAN_POINT('Ctrl Pts',(0.77978799547424,-12.2795989435345,24.6049458735447));
#61629=CARTESIAN_POINT('Ctrl Pts',(0.797807765757056,-12.2788080308129,
24.6052893402592));
#61630=CARTESIAN_POINT('Ctrl Pts',(0.815840187458312,-12.2779900166903,
24.6056447425024));
#61631=CARTESIAN_POINT('Ctrl Pts',(0.833872609159567,-12.2771720025676,
24.6060001447456));
#61632=CARTESIAN_POINT('Ctrl Pts',(0.853533015103848,-12.2762488605904,
24.6064014130275));
#61633=CARTESIAN_POINT('Ctrl Pts',(0.869975406804535,-12.2754546381132,
24.6067467875715));
#61634=CARTESIAN_POINT('Ctrl Pts',(0.954838144713319,-12.2713554842222,
24.6085293402528));
#61635=CARTESIAN_POINT('Ctrl Pts',(1.03908076610755,-12.2666952328111,24.6105599527878));
#61636=CARTESIAN_POINT('Ctrl Pts',(1.12269744174171,-12.2615009244909,24.6128288068564));
#61637=CARTESIAN_POINT('Ctrl Pts',(1.34022666710179,-12.2479879038332,24.6187312427553));
#61638=CARTESIAN_POINT('Ctrl Pts',(1.55351828284116,-12.2308639657858,24.6262450190716));
#61639=CARTESIAN_POINT('Ctrl Pts',(1.76257209799047,-12.2106134075563,24.6351868042739));
#61640=CARTESIAN_POINT('Ctrl Pts',(1.93920899338593,-12.193503001161,24.6427420319854));
#61641=CARTESIAN_POINT('Ctrl Pts',(2.1128209108483,-12.1741595331882,24.6513170009043));
#61642=CARTESIAN_POINT('Ctrl Pts',(2.28341906446789,-12.1528496006427,24.6608086010793));
#61643=CARTESIAN_POINT('Ctrl Pts',(2.31450099185576,-12.1489670628663,24.6625379118671));
#61644=CARTESIAN_POINT('Ctrl Pts',(2.34548290429981,-12.1450191894154,24.6642976673795));
#61645=CARTESIAN_POINT('Ctrl Pts',(2.37636489708942,-12.1410075682698,24.6660872274319));
#61646=CARTESIAN_POINT('Ctrl Pts',(2.47701179056917,-12.1279333729328,24.6719195472952));
#61647=CARTESIAN_POINT('Ctrl Pts',(2.57747204661453,-12.1140718251945,24.6781174316816));
#61648=CARTESIAN_POINT('Ctrl Pts',(2.67697489282744,-12.0995577541734,24.6846234144293));
#61649=CARTESIAN_POINT('Ctrl Pts',(2.77861440864647,-12.0847320159428,24.6912691030861));
#61650=CARTESIAN_POINT('Ctrl Pts',(2.8792548073093,-12.0692255340046,24.6982362519364));
#61651=CARTESIAN_POINT('Ctrl Pts',(2.9780848394563,-12.0532304524573,24.7054405178432));
#61652=CARTESIAN_POINT('Ctrl Pts',(3.0123039965395,-12.0476922754868,24.707934940858));
#61653=CARTESIAN_POINT('Ctrl Pts',(3.04630621857371,-12.0420959332209,24.7104575923126));
#61654=CARTESIAN_POINT('Ctrl Pts',(3.08005815461792,-12.0364506606366,24.7130043583632));
#61655=CARTESIAN_POINT('Ctrl Pts',(3.15872540585718,-12.0232929538869,24.7189402277749));
#61656=CARTESIAN_POINT('Ctrl Pts',(3.23624816580929,-12.0098356819973,24.7250222887154));
#61657=CARTESIAN_POINT('Ctrl Pts',(3.31262495126853,-11.9961231064857,24.7312311044611));
#61658=CARTESIAN_POINT('Ctrl Pts',(3.45631259761645,-11.9703256382004,24.7429117495125));
#61659=CARTESIAN_POINT('Ctrl Pts',(3.59594394370824,-11.9436260683294,24.7550405618913));
#61660=CARTESIAN_POINT('Ctrl Pts',(3.73152323809938,-11.9163084789191,24.7674937459439));
#61661=CARTESIAN_POINT('Ctrl Pts',(3.83534629158847,-11.895389388292,24.7770300663666));
#61662=CARTESIAN_POINT('Ctrl Pts',(3.93679211525432,-11.8741075813535,24.7867566625271));
#61663=CARTESIAN_POINT('Ctrl Pts',(4.03586070844626,-11.8525830145618,24.7966201217043));
#61664=CARTESIAN_POINT('Ctrl Pts',(4.06062785674425,-11.8472018728639,24.7990859864985));
#61665=CARTESIAN_POINT('Ctrl Pts',(4.08626076073108,-11.8415877062263,24.8016601504212));
#61666=CARTESIAN_POINT('Ctrl Pts',(4.11422298318758,-11.835398101637,24.8045003838752));
#61667=CARTESIAN_POINT('Ctrl Pts',(4.14218520564409,-11.8292084970477,24.8073406173293));
#61668=CARTESIAN_POINT('Ctrl Pts',(4.16996881025387,-11.8229965347247,24.8101932086679));
#61669=CARTESIAN_POINT('Ctrl Pts',(4.1975737970365,-11.8167648448493,24.8130569697881));
#61670=CARTESIAN_POINT('Ctrl Pts',(4.20543951623015,-11.8149891974618,24.8138729651366));
#61671=CARTESIAN_POINT('Ctrl Pts',(4.21329073408853,-11.8132119477631,24.8146898676183));
#61672=CARTESIAN_POINT('Ctrl Pts',(4.22112745001383,-11.8114331549952,24.8155076504106));
#61673=CARTESIAN_POINT('Ctrl Pts',(4.26829713190448,-11.8007264903911,24.8204299360386));
#61674=CARTESIAN_POINT('Ctrl Pts',(4.3149414118535,-11.7899639527628,24.8253841062339));
#61675=CARTESIAN_POINT('Ctrl Pts',(4.36106030408131,-11.77915846756,24.8303645098757));
#61676=CARTESIAN_POINT('Ctrl Pts',(4.5190215100943,-11.742148743524,24.8474228243255));
#61677=CARTESIAN_POINT('Ctrl Pts',(4.67082010192686,-11.7046406077475,24.8647871087404));
#61678=CARTESIAN_POINT('Ctrl Pts',(4.81645382359858,-11.6671135529552,24.8822424723097));
#61679=CARTESIAN_POINT('Ctrl Pts',(4.86915567872832,-11.6535332819685,24.8885592101608));
#61680=CARTESIAN_POINT('Ctrl Pts',(4.9210503274101,-11.6399500662591,24.8948880037593));
#61681=CARTESIAN_POINT('Ctrl Pts',(4.97213805285758,-11.6263850694136,24.9012191073043));
#61682=CARTESIAN_POINT('Ctrl Pts',(5.00446500995171,-11.6178014993453,24.9052252616372));
#61683=CARTESIAN_POINT('Ctrl Pts',(5.03646882664084,-11.6092260567639,24.9092319631941));
#61684=CARTESIAN_POINT('Ctrl Pts',(5.06814946717143,-11.6006633548531,24.9132370544178));
#61685=CARTESIAN_POINT('Ctrl Pts',(5.21038741293057,-11.562219020725,24.9312188861827));
#61686=CARTESIAN_POINT('Ctrl Pts',(5.34611056112384,-11.5240356189547,24.9491675989117));
#61687=CARTESIAN_POINT('Ctrl Pts',(5.47531845837768,-11.4865046012324,24.9669050009867));
#61688=CARTESIAN_POINT('Ctrl Pts',(5.60704277519038,-11.4482426391245,24.984987852113));
#61689=CARTESIAN_POINT('Ctrl Pts',(5.73199578464032,-11.4106585980952,25.0028509325174));
#61690=CARTESIAN_POINT('Ctrl Pts',(5.85017903341744,-11.3741144711569,25.0203156695206));
#61691=CARTESIAN_POINT('Ctrl Pts',(5.86231997951077,-11.3703602988882,25.0221098191373));
#61692=CARTESIAN_POINT('Ctrl Pts',(5.87438948168156,-11.3666170571579,25.0238997747802));
#61693=CARTESIAN_POINT('Ctrl Pts',(5.88638754150042,-11.3628851084615,25.0256853498019));
#61694=CARTESIAN_POINT('Ctrl Pts',(5.9210293540039,-11.3521099107238,25.0308408129391));
#61695=CARTESIAN_POINT('Ctrl Pts',(5.95507558688705,-11.3414288775921,25.0359597592798));
#61696=CARTESIAN_POINT('Ctrl Pts',(5.98852582557976,-11.3308501354331,25.0410382779965));
#61697=CARTESIAN_POINT('',(-6.27159361731041,-11.8794975616087,24.2690120888651));
#61698=CARTESIAN_POINT('Origin',(-5.9999949808,-10.9277770011797,24.1259380084106));
#61699=CARTESIAN_POINT('Ctrl Pts',(-6.27159386307184,-11.8794985003198,
24.2690123724987));
#61700=CARTESIAN_POINT('Ctrl Pts',(-6.19708064714059,-11.9025009409338,
24.2574475533713));
#61701=CARTESIAN_POINT('Ctrl Pts',(-6.11543894003613,-11.9272858575891,
24.2450493547133));
#61702=CARTESIAN_POINT('Ctrl Pts',(-6.02658470930716,-11.9536191428594,
24.2319368725984));
#61703=CARTESIAN_POINT('Ctrl Pts',(-5.93855995222029,-11.9797066011628,
24.2189467983666));
#61704=CARTESIAN_POINT('Ctrl Pts',(-5.84345655035932,-12.0073137872402,
24.2052557335694));
#61705=CARTESIAN_POINT('Ctrl Pts',(-5.7411838234057,-12.0361672792979,24.1909996691092));
#61706=CARTESIAN_POINT('Ctrl Pts',(-5.64049533840775,-12.0645738202079,
24.1769644363028));
#61707=CARTESIAN_POINT('Ctrl Pts',(-5.53285775062703,-12.0941884570633,
24.1623816092192));
#61708=CARTESIAN_POINT('Ctrl Pts',(-5.41817817581817,-12.1247040018455,
24.1474001817781));
#61709=CARTESIAN_POINT('Ctrl Pts',(-5.37925167383706,-12.1350621097858,
24.1423149295356));
#61710=CARTESIAN_POINT('Ctrl Pts',(-5.33951376816848,-12.1455236128537,
24.1371839145072));
#61711=CARTESIAN_POINT('Ctrl Pts',(-5.2989607104461,-12.1560752216459,24.1320134677298));
#61712=CARTESIAN_POINT('Ctrl Pts',(-5.21821245862246,-12.1770853257353,
24.1217182011858));
#61713=CARTESIAN_POINT('Ctrl Pts',(-5.13423231221224,-12.1984533510321,
24.1112662369327));
#61714=CARTESIAN_POINT('Ctrl Pts',(-5.0469909259153,-12.2200666319346,24.1007138157334));
#61715=CARTESIAN_POINT('Ctrl Pts',(-4.92201084106593,-12.2510293412144,
24.085596649984));
#61716=CARTESIAN_POINT('Ctrl Pts',(-4.79033765404794,-12.2824975295437,
24.0702722548015));
#61717=CARTESIAN_POINT('Ctrl Pts',(-4.65188544733252,-12.3141001739185,
24.0549257642203));
#61718=CARTESIAN_POINT('Ctrl Pts',(-4.5134332406171,-12.3457028182933,24.039579273639));
#61719=CARTESIAN_POINT('Ctrl Pts',(-4.36820181664654,-12.3774401803882,
24.0242105653309));
#61720=CARTESIAN_POINT('Ctrl Pts',(-4.21610826590916,-12.4088909807736,
24.0090296785428));
#61721=CARTESIAN_POINT('Ctrl Pts',(-4.07082504414953,-12.4389335012141,
23.9945285499213));
#61722=CARTESIAN_POINT('Ctrl Pts',(-3.91927991557136,-12.4687142331352,
23.9801988310894));
#61723=CARTESIAN_POINT('Ctrl Pts',(-3.76141769099652,-12.4978253761718,
23.966247356158));
#61724=CARTESIAN_POINT('Ctrl Pts',(-3.73054470085429,-12.5035186193426,
23.9635188772633));
#61725=CARTESIAN_POINT('Ctrl Pts',(-3.69943013468555,-12.5091861150751,
23.9608049377641));
#61726=CARTESIAN_POINT('Ctrl Pts',(-3.66807363502218,-12.514824609958,23.9581071920514));
#61727=CARTESIAN_POINT('Ctrl Pts',(-3.58017498710756,-12.5306304582447,
23.9505448619729));
#61728=CARTESIAN_POINT('Ctrl Pts',(-3.49037513941867,-12.5462087327828,
23.9431096159783));
#61729=CARTESIAN_POINT('Ctrl Pts',(-3.39866711822361,-12.5614848718521,
23.9358394498037));
#61730=CARTESIAN_POINT('Ctrl Pts',(-3.35281310762608,-12.5691229413868,
23.9322043667164));
#61731=CARTESIAN_POINT('Ctrl Pts',(-3.30648204469947,-12.5766854194222,
23.9286105469247));
#61732=CARTESIAN_POINT('Ctrl Pts',(-3.25967322796412,-12.5841625638991,
23.9250630077419));
#61733=CARTESIAN_POINT('Ctrl Pts',(-3.23626881959645,-12.5879011361376,
23.9232892381504));
#61734=CARTESIAN_POINT('Ctrl Pts',(-3.21274497218075,-12.5916183713035,
23.9215270382812));
#61735=CARTESIAN_POINT('Ctrl Pts',(-3.18910160199944,-12.595313027064,23.9197770418822));
#61736=CARTESIAN_POINT('Ctrl Pts',(-3.17727991690878,-12.5971603549442,
23.9189020436828));
#61737=CARTESIAN_POINT('Ctrl Pts',(-3.16542835109203,-12.5990020377369,
23.918030096324));
#61738=CARTESIAN_POINT('Ctrl Pts',(-3.15354689471706,-12.6008379184752,
23.9171612799832));
#61739=CARTESIAN_POINT('Ctrl Pts',(-3.1416654383421,-12.6026737992134,23.9162924636424));
#61740=CARTESIAN_POINT('Ctrl Pts',(-3.1281400511785,-12.6047504351401,23.9153102018295));
#61741=CARTESIAN_POINT('Ctrl Pts',(-3.11781284420954,-12.6063279965277,
23.9145643044261));
#61742=CARTESIAN_POINT('Ctrl Pts',(-3.07661938484431,-12.6126206186387,
23.9115890474692));
#61743=CARTESIAN_POINT('Ctrl Pts',(-3.03568519935775,-12.6187487292425,
23.9086931412116));
#61744=CARTESIAN_POINT('Ctrl Pts',(-2.99501202309511,-12.6247166820769,
23.9058744407652));
#61745=CARTESIAN_POINT('Ctrl Pts',(-2.79739625318866,-12.6537127355573,
23.8921794282279));
#61746=CARTESIAN_POINT('Ctrl Pts',(-2.60594586740788,-12.6789296984963,
23.8803064010344));
#61747=CARTESIAN_POINT('Ctrl Pts',(-2.42085391603547,-12.7008778071539,
23.870005028324));
#61748=CARTESIAN_POINT('Ctrl Pts',(-2.23092606413269,-12.723399354416,23.8594345114753));
#61749=CARTESIAN_POINT('Ctrl Pts',(-2.04769292395376,-12.7424793193334,
23.8505186523863));
#61750=CARTESIAN_POINT('Ctrl Pts',(-1.87131426315632,-12.7586451232207,
23.8429958321136));
#61751=CARTESIAN_POINT('Ctrl Pts',(-1.78116939726151,-12.7669072577495,
23.8391510153905));
#61752=CARTESIAN_POINT('Ctrl Pts',(-1.69281424560786,-12.7744077750593,
23.8356702336904));
#61753=CARTESIAN_POINT('Ctrl Pts',(-1.60626582519892,-12.7812143692985,
23.8325196677634));
#61754=CARTESIAN_POINT('Ctrl Pts',(-1.43907203963571,-12.7943633124251,
23.8264334209953));
#61755=CARTESIAN_POINT('Ctrl Pts',(-1.27862277410174,-12.8049251375061,
23.8215784341343));
#61756=CARTESIAN_POINT('Ctrl Pts',(-1.1250175870215,-12.8133803812603,23.8177150430602));
#61757=CARTESIAN_POINT('Ctrl Pts',(-0.969940669440592,-12.8219166368629,
23.8138146358503));
#61758=CARTESIAN_POINT('Ctrl Pts',(-0.821839215358774,-12.8283058798147,
23.8109248045128));
#61759=CARTESIAN_POINT('Ctrl Pts',(-0.680783296076854,-12.8330036704535,
23.8088159024075));
#61760=CARTESIAN_POINT('Ctrl Pts',(-0.53838902393423,-12.837746034206,23.8066869908252));
#61761=CARTESIAN_POINT('Ctrl Pts',(-0.403174234552946,-12.8407648333977,
23.8053537869326));
#61762=CARTESIAN_POINT('Ctrl Pts',(-0.275184076784705,-12.8424872179352,
23.8045989542072));
#61763=CARTESIAN_POINT('Ctrl Pts',(-0.236233659390891,-12.8430113800881,
23.804369240843));
#61764=CARTESIAN_POINT('Ctrl Pts',(-0.197952170246763,-12.8434151814382,
23.8041932297371));
#61765=CARTESIAN_POINT('Ctrl Pts',(-0.160340475176224,-12.8437098785878,
23.8040651618987));
#61766=CARTESIAN_POINT('Ctrl Pts',(-0.154018237855442,-12.8437594149172,
23.8040436346779));
#61767=CARTESIAN_POINT('Ctrl Pts',(-0.147714925196181,-12.8438058676637,
23.8040234624916));
#61768=CARTESIAN_POINT('Ctrl Pts',(-0.141430540525102,-12.8438492902627,
23.8040046172673));
#61769=CARTESIAN_POINT('Ctrl Pts',(-0.103048091275479,-12.8441144977235,
23.8038895183507));
#61770=CARTESIAN_POINT('Ctrl Pts',(-0.0662562838150946,-12.8442643991019,
23.8038251218336));
#61771=CARTESIAN_POINT('Ctrl Pts',(-0.0289819554348571,-12.844317014175,
23.8038019501873));
#61772=CARTESIAN_POINT('Ctrl Pts',(-0.0185596180577554,-12.8443317259637,
23.8037954711245));
#61773=CARTESIAN_POINT('Ctrl Pts',(-0.00809955461635552,-12.844338555091,
23.8037923587938));
#61774=CARTESIAN_POINT('Ctrl Pts',(0.00244355647455851,-12.844337252009,
23.803792740049));
#61775=CARTESIAN_POINT('Ctrl Pts',(0.127128013150683,-12.8443218415601,
23.8037972488312));
#61776=CARTESIAN_POINT('Ctrl Pts',(0.258986464546909,-12.8431696756197,
23.8042924754873));
#61777=CARTESIAN_POINT('Ctrl Pts',(0.397985692314567,-12.8404650149112,
23.8054910559536));
#61778=CARTESIAN_POINT('Ctrl Pts',(0.535666794351003,-12.8377860024234,
23.8066782703155));
#61779=CARTESIAN_POINT('Ctrl Pts',(0.680354207936333,-12.833583687344,23.8085556447809));
#61780=CARTESIAN_POINT('Ctrl Pts',(0.831993697184611,-12.8274126453801,
23.8113495723966));
#61781=CARTESIAN_POINT('Ctrl Pts',(0.94225644354008,-12.8229254498733,23.8133811417033));
#61782=CARTESIAN_POINT('Ctrl Pts',(1.05619452308235,-12.8173964738687,23.8158977309064));
#61783=CARTESIAN_POINT('Ctrl Pts',(1.17377814699504,-12.8106410003335,23.8189926615624));
#61784=CARTESIAN_POINT('Ctrl Pts',(1.33433786019959,-12.8014164428886,23.8232187702838));
#61785=CARTESIAN_POINT('Ctrl Pts',(1.50169675089625,-12.7899057935866,23.8285229658335));
#61786=CARTESIAN_POINT('Ctrl Pts',(1.6757438097164,-12.7756233796364,23.8351480557093));
#61787=CARTESIAN_POINT('Ctrl Pts',(1.84376169748946,-12.7618357233527,23.8415436455848));
#61788=CARTESIAN_POINT('Ctrl Pts',(2.01801263886451,-12.7454647212648,23.8491703749819));
#61789=CARTESIAN_POINT('Ctrl Pts',(2.19836007197658,-12.7260475718018,23.8582571266038));
#61790=CARTESIAN_POINT('Ctrl Pts',(2.26107777821509,-12.7192950549792,23.8614171395247));
#61791=CARTESIAN_POINT('Ctrl Pts',(2.32453242794122,-12.7121739290865,23.8647538068919));
#61792=CARTESIAN_POINT('Ctrl Pts',(2.38871710222971,-12.7046640542677,23.8682770054759));
#61793=CARTESIAN_POINT('Ctrl Pts',(2.47498633891838,-12.6945701934602,23.8730124607214));
#61794=CARTESIAN_POINT('Ctrl Pts',(2.5625744551735,-12.6837740476544,23.8780848912508));
#61795=CARTESIAN_POINT('Ctrl Pts',(2.65146478041537,-12.6722277327554,23.8835179409207));
#61796=CARTESIAN_POINT('Ctrl Pts',(2.72897733062453,-12.6621593219255,23.8882555716379));
#61797=CARTESIAN_POINT('Ctrl Pts',(2.80748007424341,-12.6515204683365,23.8932674718265));
#61798=CARTESIAN_POINT('Ctrl Pts',(2.88696072282057,-12.6402790211584,23.8985693908055));
#61799=CARTESIAN_POINT('Ctrl Pts',(2.92670104710914,-12.6346582975693,23.9012203502951));
#61800=CARTESIAN_POINT('Ctrl Pts',(2.96668584644875,-12.6288869179267,23.9039438136002));
#61801=CARTESIAN_POINT('Ctrl Pts',(3.00691346377708,-12.6229608302188,23.9067417754196));
#61802=CARTESIAN_POINT('Ctrl Pts',(3.02702727244124,-12.6199977863648,23.9081407563294));
#61803=CARTESIAN_POINT('Ctrl Pts',(3.04720178554791,-12.6169960650334,23.9095583618172));
#61804=CARTESIAN_POINT('Ctrl Pts',(3.06743679137486,-12.6139551575869,23.9109948405961));
#61805=CARTESIAN_POINT('Ctrl Pts',(3.07755429428834,-12.6124347038637,23.9117130799855));
#61806=CARTESIAN_POINT('Ctrl Pts',(3.08768692037775,-12.6109044535828,23.9124360376945));
#61807=CARTESIAN_POINT('Ctrl Pts',(3.09783464270007,-12.6093643430508,23.9131637448486));
#61808=CARTESIAN_POINT('Ctrl Pts',(3.10798236502239,-12.6078242325187,23.9138914520027));
#61809=CARTESIAN_POINT('Ctrl Pts',(3.11649244848053,-12.6065275650744,23.9145041924201));
#61810=CARTESIAN_POINT('Ctrl Pts',(3.12832307126662,-12.6047143669116,23.915361145775));
#61811=CARTESIAN_POINT('Ctrl Pts',(3.24396552605183,-12.5869906434566,23.9237377284268));
#61812=CARTESIAN_POINT('Ctrl Pts',(3.35681651989267,-12.5687093250851,23.9324152959104));
#61813=CARTESIAN_POINT('Ctrl Pts',(3.46688415179261,-12.5500070581239,23.9413237929068));
#61814=CARTESIAN_POINT('Ctrl Pts',(3.63912326404861,-12.5207408533099,23.9552642365022));
#61815=CARTESIAN_POINT('Ctrl Pts',(3.80454615891661,-12.4904466297004,23.9697687507377));
#61816=CARTESIAN_POINT('Ctrl Pts',(3.96320907665928,-12.4596127305724,23.9845897060615));
#61817=CARTESIAN_POINT('Ctrl Pts',(4.12187199440194,-12.4287788314444,23.9994106613853));
#61818=CARTESIAN_POINT('Ctrl Pts',(4.27377520622497,-12.3974049903084,24.0145481991502));
#61819=CARTESIAN_POINT('Ctrl Pts',(4.41898721777619,-12.3659267693461,24.0297822509075));
#61820=CARTESIAN_POINT('Ctrl Pts',(4.56351696175518,-12.3345964464066,24.0449447266334));
#61821=CARTESIAN_POINT('Ctrl Pts',(4.70141874662422,-12.3031625796294,24.0602030464379));
#61822=CARTESIAN_POINT('Ctrl Pts',(4.83277339477483,-12.2720089508995,24.0753670005252));
#61823=CARTESIAN_POINT('Ctrl Pts',(4.90532264871698,-12.254802308015,24.0837422926929));
#61824=CARTESIAN_POINT('Ctrl Pts',(4.975874747427,-12.2376802960697,24.0920892107805));
#61825=CARTESIAN_POINT('Ctrl Pts',(5.04444361185108,-12.2207014895619,24.1003786510992));
#61826=CARTESIAN_POINT('Ctrl Pts',(5.13538803840724,-12.198182116747,24.1113731221698));
#61827=CARTESIAN_POINT('Ctrl Pts',(5.22284371582237,-12.1759150854809,24.1222662743539));
#61828=CARTESIAN_POINT('Ctrl Pts',(5.3068432141015,-12.1540259495273,24.1329956083273));
#61829=CARTESIAN_POINT('Ctrl Pts',(5.42689803314422,-12.122741283431,24.1483303219271));
#61830=CARTESIAN_POINT('Ctrl Pts',(5.53989334717833,-12.0922305098064,24.1633297223276));
#61831=CARTESIAN_POINT('Ctrl Pts',(5.64592620334713,-12.0628176246999,24.1778361176492));
#61832=CARTESIAN_POINT('Ctrl Pts',(5.75378553571296,-12.0328980859346,24.192592393873));
#61833=CARTESIAN_POINT('Ctrl Pts',(5.85444062957484,-12.0041144877992,24.2068385125593));
#61834=CARTESIAN_POINT('Ctrl Pts',(5.94798628536258,-11.976758368691,24.2204298262157));
#61835=CARTESIAN_POINT('Ctrl Pts',(6.02496352185606,-11.9542474521508,24.2316139026625));
#61836=CARTESIAN_POINT('Ctrl Pts',(6.09712657776811,-11.9327021773434,24.2423549858525));
#61837=CARTESIAN_POINT('Ctrl Pts',(6.16452362202879,-11.9122612713575,24.2525831370081));
#61838=CARTESIAN_POINT('Ctrl Pts',(6.20165855736736,-11.9009985857253,24.2582187214163));
#61839=CARTESIAN_POINT('Ctrl Pts',(6.23734650792921,-11.8900707994031,24.2636987908079));
#61840=CARTESIAN_POINT('Ctrl Pts',(6.27159479316527,-11.8794983798055,24.2690136880117));
#61841=CARTESIAN_POINT('Ctrl Pts',(-6.390311350328,-11.8061935254293,24.5118466387929));
#61842=CARTESIAN_POINT('Ctrl Pts',(-4.260207566885,-12.4817978211448,24.1870549186574));
#61843=CARTESIAN_POINT('Ctrl Pts',(0.0001663377189254,-13.1582627349181,
23.8622596453287));
#61844=CARTESIAN_POINT('Ctrl Pts',(4.260540242323,-12.4817449966618,24.187080281601));
#61845=CARTESIAN_POINT('Ctrl Pts',(6.390810363485,-11.8060352474225,24.5119227297642));
#61846=CARTESIAN_POINT('Ctrl Pts',(-6.390311350328,-11.9720500990187,23.5458954363187));
#61847=CARTESIAN_POINT('Ctrl Pts',(-4.260207566885,-12.6077625183053,23.2652555130157));
#61848=CARTESIAN_POINT('Ctrl Pts',(0.0001663377189254,-13.2461470236974,
22.9846373688158));
#61849=CARTESIAN_POINT('Ctrl Pts',(4.260540242323,-12.6077126674846,23.2652774262116));
#61850=CARTESIAN_POINT('Ctrl Pts',(6.390810363485,-11.9719011667457,23.5459611835739));
#61851=CARTESIAN_POINT('Ctrl Pts',(-6.390311350328,-12.0713617692531,21.4528915452424));
#61852=CARTESIAN_POINT('Ctrl Pts',(-4.260207566885,-12.659242522167,21.2792390801719));
#61853=CARTESIAN_POINT('Ctrl Pts',(0.0001663377189254,-13.2456907932709,
21.1056336066131));
#61854=CARTESIAN_POINT('Ctrl Pts',(4.260540242323,-12.6591967269967,21.279252636856));
#61855=CARTESIAN_POINT('Ctrl Pts',(6.390810363485,-12.0712240427635,21.4529322278795));
#61856=CARTESIAN_POINT('Ctrl Pts',(-6.390311350328,-11.3879808552225,18.3168609136282));
#61857=CARTESIAN_POINT('Ctrl Pts',(-4.260207566885,-12.0191856806185,18.3050659001811));
#61858=CARTESIAN_POINT('Ctrl Pts',(0.0001663377189254,-12.6510858023129,
18.2929947474269));
#61859=CARTESIAN_POINT('Ctrl Pts',(4.260540242323,-12.0191363361555,18.3050668428024));
#61860=CARTESIAN_POINT('Ctrl Pts',(6.390810363485,-11.3878329789516,18.3168636769094));
#61861=CARTESIAN_POINT('Ctrl Pts',(-6.390311350328,-9.96973039617433,15.6641171406436));
#61862=CARTESIAN_POINT('Ctrl Pts',(-4.260207566885,-10.7489883683133,15.7526875000242));
#61863=CARTESIAN_POINT('Ctrl Pts',(0.0001663377189254,-11.5273045000232,
15.8421713762416));
#61864=CARTESIAN_POINT('Ctrl Pts',(4.260540242323,-10.748927590366,15.7526805123096));
#61865=CARTESIAN_POINT('Ctrl Pts',(6.390810363485,-9.9695478345618,15.6640963907245));
#61866=CARTESIAN_POINT('Ctrl Pts',(-6.390311350328,-8.71308977409159,14.2543209333947));
#61867=CARTESIAN_POINT('Ctrl Pts',(-4.260207566885,-9.62712791089626,14.3567599107344));
#61868=CARTESIAN_POINT('Ctrl Pts',(0.0001663377189254,-10.542551067134,
14.4578276726223));
#61869=CARTESIAN_POINT('Ctrl Pts',(4.260540242323,-9.62705642639862,14.3567520184532));
#61870=CARTESIAN_POINT('Ctrl Pts',(6.390810363485,-8.71287563671292,14.2542969343644));
#61871=CARTESIAN_POINT('Ctrl Pts',(-6.390311350328,-8.1393678365502,13.7249554217385));
#61872=CARTESIAN_POINT('Ctrl Pts',(-4.260207566885,-9.11425616282747,13.8221631313431));
#61873=CARTESIAN_POINT('Ctrl Pts',(0.0001663377189254,-10.0902570778465,
13.9182879348291));
#61874=CARTESIAN_POINT('Ctrl Pts',(4.260540242323,-9.11417994787105,13.8221556250518));
#61875=CARTESIAN_POINT('Ctrl Pts',(6.390810363485,-8.13913944341977,13.7249326482792));
#61876=CARTESIAN_POINT('',(-6.26386060047837,-8.42071136785102,13.944258352743));
#61877=CARTESIAN_POINT('Ctrl Pts',(-6.27159552384391,-11.8794980574192,
24.2690121660514));
#61878=CARTESIAN_POINT('Ctrl Pts',(-6.27195777356616,-11.915653437869,24.0278185457168));
#61879=CARTESIAN_POINT('Ctrl Pts',(-6.27229031321601,-11.9441024432717,
23.7878332652866));
#61880=CARTESIAN_POINT('Ctrl Pts',(-6.27259314303954,-11.9652318790949,
23.5495554059373));
#61881=CARTESIAN_POINT('Ctrl Pts',(-6.27289863569945,-11.9865471097967,
23.3091823270881));
#61882=CARTESIAN_POINT('Ctrl Pts',(-6.27317389374832,-12.0004135038023,
23.0705467396266));
#61883=CARTESIAN_POINT('Ctrl Pts',(-6.27341891743877,-12.0072245116416,
22.8341074875309));
#61884=CARTESIAN_POINT('Ctrl Pts',(-6.27366754257446,-12.0141356300935,
22.5941929673217));
#61885=CARTESIAN_POINT('Ctrl Pts',(-6.27388503802917,-12.0137824618086,
22.3565397769456));
#61886=CARTESIAN_POINT('Ctrl Pts',(-6.27407140406683,-12.0065719197372,
22.1215733736428));
#61887=CARTESIAN_POINT('Ctrl Pts',(-6.2742180445919,-12.0008983662902,21.9366920659419));
#61888=CARTESIAN_POINT('Ctrl Pts',(-6.27434541228839,-11.9909792002045,
21.7534731040869));
#61889=CARTESIAN_POINT('Ctrl Pts',(-6.27445350728488,-11.9770107165648,
21.5721011929025));
#61890=CARTESIAN_POINT('Ctrl Pts',(-6.274502629551,-11.9706629336613,21.4896792531497));
#61891=CARTESIAN_POINT('Ctrl Pts',(-6.27454777177045,-11.9634789140546,
21.4076384849629));
#61892=CARTESIAN_POINT('Ctrl Pts',(-6.27458893395529,-11.9554822034544,
21.3259945718025));
#61893=CARTESIAN_POINT('Ctrl Pts',(-6.274707125726,-11.9325207064088,21.0915648713221));
#61894=CARTESIAN_POINT('Ctrl Pts',(-6.27479250271421,-11.9028603482648,
20.8604109425169));
#61895=CARTESIAN_POINT('Ctrl Pts',(-6.27484506491992,-11.8670439537005,
20.6328687479079));
#61896=CARTESIAN_POINT('Ctrl Pts',(-6.27489762712562,-11.8312275591362,
20.4053265532988));
#61897=CARTESIAN_POINT('Ctrl Pts',(-6.27491737454883,-11.7892550892312,
20.1813959027504));
#61898=CARTESIAN_POINT('Ctrl Pts',(-6.27490430718954,-11.7416481920867,
19.9613626470728));
#61899=CARTESIAN_POINT('Ctrl Pts',(-6.27489476683278,-11.7068908418988,
19.8007184257666));
#61900=CARTESIAN_POINT('Ctrl Pts',(-6.2748675368223,-11.6690630215386,19.6418631629783));
#61901=CARTESIAN_POINT('Ctrl Pts',(-6.27482283433795,-11.6284198495329,
19.4852105192767));
#61902=CARTESIAN_POINT('Ctrl Pts',(-6.2747779149856,-11.5875795027186,19.3277978966284));
#61903=CARTESIAN_POINT('Ctrl Pts',(-6.27471535321751,-11.5438966073892,
19.1726096136311));
#61904=CARTESIAN_POINT('Ctrl Pts',(-6.27463536938977,-11.4976754978955,
19.0200386342048));
#61905=CARTESIAN_POINT('Ctrl Pts',(-6.27457690215347,-11.4638884110919,
18.9085110447105));
#61906=CARTESIAN_POINT('Ctrl Pts',(-6.27450912554786,-11.4287460092372,
18.7983814464739));
#61907=CARTESIAN_POINT('Ctrl Pts',(-6.27443212564381,-11.3923814819426,
18.6897930754465));
#61908=CARTESIAN_POINT('Ctrl Pts',(-6.2743563538205,-11.3565969368728,18.5829365934247));
#61909=CARTESIAN_POINT('Ctrl Pts',(-6.27427024653004,-11.3190562665239,
18.4758584939686));
#61910=CARTESIAN_POINT('Ctrl Pts',(-6.27417380377242,-11.279707466543,18.3686262100674));
#61911=CARTESIAN_POINT('Ctrl Pts',(-6.27399075391238,-11.2050228296955,
18.1650976606481));
#61912=CARTESIAN_POINT('Ctrl Pts',(-6.27377047091144,-11.1238233577958,
17.9610107904066));
#61913=CARTESIAN_POINT('Ctrl Pts',(-6.2735129547696,-11.0358409761326,17.7568349441134));
#61914=CARTESIAN_POINT('Ctrl Pts',(-6.27325823077298,-10.9488125524818,
17.5548728954104));
#61915=CARTESIAN_POINT('Ctrl Pts',(-6.27296707666657,-10.8551474376645,
17.3528237006521));
#61916=CARTESIAN_POINT('Ctrl Pts',(-6.27263949245036,-10.7546000178705,
17.1511902357532));
#61917=CARTESIAN_POINT('Ctrl Pts',(-6.27231699539509,-10.6556140313846,
16.9526880019566));
#61918=CARTESIAN_POINT('Ctrl Pts',(-6.27195919091438,-10.5499577801541,
16.754588644364));
#61919=CARTESIAN_POINT('Ctrl Pts',(-6.27156607900826,-10.4374113233089,
16.5574202692555));
#61920=CARTESIAN_POINT('Ctrl Pts',(-6.27136274846917,-10.3791985564473,
16.4554382346859));
#61921=CARTESIAN_POINT('Ctrl Pts',(-6.27114997212718,-10.319142693358,16.3537060639873));
#61922=CARTESIAN_POINT('Ctrl Pts',(-6.27092774998227,-10.2572149239311,
16.2523020893105));
#61923=CARTESIAN_POINT('Ctrl Pts',(-6.270506080497,-10.139706155087,16.0598866942392));
#61924=CARTESIAN_POINT('Ctrl Pts',(-6.27005040092663,-10.0154565177156,
15.8686500111997));
#61925=CARTESIAN_POINT('Ctrl Pts',(-6.26956071122401,-9.88428092908672,
15.6791641145428));
#61926=CARTESIAN_POINT('Ctrl Pts',(-6.269385046217,-9.83722467984934,15.6111903728333));
#61927=CARTESIAN_POINT('Ctrl Pts',(-6.26920500460963,-9.78927731157033,
15.5434423912217));
#61928=CARTESIAN_POINT('Ctrl Pts',(-6.26902058639972,-9.74043078973703,
15.4759481428237));
#61929=CARTESIAN_POINT('Ctrl Pts',(-6.26850853728607,-9.60480525567523,
15.2885459872248));
#61930=CARTESIAN_POINT('Ctrl Pts',(-6.26796274757707,-9.46224556682946,
15.103096995557));
#61931=CARTESIAN_POINT('Ctrl Pts',(-6.26738321722616,-9.31269176801434,
14.9201584331212));
#61932=CARTESIAN_POINT('Ctrl Pts',(-6.26681230202503,-9.16536119767451,
14.7399393885074));
#61933=CARTESIAN_POINT('Ctrl Pts',(-6.26620864188511,-9.01124286675024,
14.5621566742659));
#61934=CARTESIAN_POINT('Ctrl Pts',(-6.26557223676186,-8.85030877350661,
14.3873838069623));
#61935=CARTESIAN_POINT('Ctrl Pts',(-6.26502582981991,-8.71213341549658,
14.2373267058013));
#61936=CARTESIAN_POINT('Ctrl Pts',(-6.26445528440148,-8.56893413725298,
14.0894889713098));
#61937=CARTESIAN_POINT('Ctrl Pts',(-6.26386060047837,-8.42071136785102,
13.944258352743));
#61938=CARTESIAN_POINT('Ctrl Pts',(6.26385989014072,-8.4207183952526,13.9442649556632));
#61939=CARTESIAN_POINT('Ctrl Pts',(5.97439127923632,-8.54554836940733,13.9556074956481));
#61940=CARTESIAN_POINT('Ctrl Pts',(5.68299007296676,-8.66170806319399,13.9653100424049));
#61941=CARTESIAN_POINT('Ctrl Pts',(5.39014689160465,-8.76905158074534,13.973629824907));
#61942=CARTESIAN_POINT('Ctrl Pts',(5.11540307099319,-8.86976066330876,13.9814353979125));
#61943=CARTESIAN_POINT('Ctrl Pts',(4.83939001142658,-8.96270901393859,13.9880240320898));
#61944=CARTESIAN_POINT('Ctrl Pts',(4.56251287045879,-9.04781787373074,13.9936194822245));
#61945=CARTESIAN_POINT('Ctrl Pts',(4.30529839834099,-9.12688265447598,13.9988175666444));
#61946=CARTESIAN_POINT('Ctrl Pts',(4.04733821401237,-9.19918161327066,14.0031586462239));
#61947=CARTESIAN_POINT('Ctrl Pts',(3.78895714201621,-9.26469470268314,14.0068301382572));
#61948=CARTESIAN_POINT('Ctrl Pts',(3.5726868546934,-9.31953050997035,14.009903252827));
#61949=CARTESIAN_POINT('Ctrl Pts',(3.35612169198377,-9.3696126353749,14.0125073906));
#61950=CARTESIAN_POINT('Ctrl Pts',(3.13945213736916,-9.41495729916426,14.0147564904394));
#61951=CARTESIAN_POINT('Ctrl Pts',(2.89877806005409,-9.46532563604517,14.0172547649644));
#61952=CARTESIAN_POINT('Ctrl Pts',(2.65798320741555,-9.50986231004713,14.0193332725718));
#61953=CARTESIAN_POINT('Ctrl Pts',(2.41731281525442,-9.54854310212053,14.021048344074));
#61954=CARTESIAN_POINT('Ctrl Pts',(2.18015968341001,-9.58665859651125,14.0227383507859));
#61955=CARTESIAN_POINT('Ctrl Pts',(1.94312740078789,-9.61908808142941,14.0240754870134));
#61956=CARTESIAN_POINT('Ctrl Pts',(1.70645060761349,-9.64585877898722,14.0251184015268));
#61957=CARTESIAN_POINT('Ctrl Pts',(1.47135448327552,-9.6724506858542,14.0261543508348));
#61958=CARTESIAN_POINT('Ctrl Pts',(1.23660911590013,-9.69345906616529,14.0269000092261));
#61959=CARTESIAN_POINT('Ctrl Pts',(1.00244447583806,-9.7089616077502,14.0274173350616));
#61960=CARTESIAN_POINT('Ctrl Pts',(0.769963846594297,-9.72435266176066,
14.0279309405135));
#61961=CARTESIAN_POINT('Ctrl Pts',(0.538055622018907,-9.73431674912164,
14.0282194987896));
#61962=CARTESIAN_POINT('Ctrl Pts',(0.30694484651642,-9.73898112574318,14.0283478661244));
#61963=CARTESIAN_POINT('Ctrl Pts',(0.204466564770979,-9.74104938630157,
14.0284047862913));
#61964=CARTESIAN_POINT('Ctrl Pts',(0.102145075869552,-9.74207630888253,
14.0284302647289));
#61965=CARTESIAN_POINT('Ctrl Pts',(-9.86274122834492E-13,-9.74207626567393,
14.028430215033));
#61966=CARTESIAN_POINT('Ctrl Pts',(-0.000185913574553349,-9.74207626559528,
14.0284302149425));
#61967=CARTESIAN_POINT('Ctrl Pts',(-0.000371826563709544,-9.74207626211513,
14.0284302147675));
#61968=CARTESIAN_POINT('Ctrl Pts',(-0.000557738968337773,-9.74207625523356,
14.0284302145081));
#61969=CARTESIAN_POINT('Ctrl Pts',(-0.230883208579248,-9.74206772970903,
14.028429893058));
#61970=CARTESIAN_POINT('Ctrl Pts',(-0.462099352355539,-9.73683400689415,
14.0282994240873));
#61971=CARTESIAN_POINT('Ctrl Pts',(-0.693981990386209,-9.72622568352782,
14.0279722040158));
#61972=CARTESIAN_POINT('Ctrl Pts',(-0.927845006148299,-9.71552676050494,
14.0276421893438));
#61973=CARTESIAN_POINT('Ctrl Pts',(-1.16238594907491,-9.699361051742,14.0271120352145));
#61974=CARTESIAN_POINT('Ctrl Pts',(-1.39737484628166,-9.67762830339212,
14.0263176856921));
#61975=CARTESIAN_POINT('Ctrl Pts',(-1.63392438984921,-9.65575121999055,
14.0255180606067));
#61976=CARTESIAN_POINT('Ctrl Pts',(-1.87092785750831,-9.62823296750948,
14.024450705365));
#61977=CARTESIAN_POINT('Ctrl Pts',(-2.1081506638769,-9.59502420670042,14.023054791648));
#61978=CARTESIAN_POINT('Ctrl Pts',(-2.34834588913176,-9.56139933772146,
14.0216413870314));
#61979=CARTESIAN_POINT('Ctrl Pts',(-2.5887659841926,-9.52194050765764,14.0198911192562));
#61980=CARTESIAN_POINT('Ctrl Pts',(-2.82916743460895,-9.4766498428339,14.017745715887));
#61981=CARTESIAN_POINT('Ctrl Pts',(-2.93286958992579,-9.45711277452661,
14.0168202516146));
#61982=CARTESIAN_POINT('Ctrl Pts',(-3.03656827583359,-9.43649117750807,
14.0158213229269));
#61983=CARTESIAN_POINT('Ctrl Pts',(-3.14024394547988,-9.41478818616068,
14.0147445403436));
#61984=CARTESIAN_POINT('Ctrl Pts',(-3.40299004548275,-9.3597861171663,14.0120156414103));
#61985=CARTESIAN_POINT('Ctrl Pts',(-3.66557749758006,-9.29781677171979,
14.0087642670787));
#61986=CARTESIAN_POINT('Ctrl Pts',(-3.92766690418479,-9.22885719918551,
14.0047880768363));
#61987=CARTESIAN_POINT('Ctrl Pts',(-4.19856644078887,-9.15757955204227,
14.0006782270409));
#61988=CARTESIAN_POINT('Ctrl Pts',(-4.46893388554754,-9.07883436253647,
13.9957939467473));
#61989=CARTESIAN_POINT('Ctrl Pts',(-4.73839445092947,-8.99265632800915,
13.9899207517277));
#61990=CARTESIAN_POINT('Ctrl Pts',(-5.03365159885242,-8.89822811120468,
13.9834852912801));
#61991=CARTESIAN_POINT('Ctrl Pts',(-5.32781991713952,-8.79487607792431,
13.9758622779781));
#61992=CARTESIAN_POINT('Ctrl Pts',(-5.62040634468541,-8.68271089253479,
13.9667825708472));
#61993=CARTESIAN_POINT('Ctrl Pts',(-5.83581409549622,-8.60013272748902,
13.9600979159659));
#61994=CARTESIAN_POINT('Ctrl Pts',(-6.05036443188607,-8.51277917745374,
13.9526239758041));
#61995=CARTESIAN_POINT('Ctrl Pts',(-6.26386060047837,-8.42071136785102,
13.944258352743));
#61996=CARTESIAN_POINT('Ctrl Pts',(6.39615021386663,-8.39409409953866,13.9680027128311));
#61997=CARTESIAN_POINT('Ctrl Pts',(6.0981394504413,-8.52955034249946,13.9841958606635));
#61998=CARTESIAN_POINT('Ctrl Pts',(5.13855911511434,-8.93196846881188,14.0292676298103));
#61999=CARTESIAN_POINT('Ctrl Pts',(3.4042278071613,-9.47086396710915,14.0771763067071));
#62000=CARTESIAN_POINT('Ctrl Pts',(1.16260698888612,-9.8259538455241,14.100750462816));
#62001=CARTESIAN_POINT('Ctrl Pts',(-1.16569733333535,-9.82569779920851,
14.1007357383411));
#62002=CARTESIAN_POINT('Ctrl Pts',(-3.40685010597653,-9.47022124827926,
14.0771275227186));
#62003=CARTESIAN_POINT('Ctrl Pts',(-5.140066644375,-8.93138328509499,14.0292067344484));
#62004=CARTESIAN_POINT('Ctrl Pts',(-6.09875459911923,-8.52927070381225,
13.9841624342243));
#62005=CARTESIAN_POINT('Ctrl Pts',(-6.39614996063647,-8.39409419402682,
13.9680027190745));
#62006=CARTESIAN_POINT('Ctrl Pts',(6.17590518600828,-7.95710732525973,13.4973889894963));
#62007=CARTESIAN_POINT('Ctrl Pts',(5.88795326937256,-8.08714184605563,13.5139089189715));
#62008=CARTESIAN_POINT('Ctrl Pts',(4.96084266091442,-8.47346685614734,13.560052102495));
#62009=CARTESIAN_POINT('Ctrl Pts',(3.28578921021426,-8.99076845677069,13.6098152835045));
#62010=CARTESIAN_POINT('Ctrl Pts',(1.12196199728683,-9.33150995192134,13.6348906738451));
#62011=CARTESIAN_POINT('Ctrl Pts',(-1.12494446487316,-9.33126430248581,
13.6348747843078));
#62012=CARTESIAN_POINT('Ctrl Pts',(-3.28832124960869,-8.99015159077933,
13.6097640000083));
#62013=CARTESIAN_POINT('Ctrl Pts',(-4.96229906404752,-8.47290506114866,
13.5599894946589));
#62014=CARTESIAN_POINT('Ctrl Pts',(-5.88854765313263,-8.0868734027617,13.5138748169163));
#62015=CARTESIAN_POINT('Ctrl Pts',(-6.17590494057391,-7.95710741697555,
13.4973889956498));
#62016=CARTESIAN_POINT('Ctrl Pts',(6.16915737727431,-8.01757364818157,12.8211920463632));
#62017=CARTESIAN_POINT('Ctrl Pts',(5.88220122989312,-8.14587304019011,12.8375467559628));
#62018=CARTESIAN_POINT('Ctrl Pts',(4.95802580678134,-8.52723293522564,12.8832472984301));
#62019=CARTESIAN_POINT('Ctrl Pts',(3.28628703195018,-9.03882920094257,12.9325846801364));
#62020=CARTESIAN_POINT('Ctrl Pts',(1.12279040062947,-9.37660072493885,12.9574622751438));
#62021=CARTESIAN_POINT('Ctrl Pts',(-1.12577452523575,-9.3763569576825,12.9574465121303));
#62022=CARTESIAN_POINT('Ctrl Pts',(-3.28881618122004,-9.03821837019887,
12.9325338080592));
#62023=CARTESIAN_POINT('Ctrl Pts',(-4.95947798566805,-8.52667806159099,
12.8831852649638));
#62024=CARTESIAN_POINT('Ctrl Pts',(-5.88279356364298,-8.14560817488497,
12.8375129981983));
#62025=CARTESIAN_POINT('Ctrl Pts',(-6.16915713521142,-8.01757373702705,
12.8211920538159));
#62026=CARTESIAN_POINT('Ctrl Pts',(6.38081597772446,-8.53150930643574,12.4312991541261));
#62027=CARTESIAN_POINT('Ctrl Pts',(6.08506814081239,-8.66302236326436,12.4471168272863));
#62028=CARTESIAN_POINT('Ctrl Pts',(5.1321581266024,-9.05415696406033,12.491182660567));
#62029=CARTESIAN_POINT('Ctrl Pts',(3.40535948165785,-9.58008675116646,12.5381236733996));
#62030=CARTESIAN_POINT('Ctrl Pts',(1.16448971008638,-9.92842720330246,12.5612483214676));
#62031=CARTESIAN_POINT('Ctrl Pts',(-1.16758382053923,-9.92817543434746,
12.5612338845422));
#62032=CARTESIAN_POINT('Ctrl Pts',(-3.40797521272135,-9.579457747783,12.5380758243915));
#62033=CARTESIAN_POINT('Ctrl Pts',(-5.13365605611323,-9.05358750956378,
12.4911230705099));
#62034=CARTESIAN_POINT('Ctrl Pts',(-6.08567863075684,-8.66275085577762,
12.4470841832806));
#62035=CARTESIAN_POINT('Ctrl Pts',(-6.38081573215519,-8.53150939440301,
12.4312991633297));
#62036=CARTESIAN_POINT('',(-6.2499460327501,-8.55169213656735,12.4626541460308));
#62037=CARTESIAN_POINT('Origin',(-6.52772595968144,-9.09522655590529,13.2547537702088));
#62038=CARTESIAN_POINT('Ctrl Pts',(6.2499456683813,-8.55169360934562,12.4626524817952));
#62039=CARTESIAN_POINT('Ctrl Pts',(5.99497571757143,-8.66276623416142,12.4758503685831));
#62040=CARTESIAN_POINT('Ctrl Pts',(5.73509544265912,-8.76842077642134,12.4877092255716));
#62041=CARTESIAN_POINT('Ctrl Pts',(5.47038343317498,-8.868056192506,12.4983674133053));
#62042=CARTESIAN_POINT('Ctrl Pts',(5.26894837630338,-8.94387468576043,12.5064778600375));
#62043=CARTESIAN_POINT('Ctrl Pts',(5.06471576319851,-9.01620688869194,12.5138932611287));
#62044=CARTESIAN_POINT('Ctrl Pts',(4.85775981274984,-9.08476991994723,12.5206818391115));
#62045=CARTESIAN_POINT('Ctrl Pts',(4.61829824467732,-9.1641018306297,12.528536667761));
#62046=CARTESIAN_POINT('Ctrl Pts',(4.3751803125037,-9.23840063347297,12.5355463889511));
#62047=CARTESIAN_POINT('Ctrl Pts',(4.12852312077457,-9.30727351514831,12.5417718905077));
#62048=CARTESIAN_POINT('Ctrl Pts',(4.00519452491001,-9.34170995598598,12.544884641286));
#62049=CARTESIAN_POINT('Ctrl Pts',(3.88098152000299,-9.37479021607175,12.5478007973506));
#62050=CARTESIAN_POINT('Ctrl Pts',(3.75590130472956,-9.40646721059036,12.5505244941746));
#62051=CARTESIAN_POINT('Ctrl Pts',(3.69336119709285,-9.42230570784966,12.5518863425865));
#62052=CARTESIAN_POINT('Ctrl Pts',(3.63060428550466,-9.4377933813947,12.553200066749));
#62053=CARTESIAN_POINT('Ctrl Pts',(3.56763292198375,-9.45292452381646,12.5544659168596));
#62054=CARTESIAN_POINT('Ctrl Pts',(3.5361472402233,-9.46049009502734,12.5550988419149));
#62055=CARTESIAN_POINT('Ctrl Pts',(3.50460794541682,-9.46796653300947,12.5557197978829));
#62056=CARTESIAN_POINT('Ctrl Pts',(3.47301533729935,-9.47535312881161,12.5563288059489));
#62057=CARTESIAN_POINT('Ctrl Pts',(3.46349483562411,-9.47757909564053,12.556512331864));
#62058=CARTESIAN_POINT('Ctrl Pts',(3.45396949300403,-9.47979690408182,12.5566947722591));
#62059=CARTESIAN_POINT('Ctrl Pts',(3.44443931646769,-9.48200653383592,12.5568761285555));
#62060=CARTESIAN_POINT('Ctrl Pts',(3.43815713652989,-9.48346309570109,12.5569956764864));
#62061=CARTESIAN_POINT('Ctrl Pts',(3.43187285611465,-9.48491610368712,12.5571147533454));
#62062=CARTESIAN_POINT('Ctrl Pts',(3.42558647838356,-9.48636555303398,12.5572333589227));
#62063=CARTESIAN_POINT('Ctrl Pts',(3.40976355599046,-9.49001384232061,12.5575318912294));
#62064=CARTESIAN_POINT('Ctrl Pts',(3.39530296967644,-9.49332685868534,12.5578020467836));
#62065=CARTESIAN_POINT('Ctrl Pts',(3.37807788093079,-9.4972426942353,12.5581200099282));
#62066=CARTESIAN_POINT('Ctrl Pts',(3.0751556918768,-9.56610698250018,12.5637117426157));
#62067=CARTESIAN_POINT('Ctrl Pts',(2.76997585607743,-9.62598687169383,12.5682700097437));
#62068=CARTESIAN_POINT('Ctrl Pts',(2.4629153139001,-9.67662910251466,12.5719614267642));
#62069=CARTESIAN_POINT('Ctrl Pts',(2.16108112038875,-9.72640937317084,12.5755900137242));
#62070=CARTESIAN_POINT('Ctrl Pts',(1.85742917537775,-9.76726384928626,12.5783808667533));
#62071=CARTESIAN_POINT('Ctrl Pts',(1.55231579736879,-9.79890195725704,12.5804891643225));
#62072=CARTESIAN_POINT('Ctrl Pts',(1.4240166092259,-9.81220567928168,12.5813756966281));
#62073=CARTESIAN_POINT('Ctrl Pts',(1.29545903789866,-9.82387916506831,12.5821415155451));
#62074=CARTESIAN_POINT('Ctrl Pts',(1.16666981828216,-9.83389804518222,12.5827980829505));
#62075=CARTESIAN_POINT('Ctrl Pts',(0.860216072588966,-9.85773795466922,
12.5843603840599));
#62076=CARTESIAN_POINT('Ctrl Pts',(0.552449700108069,-9.87221279988117,
12.5853043714385));
#62077=CARTESIAN_POINT('Ctrl Pts',(0.243803444773064,-9.87721198877206,
12.5856295548017));
#62078=CARTESIAN_POINT('Ctrl Pts',(0.162408034707189,-9.87853036222625,
12.585715311336));
#62079=CARTESIAN_POINT('Ctrl Pts',(0.0809515130470044,-9.87918946580259,
12.5857580138753));
#62080=CARTESIAN_POINT('Ctrl Pts',(-0.000557986953597959,-9.87918669603315,
12.5857576143789));
#62081=CARTESIAN_POINT('Ctrl Pts',(-0.299520873003152,-9.87917653699318,
12.5857561490943));
#62082=CARTESIAN_POINT('Ctrl Pts',(-0.597728166319448,-9.87028485226777,
12.5851605051845));
#62083=CARTESIAN_POINT('Ctrl Pts',(-0.894817219028394,-9.85261539770727,
12.5839820704873));
#62084=CARTESIAN_POINT('Ctrl Pts',(-0.986618306464046,-9.84715550233833,
12.5836179319043));
#62085=CARTESIAN_POINT('Ctrl Pts',(-1.07831270681731,-9.84085711977231,
12.583198122586));
#62086=CARTESIAN_POINT('Ctrl Pts',(-1.16988990879901,-9.83372233090494,
12.5827229125624));
#62087=CARTESIAN_POINT('Ctrl Pts',(-1.34879551606369,-9.81978377734141,
12.5817945402602));
#62088=CARTESIAN_POINT('Ctrl Pts',(-1.5272538175031,-9.8026534714518,12.5806547311173));
#62089=CARTESIAN_POINT('Ctrl Pts',(-1.70519969857571,-9.78239209576105,
12.57927485804));
#62090=CARTESIAN_POINT('Ctrl Pts',(-1.9871029518838,-9.7502938662921,12.5770888523437));
#62091=CARTESIAN_POINT('Ctrl Pts',(-2.26770623515151,-9.71031298494122,
12.5743222105347));
#62092=CARTESIAN_POINT('Ctrl Pts',(-2.54672767284504,-9.66267617985082,
12.5708491197125));
#62093=CARTESIAN_POINT('Ctrl Pts',(-2.68623839169181,-9.63885777730561,
12.5691125743015));
#62094=CARTESIAN_POINT('Ctrl Pts',(-2.82535386091671,-9.61312634948936,
12.5671981611192));
#62095=CARTESIAN_POINT('Ctrl Pts',(-2.96404008610357,-9.58551587818721,
12.5650827887556));
#62096=CARTESIAN_POINT('Ctrl Pts',(-3.03338319869701,-9.57171064253614,
12.5640251025738));
#62097=CARTESIAN_POINT('Ctrl Pts',(-3.10261899674013,-9.55743563238489,
12.5629171586651));
#62098=CARTESIAN_POINT('Ctrl Pts',(-3.17174332330947,-9.54269552091794,
12.5617555625508));
#62099=CARTESIAN_POINT('Ctrl Pts',(-3.20630548659414,-9.53532546518447,
12.5611747644936));
#62100=CARTESIAN_POINT('Ctrl Pts',(-3.24083978174743,-9.52783913333813,
12.5605805523299));
#62101=CARTESIAN_POINT('Ctrl Pts',(-3.27534569080372,-9.52023711797875,
12.5599724850652));
#62102=CARTESIAN_POINT('Ctrl Pts',(-3.29259864533187,-9.51643611029907,
12.5596684514329));
#62103=CARTESIAN_POINT('Ctrl Pts',(-3.30984450331694,-9.512606181695,12.5593609539618));
#62104=CARTESIAN_POINT('Ctrl Pts',(-3.32708320031767,-9.50874740771603,
12.5590499357491));
#62105=CARTESIAN_POINT('Ctrl Pts',(-3.3443218973184,-9.50488863373705,12.5587389175364));
#62106=CARTESIAN_POINT('Ctrl Pts',(-3.36293312666133,-9.5006873055441,12.5583988970378));
#62107=CARTESIAN_POINT('Ctrl Pts',(-3.378777743974,-9.49708462554388,12.5581062613217));
#62108=CARTESIAN_POINT('Ctrl Pts',(-3.40160033225428,-9.49189532492979,
12.5576847488084));
#62109=CARTESIAN_POINT('Ctrl Pts',(-3.42439545405496,-9.4866585593598,12.5572574659275));
#62110=CARTESIAN_POINT('Ctrl Pts',(-3.44716295235235,-9.48137461708584,
12.5568243760515));
#62111=CARTESIAN_POINT('Ctrl Pts',(-3.72185578882046,-9.41762316437855,
12.5515990902102));
#62112=CARTESIAN_POINT('Ctrl Pts',(-3.99252581059805,-9.34700823075725,
12.5455274359759));
#62113=CARTESIAN_POINT('Ctrl Pts',(-4.2590050846537,-9.27009997597244,12.5385001292223));
#62114=CARTESIAN_POINT('Ctrl Pts',(-4.53204587047232,-9.19129801136636,
12.5312997892896));
#62115=CARTESIAN_POINT('Ctrl Pts',(-4.80068706808185,-9.10588893380199,
12.5230962144446));
#62116=CARTESIAN_POINT('Ctrl Pts',(-5.06476941248447,-9.01443703992606,
12.5137847237623));
#62117=CARTESIAN_POINT('Ctrl Pts',(-5.20182127086784,-8.9669758889857,12.5089523026279));
#62118=CARTESIAN_POINT('Ctrl Pts',(-5.33764561460797,-8.91788641265564,
12.5038216852713));
#62119=CARTESIAN_POINT('Ctrl Pts',(-5.4722222565736,-8.86724255974421,12.498379474696));
#62120=CARTESIAN_POINT('Ctrl Pts',(-5.73629434307178,-8.76786700904469,
12.4877005345708));
#62121=CARTESIAN_POINT('Ctrl Pts',(-5.99556164303099,-8.66250926796784,
12.4758212277278));
#62122=CARTESIAN_POINT('Ctrl Pts',(-6.24994585737753,-8.55169179341496,
12.4626536459473));
#62123=CARTESIAN_POINT('Ctrl Pts',(-6.23452463023104,-8.46817777445814,
13.9793247860141));
#62124=CARTESIAN_POINT('Ctrl Pts',(-6.26883579448648,-8.45422023761174,
13.9766717378257));
#62125=CARTESIAN_POINT('Ctrl Pts',(-6.38681948165088,-8.4004620524671,13.9705684989092));
#62126=CARTESIAN_POINT('Ctrl Pts',(-6.58037374888043,-8.27697442816996,
13.9789814227231));
#62127=CARTESIAN_POINT('Ctrl Pts',(-6.79245627860415,-8.07356528041172,
14.0233019893044));
#62128=CARTESIAN_POINT('Ctrl Pts',(-6.96282724046887,-7.82819097507957,
14.1005711232815));
#62129=CARTESIAN_POINT('Ctrl Pts',(-7.07881819325669,-7.55335221044515,
14.2073541386468));
#62130=CARTESIAN_POINT('Ctrl Pts',(-7.11903847741079,-7.3320169206708,14.3074069407329));
#62131=CARTESIAN_POINT('Ctrl Pts',(-7.1223300547874,-7.20833635409889,14.3683840363599));
#62132=CARTESIAN_POINT('Ctrl Pts',(-7.12201750162379,-7.17914631343674,
14.3830673400188));
#62133=CARTESIAN_POINT('Ctrl Pts',(-6.02296491909003,-8.0229515174066,13.5080161017831));
#62134=CARTESIAN_POINT('Ctrl Pts',(-6.05240779820068,-8.01109502665855,
13.5055635345619));
#62135=CARTESIAN_POINT('Ctrl Pts',(-6.15384509230703,-7.96537876837031,
13.4996013967755));
#62136=CARTESIAN_POINT('Ctrl Pts',(-6.32132139184434,-7.85990580767669,
13.5050734421016));
#62137=CARTESIAN_POINT('Ctrl Pts',(-6.5061768145196,-7.68510794243105,13.5407886398096));
#62138=CARTESIAN_POINT('Ctrl Pts',(-6.65550942751407,-7.4733210730188,13.6052594269033));
#62139=CARTESIAN_POINT('Ctrl Pts',(-6.75751726625292,-7.23561030969866,
13.6959374225502));
#62140=CARTESIAN_POINT('Ctrl Pts',(-6.79287018228396,-7.04443217880955,
13.7817350544861));
#62141=CARTESIAN_POINT('Ctrl Pts',(-6.79574426882679,-6.93808341830671,
13.8341161676123));
#62142=CARTESIAN_POINT('Ctrl Pts',(-6.79546946623675,-6.91302049420525,
13.8467286811972));
#62143=CARTESIAN_POINT('Ctrl Pts',(-6.00126870307733,-8.08913998801194,
12.8295907586597));
#62144=CARTESIAN_POINT('Ctrl Pts',(-6.04284582198358,-8.07265129772834,
12.8262979975003));
#62145=CARTESIAN_POINT('Ctrl Pts',(-6.18536698153368,-8.009419057336,12.8186086282347));
#62146=CARTESIAN_POINT('Ctrl Pts',(-6.41671326094832,-7.86606558233941,
12.8278122909668));
#62147=CARTESIAN_POINT('Ctrl Pts',(-6.66709581952829,-7.63353122744836,
12.8781674889523));
#62148=CARTESIAN_POINT('Ctrl Pts',(-6.86630942062206,-7.35614457211733,
12.9654853766482));
#62149=CARTESIAN_POINT('Ctrl Pts',(-7.00115184090513,-7.04757262155766,
13.085461092087));
#62150=CARTESIAN_POINT('Ctrl Pts',(-7.04795204044777,-6.79933349998106,
13.1977178770678));
#62151=CARTESIAN_POINT('Ctrl Pts',(-7.05182631606654,-6.65991344971732,
13.2664548440122));
#62152=CARTESIAN_POINT('Ctrl Pts',(-7.05146280075313,-6.62694954794606,
13.283035607156));
#62153=CARTESIAN_POINT('Ctrl Pts',(-6.18531856502411,-8.6182879511144,12.440699239874));
#62154=CARTESIAN_POINT('Ctrl Pts',(-6.24714938480481,-8.59382489176563,
12.4361406869405));
#62155=CARTESIAN_POINT('Ctrl Pts',(-6.45830856891384,-8.50034161670644,
12.4261201997568));
#62156=CARTESIAN_POINT('Ctrl Pts',(-6.79671573688593,-8.29094349054743,
12.442996182583));
#62157=CARTESIAN_POINT('Ctrl Pts',(-7.15740948686567,-7.95659180419277,
12.5205192982545));
#62158=CARTESIAN_POINT('Ctrl Pts',(-7.44090723754234,-7.56244152691377,
12.6496041416091));
#62159=CARTESIAN_POINT('Ctrl Pts',(-7.63136485385938,-7.12689428226258,
12.8228324436505));
#62160=CARTESIAN_POINT('Ctrl Pts',(-7.6975468214002,-6.77614844491688,12.9828928517768));
#62161=CARTESIAN_POINT('Ctrl Pts',(-7.70310676159879,-6.5774643832572,13.080963940675));
#62162=CARTESIAN_POINT('Ctrl Pts',(-7.70259301383401,-6.53035544843766,
13.1046469715588));
#62163=CARTESIAN_POINT('',(-7.000004044956,-6.97711954662123,13.9487143140163));
#62164=CARTESIAN_POINT('',(-7.,-8.04450891402614,12.5220421917952));
#62165=CARTESIAN_POINT('Ctrl Pts',(-7.,-6.97711954662123,13.9487143140163));
#62166=CARTESIAN_POINT('Ctrl Pts',(-7.,-7.02109862854982,13.8470307249955));
#62167=CARTESIAN_POINT('Ctrl Pts',(-7.,-7.06256666149218,13.7566966111574));
#62168=CARTESIAN_POINT('Ctrl Pts',(-7.,-7.10064521379527,13.6790951563344));
#62169=CARTESIAN_POINT('Ctrl Pts',(-7.,-7.11968448994682,13.6402944289229));
#62170=CARTESIAN_POINT('Ctrl Pts',(-7.,-7.13783856938113,13.6046507331564));
#62171=CARTESIAN_POINT('Ctrl Pts',(-7.,-7.1548263061793,13.5722133313273));
#62172=CARTESIAN_POINT('Ctrl Pts',(-7.,-7.16332017457839,13.5559946304127));
#62173=CARTESIAN_POINT('Ctrl Pts',(-7.,-7.17152128706493,13.540576415578));
#62174=CARTESIAN_POINT('Ctrl Pts',(-7.,-7.17939021066077,13.5259591637652));
#62175=CARTESIAN_POINT('Ctrl Pts',(-7.,-7.18332467245869,13.5186505378588));
#62176=CARTESIAN_POINT('Ctrl Pts',(-7.,-7.18717608703393,13.5115421527079));
#62177=CARTESIAN_POINT('Ctrl Pts',(-7.,-7.19093943869574,13.5046337282638));
#62178=CARTESIAN_POINT('Ctrl Pts',(-7.,-7.19282111452665,13.5011795160418));
#62179=CARTESIAN_POINT('Ctrl Pts',(-7.,-7.19468077462919,13.4977752939964));
#62180=CARTESIAN_POINT('Ctrl Pts',(-7.,-7.19651779951958,13.4944210212393));
#62181=CARTESIAN_POINT('Ctrl Pts',(-7.,-7.19835482440998,13.4910667484821));
#62182=CARTESIAN_POINT('Ctrl Pts',(-7.,-7.19936191322088,13.4892292594739));
#62183=CARTESIAN_POINT('Ctrl Pts',(-7.,-7.20196035000388,13.4845080053656));
#62184=CARTESIAN_POINT('Ctrl Pts',(-7.,-7.24353533853188,13.4089679396339));
#62185=CARTESIAN_POINT('Ctrl Pts',(-7.,-7.2857875477303,13.3377228575316));
#62186=CARTESIAN_POINT('Ctrl Pts',(-7.,-7.32834490361038,13.2712597190853));
#62187=CARTESIAN_POINT('Ctrl Pts',(-7.,-7.37090225949045,13.204796580639));
#62188=CARTESIAN_POINT('Ctrl Pts',(-7.,-7.41277352570555,13.1444220728118));
#62189=CARTESIAN_POINT('Ctrl Pts',(-7.,-7.45595082571483,13.0864229416019));
#62190=CARTESIAN_POINT('Ctrl Pts',(-7.,-7.54230542573338,12.970424679182));
#62191=CARTESIAN_POINT('Ctrl Pts',(-7.,-7.63588413976072,12.862461076247));
#62192=CARTESIAN_POINT('Ctrl Pts',(-7.,-7.73525747692535,12.7671752392972));
#62193=CARTESIAN_POINT('Ctrl Pts',(-7.,-7.83463081408998,12.6718894023474));
#62194=CARTESIAN_POINT('Ctrl Pts',(-7.,-7.93960130471208,12.589438500359));
#62195=CARTESIAN_POINT('Ctrl Pts',(-7.,-8.04450891402614,12.5220421917952));
#62196=CARTESIAN_POINT('Ctrl Pts',(-6.24994618627715,-8.55169243697437,
12.4626545838199));
#62197=CARTESIAN_POINT('Ctrl Pts',(-6.33574809474198,-8.51432360343295,
12.4582072698156));
#62198=CARTESIAN_POINT('Ctrl Pts',(-6.41863145615134,-8.47241225434573,
12.4571381176112));
#62199=CARTESIAN_POINT('Ctrl Pts',(-6.49887786889414,-8.42605295672793,
12.4592634833518));
#62200=CARTESIAN_POINT('Ctrl Pts',(-6.50612048271016,-8.42186881343789,
12.4594553075437));
#62201=CARTESIAN_POINT('Ctrl Pts',(-6.5133416130754,-8.41764841768038,12.4596731254631));
#62202=CARTESIAN_POINT('Ctrl Pts',(-6.5205414651617,-8.41339182738887,12.4599167852897));
#62203=CARTESIAN_POINT('Ctrl Pts',(-6.60751394034807,-8.3619732441917,12.4628601371768));
#62204=CARTESIAN_POINT('Ctrl Pts',(-6.69138037805353,-8.30527348498648,
12.4695747574696));
#62205=CARTESIAN_POINT('Ctrl Pts',(-6.77140175261942,-8.24377163592341,
12.4799351200026));
#62206=CARTESIAN_POINT('Ctrl Pts',(-6.84299358299183,-8.18874846280749,
12.4892041099578));
#62207=CARTESIAN_POINT('Ctrl Pts',(-6.91150928010844,-8.12988371948789,
12.5013942350656));
#62208=CARTESIAN_POINT('Ctrl Pts',(-6.97699397705138,-8.06692162074103,
12.5165626773547));
#62209=CARTESIAN_POINT('Ctrl Pts',(-6.98470443987939,-8.05950817997358,
12.5183486779913));
#62210=CARTESIAN_POINT('Ctrl Pts',(-6.99237288001724,-8.05203790662405,
12.5201759166414));
#62211=CARTESIAN_POINT('Ctrl Pts',(-6.99999936979046,-8.04451036076635,
12.5220444437838));
#62212=CARTESIAN_POINT('Ctrl Pts',(-6.26385884533749,-8.42070687883871,
13.9442629411756));
#62213=CARTESIAN_POINT('Ctrl Pts',(-6.28164430916676,-8.40909725695394,
13.9397078360192));
#62214=CARTESIAN_POINT('Ctrl Pts',(-6.2993722741453,-8.39692701207701,13.9353443706832));
#62215=CARTESIAN_POINT('Ctrl Pts',(-6.31700919643268,-8.38419168734846,
13.9311816754727));
#62216=CARTESIAN_POINT('Ctrl Pts',(-6.35928365267996,-8.35366601403318,
13.9212039892483));
#62217=CARTESIAN_POINT('Ctrl Pts',(-6.40103811124441,-8.31989232938067,
13.9123793956503));
#62218=CARTESIAN_POINT('Ctrl Pts',(-6.44183020701902,-8.28290854509716,
13.9047743211951));
#62219=CARTESIAN_POINT('Ctrl Pts',(-6.47172512654695,-8.25580458698962,
13.8992008618146));
#62220=CARTESIAN_POINT('Ctrl Pts',(-6.5011023245919,-8.22697699908308,13.8942824354648));
#62221=CARTESIAN_POINT('Ctrl Pts',(-6.52977104801251,-8.19644600892697,
13.8900489259368));
#62222=CARTESIAN_POINT('Ctrl Pts',(-6.53701932860586,-8.1887268935622,13.8889785725589));
#62223=CARTESIAN_POINT('Ctrl Pts',(-6.54422224509448,-8.18089890918468,
13.8879520232168));
#62224=CARTESIAN_POINT('Ctrl Pts',(-6.55137703981767,-8.17296294031462,
13.8869693750377));
#62225=CARTESIAN_POINT('Ctrl Pts',(-6.58908889829235,-8.1311336291371,13.8817899826867));
#62226=CARTESIAN_POINT('Ctrl Pts',(-6.62546758482145,-8.08630270607222,
13.877829455221));
#62227=CARTESIAN_POINT('Ctrl Pts',(-6.66008338922819,-8.03861158643723,
13.8751074498926));
#62228=CARTESIAN_POINT('Ctrl Pts',(-6.66685492532913,-8.02928226002585,
13.8745749718045));
#62229=CARTESIAN_POINT('Ctrl Pts',(-6.67355885667037,-8.01984353880004,
13.8740899238172));
#62230=CARTESIAN_POINT('Ctrl Pts',(-6.68019174663662,-8.01029656021264,
13.8736525109273));
#62231=CARTESIAN_POINT('Ctrl Pts',(-6.69130314370655,-7.99430349075988,
13.8729197581863));
#62232=CARTESIAN_POINT('Ctrl Pts',(-6.70221521440315,-7.97800661125738,
13.8723206718115));
#62233=CARTESIAN_POINT('Ctrl Pts',(-6.71291129475068,-7.96141141158149,
13.8718563685801));
#62234=CARTESIAN_POINT('Ctrl Pts',(-6.72172754331972,-7.94773281151101,
13.8714736664531));
#62235=CARTESIAN_POINT('Ctrl Pts',(-6.73039703334244,-7.93385153469644,
13.8711825417838));
#62236=CARTESIAN_POINT('Ctrl Pts',(-6.73891198148699,-7.91977220431998,
13.8709824492016));
#62237=CARTESIAN_POINT('Ctrl Pts',(-6.74833472334838,-7.90419185157249,
13.8707610243946));
#62238=CARTESIAN_POINT('Ctrl Pts',(-6.75756822273766,-7.88836896209251,
13.8706510740985));
#62239=CARTESIAN_POINT('Ctrl Pts',(-6.76660156287043,-7.87230998751464,
13.8706519436779));
#62240=CARTESIAN_POINT('Ctrl Pts',(-6.77111823293682,-7.8642805002257,13.8706523784676));
#62241=CARTESIAN_POINT('Ctrl Pts',(-6.77558485989446,-7.8561919898451,13.8706805202337));
#62242=CARTESIAN_POINT('Ctrl Pts',(-6.78000003558841,-7.84804528745407,
13.8707362961633));
#62243=CARTESIAN_POINT('Ctrl Pts',(-6.78270660742908,-7.84305123131353,
13.8707704876817));
#62244=CARTESIAN_POINT('Ctrl Pts',(-6.78573601458584,-7.83739413688215,
13.8708206650807));
#62245=CARTESIAN_POINT('Ctrl Pts',(-6.78845606288443,-7.83225166154178,
13.8708779062954));
#62246=CARTESIAN_POINT('Ctrl Pts',(-6.79017317415198,-7.82900532126369,
13.8709140415121));
#62247=CARTESIAN_POINT('Ctrl Pts',(-6.79176802387397,-7.8259647425448,13.870952434692));
#62248=CARTESIAN_POINT('Ctrl Pts',(-6.7930897838889,-7.82343142964423,13.8709864626005));
#62249=CARTESIAN_POINT('Ctrl Pts',(-6.81076623182257,-7.78955237967999,
13.8714415320118));
#62250=CARTESIAN_POINT('Ctrl Pts',(-6.82804731998309,-7.75374239582446,
13.8723500658969));
#62251=CARTESIAN_POINT('Ctrl Pts',(-6.84464290043939,-7.71596402803055,
13.8737975583038));
#62252=CARTESIAN_POINT('Ctrl Pts',(-6.84884551603565,-7.70639714616643,
13.8741641169897));
#62253=CARTESIAN_POINT('Ctrl Pts',(-6.85300394537083,-7.69670415794422,
13.8745652494736));
#62254=CARTESIAN_POINT('Ctrl Pts',(-6.85711299825419,-7.68688471531696,
13.8750023702786));
#62255=CARTESIAN_POINT('Ctrl Pts',(-6.87261613350537,-7.64983672604478,
13.8766515928983));
#62256=CARTESIAN_POINT('Ctrl Pts',(-6.88741903444732,-7.6109861396205,13.8788133699042));
#62257=CARTESIAN_POINT('Ctrl Pts',(-6.90125024927014,-7.57035421419371,
13.8815453788709));
#62258=CARTESIAN_POINT('Ctrl Pts',(-6.91403168206642,-7.53280623081852,
13.8840700297749));
#62259=CARTESIAN_POINT('Ctrl Pts',(-6.92598337927363,-7.49373721201718,
13.8870815422083));
#62260=CARTESIAN_POINT('Ctrl Pts',(-6.93686114758191,-7.45318980081384,
13.8906237642641));
#62261=CARTESIAN_POINT('Ctrl Pts',(-6.94303774585016,-7.43016622991928,
13.8926351035384));
#62262=CARTESIAN_POINT('Ctrl Pts',(-6.94886754432856,-7.40666644740578,
13.8948175490587));
#62263=CARTESIAN_POINT('Ctrl Pts',(-6.95430081976807,-7.38270217973598,
13.8971790243926));
#62264=CARTESIAN_POINT('Ctrl Pts',(-6.96395630575806,-7.34011522582167,
13.9013756075138));
#62265=CARTESIAN_POINT('Ctrl Pts',(-6.9723612927587,-7.29605906095144,13.9061378933399));
#62266=CARTESIAN_POINT('Ctrl Pts',(-6.97925043175555,-7.25064769251095,
13.9114910616584));
#62267=CARTESIAN_POINT('Ctrl Pts',(-6.98579308269724,-7.20752028099744,
13.9165749933015));
#62268=CARTESIAN_POINT('Ctrl Pts',(-6.99096887006084,-7.16317064731089,
13.9221917460347));
#62269=CARTESIAN_POINT('Ctrl Pts',(-6.99451703428925,-7.11772928270794,
13.9283605810957));
#62270=CARTESIAN_POINT('Ctrl Pts',(-6.99591396140104,-7.09983882721493,
13.9307892772863));
#62271=CARTESIAN_POINT('Ctrl Pts',(-6.99705819555185,-7.08177951502153,
13.9333035312008));
#62272=CARTESIAN_POINT('Ctrl Pts',(-6.9979320935569,-7.06356077431209,13.9359044736482));
#62273=CARTESIAN_POINT('Ctrl Pts',(-6.99929644409143,-7.03511723916062,
13.9399651274063));
#62274=CARTESIAN_POINT('Ctrl Pts',(-7.00000204474255,-7.00628463245252,
13.9442371933808));
#62275=CARTESIAN_POINT('Ctrl Pts',(-6.99999554931096,-6.9771195483688,13.9487143130749));
#62276=CARTESIAN_POINT('Ctrl Pts',(-6.2341316903218,-11.8700315082968,24.3933909558656));
#62277=CARTESIAN_POINT('Ctrl Pts',(-6.23490699037994,-11.9504773632788,
23.8924703016508));
#62278=CARTESIAN_POINT('Ctrl Pts',(-6.23649478643264,-12.0627644821299,
22.7260267664735));
#62279=CARTESIAN_POINT('Ctrl Pts',(-6.23804164013149,-11.9701367284916,
20.8893389425408));
#62280=CARTESIAN_POINT('Ctrl Pts',(-6.23759444471014,-11.5416371344917,
18.9411595572409));
#62281=CARTESIAN_POINT('Ctrl Pts',(-6.23570527570309,-10.7961451800346,
17.0892602672504));
#62282=CARTESIAN_POINT('Ctrl Pts',(-6.23205146828093,-9.75631874546476,
15.3875905681178));
#62283=CARTESIAN_POINT('Ctrl Pts',(-6.22726292200935,-8.61699832153917,
14.0755233161913));
#62284=CARTESIAN_POINT('Ctrl Pts',(-6.22400337583775,-7.81350279629324,
13.3673858160704));
#62285=CARTESIAN_POINT('Ctrl Pts',(-6.2226678388619,-7.49367893859873,13.1134099685414));
#62286=CARTESIAN_POINT('Ctrl Pts',(-6.72599077992547,-11.7530848388885,
24.374565981612));
#62287=CARTESIAN_POINT('Ctrl Pts',(-6.72668393615475,-11.832344276316,23.8785345357962));
#62288=CARTESIAN_POINT('Ctrl Pts',(-6.72805219773479,-11.9427130855079,
22.723533396798));
#62289=CARTESIAN_POINT('Ctrl Pts',(-6.7294197444849,-11.8502304322583,20.9054813875764));
#62290=CARTESIAN_POINT('Ctrl Pts',(-6.72902474491262,-11.4262585077992,
18.976797872896));
#62291=CARTESIAN_POINT('Ctrl Pts',(-6.72736869125189,-10.6891570039499,
17.1431712553454));
#62292=CARTESIAN_POINT('Ctrl Pts',(-6.72416503158331,-9.66125809165063,
15.457401490674));
#62293=CARTESIAN_POINT('Ctrl Pts',(-6.71993417357258,-8.53486250336011,
14.1564714981381));
#62294=CARTESIAN_POINT('Ctrl Pts',(-6.717079659789,-7.74007006277861,13.4537931851715));
#62295=CARTESIAN_POINT('Ctrl Pts',(-6.71589093229416,-7.42368913606096,
13.2016833831309));
#62296=CARTESIAN_POINT('Ctrl Pts',(-7.02718513800354,-11.3520754412046,
24.3100156203626));
#62297=CARTESIAN_POINT('Ctrl Pts',(-7.02756383162633,-11.4283591366048,
23.830925349047));
#62298=CARTESIAN_POINT('Ctrl Pts',(-7.02824874199597,-11.5344313266266,
22.7152029731697));
#62299=CARTESIAN_POINT('Ctrl Pts',(-7.02897706253925,-11.4446314644105,
20.9601359261015));
#62300=CARTESIAN_POINT('Ctrl Pts',(-7.02876713792981,-11.035338635164,19.0974438705216));
#62301=CARTESIAN_POINT('Ctrl Pts',(-7.02790260273523,-10.3242142898863,
17.3268280635606));
#62302=CARTESIAN_POINT('Ctrl Pts',(-7.02622925523404,-9.33267502688829,
15.6982407576233));
#62303=CARTESIAN_POINT('Ctrl Pts',(-7.02397923349865,-8.2459987393316,14.440709165306));
#62304=CARTESIAN_POINT('Ctrl Pts',(-7.02249255579137,-7.47887749031547,
13.7610287608176));
#62305=CARTESIAN_POINT('Ctrl Pts',(-7.02184959359837,-7.1735607452346,13.5171523616262));
#62306=CARTESIAN_POINT('Ctrl Pts',(-6.9983806301446,-10.8539092122116,24.2298260574574));
#62307=CARTESIAN_POINT('Ctrl Pts',(-6.99835913464222,-10.9268139731601,
23.7718327055695));
#62308=CARTESIAN_POINT('Ctrl Pts',(-6.99821532667477,-11.0282121120616,
22.7049180447452));
#62309=CARTESIAN_POINT('Ctrl Pts',(-6.99814245624674,-10.9423806584636,
21.0278292308067));
#62310=CARTESIAN_POINT('Ctrl Pts',(-6.99816421977348,-10.5510772324376,
19.2468670090286));
#62311=CARTESIAN_POINT('Ctrl Pts',(-6.99828069438708,-9.87141121253356,
17.5546312641458));
#62312=CARTESIAN_POINT('Ctrl Pts',(-6.99850457248202,-8.92372034671503,
15.9978548351403));
#62313=CARTESIAN_POINT('Ctrl Pts',(-6.99873523799494,-7.88504859624807,
14.795751341076));
#62314=CARTESIAN_POINT('Ctrl Pts',(-6.99894168320714,-7.15167106408799,
14.1458852642028));
#62315=CARTESIAN_POINT('Ctrl Pts',(-6.99898903509106,-6.85988342429147,
13.9127707408451));
#62316=CARTESIAN_POINT('',(-7.00000308919771,-10.9277695878957,24.1259430625668));
#62317=CARTESIAN_POINT('Origin',(-5.99998370364536,-10.9277595200191,24.1259473098659));
#62318=CARTESIAN_POINT('Ctrl Pts',(-7.00001101651408,-10.9277661740993,
24.1259401090719));
#62319=CARTESIAN_POINT('Ctrl Pts',(-7.00001786889488,-10.9560762031794,
23.9375964225754));
#62320=CARTESIAN_POINT('Ctrl Pts',(-7.0000180252376,-10.9791075349139,23.751169245318));
#62321=CARTESIAN_POINT('Ctrl Pts',(-7.0000155683987,-10.9972399153364,23.5670036403763));
#62322=CARTESIAN_POINT('Ctrl Pts',(-7.00001306417673,-11.0157220002865,
23.3792861826514));
#62323=CARTESIAN_POINT('Ctrl Pts',(-7.00000784356584,-11.0291144018999,
23.1939182824481));
#62324=CARTESIAN_POINT('Ctrl Pts',(-7.00000354838541,-11.0378129296526,
23.011211620191));
#62325=CARTESIAN_POINT('Ctrl Pts',(-7.00000225630628,-11.04042962677,22.9562496760505));
#62326=CARTESIAN_POINT('Ctrl Pts',(-7.00000104345542,-11.0426215149221,
22.9015281983146));
#62327=CARTESIAN_POINT('Ctrl Pts',(-6.99999999753982,-11.0443992483831,
22.8470547661776));
#62328=CARTESIAN_POINT('Ctrl Pts',(-6.99999887666316,-11.046304392478,22.7886772085523));
#62329=CARTESIAN_POINT('Ctrl Pts',(-6.99999794690482,-11.0477338974152,
22.7305845211254));
#62330=CARTESIAN_POINT('Ctrl Pts',(-6.99999718086736,-11.0487021770247,
22.6727837229349));
#62331=CARTESIAN_POINT('Ctrl Pts',(-6.99999462214162,-11.0519364339199,
22.4797169390654));
#62332=CARTESIAN_POINT('Ctrl Pts',(-6.99999387750136,-11.0500263261682,
22.2899104602776));
#62333=CARTESIAN_POINT('Ctrl Pts',(-6.99999403434629,-11.043495911084,22.1035935549034));
#62334=CARTESIAN_POINT('Ctrl Pts',(-6.99999406716594,-11.0421294278094,
22.0646069159697));
#62335=CARTESIAN_POINT('Ctrl Pts',(-6.99999414003137,-11.0405605734448,
22.0257729004208));
#62336=CARTESIAN_POINT('Ctrl Pts',(-6.99999424548543,-11.0387940382169,
21.9870933459717));
#62337=CARTESIAN_POINT('Ctrl Pts',(-6.99999432422075,-11.0374750876385,
21.9582139780964));
#62338=CARTESIAN_POINT('Ctrl Pts',(-6.99999441862992,-11.0360814573681,
21.9301066666266));
#62339=CARTESIAN_POINT('Ctrl Pts',(-6.99999453138847,-11.0345337323243,
21.9011846437886));
#62340=CARTESIAN_POINT('Ctrl Pts',(-6.99999463682025,-11.0330865746049,
21.8741419020701));
#62341=CARTESIAN_POINT('Ctrl Pts',(-6.9999947584713,-11.0315045785116,21.8463868423182));
#62342=CARTESIAN_POINT('Ctrl Pts',(-6.99999490350797,-11.0296819417538,
21.8166248372066));
#62343=CARTESIAN_POINT('Ctrl Pts',(-6.99999520366033,-11.025910007751,21.755032576106));
#62344=CARTESIAN_POINT('Ctrl Pts',(-6.99999556265624,-11.0216269204843,
21.6935869074157));
#62345=CARTESIAN_POINT('Ctrl Pts',(-6.99999595370107,-11.0168388725623,
21.632295583509));
#62346=CARTESIAN_POINT('Ctrl Pts',(-6.99999673579073,-11.0072627767184,
21.5097129356955));
#62347=CARTESIAN_POINT('Ctrl Pts',(-6.99999764537197,-10.9956668382537,
21.3877476670165));
#62348=CARTESIAN_POINT('Ctrl Pts',(-6.99999847632105,-10.9821001926362,
21.2664591708761));
#62349=CARTESIAN_POINT('Ctrl Pts',(-6.99999902465854,-10.9731476580993,
21.1864217407523));
#62350=CARTESIAN_POINT('Ctrl Pts',(-6.99999953897964,-10.9633369529758,
21.1066789596586));
#62351=CARTESIAN_POINT('Ctrl Pts',(-6.99999996276679,-10.9526820926811,
21.0272472280891));
#62352=CARTESIAN_POINT('Ctrl Pts',(-7.00000126736906,-10.919881771297,20.7827216077141));
#62353=CARTESIAN_POINT('Ctrl Pts',(-7.00000171385151,-10.8790827758835,
20.5411475182533));
#62354=CARTESIAN_POINT('Ctrl Pts',(-7.00000170643222,-10.8307712017266,
20.303018538099));
#62355=CARTESIAN_POINT('Ctrl Pts',(-7.0000016989336,-10.7819430682013,20.0623434236541));
#62356=CARTESIAN_POINT('Ctrl Pts',(-7.00000122940885,-10.7254408509918,
19.8251874411523));
#62357=CARTESIAN_POINT('Ctrl Pts',(-7.00000072342005,-10.6617508826813,
19.5920091224918));
#62358=CARTESIAN_POINT('Ctrl Pts',(-7.00000046988404,-10.6298377246556,
19.4751703686194));
#62359=CARTESIAN_POINT('Ctrl Pts',(-7.00000020716509,-10.596119684273,19.3593295013968));
#62360=CARTESIAN_POINT('Ctrl Pts',(-6.99999998766534,-10.5606564961048,
19.2445395219721));
#62361=CARTESIAN_POINT('Ctrl Pts',(-6.9999999392903,-10.5528408476764,19.2192412290483));
#62362=CARTESIAN_POINT('Ctrl Pts',(-6.99999989300842,-10.5449404325926,
19.1939939665953));
#62363=CARTESIAN_POINT('Ctrl Pts',(-6.9999998487871,-10.5369560034589,19.168798203842));
#62364=CARTESIAN_POINT('Ctrl Pts',(-6.99999965374745,-10.5017404042032,
19.0576714258086));
#62365=CARTESIAN_POINT('Ctrl Pts',(-6.99999949863786,-10.4648906001592,
18.9475466497737));
#62366=CARTESIAN_POINT('Ctrl Pts',(-6.99999938184555,-10.4264703353217,
18.8384626494681));
#62367=CARTESIAN_POINT('Ctrl Pts',(-6.99999932344939,-10.4072602029029,
18.7839206493154));
#62368=CARTESIAN_POINT('Ctrl Pts',(-6.99999927466386,-10.3876574552857,
18.7296388430949));
#62369=CARTESIAN_POINT('Ctrl Pts',(-6.99999923547135,-10.3676699120197,
18.6756218120257));
#62370=CARTESIAN_POINT('Ctrl Pts',(-6.9999992158751,-10.3576761403867,18.6486132964911));
#62371=CARTESIAN_POINT('Ctrl Pts',(-6.99999919867912,-10.3475861698415,
18.6216709747444));
#62372=CARTESIAN_POINT('Ctrl Pts',(-6.99999918389318,-10.3374009734139,
18.5947954116279));
#62373=CARTESIAN_POINT('Ctrl Pts',(-6.99999917282785,-10.329778691202,18.5746825813911));
#62374=CARTESIAN_POINT('Ctrl Pts',(-6.99999916268459,-10.321739978571,18.5536617628498));
#62375=CARTESIAN_POINT('Ctrl Pts',(-6.99999915445592,-10.31409939832,18.5338560637672));
#62376=CARTESIAN_POINT('Ctrl Pts',(-6.99999915168912,-10.3115303315763,
18.5271966005881));
#62377=CARTESIAN_POINT('Ctrl Pts',(-6.99999914912874,-10.3090066973727,
18.5206743536049));
#62378=CARTESIAN_POINT('Ctrl Pts',(-6.9999991467833,-10.3065606770019,18.5143695585423));
#62379=CARTESIAN_POINT('Ctrl Pts',(-6.99999907528818,-10.231999700937,18.3221832303493));
#62380=CARTESIAN_POINT('Ctrl Pts',(-6.99999912491176,-10.1510711355307,
18.1296181412436));
#62381=CARTESIAN_POINT('Ctrl Pts',(-6.99999933315459,-10.0634926000564,
17.9371553317586));
#62382=CARTESIAN_POINT('Ctrl Pts',(-6.99999947285314,-10.0047410237252,
17.8080427200765));
#62383=CARTESIAN_POINT('Ctrl Pts',(-6.99999968442971,-9.94299694259285,
17.6789771457935));
#62384=CARTESIAN_POINT('Ctrl Pts',(-6.99999998816768,-9.87817779118915,
17.5501167562952));
#62385=CARTESIAN_POINT('Ctrl Pts',(-7.00000042904169,-9.78409314535192,
17.3630766015592));
#62386=CARTESIAN_POINT('Ctrl Pts',(-7.00000106782039,-9.68352889475653,
17.1764665511887));
#62387=CARTESIAN_POINT('Ctrl Pts',(-7.00000153333001,-9.57627847396805,
16.9908083130017));
#62388=CARTESIAN_POINT('Ctrl Pts',(-7.00000199137045,-9.47074890330964,
16.8081289908971));
#62389=CARTESIAN_POINT('Ctrl Pts',(-7.00000228134333,-9.35874595195695,
16.6263711514362));
#62390=CARTESIAN_POINT('Ctrl Pts',(-7.00000202664151,-9.24008883380642,
16.446079218847));
#62391=CARTESIAN_POINT('Ctrl Pts',(-7.00000181210071,-9.1401414001778,16.2942154600847));
#62392=CARTESIAN_POINT('Ctrl Pts',(-7.00000121063313,-9.03547304290156,
16.1433925290633));
#62393=CARTESIAN_POINT('Ctrl Pts',(-6.99999998662452,-8.92598518393872,
15.9939629313457));
#62394=CARTESIAN_POINT('Ctrl Pts',(-6.99999852879618,-8.79558209416524,
15.8159881181512));
#62395=CARTESIAN_POINT('Ctrl Pts',(-6.9999961728163,-8.6583410520032,15.6399892306821));
#62396=CARTESIAN_POINT('Ctrl Pts',(-6.9999944983877,-8.51418146148609,15.4665322542966));
#62397=CARTESIAN_POINT('Ctrl Pts',(-6.99999284818175,-8.37210731493886,
15.2955845442328));
#62398=CARTESIAN_POINT('Ctrl Pts',(-6.99999186149943,-8.22331328898852,
15.1271057140513));
#62399=CARTESIAN_POINT('Ctrl Pts',(-6.99999320063754,-8.0677498898833,14.9616796343078));
#62400=CARTESIAN_POINT('Ctrl Pts',(-6.99999413393874,-7.9593312685555,14.8463872994744));
#62401=CARTESIAN_POINT('Ctrl Pts',(-6.99999620011487,-7.84762514473388,
14.7325786384935));
#62402=CARTESIAN_POINT('Ctrl Pts',(-6.99999999965493,-7.73262311891675,
14.6204637825058));
#62403=CARTESIAN_POINT('Ctrl Pts',(-7.00000506889666,-7.57919058243494,
14.4708832285177));
#62404=CARTESIAN_POINT('Ctrl Pts',(-7.00001329865542,-7.4198895840185,14.3243159680113));
#62405=CARTESIAN_POINT('Ctrl Pts',(-7.00001657747118,-7.25480415599887,
14.1813331106406));
#62406=CARTESIAN_POINT('Ctrl Pts',(-7.00001838123028,-7.16398650538121,
14.1026746406546));
#62407=CARTESIAN_POINT('Ctrl Pts',(-7.00001867170311,-7.07141884697089,
14.0251016321159));
#62408=CARTESIAN_POINT('Ctrl Pts',(-7.00001598754464,-6.97711954671267,
13.9487143134838));
#62409=CARTESIAN_POINT('Origin',(-5.9999949808,-10.9277770011797,24.1259380084106));
#62410=CARTESIAN_POINT('Origin',(-6.,-10.9277790621883,24.1259427055448));
#62411=CARTESIAN_POINT('Ctrl Pts',(-7.10692994354395,-5.08477020587198,
15.2195232722513));
#62412=CARTESIAN_POINT('Ctrl Pts',(-7.10723905417148,-5.05413024983052,
15.2296541384606));
#62413=CARTESIAN_POINT('Ctrl Pts',(-7.10399806473613,-4.92454784617344,
15.2736511084783));
#62414=CARTESIAN_POINT('Ctrl Pts',(-7.06411031942477,-4.69882499679942,
15.3588366457335));
#62415=CARTESIAN_POINT('Ctrl Pts',(-6.94880758813024,-4.43055877160903,
15.4770235844201));
#62416=CARTESIAN_POINT('Ctrl Pts',(-6.77939710086492,-4.20377723167178,
15.5952641304998));
#62417=CARTESIAN_POINT('Ctrl Pts',(-6.56851488585849,-4.02968927075824,
15.7071589740343));
#62418=CARTESIAN_POINT('Ctrl Pts',(-6.38416972253453,-3.94091623381668,
15.7846830843128));
#62419=CARTESIAN_POINT('Ctrl Pts',(-6.27575645452224,-3.90850154064671,
15.8240515790601));
#62420=CARTESIAN_POINT('Ctrl Pts',(-6.25032976362752,-3.90191196399198,
15.8329676265128));
#62421=CARTESIAN_POINT('Ctrl Pts',(-6.8147193961081,-4.89995455584871,14.669953164421));
#62422=CARTESIAN_POINT('Ctrl Pts',(-6.81499727225807,-4.87301572262855,
14.678855934617));
#62423=CARTESIAN_POINT('Ctrl Pts',(-6.812099620586,-4.75899734568318,14.7176111603106));
#62424=CARTESIAN_POINT('Ctrl Pts',(-6.77625084285897,-4.55998596348717,
14.7932537684509));
#62425=CARTESIAN_POINT('Ctrl Pts',(-6.67257963290984,-4.323764131131,14.8988444918356));
#62426=CARTESIAN_POINT('Ctrl Pts',(-6.52065733174994,-4.12487388367177,
15.0046751914328));
#62427=CARTESIAN_POINT('Ctrl Pts',(-6.33237309875386,-3.97312546011465,
15.1046826999853));
#62428=CARTESIAN_POINT('Ctrl Pts',(-6.16872308841693,-3.89638081767529,
15.1736714985496));
#62429=CARTESIAN_POINT('Ctrl Pts',(-6.07292775271076,-3.86852699329058,
15.2085479485238));
#62430=CARTESIAN_POINT('Ctrl Pts',(-6.05048519755294,-3.86287441690861,
15.21643737952));
#62431=CARTESIAN_POINT('Ctrl Pts',(-7.05843403097223,-4.7130617286742,14.0978966120729));
#62432=CARTESIAN_POINT('Ctrl Pts',(-7.05879586671931,-4.67818074142654,
14.1094309207911));
#62433=CARTESIAN_POINT('Ctrl Pts',(-7.05495515045979,-4.53092818779582,
14.1594239869758));
#62434=CARTESIAN_POINT('Ctrl Pts',(-7.00823869674784,-4.2757195561268,14.2556529815483));
#62435=CARTESIAN_POINT('Ctrl Pts',(-6.87332612944898,-3.97204539859998,
14.3892289048133));
#62436=CARTESIAN_POINT('Ctrl Pts',(-6.67392435495462,-3.71358706477726,
14.5238465046092));
#62437=CARTESIAN_POINT('Ctrl Pts',(-6.42325605566937,-3.51309045810733,
14.6528732158932));
#62438=CARTESIAN_POINT('Ctrl Pts',(-6.20134644756911,-3.40949261292977,
14.7438913470207));
#62439=CARTESIAN_POINT('Ctrl Pts',(-6.06951804969259,-3.37139329470379,
14.7908144841238));
#62440=CARTESIAN_POINT('Ctrl Pts',(-6.03852631344346,-3.3636365870849,14.8014824694433));
#62441=CARTESIAN_POINT('Ctrl Pts',(-7.6717391352104,-4.65164535922602,13.8937800218627));
#62442=CARTESIAN_POINT('Ctrl Pts',(-7.67224282244008,-4.60259943959517,
13.9100094857634));
#62443=CARTESIAN_POINT('Ctrl Pts',(-7.66681627817998,-4.39599674101868,
13.9800501817312));
#62444=CARTESIAN_POINT('Ctrl Pts',(-7.60174266337897,-4.04003661333773,
14.1129447256398));
#62445=CARTESIAN_POINT('Ctrl Pts',(-7.41403799907221,-3.61544944133095,
14.2959874416183));
#62446=CARTESIAN_POINT('Ctrl Pts',(-7.13459369944867,-3.25061869911762,
14.4809417081011));
#62447=CARTESIAN_POINT('Ctrl Pts',(-6.77913623589666,-2.96355669078003,
14.6600886342619));
#62448=CARTESIAN_POINT('Ctrl Pts',(-6.45977429108566,-2.81255128298632,
14.7886657841067));
#62449=CARTESIAN_POINT('Ctrl Pts',(-6.2678543001219,-2.75639262976502,14.8559525099445));
#62450=CARTESIAN_POINT('Ctrl Pts',(-6.22261485799,-2.74492672320326,14.8713078648157));
#62451=CARTESIAN_POINT('',(-6.26385971950436,-3.9057407515351,15.8144217911625));
#62452=CARTESIAN_POINT('',(-6.249946055744,-2.76546777341919,14.8593868371358));
#62453=CARTESIAN_POINT('Ctrl Pts',(-6.26385883867456,-3.90574397279466,
15.8144218264466));
#62454=CARTESIAN_POINT('Ctrl Pts',(-6.2543726558507,-3.90347224101743,15.7850081696593));
#62455=CARTESIAN_POINT('Ctrl Pts',(-6.24505636291581,-3.8997586331618,15.754970629442));
#62456=CARTESIAN_POINT('Ctrl Pts',(-6.23601489483689,-3.89445412934997,
15.7244810600636));
#62457=CARTESIAN_POINT('Ctrl Pts',(-6.22720005999169,-3.88928258811033,
15.6947557415395));
#62458=CARTESIAN_POINT('Ctrl Pts',(-6.21864673046565,-3.88259822555066,
15.6646010810059));
#62459=CARTESIAN_POINT('Ctrl Pts',(-6.21045783981734,-3.87429084484968,
15.6342165675576));
#62460=CARTESIAN_POINT('Ctrl Pts',(-6.20239515995553,-3.86611150115605,
15.6043003536025));
#62461=CARTESIAN_POINT('Ctrl Pts',(-6.194686087777,-3.85635816263781,15.5741617702321));
#62462=CARTESIAN_POINT('Ctrl Pts',(-6.18743004151878,-3.84496269666555,
15.5440252032908));
#62463=CARTESIAN_POINT('Ctrl Pts',(-6.1803014986827,-3.83376747209979,15.5144181968401));
#62464=CARTESIAN_POINT('Ctrl Pts',(-6.17361052747927,-3.82098688893042,
15.4848137750982));
#62465=CARTESIAN_POINT('Ctrl Pts',(-6.16744778180624,-3.80660015448518,
15.455449660021));
#62466=CARTESIAN_POINT('Ctrl Pts',(-6.16664974576687,-3.80473716464505,
15.4516471954477));
#62467=CARTESIAN_POINT('Ctrl Pts',(-6.16586055826526,-3.80284730797896,
15.4478487871275));
#62468=CARTESIAN_POINT('Ctrl Pts',(-6.16508040712673,-3.80093059948325,
15.4440549731565));
#62469=CARTESIAN_POINT('Ctrl Pts',(-6.15914772012249,-3.78635492174353,
15.415204780251));
#62470=CARTESIAN_POINT('Ctrl Pts',(-6.15373872498253,-3.77022241680086,
15.3866195641388));
#62471=CARTESIAN_POINT('Ctrl Pts',(-6.14892799956234,-3.75256704171994,
15.3585423290757));
#62472=CARTESIAN_POINT('Ctrl Pts',(-6.14417890446739,-3.73513785009647,
15.3308247921824));
#62473=CARTESIAN_POINT('Ctrl Pts',(-6.1400131210743,-3.71622457870713,15.3036031100997));
#62474=CARTESIAN_POINT('Ctrl Pts',(-6.13648912711731,-3.69590886727287,
15.2771119965196));
#62475=CARTESIAN_POINT('Ctrl Pts',(-6.13298582646184,-3.67571245205408,
15.2507764418331));
#62476=CARTESIAN_POINT('Ctrl Pts',(-6.13011701977104,-3.65413023060548,
15.2251637063787));
#62477=CARTESIAN_POINT('Ctrl Pts',(-6.12792325820837,-3.63128946871226,
15.2004932784671));
#62478=CARTESIAN_POINT('Ctrl Pts',(-6.12573694009297,-3.60852620567283,
15.1759065574781));
#62479=CARTESIAN_POINT('Ctrl Pts',(-6.12422123270962,-3.58451335694736,
15.1522565058577));
#62480=CARTESIAN_POINT('Ctrl Pts',(-6.12339673479099,-3.55941899377354,
15.1297376556406));
#62481=CARTESIAN_POINT('Ctrl Pts',(-6.12257297899932,-3.53434721792593,
15.1072390745419));
#62482=CARTESIAN_POINT('Ctrl Pts',(-6.12243923347756,-3.50819648918428,
15.0858702824523));
#62483=CARTESIAN_POINT('Ctrl Pts',(-6.12299510830259,-3.48116867719233,
15.0657922315937));
#62484=CARTESIAN_POINT('Ctrl Pts',(-6.12355369181233,-3.45400916321,15.045616343764));
#62485=CARTESIAN_POINT('Ctrl Pts',(-6.12480858945358,-3.42596474665878,
15.0267442829828));
#62486=CARTESIAN_POINT('Ctrl Pts',(-6.12673821499426,-3.39726457790098,
15.0092975879348));
#62487=CARTESIAN_POINT('Ctrl Pts',(-6.12867530627466,-3.36845336791503,
14.9917833914565));
#62488=CARTESIAN_POINT('Ctrl Pts',(-6.13129220496638,-3.33898216552069,
14.9757058503849));
#62489=CARTESIAN_POINT('Ctrl Pts',(-6.13454725450644,-3.30909513575427,
14.9611404987692));
#62490=CARTESIAN_POINT('Ctrl Pts',(-6.13783970378742,-3.27886471116188,
14.9464077947461));
#62491=CARTESIAN_POINT('Ctrl Pts',(-6.14178482931182,-3.24820971518353,
14.9332222789991));
#62492=CARTESIAN_POINT('Ctrl Pts',(-6.14632210404467,-3.21738239942496,
14.9216113893742));
#62493=CARTESIAN_POINT('Ctrl Pts',(-6.14962626908504,-3.19493312204694,
14.9131560284262));
#62494=CARTESIAN_POINT('Ctrl Pts',(-6.15324407131646,-3.17239248102998,
14.9055346078699));
#62495=CARTESIAN_POINT('Ctrl Pts',(-6.15714760202756,-3.14985391999966,
14.8987414182892));
#62496=CARTESIAN_POINT('Ctrl Pts',(-6.16260353328767,-3.11835196733577,
14.8892466357111));
#62497=CARTESIAN_POINT('Ctrl Pts',(-6.16861736085895,-3.08685531503858,
14.8813716106451));
#62498=CARTESIAN_POINT('Ctrl Pts',(-6.17510251310507,-3.05559890399993,
14.8750608827783));
#62499=CARTESIAN_POINT('Ctrl Pts',(-6.1817360245337,-3.02362744797641,14.8686057859913));
#62500=CARTESIAN_POINT('Ctrl Pts',(-6.18886232032284,-2.99190798960375,
14.8637868692114));
#62501=CARTESIAN_POINT('Ctrl Pts',(-6.1963828858837,-2.96065839512122,14.8605021501051));
#62502=CARTESIAN_POINT('Ctrl Pts',(-6.20401485935838,-2.92894587639438,
14.8571687719318));
#62503=CARTESIAN_POINT('Ctrl Pts',(-6.21205251543249,-2.89771762699749,
14.8554146667487));
#62504=CARTESIAN_POINT('Ctrl Pts',(-6.22039239040567,-2.86715933990464,
14.8550993693122));
#62505=CARTESIAN_POINT('Ctrl Pts',(-6.22893231697086,-2.83586804014653,
14.8547765087223));
#62506=CARTESIAN_POINT('Ctrl Pts',(-6.23778880583662,-2.8052794442995,14.8559615384475));
#62507=CARTESIAN_POINT('Ctrl Pts',(-6.24685554194399,-2.77554449068749,
14.8584798139296));
#62508=CARTESIAN_POINT('Ctrl Pts',(-6.24788307588537,-2.77217462597323,
14.858765210295));
#62509=CARTESIAN_POINT('Ctrl Pts',(-6.24891331808174,-2.76881567367841,
14.8590677131818));
#62510=CARTESIAN_POINT('Ctrl Pts',(-6.24994612027011,-2.76546781425246,
14.8593870565277));
#62511=CARTESIAN_POINT('',(-6.99999916823336,-3.16610397564684,14.5427478336087));
#62512=CARTESIAN_POINT('Ctrl Pts',(-6.99999900599707,-3.16610410860577,
14.542748444324));
#62513=CARTESIAN_POINT('Ctrl Pts',(-6.93510613246198,-3.10957084743748,
14.5767970301523));
#62514=CARTESIAN_POINT('Ctrl Pts',(-6.86717629266027,-3.05807923643768,
14.6100325970789));
#62515=CARTESIAN_POINT('Ctrl Pts',(-6.79616395204171,-3.01141659815692,
14.6426005706686));
#62516=CARTESIAN_POINT('Ctrl Pts',(-6.7879512091426,-3.00601995515295,14.6463671328112));
#62517=CARTESIAN_POINT('Ctrl Pts',(-6.77969723483539,-3.0006878852849,14.6501247109457));
#62518=CARTESIAN_POINT('Ctrl Pts',(-6.77140195753717,-2.99542004685623,
14.6538734876845));
#62519=CARTESIAN_POINT('Ctrl Pts',(-6.6913806973046,-2.9446032923814,14.6900364546582));
#62520=CARTESIAN_POINT('Ctrl Pts',(-6.60751418106424,-2.89976441230501,
14.7253809261968));
#62521=CARTESIAN_POINT('Ctrl Pts',(-6.52054164996745,-2.86132532829294,
14.7596579913119));
#62522=CARTESIAN_POINT('Ctrl Pts',(-6.44075323615254,-2.8260613949206,14.7911036974594));
#62523=CARTESIAN_POINT('Ctrl Pts',(-6.35835204191316,-2.79618437114786,
14.8216547520575));
#62524=CARTESIAN_POINT('Ctrl Pts',(-6.27305667611768,-2.77189333807855,
14.8513785255834));
#62525=CARTESIAN_POINT('Ctrl Pts',(-6.2653767150535,-2.76970618305036,14.8540548424176));
#62526=CARTESIAN_POINT('Ctrl Pts',(-6.25767328747102,-2.76756430839692,
14.8567244179092));
#62527=CARTESIAN_POINT('Ctrl Pts',(-6.24994618613909,-2.76546785592883,
14.8593872804758));
#62528=CARTESIAN_POINT('',(-7.000004116699,-4.92966193703766,14.7967990007598));
#62529=CARTESIAN_POINT('Ctrl Pts',(-7.000004116699,-4.92966193703766,14.7967990007598));
#62530=CARTESIAN_POINT('Ctrl Pts',(-7.,-4.84202472118207,14.7620803736131));
#62531=CARTESIAN_POINT('Ctrl Pts',(-7.,-4.69429463291145,14.707019515926));
#62532=CARTESIAN_POINT('Ctrl Pts',(-7.,-4.55642586372495,14.6619279529231));
#62533=CARTESIAN_POINT('Ctrl Pts',(-7.,-4.48005872682265,14.6386028054155));
#62534=CARTESIAN_POINT('Ctrl Pts',(-7.,-4.46232340867955,14.6333102630297));
#62535=CARTESIAN_POINT('Ctrl Pts',(-7.,-4.28372294397391,14.5814732655434));
#62536=CARTESIAN_POINT('Ctrl Pts',(-7.,-4.12833425220785,14.5473037835001));
#62537=CARTESIAN_POINT('Ctrl Pts',(-7.,-3.68749188829301,14.4827479384111));
#62538=CARTESIAN_POINT('Ctrl Pts',(-7.,-3.41573088208626,14.4884018589627));
#62539=CARTESIAN_POINT('Ctrl Pts',(-6.999998498703,-3.16610377894933,14.5427469301253));
#62540=CARTESIAN_POINT('Ctrl Pts',(-6.99999573616303,-4.92966193411623,
14.796799002087));
#62541=CARTESIAN_POINT('Ctrl Pts',(-7.00000221239064,-4.90604265398912,
14.8141315164145));
#62542=CARTESIAN_POINT('Ctrl Pts',(-6.9993066547385,-4.88279824389592,14.8313751281873));
#62543=CARTESIAN_POINT('Ctrl Pts',(-6.99796128285892,-4.85997235031371,
14.8484950322261));
#62544=CARTESIAN_POINT('Ctrl Pts',(-6.9957659811257,-4.82272634829462,14.876430323263));
#62545=CARTESIAN_POINT('Ctrl Pts',(-6.99184296717533,-4.78659534704214,
14.9040352250922));
#62546=CARTESIAN_POINT('Ctrl Pts',(-6.98646530326381,-4.75166688168638,
14.9311959838139));
#62547=CARTESIAN_POINT('Ctrl Pts',(-6.98080871742447,-4.71492679049211,
14.9597654827076));
#62548=CARTESIAN_POINT('Ctrl Pts',(-6.97354226261009,-4.67951736798576,
14.9878435992541));
#62549=CARTESIAN_POINT('Ctrl Pts',(-6.96494107209083,-4.64551155726207,
15.0153240744984));
#62550=CARTESIAN_POINT('Ctrl Pts',(-6.96162739700404,-4.63241055600544,
15.0259111398571));
#62551=CARTESIAN_POINT('Ctrl Pts',(-6.95811521673422,-4.6195175780179,15.0364097634807));
#62552=CARTESIAN_POINT('Ctrl Pts',(-6.95441888664791,-4.60683565951141,
15.0468148125601));
#62553=CARTESIAN_POINT('Ctrl Pts',(-6.94894998148114,-4.58807212702781,
15.0622096028904));
#62554=CARTESIAN_POINT('Ctrl Pts',(-6.94307818160796,-4.56977068691385,
15.0773994620523));
#62555=CARTESIAN_POINT('Ctrl Pts',(-6.93685437929836,-4.55193409922293,
15.0923701643997));
#62556=CARTESIAN_POINT('Ctrl Pts',(-6.92516109036544,-4.51842269203608,
15.1204971419883));
#62557=CARTESIAN_POINT('Ctrl Pts',(-6.91222767712603,-4.48655359241521,
15.1478491401164));
#62558=CARTESIAN_POINT('Ctrl Pts',(-6.89835605056547,-4.45632482916625,
15.1743509988416));
#62559=CARTESIAN_POINT('Ctrl Pts',(-6.88963414684376,-4.43731823599328,
15.1910142689519));
#62560=CARTESIAN_POINT('Ctrl Pts',(-6.88054042884793,-4.41895960534933,
15.2073419408165));
#62561=CARTESIAN_POINT('Ctrl Pts',(-6.87114205357841,-4.40124336406645,
15.2233198223925));
#62562=CARTESIAN_POINT('Ctrl Pts',(-6.86659238605382,-4.39266709366747,
15.2310545687537));
#62563=CARTESIAN_POINT('Ctrl Pts',(-6.86197124058544,-4.38424130608127,
15.2387073925565));
#62564=CARTESIAN_POINT('Ctrl Pts',(-6.85728579233503,-4.37596505290805,
15.2462769460957));
#62565=CARTESIAN_POINT('Ctrl Pts',(-6.84943500692511,-4.36209763101185,
15.2589602449625));
#62566=CARTESIAN_POINT('Ctrl Pts',(-6.84140385349202,-4.3486500597749,15.2714097024552));
#62567=CARTESIAN_POINT('Ctrl Pts',(-6.83322795534013,-4.33561341799617,
15.2836203187907));
#62568=CARTESIAN_POINT('Ctrl Pts',(-6.82670026643618,-4.32520488057279,
15.2933693522648));
#62569=CARTESIAN_POINT('Ctrl Pts',(-6.8200802521166,-4.31505827299739,15.3029661600629));
#62570=CARTESIAN_POINT('Ctrl Pts',(-6.81338485309185,-4.30516863997901,
15.312408702571));
#62571=CARTESIAN_POINT('Ctrl Pts',(-6.81003715357948,-4.30022382346981,
15.317129973825));
#62572=CARTESIAN_POINT('Ctrl Pts',(-6.80667060001253,-4.29534325631977,
15.3218126790656));
#62573=CARTESIAN_POINT('Ctrl Pts',(-6.80328720608736,-4.29052626895533,
15.3264566119654));
#62574=CARTESIAN_POINT('Ctrl Pts',(-6.80115374659458,-4.28748883150449,
15.3293849268315));
#62575=CARTESIAN_POINT('Ctrl Pts',(-6.79936460844594,-4.28496954309885,
15.3318215832851));
#62576=CARTESIAN_POINT('Ctrl Pts',(-6.79725830305816,-4.2820342222537,15.3346675785447));
#62577=CARTESIAN_POINT('Ctrl Pts',(-6.79602427745879,-4.28031449961219,
15.3363349678161));
#62578=CARTESIAN_POINT('Ctrl Pts',(-6.79468083205484,-4.27845241274624,
15.3381428279873));
#62579=CARTESIAN_POINT('Ctrl Pts',(-6.79308848615342,-4.27626539522726,
15.3402718894587));
#62580=CARTESIAN_POINT('Ctrl Pts',(-6.76811254009625,-4.24196202462714,
15.3736662194302));
#62581=CARTESIAN_POINT('Ctrl Pts',(-6.74136333482385,-4.20967407704942,
15.4063529011943));
#62582=CARTESIAN_POINT('Ctrl Pts',(-6.71310658826184,-4.17952400533597,
15.4382319962378));
#62583=CARTESIAN_POINT('Ctrl Pts',(-6.68059306941946,-4.14483193905004,
15.4749135566963));
#62584=CARTESIAN_POINT('Ctrl Pts',(-6.64608492528658,-4.11296986352685,
15.5105256057665));
#62585=CARTESIAN_POINT('Ctrl Pts',(-6.6100324935685,-4.08402521452437,15.5449441229869));
#62586=CARTESIAN_POINT('Ctrl Pts',(-6.58409154092629,-4.06319855365195,
15.5697094184935));
#62587=CARTESIAN_POINT('Ctrl Pts',(-6.55734985374155,-4.04388242560808,
15.5938572668279));
#62588=CARTESIAN_POINT('Ctrl Pts',(-6.52996021466892,-4.02610795854003,
15.617348183742));
#62589=CARTESIAN_POINT('Ctrl Pts',(-6.49082222870598,-4.00070941857521,
15.6509151531351));
#62590=CARTESIAN_POINT('Ctrl Pts',(-6.45036364595694,-3.9784582337298,15.6831400763665));
#62591=CARTESIAN_POINT('Ctrl Pts',(-6.40906282430625,-3.95933753692462,
15.7139351622328));
#62592=CARTESIAN_POINT('Ctrl Pts',(-6.37882678006827,-3.94533940779895,
15.736480030382));
#62593=CARTESIAN_POINT('Ctrl Pts',(-6.34813818136118,-3.9330192341771,15.7582589726189));
#62594=CARTESIAN_POINT('Ctrl Pts',(-6.3171683875425,-3.92236897336695,15.7792438726914));
#62595=CARTESIAN_POINT('Ctrl Pts',(-6.29947922520236,-3.91628581396529,
15.7912299164554));
#62596=CARTESIAN_POINT('Ctrl Pts',(-6.28169810243252,-3.91074736146905,
15.8029570173119));
#62597=CARTESIAN_POINT('Ctrl Pts',(-6.26385883869961,-3.90574397280168,
15.8144218264305));
#62598=CARTESIAN_POINT('Ctrl Pts',(-6.2226708194252,-3.9737511002187,14.5714076900287));
#62599=CARTESIAN_POINT('Ctrl Pts',(-6.22400636097445,-3.92718923052127,
14.9771467016005));
#62600=CARTESIAN_POINT('Ctrl Pts',(-6.2272659484764,-3.85976063408221,16.0460349316959));
#62601=CARTESIAN_POINT('Ctrl Pts',(-6.23205447278337,-3.98191121156329,
17.77942854308));
#62602=CARTESIAN_POINT('Ctrl Pts',(-6.2357082843596,-4.449905047104,19.7179590903193));
#62603=CARTESIAN_POINT('Ctrl Pts',(-6.23759745006902,-5.23225314551589,
21.5545919051479));
#62604=CARTESIAN_POINT('Ctrl Pts',(-6.23804464574047,-6.30682892892631,
23.2351575907732));
#62605=CARTESIAN_POINT('Ctrl Pts',(-6.23649779618595,-7.5400629509749,24.5993867713103));
#62606=CARTESIAN_POINT('Ctrl Pts',(-6.23491000958653,-8.44425820931118,
25.3447854154734));
#62607=CARTESIAN_POINT('Ctrl Pts',(-6.23413471759127,-8.85534285870587,
25.642104093556));
#62608=CARTESIAN_POINT('Ctrl Pts',(-6.71589153124125,-4.08566112089493,
14.5843363286704));
#62609=CARTESIAN_POINT('Ctrl Pts',(-6.71708025714564,-4.04021428388655,
14.9863212787434));
#62610=CARTESIAN_POINT('Ctrl Pts',(-6.71993478201462,-3.97507949372222,
16.045195140519));
#62611=CARTESIAN_POINT('Ctrl Pts',(-6.72416562750028,-4.09849404470664,
17.7615741310517));
#62612=CARTESIAN_POINT('Ctrl Pts',(-6.72736928264046,-4.56367891552375,
19.680427526418));
#62613=CARTESIAN_POINT('Ctrl Pts',(-6.72902533305614,-5.33903915516719,
21.4982065115222));
#62614=CARTESIAN_POINT('Ctrl Pts',(-6.72942032908318,-6.40303073142038,
23.1617848480856));
#62615=CARTESIAN_POINT('Ctrl Pts',(-6.72805279807952,-7.62318976665027,
24.5127338221719));
#62616=CARTESIAN_POINT('Ctrl Pts',(-6.72668452560022,-8.5179375479919,25.2513978787936));
#62617=CARTESIAN_POINT('Ctrl Pts',(-6.72599138112137,-8.92472608290391,
25.5460982756379));
#62618=CARTESIAN_POINT('Ctrl Pts',(-7.02184863765555,-4.48559734860376,
14.6305391207282));
#62619=CARTESIAN_POINT('Ctrl Pts',(-7.02249159491149,-4.44215217831574,
15.0188786224887));
#62620=CARTESIAN_POINT('Ctrl Pts',(-7.02397825402112,-4.38032190132887,
16.0419240163869));
#62621=CARTESIAN_POINT('Ctrl Pts',(-7.02622828780661,-4.50113493796852,
17.6995301397592));
#62622=CARTESIAN_POINT('Ctrl Pts',(-7.02790163053151,-4.95159591349138,
19.5522395072536));
#62623=CARTESIAN_POINT('Ctrl Pts',(-7.02876616760263,-5.70076950232316,
21.3070947338483));
#62624=CARTESIAN_POINT('Ctrl Pts',(-7.02897608662855,-6.72847789631824,
22.9136305902866));
#62625=CARTESIAN_POINT('Ctrl Pts',(-7.02824778608318,-7.90599710067593,
24.2181457116981));
#62626=CARTESIAN_POINT('Ctrl Pts',(-7.02756284280684,-8.7699326895579,24.9320738472432));
#62627=CARTESIAN_POINT('Ctrl Pts',(-7.02718415948163,-9.16263800955179,
25.2168992871523));
#62628=CARTESIAN_POINT('Ctrl Pts',(-6.99898915419192,-4.98714300774216,
14.6884801944114));
#62629=CARTESIAN_POINT('Ctrl Pts',(-6.99894179675862,-4.9456545700149,15.0596433930229));
#62630=CARTESIAN_POINT('Ctrl Pts',(-6.99873531351085,-4.8866027815796,16.0377464795711));
#62631=CARTESIAN_POINT('Ctrl Pts',(-6.99850468239117,-5.00216659736996,
17.6222150007892));
#62632=CARTESIAN_POINT('Ctrl Pts',(-6.99828080321693,-5.43285519889442,
19.3931412354428));
#62633=CARTESIAN_POINT('Ctrl Pts',(-6.99816433590801,-6.14885025059248,
21.0703293239026));
#62634=CARTESIAN_POINT('Ctrl Pts',(-6.99814256690665,-7.13148754762239,
22.6063533322588));
#62635=CARTESIAN_POINT('Ctrl Pts',(-6.9982154541888,-8.25667422537784,23.8529237825218));
#62636=CARTESIAN_POINT('Ctrl Pts',(-6.99835921786227,-9.08279282579766,
24.5356449639657));
#62637=CARTESIAN_POINT('Ctrl Pts',(-6.99838071869229,-9.4581913229097,24.807942025549));
#62638=CARTESIAN_POINT('',(-7.00000355772211,-9.33251602987223,24.7867164860314));
#62639=CARTESIAN_POINT('Ctrl Pts',(-7.00001601661652,-4.92966193654956,
14.796799000911));
#62640=CARTESIAN_POINT('Ctrl Pts',(-7.00002088999999,-4.90663940747915,
15.0161850414432));
#62641=CARTESIAN_POINT('Ctrl Pts',(-7.00001598308917,-4.89043247070465,
15.2342926627982));
#62642=CARTESIAN_POINT('Ctrl Pts',(-7.00000988156703,-4.8806944323136,15.4506299953074));
#62643=CARTESIAN_POINT('Ctrl Pts',(-7.00000652467011,-4.87533681985134,
15.569653102648));
#62644=CARTESIAN_POINT('Ctrl Pts',(-7.0000027909423,-4.87193735837233,15.6881412924022));
#62645=CARTESIAN_POINT('Ctrl Pts',(-6.99999999965555,-4.87043886014772,
15.8060193287844));
#62646=CARTESIAN_POINT('Ctrl Pts',(-6.9999945542241,-4.86751548822153,16.0359837936163));
#62647=CARTESIAN_POINT('Ctrl Pts',(-6.99999266080783,-4.87182625069152,
16.2636232331228));
#62648=CARTESIAN_POINT('Ctrl Pts',(-6.99999257345254,-4.88291897763752,
16.4885266234839));
#62649=CARTESIAN_POINT('Ctrl Pts',(-6.99999248483235,-4.89417232596976,
16.7166865885812));
#62650=CARTESIAN_POINT('Ctrl Pts',(-6.99999425319978,-4.91240544047496,
16.942030746898));
#62651=CARTESIAN_POINT('Ctrl Pts',(-6.99999619758638,-4.93715680472449,
17.1641828826339));
#62652=CARTESIAN_POINT('Ctrl Pts',(-6.99999754425264,-4.95429939706919,
17.3180436340265));
#62653=CARTESIAN_POINT('Ctrl Pts',(-6.99999897835612,-4.97456890745326,
17.4703743349893));
#62654=CARTESIAN_POINT('Ctrl Pts',(-6.99999998662336,-4.99781500190131,
17.621064298088));
#62655=CARTESIAN_POINT('Ctrl Pts',(-7.00000143709326,-5.0312562950098,17.83784338912));
#62656=CARTESIAN_POINT('Ctrl Pts',(-7.00000201442432,-5.07085616110269,
18.0512249470974));
#62657=CARTESIAN_POINT('Ctrl Pts',(-7.00000210876094,-5.11608689795626,
18.2609145834918));
#62658=CARTESIAN_POINT('Ctrl Pts',(-7.00000220461171,-5.16204361117133,
18.4739698453407));
#62659=CARTESIAN_POINT('Ctrl Pts',(-7.00000180216916,-5.21381338809911,
18.6832137767012));
#62660=CARTESIAN_POINT('Ctrl Pts',(-7.00000129011751,-5.27086637534113,
18.8883864605185));
#62661=CARTESIAN_POINT('Ctrl Pts',(-7.00000086166881,-5.31860429121544,
19.0600604918576));
#62662=CARTESIAN_POINT('Ctrl Pts',(-7.00000035619199,-5.37004149973613,
19.2288850931687));
#62663=CARTESIAN_POINT('Ctrl Pts',(-6.99999998816684,-5.42488007155213,
19.3947330695011));
#62664=CARTESIAN_POINT('Ctrl Pts',(-6.9999997037336,-5.46726280749537,19.5229109332719));
#62665=CARTESIAN_POINT('Ctrl Pts',(-6.99999950019787,-5.51167741653189,
19.6493113182398));
#62666=CARTESIAN_POINT('Ctrl Pts',(-6.99999936067318,-5.55798420403389,
19.7738901676013));
#62667=CARTESIAN_POINT('Ctrl Pts',(-6.99999924478743,-5.59644547559882,
19.8773622764436));
#62668=CARTESIAN_POINT('Ctrl Pts',(-6.99999917321303,-5.63621215991117,
19.9795779219696));
#62669=CARTESIAN_POINT('Ctrl Pts',(-6.99999913936352,-5.67720658690967,
20.0805154959337));
#62670=CARTESIAN_POINT('Ctrl Pts',(-6.99999912243876,-5.69770380040891,
20.1309842829157));
#62671=CARTESIAN_POINT('Ctrl Pts',(-6.99999911498658,-5.71850794957971,
20.1811335520072));
#62672=CARTESIAN_POINT('Ctrl Pts',(-6.99999911639991,-5.73960956221651,
20.2309609599606));
#62673=CARTESIAN_POINT('Ctrl Pts',(-6.99999911710658,-5.75016036853491,
20.2558746639373));
#62674=CARTESIAN_POINT('Ctrl Pts',(-6.99999912003183,-5.76078554071981,
20.2807079026295));
#62675=CARTESIAN_POINT('Ctrl Pts',(-6.99999912511198,-5.77148390107702,
20.3054603924112));
#62676=CARTESIAN_POINT('Ctrl Pts',(-6.99999912765206,-5.77683308125563,
20.3178366373021));
#62677=CARTESIAN_POINT('Ctrl Pts',(-6.99999913073098,-5.78220055847731,
20.3301926949653));
#62678=CARTESIAN_POINT('Ctrl Pts',(-6.99999913434149,-5.78758618636081,
20.3425285311915));
#62679=CARTESIAN_POINT('Ctrl Pts',(-6.9999991374978,-5.79229430622029,20.3533125282993));
#62680=CARTESIAN_POINT('Ctrl Pts',(-6.99999914056833,-5.79641054508912,
20.362704005978));
#62681=CARTESIAN_POINT('Ctrl Pts',(-6.99999914483362,-5.8015232358369,20.3743145323038));
#62682=CARTESIAN_POINT('Ctrl Pts',(-6.9999991454474,-5.80225896243464,20.3759853106577));
#62683=CARTESIAN_POINT('Ctrl Pts',(-6.99999914608787,-5.80301540258001,
20.3777020058122));
#62684=CARTESIAN_POINT('Ctrl Pts',(-6.99999914676096,-5.80379737586325,
20.3794753417173));
#62685=CARTESIAN_POINT('Ctrl Pts',(-6.99999923697272,-5.9086019813435,20.6171481291404));
#62686=CARTESIAN_POINT('Ctrl Pts',(-6.9999995214456,-6.02101207659238,20.8492773392419));
#62687=CARTESIAN_POINT('Ctrl Pts',(-6.9999999901846,-6.14041758229643,21.0754641373822));
#62688=CARTESIAN_POINT('Ctrl Pts',(-7.00000044364547,-6.25593116937927,
21.2942785735333));
#62689=CARTESIAN_POINT('Ctrl Pts',(-7.00000106797197,-6.37799088575244,
21.5075321997706));
#62690=CARTESIAN_POINT('Ctrl Pts',(-7.00000142593383,-6.50595763999341,
21.7149317398955));
#62691=CARTESIAN_POINT('Ctrl Pts',(-7.00000178765916,-6.63526978485192,
21.9245117947721));
#62692=CARTESIAN_POINT('Ctrl Pts',(-7.0000018762761,-6.77061383934092,22.128114062787));
#62693=CARTESIAN_POINT('Ctrl Pts',(-7.00000131559658,-6.9113633296045,22.3254778245801));
#62694=CARTESIAN_POINT('Ctrl Pts',(-7.00000103873753,-6.9808642997602,22.4229344682418));
#62695=CARTESIAN_POINT('Ctrl Pts',(-7.0000006048128,-7.05168378324631,22.5188706100842));
#62696=CARTESIAN_POINT('Ctrl Pts',(-6.99999997635844,-7.12374925579272,
22.6132585158635));
#62697=CARTESIAN_POINT('Ctrl Pts',(-6.99999887928061,-7.24955223556239,
22.7780292359001));
#62698=CARTESIAN_POINT('Ctrl Pts',(-6.99999719586419,-7.37915115146265,
22.938081068345));
#62699=CARTESIAN_POINT('Ctrl Pts',(-6.99999590263475,-7.51215861026573,
23.0933375004005));
#62700=CARTESIAN_POINT('Ctrl Pts',(-6.99999568171318,-7.53488019054777,
23.1198598587479));
#62701=CARTESIAN_POINT('Ctrl Pts',(-6.99999546002071,-7.55895205348164,
23.1476959584348));
#62702=CARTESIAN_POINT('Ctrl Pts',(-6.99999525388495,-7.58352667533906,
23.1758121710142));
#62703=CARTESIAN_POINT('Ctrl Pts',(-6.99999512029718,-7.59945243752027,
23.1940330867854));
#62704=CARTESIAN_POINT('Ctrl Pts',(-6.99999499323651,-7.61558858282698,
23.212372274829));
#62705=CARTESIAN_POINT('Ctrl Pts',(-6.99999487630705,-7.63169547194886,
23.2305561143529));
#62706=CARTESIAN_POINT('Ctrl Pts',(-6.99999457894682,-7.67265647511351,
23.2767989550805));
#62707=CARTESIAN_POINT('Ctrl Pts',(-6.99999434327586,-7.71387574907449,
23.3225495461325));
#62708=CARTESIAN_POINT('Ctrl Pts',(-6.99999419420493,-7.75533999032782,
23.3678081095132));
#62709=CARTESIAN_POINT('Ctrl Pts',(-6.9999936547506,-7.90538979191992,23.5315887130004));
#62710=CARTESIAN_POINT('Ctrl Pts',(-6.99999426200499,-8.05864834217112,
23.6889265209168));
#62711=CARTESIAN_POINT('Ctrl Pts',(-6.99999708872685,-8.21453766136163,
23.8398712965581));
#62712=CARTESIAN_POINT('Ctrl Pts',(-6.99999738651101,-8.23095999526624,
23.8557727420171));
#62713=CARTESIAN_POINT('Ctrl Pts',(-6.99999770877356,-8.24741156308034,
23.8716032672587));
#62714=CARTESIAN_POINT('Ctrl Pts',(-6.9999980566607,-8.26389171586799,23.8873629503283));
#62715=CARTESIAN_POINT('Ctrl Pts',(-6.99999863110429,-8.29110432907967,
23.91338589837));
#62716=CARTESIAN_POINT('Ctrl Pts',(-6.99999927542335,-8.3183948795832,23.939215688115));
#62717=CARTESIAN_POINT('Ctrl Pts',(-6.99999999465543,-8.3457604764835,23.9648526933387));
#62718=CARTESIAN_POINT('Ctrl Pts',(-7.00000393348348,-8.49562640279979,
24.1052520988337));
#62719=CARTESIAN_POINT('Ctrl Pts',(-7.00001006471687,-8.64773932553411,
24.2398676036782));
#62720=CARTESIAN_POINT('Ctrl Pts',(-7.00001375741759,-8.80155013567985,
24.3687621556948));
#62721=CARTESIAN_POINT('Ctrl Pts',(-7.00001750460692,-8.95763054129899,
24.4995586448479));
#62722=CARTESIAN_POINT('Ctrl Pts',(-7.00001874206943,-9.11545935639289,
24.624464169466));
#62723=CARTESIAN_POINT('Ctrl Pts',(-7.00001328591826,-9.27450984411414,
24.7435698673835));
#62724=CARTESIAN_POINT('Ctrl Pts',(-7.0000126232107,-9.29382821661489,24.7580365205343));
#62725=CARTESIAN_POINT('Ctrl Pts',(-7.00001186252235,-9.31316466773027,
24.7724176402076));
#62726=CARTESIAN_POINT('Ctrl Pts',(-7.00001099698708,-9.33251829944508,
24.786713413932));
#62727=CARTESIAN_POINT('',(-6.271594443024,-8.76071211955051,25.5608538793679));
#62728=CARTESIAN_POINT('Origin',(-5.99998362344619,-9.33252812839836,24.7867137519315));
#62729=CARTESIAN_POINT('Ctrl Pts',(-6.26386060032414,-3.90573753027274,
15.8144217558848));
#62730=CARTESIAN_POINT('Ctrl Pts',(-6.26455152175083,-3.90327936026393,
16.0555052700955));
#62731=CARTESIAN_POINT('Ctrl Pts',(-6.26520986012939,-3.9081043619149,16.2942816114619));
#62732=CARTESIAN_POINT('Ctrl Pts',(-6.26583561550458,-3.91978362271735,
16.5303239214902));
#62733=CARTESIAN_POINT('Ctrl Pts',(-6.26647067022013,-3.93163644882302,
16.769874052416));
#62734=CARTESIAN_POINT('Ctrl Pts',(-6.26707216630542,-3.95054874472424,
17.0066083324543));
#62735=CARTESIAN_POINT('Ctrl Pts',(-6.26764010380723,-3.97608047843518,
17.2401341043066));
#62736=CARTESIAN_POINT('Ctrl Pts',(-6.26812468823025,-3.99786505932561,
17.4393865767204));
#62737=CARTESIAN_POINT('Ctrl Pts',(-6.26858484164298,-4.02446879834471,
17.6363041707521));
#62738=CARTESIAN_POINT('Ctrl Pts',(-6.26902056407448,-4.05562321000105,
17.8306725463686));
#62739=CARTESIAN_POINT('Ctrl Pts',(-6.26953467329408,-4.09238232338637,
18.0600079367018));
#62740=CARTESIAN_POINT('Ctrl Pts',(-6.2700147705382,-4.13547525594668,18.2857935310089));
#62741=CARTESIAN_POINT('Ctrl Pts',(-6.27046085585454,-4.18435811903019,
18.5077389773028));
#62742=CARTESIAN_POINT('Ctrl Pts',(-6.27062083612231,-4.2018890559131,18.5873356163904));
#62743=CARTESIAN_POINT('Ctrl Pts',(-6.27077644189198,-4.22016489628043,
18.6664387862204));
#62744=CARTESIAN_POINT('Ctrl Pts',(-6.27092767316578,-4.23916129209173,
18.7450365386642));
#62745=CARTESIAN_POINT('Ctrl Pts',(-6.27136815335618,-4.29449069476137,
18.9739624221364));
#62746=CARTESIAN_POINT('Ctrl Pts',(-6.27177152290998,-4.3559308539005,19.1985968468994));
#62747=CARTESIAN_POINT('Ctrl Pts',(-6.27213778182718,-4.42289857364307,
19.418679912614));
#62748=CARTESIAN_POINT('Ctrl Pts',(-6.27250404074439,-4.48986629338564,
19.6387629783285));
#62749=CARTESIAN_POINT('Ctrl Pts',(-6.27283318902499,-4.56236163369194,
19.8542948916035));
#62750=CARTESIAN_POINT('Ctrl Pts',(-6.27312522666899,-4.6398280945072,20.0650658431881));
#62751=CARTESIAN_POINT('Ctrl Pts',(-6.27334041971111,-4.69691061009187,
20.2203761026475));
#62752=CARTESIAN_POINT('Ctrl Pts',(-6.27353526211499,-4.75658572964704,
20.372823953505));
#62753=CARTESIAN_POINT('Ctrl Pts',(-6.273709975537,-4.8187447529144,20.5226551291307));
#62754=CARTESIAN_POINT('Ctrl Pts',(-6.27388468895901,-4.88090377618176,
20.6724863047565));
#62755=CARTESIAN_POINT('Ctrl Pts',(-6.27403927339914,-4.94554697291618,
20.8197011373369));
#62756=CARTESIAN_POINT('Ctrl Pts',(-6.27417395051376,-5.01262254851192,
20.9645377631236));
#62757=CARTESIAN_POINT('Ctrl Pts',(-6.2742701358658,-5.06052740502531,21.0679789593351));
#62758=CARTESIAN_POINT('Ctrl Pts',(-6.27435616707685,-5.10967408453046,
21.1702069755043));
#62759=CARTESIAN_POINT('Ctrl Pts',(-6.27443212489378,-5.16004936933893,
21.2713099134374));
#62760=CARTESIAN_POINT('Ctrl Pts',(-6.27457884399237,-5.25735359261647,
21.4665989898976));
#62761=CARTESIAN_POINT('Ctrl Pts',(-6.27469165383684,-5.36122084707669,
21.6616529330288));
#62762=CARTESIAN_POINT('Ctrl Pts',(-6.27477055442719,-5.47186421246134,
21.8559699205302));
#62763=CARTESIAN_POINT('Ctrl Pts',(-6.27484862758721,-5.58134726110199,
22.0482491061854));
#62764=CARTESIAN_POINT('Ctrl Pts',(-6.27489349897643,-5.697465120118,22.239806792428));
#62765=CARTESIAN_POINT('Ctrl Pts',(-6.27490516859484,-5.82040639948584,
22.4301097733835));
#62766=CARTESIAN_POINT('Ctrl Pts',(-6.27491664462263,-5.94130817094473,
22.6172557639712));
#62767=CARTESIAN_POINT('Ctrl Pts',(-6.27489601132961,-6.06880890001566,
22.8031883574526));
#62768=CARTESIAN_POINT('Ctrl Pts',(-6.27484326871578,-6.20306971746703,
22.9873540527557));
#62769=CARTESIAN_POINT('Ctrl Pts',(-6.27479056618878,-6.33722849050585,
23.1713797736377));
#62770=CARTESIAN_POINT('Ctrl Pts',(-6.27470580313154,-6.4781371784492,23.3536414281399));
#62771=CARTESIAN_POINT('Ctrl Pts',(-6.27458897954408,-6.62593698870859,
23.5335386059839));
#62772=CARTESIAN_POINT('Ctrl Pts',(-6.27454781339659,-6.67801849828322,
23.5969305452151));
#62773=CARTESIAN_POINT('Ctrl Pts',(-6.27450266631469,-6.73095549786687,
23.6600284363159));
#62774=CARTESIAN_POINT('Ctrl Pts',(-6.2744535382863,-6.78475355160887,23.7228045291512));
#62775=CARTESIAN_POINT('Ctrl Pts',(-6.27431624073854,-6.9351023666132,23.8982441689131));
#62776=CARTESIAN_POINT('Ctrl Pts',(-6.27414785086344,-7.09217875388589,
24.0711732067128));
#62777=CARTESIAN_POINT('Ctrl Pts',(-6.27394836839685,-7.25599608303936,
24.2410353888947));
#62778=CARTESIAN_POINT('Ctrl Pts',(-6.27375072698655,-7.41830151528236,
24.4093298852295));
#62779=CARTESIAN_POINT('Ctrl Pts',(-6.27352256425359,-7.58722412006469,
24.5746139216277));
#62780=CARTESIAN_POINT('Ctrl Pts',(-6.27326387994108,-7.76274424252956,
24.7363078359475));
#62781=CARTESIAN_POINT('Ctrl Pts',(-6.27300884359698,-7.93578917870382,
24.8957215412841));
#62782=CARTESIAN_POINT('Ctrl Pts',(-6.27272414043476,-8.11524691732745,
25.05164567822));
#62783=CARTESIAN_POINT('Ctrl Pts',(-6.27240977020824,-8.30106579828263,
25.2034866126879));
#62784=CARTESIAN_POINT('Ctrl Pts',(-6.27215746706192,-8.45019788635873,
25.3253491247008));
#62785=CARTESIAN_POINT('Ctrl Pts',(-6.27188605495391,-8.60342667624941,
25.444580887195));
#62786=CARTESIAN_POINT('Ctrl Pts',(-6.27159553375696,-8.76070944735565,
25.5608567073969));
#62787=CARTESIAN_POINT('Origin',(-5.999994993365,-9.33250915082771,24.786719601394));
#62788=CARTESIAN_POINT('',(-5.98852246669791,-9.69456809148781,25.7188096068216));
#62789=CARTESIAN_POINT('Origin',(-5.999994993365,-9.33250915082771,24.786719601394));
#62790=CARTESIAN_POINT('Origin',(-6.,-9.33251101023518,24.7867243682986));
#62791=CARTESIAN_POINT('Ctrl Pts',(-5.98841833135407,-9.69410638613233,
25.7189877568217));
#62792=CARTESIAN_POINT('Ctrl Pts',(-5.98810627251156,-9.81679902707702,
25.6713270235229));
#62793=CARTESIAN_POINT('Ctrl Pts',(-5.9872640505419,-10.2439465987631,25.5029619509409));
#62794=CARTESIAN_POINT('Ctrl Pts',(-5.98726405054096,-10.7897532367295,
25.2768814390181));
#62795=CARTESIAN_POINT('Ctrl Pts',(-5.9881062725289,-11.2108442676179,25.0938945781174));
#62796=CARTESIAN_POINT('Ctrl Pts',(-5.98841833138675,-11.331302297366,25.0408390057578));
#62797=CARTESIAN_POINT('Ctrl Pts',(-6.5801963768428,-9.69658810056987,25.7253769392478));
#62798=CARTESIAN_POINT('Ctrl Pts',(-6.57988216944744,-9.81936870227868,
25.6778801647674));
#62799=CARTESIAN_POINT('Ctrl Pts',(-6.57903377815079,-10.246776088706,25.509948484126));
#62800=CARTESIAN_POINT('Ctrl Pts',(-6.57903377814996,-10.7926927101977,
25.2838224155365));
#62801=CARTESIAN_POINT('Ctrl Pts',(-6.57988216946375,-11.2136610034673,
25.1003453834807));
#62802=CARTESIAN_POINT('Ctrl Pts',(-6.58019637687482,-11.3340652944744,
25.0471116770712));
#62803=CARTESIAN_POINT('Ctrl Pts',(-7.00079677511913,-9.5458459940663,25.3372908855745));
#62804=CARTESIAN_POINT('Ctrl Pts',(-7.00061249046053,-9.66739287514854,
25.2904141399614));
#62805=CARTESIAN_POINT('Ctrl Pts',(-7.00011448997313,-10.0904742321413,
25.1245686165554));
#62806=CARTESIAN_POINT('Ctrl Pts',(-7.00011448997309,-10.6307100951158,
24.9007955951957));
#62807=CARTESIAN_POINT('Ctrl Pts',(-7.00061249047014,-11.0471442876849,
24.7189023919596));
#62808=CARTESIAN_POINT('Ctrl Pts',(-7.00079677513743,-11.166237779811,24.66610263116));
#62809=CARTESIAN_POINT('Ctrl Pts',(-6.99999917318234,-9.33157249891016,
24.7856430605173));
#62810=CARTESIAN_POINT('Ctrl Pts',(-6.99999957776342,-9.45129805339181,
24.7394735044865));
#62811=CARTESIAN_POINT('Ctrl Pts',(-7.00000004362102,-9.8680415619029,24.576125658625));
#62812=CARTESIAN_POINT('Ctrl Pts',(-7.00000004362183,-10.4001860098336,
24.3557042111086));
#62813=CARTESIAN_POINT('Ctrl Pts',(-6.99999957776368,-10.8103725420085,
24.1765264188007));
#62814=CARTESIAN_POINT('Ctrl Pts',(-6.99999917318159,-10.9276781031443,
24.1245144718731));
#62815=CARTESIAN_POINT('Origin',(-5.98852353414949,4.7522901968022,-11.4730434396584));
#62816=CARTESIAN_POINT('Origin',(-7.00021006966348,4.74293596854153,-11.4504602201464));
#62817=CARTESIAN_POINT('Ctrl Pts',(-6.05512388577107,-9.37217231939293,
25.8431943550442));
#62818=CARTESIAN_POINT('Ctrl Pts',(-4.03674925718073,-8.81555631688386,
26.0304372976439));
#62819=CARTESIAN_POINT('Ctrl Pts',(7.61020413204277E-7,-8.27057817080118,
26.2482647770642));
#62820=CARTESIAN_POINT('Ctrl Pts',(4.03675077922157,-8.81555652236587,26.0304372155136));
#62821=CARTESIAN_POINT('Ctrl Pts',(6.05512616883189,-9.37217294900257,25.8431941432457));
#62822=CARTESIAN_POINT('Ctrl Pts',(-6.05512388577107,-10.1400098573304,
25.5527871582871));
#62823=CARTESIAN_POINT('Ctrl Pts',(-4.03674925718073,-9.95059989273131,
25.6069155418854));
#62824=CARTESIAN_POINT('Ctrl Pts',(7.61020413204277E-7,-9.81341069027344,
25.7964954224481));
#62825=CARTESIAN_POINT('Ctrl Pts',(4.03675077922157,-9.95059994445685,25.6069154704024));
#62826=CARTESIAN_POINT('Ctrl Pts',(6.05512616883189,-10.1400100715769,25.5527870970548));
#62827=CARTESIAN_POINT('Ctrl Pts',(-6.05512388577107,-10.8990877228837,
25.2383593897359));
#62828=CARTESIAN_POINT('Ctrl Pts',(-4.03674925718073,-11.0715845951584,
25.1425759551505));
#62829=CARTESIAN_POINT('Ctrl Pts',(7.61020413651836E-7,-11.3029258412939,
25.1794677576838));
#62830=CARTESIAN_POINT('Ctrl Pts',(4.03675077922157,-11.0715845079327,25.1425759412421));
#62831=CARTESIAN_POINT('Ctrl Pts',(6.05512616883189,-10.8990875277674,25.238359498084));
#62832=CARTESIAN_POINT('Ctrl Pts',(-6.05512388577107,-11.6473739575525,
24.9007527141814));
#62833=CARTESIAN_POINT('Ctrl Pts',(-4.03674925718073,-12.1736465516541,
24.6394332194205));
#62834=CARTESIAN_POINT('Ctrl Pts',(7.61020413651836E-7,-12.7132798561856,
24.4078866218257));
#62835=CARTESIAN_POINT('Ctrl Pts',(4.03675077922157,-12.1736463481894,24.639433306728));
#62836=CARTESIAN_POINT('Ctrl Pts',(6.05512616883189,-11.6473733622648,24.9007530097704));
#62837=CARTESIAN_POINT('Ctrl Pts',(-5.98852262888646,-9.69456765092853,
25.7188097475992));
#62838=CARTESIAN_POINT('Ctrl Pts',(-5.93898436053355,-9.67817087502701,
25.7245691049754));
#62839=CARTESIAN_POINT('Ctrl Pts',(-5.88247527727907,-9.65963316949226,
25.7310995806593));
#62840=CARTESIAN_POINT('Ctrl Pts',(-5.81892446422276,-9.63914044126316,
25.7383491666606));
#62841=CARTESIAN_POINT('Ctrl Pts',(-5.75779203952735,-9.61942755160809,
25.745322873982));
#62842=CARTESIAN_POINT('Ctrl Pts',(-5.69014336124076,-9.59790579669414,
25.7529620583438));
#62843=CARTESIAN_POINT('Ctrl Pts',(-5.61590486620461,-9.57478231219134,
25.7612053328932));
#62844=CARTESIAN_POINT('Ctrl Pts',(-5.54019770411008,-9.55120137364199,
25.7696116849104));
#62845=CARTESIAN_POINT('Ctrl Pts',(-5.45763719809451,-9.52595445950312,
25.7786465156618));
#62846=CARTESIAN_POINT('Ctrl Pts',(-5.36813769574401,-9.49930636707747,
25.7882262167553));
#62847=CARTESIAN_POINT('Ctrl Pts',(-5.32338794456876,-9.48598232086465,
25.7930160673021));
#62848=CARTESIAN_POINT('Ctrl Pts',(-5.2769033461206,-9.47230870126358,25.7979418256434));
#62849=CARTESIAN_POINT('Ctrl Pts',(-5.2286727814214,-9.45832303024694,25.8029910315361));
#62850=CARTESIAN_POINT('Ctrl Pts',(-5.20455749907179,-9.45133019473862,
25.8055156344824));
#62851=CARTESIAN_POINT('Ctrl Pts',(-5.18000572518015,-9.44425934494013,
25.808071095541));
#62852=CARTESIAN_POINT('Ctrl Pts',(-5.15501605465378,-9.43711552411567,
25.8106556929332));
#62853=CARTESIAN_POINT('Ctrl Pts',(-5.13002638412742,-9.4299717032912,25.8132402903255));
#62854=CARTESIAN_POINT('Ctrl Pts',(-5.10342519951994,-9.42242436287353,
25.8159738674462));
#62855=CARTESIAN_POINT('Ctrl Pts',(-5.07873195594013,-9.41547021113734,
25.8184951418982));
#62856=CARTESIAN_POINT('Ctrl Pts',(-5.06392831161827,-9.41130118455604,
25.8200066505059));
#62857=CARTESIAN_POINT('Ctrl Pts',(-5.04923287210674,-9.40718159317273,
25.8215011286591));
#62858=CARTESIAN_POINT('Ctrl Pts',(-5.03464595226408,-9.40311067339794,
25.8229787770826));
#62859=CARTESIAN_POINT('Ctrl Pts',(-4.9173131829933,-9.37036542657352,25.8348645338705));
#62860=CARTESIAN_POINT('Ctrl Pts',(-4.80700429114233,-9.3407658895739,25.8456618845693));
#62861=CARTESIAN_POINT('Ctrl Pts',(-4.70385804214751,-9.31394075329404,
25.8554800114032));
#62862=CARTESIAN_POINT('Ctrl Pts',(-4.60105414252729,-9.28720465145526,
25.8652655512102));
#62863=CARTESIAN_POINT('Ctrl Pts',(-4.50536510919138,-9.26322438846416,
25.8740785601528));
#62864=CARTESIAN_POINT('Ctrl Pts',(-4.41690034486915,-9.24167510219215,
25.8820193538411));
#62865=CARTESIAN_POINT('Ctrl Pts',(-4.3842827801574,-9.2337297327012,25.8849471788794));
#62866=CARTESIAN_POINT('Ctrl Pts',(-4.35264706504086,-9.22611527434213,
25.88775633941));
#62867=CARTESIAN_POINT('Ctrl Pts',(-4.32199784036469,-9.21881698675232,
25.8904515152313));
#62868=CARTESIAN_POINT('Ctrl Pts',(-4.28740661835289,-9.21058001864,25.8934933352506));
#62869=CARTESIAN_POINT('Ctrl Pts',(-4.25407197310449,-9.20274575444108,
25.8963899723563));
#62870=CARTESIAN_POINT('Ctrl Pts',(-4.22199993581219,-9.19529432826471,
25.8991478200083));
#62871=CARTESIAN_POINT('Ctrl Pts',(-4.20596391716604,-9.19156861517652,
25.9005267438343));
#62872=CARTESIAN_POINT('Ctrl Pts',(-4.19024355050934,-9.18793861239127,
25.9018709724553));
#62873=CARTESIAN_POINT('Ctrl Pts',(-4.17483951758381,-9.18440199481933,
25.9031812605705));
#62874=CARTESIAN_POINT('Ctrl Pts',(-4.16713750112104,-9.18263368603336,
25.903836404628));
#62875=CARTESIAN_POINT('Ctrl Pts',(-4.15951456809107,-9.1808887235961,25.9044830636818));
#62876=CARTESIAN_POINT('Ctrl Pts',(-4.15197080194161,-9.17916682159851,
25.9051213311328));
#62877=CARTESIAN_POINT('Ctrl Pts',(-4.14819891886689,-9.17830587059972,
25.9054404648582));
#62878=CARTESIAN_POINT('Ctrl Pts',(-4.1444468275123,-9.1774506847135,25.9057575006902));
#62879=CARTESIAN_POINT('Ctrl Pts',(-4.1407145380735,-9.17660122874452,25.9060724501517));
#62880=CARTESIAN_POINT('Ctrl Pts',(-4.13884839335409,-9.17617650076003,
25.9062299248824));
#62881=CARTESIAN_POINT('Ctrl Pts',(-4.13698719911364,-9.17575320525501,
25.906386878021));
#62882=CARTESIAN_POINT('Ctrl Pts',(-4.13513095661149,-9.17533133786587,
25.9065433109975));
#62883=CARTESIAN_POINT('Ctrl Pts',(-4.13327471410933,-9.17490947047673,
25.9066997439741));
#62884=CARTESIAN_POINT('Ctrl Pts',(-4.13318162789786,-9.17488804538954,
25.906707680303));
#62885=CARTESIAN_POINT('Ctrl Pts',(-4.12957708557479,-9.17407001569364,
25.907011050869));
#62886=CARTESIAN_POINT('Ctrl Pts',(-4.08632512252271,-9.16425423687577,
25.9106512834799));
#62887=CARTESIAN_POINT('Ctrl Pts',(-4.04419451593996,-9.15484676570599,
25.9141451442275));
#62888=CARTESIAN_POINT('Ctrl Pts',(-4.00319215047733,-9.14582510012115,
25.9174997768095));
#62889=CARTESIAN_POINT('Ctrl Pts',(-3.90003901700451,-9.12312852972282,
25.9259393109333));
#62890=CARTESIAN_POINT('Ctrl Pts',(-3.80402833489472,-9.10287062112949,
25.9334985127824));
#62891=CARTESIAN_POINT('Ctrl Pts',(-3.71525318357639,-9.08472321242478,
25.9402858927437));
#62892=CARTESIAN_POINT('Ctrl Pts',(-3.62699494431028,-9.06668147083678,
25.9470337517529));
#62893=CARTESIAN_POINT('Ctrl Pts',(-3.54588795407541,-9.05072561884383,
25.9530188688104));
#62894=CARTESIAN_POINT('Ctrl Pts',(-3.4720030082679,-9.0365784472142,25.9583351550519));
#62895=CARTESIAN_POINT('Ctrl Pts',(-3.41340786055448,-9.02535890035922,
25.9625512856074));
#62896=CARTESIAN_POINT('Ctrl Pts',(-3.35935453569501,-9.01527776895949,
25.9663465298263));
#62897=CARTESIAN_POINT('Ctrl Pts',(-3.3098705527171,-9.00621781931329,25.9697613075137));
#62898=CARTESIAN_POINT('Ctrl Pts',(-3.27660567797744,-9.00012740233405,
25.9720568412441));
#62899=CARTESIAN_POINT('Ctrl Pts',(-3.24540555097381,-8.99449884385767,
25.9741803228472));
#62900=CARTESIAN_POINT('Ctrl Pts',(-3.21627699481478,-8.98930142713313,
25.9761424569287));
#62901=CARTESIAN_POINT('Ctrl Pts',(-3.20171271673527,-8.98670271877085,
25.9771235239694));
#62902=CARTESIAN_POINT('Ctrl Pts',(-3.18766633137259,-8.98421179646901,
25.9780642558627));
#62903=CARTESIAN_POINT('Ctrl Pts',(-3.17413856470909,-8.9818252665669,25.978965841365));
#62904=CARTESIAN_POINT('Ctrl Pts',(-3.16737468137735,-8.98063200161584,
25.9794166341161));
#62905=CARTESIAN_POINT('Ctrl Pts',(-3.16074045272067,-8.97946483479674,
25.9798576403585));
#62906=CARTESIAN_POINT('Ctrl Pts',(-3.15423596653136,-8.97832335474324,
25.9802890046405));
#62907=CARTESIAN_POINT('Ctrl Pts',(-3.15098372343671,-8.97775261471649,
25.9805046867815));
#62908=CARTESIAN_POINT('Ctrl Pts',(-3.14776391595891,-8.97718829638282,
25.9807179584371));
#62909=CARTESIAN_POINT('Ctrl Pts',(-3.14457655464353,-8.97663034991889,
25.9809288371351));
#62910=CARTESIAN_POINT('Ctrl Pts',(-3.14138919332815,-8.97607240345496,
25.9811397158331));
#62911=CARTESIAN_POINT('Ctrl Pts',(-3.13654159639592,-8.97522524816651,
25.9814599337183));
#62912=CARTESIAN_POINT('Ctrl Pts',(-3.13511181960606,-8.97497557679973,
25.9815543117296));
#62913=CARTESIAN_POINT('Ctrl Pts',(-3.11926201300701,-8.97220784207018,
25.98260054023));
#62914=CARTESIAN_POINT('Ctrl Pts',(-3.09633139320336,-8.96820454104232,
25.9841138922302));
#62915=CARTESIAN_POINT('Ctrl Pts',(-3.06630403421781,-8.96304322994323,
25.986066638726));
#62916=CARTESIAN_POINT('Ctrl Pts',(-3.0363918420494,-8.95790171451689,25.9880118956654));
#62917=CARTESIAN_POINT('Ctrl Pts',(-2.99943716317865,-8.951611038267,25.9903932118209));
#62918=CARTESIAN_POINT('Ctrl Pts',(-2.95541545647122,-8.94429571968719,
25.9931657462656));
#62919=CARTESIAN_POINT('Ctrl Pts',(-2.93782840563912,-8.94137318693372,
25.9942733976462));
#62920=CARTESIAN_POINT('Ctrl Pts',(-2.91911331508352,-8.93828765186099,
25.9954432923733));
#62921=CARTESIAN_POINT('Ctrl Pts',(-2.89926827636051,-8.93504921567418,
25.9966717693497));
#62922=CARTESIAN_POINT('Ctrl Pts',(-2.84975151646082,-8.92696876446665,
25.9997370291525));
#62923=CARTESIAN_POINT('Ctrl Pts',(-2.79320020456681,-8.91793299536115,
26.0031682944269));
#62924=CARTESIAN_POINT('Ctrl Pts',(-2.72958061231902,-8.90813227349094,
26.0068961507412));
#62925=CARTESIAN_POINT('Ctrl Pts',(-2.66637937430061,-8.8983959999031,26.0105994931533));
#62926=CARTESIAN_POINT('Ctrl Pts',(-2.5962023367641,-8.88790478805659,26.0145955811916));
#62927=CARTESIAN_POINT('Ctrl Pts',(-2.51901249338794,-8.87689297298689,
26.018797979586));
#62928=CARTESIAN_POINT('Ctrl Pts',(-2.46596176830785,-8.86932481701785,
26.0216861870514));
#62929=CARTESIAN_POINT('Ctrl Pts',(-2.40959846992732,-8.86151174051651,
26.0246714661818));
#62930=CARTESIAN_POINT('Ctrl Pts',(-2.34991019551084,-8.85354310269698,
26.0277204859783));
#62931=CARTESIAN_POINT('Ctrl Pts',(-2.31814365623095,-8.84930213495624,
26.0293431967717));
#62932=CARTESIAN_POINT('Ctrl Pts',(-2.2854353336339,-8.8450172898929,26.030983887705));
#62933=CARTESIAN_POINT('Ctrl Pts',(-2.25178337805218,-8.840703317834,26.0326370147983));
#62934=CARTESIAN_POINT('Ctrl Pts',(-2.23495740026131,-8.83854633180455,
26.0334635783449));
#62935=CARTESIAN_POINT('Ctrl Pts',(-2.21789551422063,-8.83638206375512,
26.0342932501494));
#62936=CARTESIAN_POINT('Ctrl Pts',(-2.20059749295585,-8.83421245826841,
26.0351252967679));
#62937=CARTESIAN_POINT('Ctrl Pts',(-2.19194848232346,-8.83312765552505,
26.0355413200772));
#62938=CARTESIAN_POINT('Ctrl Pts',(-2.1832404378848,-8.83204151840427,26.0359579370378));
#62939=CARTESIAN_POINT('Ctrl Pts',(-2.17447333152382,-8.83095429277892,
26.0363750546369));
#62940=CARTESIAN_POINT('Ctrl Pts',(-2.16789800175309,-8.83013887355991,
26.0366878928362));
#62941=CARTESIAN_POINT('Ctrl Pts',(-2.16128944965104,-8.82932284205554,
26.0370010126402));
#62942=CARTESIAN_POINT('Ctrl Pts',(-2.1546476634258,-8.82850630317931,26.037314374306));
#62943=CARTESIAN_POINT('Ctrl Pts',(-2.15243373468405,-8.8282341235539,26.0374188281946));
#62944=CARTESIAN_POINT('Ctrl Pts',(-2.14891110169832,-8.827801919456,26.0375847057948));
#62945=CARTESIAN_POINT('Ctrl Pts',(-2.14799479872992,-8.82768959917277,
26.037627815079));
#62946=CARTESIAN_POINT('Ctrl Pts',(-2.01247654850243,-8.81107779197115,
26.0440035390174));
#62947=CARTESIAN_POINT('Ctrl Pts',(-1.87292257322361,-8.79561898355788,
26.0499626459348));
#62948=CARTESIAN_POINT('Ctrl Pts',(-1.72934633996503,-8.78158412302116,
26.0553978387469));
#62949=CARTESIAN_POINT('Ctrl Pts',(-1.55028977293231,-8.76408098974171,
26.0621761678897));
#62950=CARTESIAN_POINT('Ctrl Pts',(-1.36497648425363,-8.74879217455378,
26.0681404534892));
#62951=CARTESIAN_POINT('Ctrl Pts',(-1.17345041796963,-8.73624782919835,
26.0730613254694));
#62952=CARTESIAN_POINT('Ctrl Pts',(-0.994937122853128,-8.72455577877448,
26.0776478608119));
#62953=CARTESIAN_POINT('Ctrl Pts',(-0.811026655105664,-8.71524826294544,
26.0813278035741));
#62954=CARTESIAN_POINT('Ctrl Pts',(-0.621779446010509,-8.70877956174966,
26.0838948793462));
#62955=CARTESIAN_POINT('Ctrl Pts',(-0.437414705199804,-8.70247774929471,
26.0863957260516));
#62956=CARTESIAN_POINT('Ctrl Pts',(-0.247983386096974,-8.69887045341315,
26.0878397960718));
#62957=CARTESIAN_POINT('Ctrl Pts',(-0.0536310989065854,-8.69839216830185,
26.0880416703161));
#62958=CARTESIAN_POINT('Ctrl Pts',(0.0580839165268676,-8.69811724676959,
26.0881577090036));
#62959=CARTESIAN_POINT('Ctrl Pts',(0.171424025792903,-8.69887651459616,
26.087863092153));
#62960=CARTESIAN_POINT('Ctrl Pts',(0.286354490943671,-8.70075531922724,
26.0871207012052));
#62961=CARTESIAN_POINT('Ctrl Pts',(0.308564744031445,-8.70111839725276,
26.0869772345376));
#62962=CARTESIAN_POINT('Ctrl Pts',(0.330834373102222,-8.70152329087806,
26.0868170413609));
#62963=CARTESIAN_POINT('Ctrl Pts',(0.353163103461588,-8.70197062504175,
26.0866398476152));
#62964=CARTESIAN_POINT('Ctrl Pts',(0.484464472008564,-8.70460111889181,
26.0855978814603));
#62965=CARTESIAN_POINT('Ctrl Pts',(0.617809998392041,-8.70869875543607,
26.0839680017488));
#62966=CARTESIAN_POINT('Ctrl Pts',(0.753157416662829,-8.71440146455451,
26.0817096126577));
#62967=CARTESIAN_POINT('Ctrl Pts',(0.832339520725286,-8.7177377122098,26.0803883905589));
#62968=CARTESIAN_POINT('Ctrl Pts',(0.912206730531842,-8.72162325745983,
26.0788521144128));
#62969=CARTESIAN_POINT('Ctrl Pts',(0.992749474308896,-8.72608667555154,
26.0770927025014));
#62970=CARTESIAN_POINT('Ctrl Pts',(1.03302084619742,-8.7283183845974,26.0762129965457));
#62971=CARTESIAN_POINT('Ctrl Pts',(1.07346110157823,-8.73069456314185,26.0752775105416));
#62972=CARTESIAN_POINT('Ctrl Pts',(1.11406896962032,-8.73321881095825,26.0742852517176));
#62973=CARTESIAN_POINT('Ctrl Pts',(1.13437290364137,-8.73448093486644,26.0737891223056));
#62974=CARTESIAN_POINT('Ctrl Pts',(1.1547187408289,-8.73578007617861,26.0732787999421));
#62975=CARTESIAN_POINT('Ctrl Pts',(1.17510631899125,-8.73711668864689,26.0727541609786));
#62976=CARTESIAN_POINT('Ctrl Pts',(1.18530010807242,-8.73778499488104,26.0724918414968));
#62977=CARTESIAN_POINT('Ctrl Pts',(1.19550433239735,-8.73846266890964,26.0722259428812));
#62978=CARTESIAN_POINT('Ctrl Pts',(1.20571897138345,-8.73914976768477,26.0719564497065));
#62979=CARTESIAN_POINT('Ctrl Pts',(1.20976726658234,-8.73942208065406,26.0718496433939));
#62980=CARTESIAN_POINT('Ctrl Pts',(1.21381719763114,-8.73969587397374,26.071742272482));
#62981=CARTESIAN_POINT('Ctrl Pts',(1.21786876323936,-8.73997115120274,26.0716343360093));
#62982=CARTESIAN_POINT('Ctrl Pts',(1.21892864306473,-8.74004316306423,26.0716061000875));
#62983=CARTESIAN_POINT('Ctrl Pts',(1.21998863474838,-8.74011527647456,26.0715778254625));
#62984=CARTESIAN_POINT('Ctrl Pts',(1.22104873826724,-8.7401874914914,26.0715495121158));
#62985=CARTESIAN_POINT('Ctrl Pts',(1.22360500038343,-8.74036162591175,26.0714812392215));
#62986=CARTESIAN_POINT('Ctrl Pts',(1.22616191276806,-8.74053635114404,26.0714127411729));
#62987=CARTESIAN_POINT('Ctrl Pts',(1.2287194750979,-8.74071166796458,26.0713440177222));
#62988=CARTESIAN_POINT('Ctrl Pts',(1.23127703742774,-8.74088698478512,26.0712752942715));
#62989=CARTESIAN_POINT('Ctrl Pts',(1.23521161045926,-8.74115782948028,26.0711691378197));
#62990=CARTESIAN_POINT('Ctrl Pts',(1.23639411159791,-8.74123939403498,26.0711371708931));
#62991=CARTESIAN_POINT('Ctrl Pts',(1.30374576804469,-8.74588506217585,26.0693164323025));
#62992=CARTESIAN_POINT('Ctrl Pts',(1.37824680873525,-8.75142078003761,26.0671523857232));
#62993=CARTESIAN_POINT('Ctrl Pts',(1.45986555292161,-8.75810195128712,26.0645490720026));
#62994=CARTESIAN_POINT('Ctrl Pts',(1.54153671708015,-8.76478741354618,26.0619440862932));
#62995=CARTESIAN_POINT('Ctrl Pts',(1.63033495238198,-8.7726198465256,26.0588991994326));
#62996=CARTESIAN_POINT('Ctrl Pts',(1.72621529430777,-8.78190290107649,26.0553019027112));
#62997=CARTESIAN_POINT('Ctrl Pts',(1.81098051183597,-8.79010979857526,26.0521216299568));
#62998=CARTESIAN_POINT('Ctrl Pts',(1.9012809281609,-8.79945118708362,26.0485093304685));
#62999=CARTESIAN_POINT('Ctrl Pts',(1.99707461557457,-8.81016746024439,26.0443773365715));
#63000=CARTESIAN_POINT('Ctrl Pts',(2.10637322501788,-8.82239450553838,26.0396628172816));
#63001=CARTESIAN_POINT('Ctrl Pts',(2.22282381531433,-8.83641075654679,26.0342718356153));
#63002=CARTESIAN_POINT('Ctrl Pts',(2.34634426221008,-8.85261426659337,26.0280625761146));
#63003=CARTESIAN_POINT('Ctrl Pts',(2.4625641280895,-8.86786008064049,26.0222203101212));
#63004=CARTESIAN_POINT('Ctrl Pts',(2.58504288732567,-8.88504271884099,26.0156534249642));
#63005=CARTESIAN_POINT('Ctrl Pts',(2.71369126659325,-8.90452916042472,26.0082345163188));
#63006=CARTESIAN_POINT('Ctrl Pts',(2.74242434444493,-8.90888137571313,26.0065775340785));
#63007=CARTESIAN_POINT('Ctrl Pts',(2.77146509461616,-8.91334864511851,26.0048780180626));
#63008=CARTESIAN_POINT('Ctrl Pts',(2.80081237645999,-8.91793523390627,26.0031345111935));
#63009=CARTESIAN_POINT('Ctrl Pts',(2.82623497984273,-8.92190844778861,26.0016241674464));
#63010=CARTESIAN_POINT('Ctrl Pts',(2.85468152296542,-8.92641169081457,25.9999134386759));
#63011=CARTESIAN_POINT('Ctrl Pts',(2.88336004684574,-8.93102387982404,25.9981627588254));
#63012=CARTESIAN_POINT('Ctrl Pts',(2.89852589836326,-8.93346290960048,25.9972369597578));
#63013=CARTESIAN_POINT('Ctrl Pts',(2.91375676620661,-8.93593162566564,25.9963002705621));
#63014=CARTESIAN_POINT('Ctrl Pts',(2.92864080883696,-8.93836217409121,25.9953784262594));
#63015=CARTESIAN_POINT('Ctrl Pts',(3.02398869251615,-8.95393238269068,25.9894730478935));
#63016=CARTESIAN_POINT('Ctrl Pts',(3.11236106131741,-8.96910574908508,25.98373320408));
#63017=CARTESIAN_POINT('Ctrl Pts',(3.19380697504853,-8.98358951228705,25.9782657807705));
#63018=CARTESIAN_POINT('Ctrl Pts',(3.25102861306154,-8.9937654022371,25.9744245209313));
#63019=CARTESIAN_POINT('Ctrl Pts',(3.30483132057741,-9.00360193840428,25.9707173021471));
#63020=CARTESIAN_POINT('Ctrl Pts',(3.3552315455841,-9.01301185398277,25.967175534456));
#63021=CARTESIAN_POINT('Ctrl Pts',(3.42777143265541,-9.02655532949947,25.9620779495085));
#63022=CARTESIAN_POINT('Ctrl Pts',(3.49326333427343,-9.03921296686623,25.9573238865908));
#63023=CARTESIAN_POINT('Ctrl Pts',(3.55175248027868,-9.05076599743781,25.9529912121744));
#63024=CARTESIAN_POINT('Ctrl Pts',(3.61052885977499,-9.06237576361814,25.9486372604906));
#63025=CARTESIAN_POINT('Ctrl Pts',(3.66223368766563,-9.07287010118517,25.9447087798008));
#63026=CARTESIAN_POINT('Ctrl Pts',(3.70690581587701,-9.08207595684254,25.9412664733879));
#63027=CARTESIAN_POINT('Ctrl Pts',(3.7518036529799,-9.09132832569636,25.9378067744935));
#63028=CARTESIAN_POINT('Ctrl Pts',(3.7895976665208,-9.09927919185978,25.9348381263405));
#63029=CARTESIAN_POINT('Ctrl Pts',(3.82031812519521,-9.10580154271587,25.9324045714528));
#63030=CARTESIAN_POINT('Ctrl Pts',(3.82672446119443,-9.10716169073748,25.9318970865077));
#63031=CARTESIAN_POINT('Ctrl Pts',(3.83282315114527,-9.10845988334454,25.9314128120963));
#63032=CARTESIAN_POINT('Ctrl Pts',(3.83861441268323,-9.10969523198207,25.9309520546069));
#63033=CARTESIAN_POINT('Ctrl Pts',(3.85088587684816,-9.11231288902232,25.9299757269135));
#63034=CARTESIAN_POINT('Ctrl Pts',(3.86177701482641,-9.11464825921153,25.9291050310371));
#63035=CARTESIAN_POINT('Ctrl Pts',(3.87128958500804,-9.11669424188912,25.9283424094287));
#63036=CARTESIAN_POINT('Ctrl Pts',(3.87604587009886,-9.11771723322791,25.9279610986245));
#63037=CARTESIAN_POINT('Ctrl Pts',(3.88045751324117,-9.11866787784305,25.9276068068093));
#63038=CARTESIAN_POINT('Ctrl Pts',(3.8845246859424,-9.11954549169954,25.9272797680479));
#63039=CARTESIAN_POINT('Ctrl Pts',(3.88655827229301,-9.11998429862778,25.9271162486671));
#63040=CARTESIAN_POINT('Ctrl Pts',(3.88850574103339,-9.12040484787707,25.9269595425791));
#63041=CARTESIAN_POINT('Ctrl Pts',(3.89036711217908,-9.12080705957815,25.9268096771908));
#63042=CARTESIAN_POINT('Ctrl Pts',(3.89129779775192,-9.12100816542869,25.9267347444967));
#63043=CARTESIAN_POINT('Ctrl Pts',(3.8922069589261,-9.12120468689288,25.9266615219794));
#63044=CARTESIAN_POINT('Ctrl Pts',(3.89309459803728,-9.12139661467507,25.926590012827));
#63045=CARTESIAN_POINT('Ctrl Pts',(3.89353841759287,-9.12149257856616,25.9265542582508));
#63046=CARTESIAN_POINT('Ctrl Pts',(3.89397685661728,-9.12158739409787,25.9265189319951));
#63047=CARTESIAN_POINT('Ctrl Pts',(3.89440722718893,-9.1216804777983,25.9264842514026));
#63048=CARTESIAN_POINT('Ctrl Pts',(3.89483759776058,-9.12177356149873,25.92644957081));
#63049=CARTESIAN_POINT('Ctrl Pts',(3.895265294967,-9.12186600409454,25.9264151272914));
#63050=CARTESIAN_POINT('Ctrl Pts',(3.89699038974,-9.12223935851648,25.9262760320526));
#63051=CARTESIAN_POINT('Ctrl Pts',(3.9058558713217,-9.12415807440555,25.9255612039185));
#63052=CARTESIAN_POINT('Ctrl Pts',(3.91470223383361,-9.12607907064862,25.924845712656));
#63053=CARTESIAN_POINT('Ctrl Pts',(3.92352948621133,-9.12800226777178,25.9241295886134));
#63054=CARTESIAN_POINT('Ctrl Pts',(4.08352764301896,-9.1628611323105,25.9111494990041));
#63055=CARTESIAN_POINT('Ctrl Pts',(4.23724642884231,-9.19843930276484,25.8979635305305));
#63056=CARTESIAN_POINT('Ctrl Pts',(4.38474644283691,-9.23428576561917,25.8847437456403));
#63057=CARTESIAN_POINT('Ctrl Pts',(4.40472431506602,-9.23914092485187,25.8829532158209));
#63058=CARTESIAN_POINT('Ctrl Pts',(4.42458812289106,-9.24400107295718,25.8811620300429));
#63059=CARTESIAN_POINT('Ctrl Pts',(4.44433803305825,-9.24886515182633,25.8793705828725));
#63060=CARTESIAN_POINT('Ctrl Pts',(4.59308014861258,-9.28549789471451,25.8658786915283));
#63061=CARTESIAN_POINT('Ctrl Pts',(4.735361183775,-9.32234986748804,25.8523740435749));
#63062=CARTESIAN_POINT('Ctrl Pts',(4.87125703060614,-9.35899576461154,25.8390153114756));
#63063=CARTESIAN_POINT('Ctrl Pts',(4.89542625203067,-9.36551327653359,25.8366394467117));
#63064=CARTESIAN_POINT('Ctrl Pts',(4.91939352613502,-9.37202438504967,25.8342681342935));
#63065=CARTESIAN_POINT('Ctrl Pts',(4.94315930694047,-9.37852684538982,25.8319021865218));
#63066=CARTESIAN_POINT('Ctrl Pts',(5.0799456786358,-9.41595241807781,25.8182847331775));
#63067=CARTESIAN_POINT('Ctrl Pts',(5.21005664561422,-9.45308782973976,25.8048471457304));
#63068=CARTESIAN_POINT('Ctrl Pts',(5.33358032146309,-9.48953465680202,25.7917336133098));
#63069=CARTESIAN_POINT('Ctrl Pts',(5.36978266052729,-9.50021649882182,25.7878902970892));
#63070=CARTESIAN_POINT('Ctrl Pts',(5.40541921763921,-9.51083948984573,25.7840746454648));
#63071=CARTESIAN_POINT('Ctrl Pts',(5.44049229352746,-9.52139432680783,25.7802898776826));
#63072=CARTESIAN_POINT('Ctrl Pts',(5.56339587865327,-9.55838074075091,25.767027239105));
#63073=CARTESIAN_POINT('Ctrl Pts',(5.67937988110502,-9.59452680014436,25.7541459868581));
#63074=CARTESIAN_POINT('Ctrl Pts',(5.78854158574026,-9.62946566961129,25.7417723345422));
#63075=CARTESIAN_POINT('Ctrl Pts',(5.84236905305293,-9.64669397197664,25.7356709057692));
#63076=CARTESIAN_POINT('Ctrl Pts',(5.89453776479577,-9.66362944720222,25.7296924705973));
#63077=CARTESIAN_POINT('Ctrl Pts',(5.94505953414157,-9.68023211648962,25.7238498365264));
#63078=CARTESIAN_POINT('Ctrl Pts',(5.95968624764569,-9.68503880656035,25.7221583174888));
#63079=CARTESIAN_POINT('Ctrl Pts',(5.97417491774219,-9.689817618351,25.7204781719848));
#63080=CARTESIAN_POINT('Ctrl Pts',(5.98852581858683,-9.69456763491412,25.7188097024708));
#63081=CARTESIAN_POINT('Ctrl Pts',(-6.39567216128937,-8.78352116600331,
25.5334667473151));
#63082=CARTESIAN_POINT('Ctrl Pts',(-6.35564926200295,-8.77012417292118,
25.5378747904695));
#63083=CARTESIAN_POINT('Ctrl Pts',(-5.98525108497463,-8.6474022387759,25.5783535630118));
#63084=CARTESIAN_POINT('Ctrl Pts',(-5.25617064763411,-8.42856486724208,
25.6522243920981));
#63085=CARTESIAN_POINT('Ctrl Pts',(-4.1757682916681,-8.16491404339211,25.7436212722339));
#63086=CARTESIAN_POINT('Ctrl Pts',(-3.01937523383598,-7.95089183270233,
25.8195369244464));
#63087=CARTESIAN_POINT('Ctrl Pts',(-1.83578803503655,-7.80507994015202,
25.8725332968182));
#63088=CARTESIAN_POINT('Ctrl Pts',(-0.697918458997622,-7.73463067220822,
25.8989855255588));
#63089=CARTESIAN_POINT('Ctrl Pts',(0.331420580112759,-7.72744138102246,
25.9017875116284));
#63090=CARTESIAN_POINT('Ctrl Pts',(1.24582508159658,-7.76509367288467,25.8874715584761));
#63091=CARTESIAN_POINT('Ctrl Pts',(2.0703196582245,-7.83520521068097,25.8615905206106));
#63092=CARTESIAN_POINT('Ctrl Pts',(2.81708947245881,-7.92875821572134,25.8276627710151));
#63093=CARTESIAN_POINT('Ctrl Pts',(3.49020566169626,-8.0378827718874,25.7886670556739));
#63094=CARTESIAN_POINT('Ctrl Pts',(4.09499065512871,-8.15592645391314,25.7470103559732));
#63095=CARTESIAN_POINT('Ctrl Pts',(4.6500687649082,-8.28093222016087,25.7034061523398));
#63096=CARTESIAN_POINT('Ctrl Pts',(5.18051476211263,-8.41545434309806,25.6570328769038));
#63097=CARTESIAN_POINT('Ctrl Pts',(5.70543165760628,-8.56333660797456,25.6067222305036));
#63098=CARTESIAN_POINT('Ctrl Pts',(6.10978786803773,-8.68891156621066,25.5646816773211));
#63099=CARTESIAN_POINT('Ctrl Pts',(6.34031815825487,-8.76499287475972,25.5395628680216));
#63100=CARTESIAN_POINT('Ctrl Pts',(6.39541677748914,-8.78343677823537,25.5334956641249));
#63101=CARTESIAN_POINT('Ctrl Pts',(-6.33018726788419,-9.06735941059648,
25.7767207816065));
#63102=CARTESIAN_POINT('Ctrl Pts',(-6.29063853345883,-9.05404377495881,
25.7811614548819));
#63103=CARTESIAN_POINT('Ctrl Pts',(-5.92460132235373,-8.93205700834798,
25.8219427981682));
#63104=CARTESIAN_POINT('Ctrl Pts',(-5.20364012968939,-8.71436432674133,
25.8964109697843));
#63105=CARTESIAN_POINT('Ctrl Pts',(-4.13466953168284,-8.4518979752872,25.9886148633439));
#63106=CARTESIAN_POINT('Ctrl Pts',(-2.99013639985378,-8.23872575964737,
26.0652406032874));
#63107=CARTESIAN_POINT('Ctrl Pts',(-1.81835116362302,-8.09343232209409,
26.1187453572149));
#63108=CARTESIAN_POINT('Ctrl Pts',(-0.691521315650298,-8.02320579194545,
26.1454462283406));
#63109=CARTESIAN_POINT('Ctrl Pts',(0.328421662670315,-8.01603646606291,
26.1482731581728));
#63110=CARTESIAN_POINT('Ctrl Pts',(1.2341212032938,-8.05357459156658,26.1338249563432));
#63111=CARTESIAN_POINT('Ctrl Pts',(2.0505435657801,-8.12345060526913,26.1076971639241));
#63112=CARTESIAN_POINT('Ctrl Pts',(2.78985534531287,-8.21666682407695,26.0734453634407));
#63113=CARTESIAN_POINT('Ctrl Pts',(3.45613744599942,-8.32537207799168,26.0340816249332));
#63114=CARTESIAN_POINT('Ctrl Pts',(4.05468755882963,-8.44293303358733,25.9920402440002));
#63115=CARTESIAN_POINT('Ctrl Pts',(4.60395024836123,-8.56739478506552,25.9480446147656));
#63116=CARTESIAN_POINT('Ctrl Pts',(5.12873138731788,-8.70129134259621,25.9012692232388));
#63117=CARTESIAN_POINT('Ctrl Pts',(5.64789963752306,-8.84843173585835,25.8505405843021));
#63118=CARTESIAN_POINT('Ctrl Pts',(6.04766646809667,-8.97331569512675,25.8081692666362));
#63119=CARTESIAN_POINT('Ctrl Pts',(6.2754891998086,-9.04894368857853,25.7828620346657));
#63120=CARTESIAN_POINT('Ctrl Pts',(6.32993458718007,-9.06727543043847,25.7767498760472));
#63121=CARTESIAN_POINT('Ctrl Pts',(-6.21932701877927,-9.42526885393706,
25.8366567723188));
#63122=CARTESIAN_POINT('Ctrl Pts',(-6.18048214170466,-9.4121663308803,25.8411264604673));
#63123=CARTESIAN_POINT('Ctrl Pts',(-5.82094578598021,-9.29212707116419,
25.8821758663682));
#63124=CARTESIAN_POINT('Ctrl Pts',(-5.11256644425228,-9.07783407043934,
25.9571568476127));
#63125=CARTESIAN_POINT('Ctrl Pts',(-4.06220274945981,-8.81944032503722,
26.0500340658684));
#63126=CARTESIAN_POINT('Ctrl Pts',(-2.93773889681033,-8.60958787110744,
26.127238451141));
#63127=CARTESIAN_POINT('Ctrl Pts',(-1.78661058007677,-8.46656410207219,
26.1811448105063));
#63128=CARTESIAN_POINT('Ctrl Pts',(-0.679622419473119,-8.39742515837133,
26.2080312380617));
#63129=CARTESIAN_POINT('Ctrl Pts',(0.322802864782609,-8.39036439860734,
26.2108752950314));
#63130=CARTESIAN_POINT('Ctrl Pts',(1.21266718731651,-8.42732524877291,26.1963309615885));
#63131=CARTESIAN_POINT('Ctrl Pts',(2.01471122069113,-8.49611283173201,26.1700131751107));
#63132=CARTESIAN_POINT('Ctrl Pts',(2.74099430211639,-8.58787416570904,26.1355048218257));
#63133=CARTESIAN_POINT('Ctrl Pts',(3.39556606614342,-8.69488456823181,26.0958439655793));
#63134=CARTESIAN_POINT('Ctrl Pts',(3.98363652396525,-8.81061649534371,26.0534875495589));
#63135=CARTESIAN_POINT('Ctrl Pts',(4.52331543764338,-8.93314488999573,26.0091674680472));
#63136=CARTESIAN_POINT('Ctrl Pts',(5.03895717721903,-9.06496118679828,25.9620547272721));
#63137=CARTESIAN_POINT('Ctrl Pts',(5.54907347998645,-9.20980765316832,25.9109704011966));
#63138=CARTESIAN_POINT('Ctrl Pts',(5.94182258892166,-9.33272612605645,25.8683120901775));
#63139=CARTESIAN_POINT('Ctrl Pts',(6.1656025554792,-9.40714791972507,25.8428381607526));
#63140=CARTESIAN_POINT('Ctrl Pts',(6.21907854257829,-9.42518611321531,25.8366860115496));
#63141=CARTESIAN_POINT('Ctrl Pts',(-6.09477777755571,-9.75501019029731,
25.6963138452313));
#63142=CARTESIAN_POINT('Ctrl Pts',(-6.05666531980665,-9.74219158610546,
25.7008006525782));
#63143=CARTESIAN_POINT('Ctrl Pts',(-5.70391204412257,-9.62475519120128,
25.742007112709));
#63144=CARTESIAN_POINT('Ctrl Pts',(-5.00898154501689,-9.41514444969426,
25.8172700391757));
#63145=CARTESIAN_POINT('Ctrl Pts',(-3.9790819862615,-9.16254640127591,25.9104947771135));
#63146=CARTESIAN_POINT('Ctrl Pts',(-2.87716051673702,-8.95753370316113,
25.98798127695));
#63147=CARTESIAN_POINT('Ctrl Pts',(-1.74963953464299,-8.81788142038787,
26.0420678997381));
#63148=CARTESIAN_POINT('Ctrl Pts',(-0.66562326086846,-8.75038371137221,
26.0690238753989));
#63149=CARTESIAN_POINT('Ctrl Pts',(0.31617042790742,-8.74348905173393,26.0718723597058));
#63150=CARTESIAN_POINT('Ctrl Pts',(1.18759586946167,-8.77957470163612,26.0572954265023));
#63151=CARTESIAN_POINT('Ctrl Pts',(1.97306545476681,-8.84673237888208,26.0308986009111));
#63152=CARTESIAN_POINT('Ctrl Pts',(2.6844732657847,-8.93633699629108,25.9962743802485));
#63153=CARTESIAN_POINT('Ctrl Pts',(3.32580559191093,-9.04086190150178,25.9564720770166));
#63154=CARTESIAN_POINT('Ctrl Pts',(3.90214690596376,-9.15394176510944,25.9139601535985));
#63155=CARTESIAN_POINT('Ctrl Pts',(4.4312128214806,-9.27370054758531,25.8694751653495));
#63156=CARTESIAN_POINT('Ctrl Pts',(4.93685264935617,-9.40257696777726,25.8221860981219));
#63157=CARTESIAN_POINT('Ctrl Pts',(5.43720062470865,-9.54423361014413,25.7709098835103));
#63158=CARTESIAN_POINT('Ctrl Pts',(5.82250913003638,-9.66447427448976,25.7280902474343));
#63159=CARTESIAN_POINT('Ctrl Pts',(6.04206637679057,-9.7372819550532,25.7025189180159));
#63160=CARTESIAN_POINT('Ctrl Pts',(6.09453380570084,-9.75492916631022,25.696343155098));
#63161=CARTESIAN_POINT('',(6.27159454902671,-8.76071457519094,25.5608537658479));
#63162=CARTESIAN_POINT('Origin',(5.999999949031,-9.33250966434584,24.7867247244592));
#63163=CARTESIAN_POINT('Ctrl Pts',(-6.27159387328075,-8.76070928018809,
25.560857166473));
#63164=CARTESIAN_POINT('Ctrl Pts',(-6.1323966152263,-8.71504797181017,25.5759656528077));
#63165=CARTESIAN_POINT('Ctrl Pts',(-5.98564485576888,-8.66855400399287,
25.5914802336782));
#63166=CARTESIAN_POINT('Ctrl Pts',(-5.83132853839285,-8.62173957209145,
25.6072278332491));
#63167=CARTESIAN_POINT('Ctrl Pts',(-5.67907395050422,-8.57555060026016,
25.622765038411));
#63168=CARTESIAN_POINT('Ctrl Pts',(-5.51945529064096,-8.52904980925714,
25.6385292621719));
#63169=CARTESIAN_POINT('Ctrl Pts',(-5.35247220392677,-8.4827683508267,25.6543232525887));
#63170=CARTESIAN_POINT('Ctrl Pts',(-5.32566844713921,-8.47533935319614,
25.6568584690957));
#63171=CARTESIAN_POINT('Ctrl Pts',(-5.2986749639072,-8.4679160874565,25.6593943834507));
#63172=CARTESIAN_POINT('Ctrl Pts',(-5.27149178336552,-8.46050084257278,
25.6619300990734));
#63173=CARTESIAN_POINT('Ctrl Pts',(-5.14595766075532,-8.42625664296592,
25.6736402385623));
#63174=CARTESIAN_POINT('Ctrl Pts',(-5.01637753192559,-8.3921823907687,25.6853467760197));
#63175=CARTESIAN_POINT('Ctrl Pts',(-4.88275736863916,-8.35851823696374,
25.6969639538638));
#63176=CARTESIAN_POINT('Ctrl Pts',(-4.71106402408442,-8.31526195725101,
25.7118912827137));
#63177=CARTESIAN_POINT('Ctrl Pts',(-4.53269542172315,-8.27268029475778,
25.7266725174848));
#63178=CARTESIAN_POINT('Ctrl Pts',(-4.34764537476528,-8.23131615277371,
25.7411116072797));
#63179=CARTESIAN_POINT('Ctrl Pts',(-4.29584306648741,-8.21973680940182,
25.7451536391144));
#63180=CARTESIAN_POINT('Ctrl Pts',(-4.24351727085387,-8.20825312966762,
25.7491687071653));
#63181=CARTESIAN_POINT('Ctrl Pts',(-4.19066810075872,-8.19687761788522,
25.7531521496353));
#63182=CARTESIAN_POINT('Ctrl Pts',(-4.14339042324644,-8.18670134119786,
25.7567156475699));
#63183=CARTESIAN_POINT('Ctrl Pts',(-4.0956939046934,-8.17661163141362,25.7602538330852));
#63184=CARTESIAN_POINT('Ctrl Pts',(-4.047578973713,-8.16661761355435,25.7637634434875));
#63185=CARTESIAN_POINT('Ctrl Pts',(-3.90056245654704,-8.13608061249819,
25.7744871562197));
#63186=CARTESIAN_POINT('Ctrl Pts',(-3.7496359565824,-8.10643536805442,25.7849451020033));
#63187=CARTESIAN_POINT('Ctrl Pts',(-3.59479964942688,-8.0779501732433,25.7950405868657));
#63188=CARTESIAN_POINT('Ctrl Pts',(-3.51738149584912,-8.06370757583774,
25.8000883292969));
#63189=CARTESIAN_POINT('Ctrl Pts',(-3.43898588186198,-8.0497552353687,25.8050453472066));
#63190=CARTESIAN_POINT('Ctrl Pts',(-3.35961278010336,-8.03612820885441,
25.8098988471816));
#63191=CARTESIAN_POINT('Ctrl Pts',(-3.31992622922405,-8.02931469559726,
25.8123255971691));
#63192=CARTESIAN_POINT('Ctrl Pts',(-3.27999530401069,-8.02258252072975,
25.81472645521));
#63193=CARTESIAN_POINT('Ctrl Pts',(-3.23982000049219,-8.01593617299398,
25.8170997788106));
#63194=CARTESIAN_POINT('Ctrl Pts',(-3.21973234873293,-8.01261299912609,
25.8182864406108));
#63195=CARTESIAN_POINT('Ctrl Pts',(-3.1995836022476,-8.00931128268966,25.8194662179862));
#63196=CARTESIAN_POINT('Ctrl Pts',(-3.17937376004829,-8.00603159000866,
25.8206389016039));
#63197=CARTESIAN_POINT('Ctrl Pts',(-3.16169014812389,-8.00316185891278,
25.8216649997694));
#63198=CARTESIAN_POINT('Ctrl Pts',(-3.14395975978476,-8.00030898979315,
25.8226856667284));
#63199=CARTESIAN_POINT('Ctrl Pts',(-3.12618259427586,-7.99747336460349,
25.8237007607655));
#63200=CARTESIAN_POINT('Ctrl Pts',(-3.12364299920317,-7.99706827529068,
25.8238457741994));
#63201=CARTESIAN_POINT('Ctrl Pts',(-3.11986202403536,-7.99646617108508,
25.8240613390158));
#63202=CARTESIAN_POINT('Ctrl Pts',(-3.11856094515192,-7.99625915356409,
25.8241354594592));
#63203=CARTESIAN_POINT('Ctrl Pts',(-3.09161528851505,-7.99197177090832,
25.8256705116704));
#63204=CARTESIAN_POINT('Ctrl Pts',(-3.06344467690482,-7.9875467889361,25.8272569731113));
#63205=CARTESIAN_POINT('Ctrl Pts',(-3.03404913715077,-7.98300009354392,
25.8288891657581));
#63206=CARTESIAN_POINT('Ctrl Pts',(-2.96198356806363,-7.97185349805207,
25.83289061948));
#63207=CARTESIAN_POINT('Ctrl Pts',(-2.88255590909974,-7.95997199195539,
25.8371681774551));
#63208=CARTESIAN_POINT('Ctrl Pts',(-2.79576579462087,-7.9476233532413,25.8416259690135));
#63209=CARTESIAN_POINT('Ctrl Pts',(-2.70930593296023,-7.93532170343557,
25.846066797831));
#63210=CARTESIAN_POINT('Ctrl Pts',(-2.61553929356376,-7.92255647438925,
25.8506865367989));
#63211=CARTESIAN_POINT('Ctrl Pts',(-2.51446660864717,-7.9096408053862,25.8553721684044));
#63212=CARTESIAN_POINT('Ctrl Pts',(-2.50260224764738,-7.90812470675151,
25.8559221886688));
#63213=CARTESIAN_POINT('Ctrl Pts',(-2.49063721965791,-7.9066065901873,25.8564730956623));
#63214=CARTESIAN_POINT('Ctrl Pts',(-2.47857152941463,-7.90508700613539,
25.8570246895332));
#63215=CARTESIAN_POINT('Ctrl Pts',(-2.37688572601341,-7.8922804346058,25.861673347404));
#63216=CARTESIAN_POINT('Ctrl Pts',(-2.26804993547395,-7.87936601620428,
25.8663725584229));
#63217=CARTESIAN_POINT('Ctrl Pts',(-2.15206295112008,-7.8667005243223,25.8709938985986));
#63218=CARTESIAN_POINT('Ctrl Pts',(-2.11969748351752,-7.86316629529255,
25.8722834556689));
#63219=CARTESIAN_POINT('Ctrl Pts',(-2.08677523011003,-7.85965173436756,
25.8735668343966));
#63220=CARTESIAN_POINT('Ctrl Pts',(-2.05329628484806,-7.85616525875198,
25.8748409739275));
#63221=CARTESIAN_POINT('Ctrl Pts',(-1.97656815473855,-7.84817484111597,
25.8777610881349));
#63222=CARTESIAN_POINT('Ctrl Pts',(-1.89691554666913,-7.84033139559416,
25.8806329582618));
#63223=CARTESIAN_POINT('Ctrl Pts',(-1.8143384154204,-7.83274216428475,25.8834176179311));
#63224=CARTESIAN_POINT('Ctrl Pts',(-1.81240217498234,-7.83256421457479,
25.8834829116823));
#63225=CARTESIAN_POINT('Ctrl Pts',(-1.81046432668551,-7.83238640486458,
25.8835481572174));
#63226=CARTESIAN_POINT('Ctrl Pts',(-1.8085248705108,-7.83220873662038,25.8836133540381));
#63227=CARTESIAN_POINT('Ctrl Pts',(-1.76910718840288,-7.82859779121116,
25.884938420098));
#63228=CARTESIAN_POINT('Ctrl Pts',(-1.72902532971431,-7.82504524963275,
25.8862433793847));
#63229=CARTESIAN_POINT('Ctrl Pts',(-1.68827931773378,-7.82156332449908,
25.8875239411442));
#63230=CARTESIAN_POINT('Ctrl Pts',(-1.66690390495163,-7.81973670188275,
25.8881957255686));
#63231=CARTESIAN_POINT('Ctrl Pts',(-1.64534571176604,-7.81792951698791,
25.8888607907406));
#63232=CARTESIAN_POINT('Ctrl Pts',(-1.62360473903617,-7.81614356896003,
25.8895184936256));
#63233=CARTESIAN_POINT('Ctrl Pts',(-1.61273425267123,-7.81525059494608,
25.8898473450681));
#63234=CARTESIAN_POINT('Ctrl Pts',(-1.60181807138526,-7.81436293042739,
25.890174355595));
#63235=CARTESIAN_POINT('Ctrl Pts',(-1.59085619528081,-7.81348080326641,
25.8904994437807));
#63236=CARTESIAN_POINT('Ctrl Pts',(-1.58537525722859,-7.81303973968592,
25.8906619878735));
#63237=CARTESIAN_POINT('Ctrl Pts',(-1.57988289546958,-7.81260006046241,
25.8908240513594));
#63238=CARTESIAN_POINT('Ctrl Pts',(-1.57437911001673,-7.81216179426874,
25.8909856239973));
#63239=CARTESIAN_POINT('Ctrl Pts',(-1.56887532456389,-7.81172352807508,
25.8911471966352));
#63240=CARTESIAN_POINT('Ctrl Pts',(-1.56205959677632,-7.81118421457966,
25.8913460660047));
#63241=CARTESIAN_POINT('Ctrl Pts',(-1.55783348258494,-7.8108512635462,25.8914688590589));
#63242=CARTESIAN_POINT('Ctrl Pts',(-1.33210030446669,-7.79306705527876,
25.8980277131554));
#63243=CARTESIAN_POINT('Ctrl Pts',(-1.11005375162319,-7.77943810586309,
25.9030588947695));
#63244=CARTESIAN_POINT('Ctrl Pts',(-0.891696882492288,-7.76958903507536,
25.9066954247431));
#63245=CARTESIAN_POINT('Ctrl Pts',(-0.848420665378784,-7.76763704461373,
25.9074161497713));
#63246=CARTESIAN_POINT('Ctrl Pts',(-0.805289271297393,-7.7658336506397,
25.9080820807832));
#63247=CARTESIAN_POINT('Ctrl Pts',(-0.76230257197877,-7.76417611439376,
25.9086942333594));
#63248=CARTESIAN_POINT('Ctrl Pts',(-0.724714216543341,-7.76272673441003,
25.9092295107587));
#63249=CARTESIAN_POINT('Ctrl Pts',(-0.687236480829822,-7.76138885372218,
25.9097236478486));
#63250=CARTESIAN_POINT('Ctrl Pts',(-0.649869562680107,-7.76016057469741,
25.9101772242416));
#63251=CARTESIAN_POINT('Ctrl Pts',(-0.558060599569084,-7.75714274424043,
25.9112916425663));
#63252=CARTESIAN_POINT('Ctrl Pts',(-0.466920649099576,-7.75478646686927,
25.912161232118));
#63253=CARTESIAN_POINT('Ctrl Pts',(-0.376448945799055,-7.75306363563768,
25.9127967462999));
#63254=CARTESIAN_POINT('Ctrl Pts',(-0.312801772326068,-7.75185161757831,
25.9132438328464));
#63255=CARTESIAN_POINT('Ctrl Pts',(-0.249485486100613,-7.75095306723222,
25.9135750128796));
#63256=CARTESIAN_POINT('Ctrl Pts',(-0.186500087442505,-7.7503583424659,
25.9137938244159));
#63257=CARTESIAN_POINT('Ctrl Pts',(-0.15500738811345,-7.75006098008275,
25.913903230184));
#63258=CARTESIAN_POINT('Ctrl Pts',(-0.123597410553174,-7.74983957602615,
25.9139845414595));
#63259=CARTESIAN_POINT('Ctrl Pts',(-0.0922701543828133,-7.74969293858145,
25.9140381884101));
#63260=CARTESIAN_POINT('Ctrl Pts',(-0.0647192855148777,-7.74956397774978,
25.914085368415));
#63261=CARTESIAN_POINT('Ctrl Pts',(-0.0383381923124055,-7.74949397676687,
25.9141107439043));
#63262=CARTESIAN_POINT('Ctrl Pts',(-0.0102093864688425,-7.74947894153103,
25.9141157544645));
#63263=CARTESIAN_POINT('Ctrl Pts',(-0.00635378156109146,-7.74947688065687,
25.9141164412601));
#63264=CARTESIAN_POINT('Ctrl Pts',(-0.0024653403777432,-7.74947592698224,
25.9141167172151));
#63265=CARTESIAN_POINT('Ctrl Pts',(0.00146345041170125,-7.74947614296011,
25.9141165584631));
#63266=CARTESIAN_POINT('Ctrl Pts',(0.124001691178138,-7.74948287926902,
25.9141116070182));
#63267=CARTESIAN_POINT('Ctrl Pts',(0.246536534909898,-7.75063935015112,
25.91369518508));
#63268=CARTESIAN_POINT('Ctrl Pts',(0.369073085050784,-7.75293732746282,
25.9128590542009));
#63269=CARTESIAN_POINT('Ctrl Pts',(0.644887810889202,-7.75810979218033,
25.910977026276));
#63270=CARTESIAN_POINT('Ctrl Pts',(0.92071099518736,-7.76906234542254,25.9069696802048));
#63271=CARTESIAN_POINT('Ctrl Pts',(1.1965320497517,-7.78581292554686,25.9008588258509));
#63272=CARTESIAN_POINT('Ctrl Pts',(1.22213119051329,-7.78736755834716,25.900291673278));
#63273=CARTESIAN_POINT('Ctrl Pts',(1.24773031471214,-7.7889721694523,25.8997063896472));
#63274=CARTESIAN_POINT('Ctrl Pts',(1.27332941464932,-7.79062679485959,25.8991029852857));
#63275=CARTESIAN_POINT('Ctrl Pts',(1.37083893333184,-7.79692942766547,25.8968045580361));
#63276=CARTESIAN_POINT('Ctrl Pts',(1.46834810130389,-7.80395767161213,25.8942432317263));
#63277=CARTESIAN_POINT('Ctrl Pts',(1.5658568717593,-7.81170938517129,25.8914183110703));
#63278=CARTESIAN_POINT('Ctrl Pts',(1.74018694254622,-7.82556820799489,25.8863678051966));
#63279=CARTESIAN_POINT('Ctrl Pts',(1.91451739829087,-7.84174034092828,25.8804757772071));
#63280=CARTESIAN_POINT('Ctrl Pts',(2.08884740122651,-7.86022612185766,25.8737415026613));
#63281=CARTESIAN_POINT('Ctrl Pts',(2.1752494959535,-7.86938811444681,25.8704038360667));
#63282=CARTESIAN_POINT('Ctrl Pts',(2.2616514622376,-7.87911855871861,25.8668592399187));
#63283=CARTESIAN_POINT('Ctrl Pts',(2.34805359106619,-7.88941699552813,25.8631079381382));
#63284=CARTESIAN_POINT('Ctrl Pts',(2.47841969135101,-7.90495558310797,25.857447862504));
#63285=CARTESIAN_POINT('Ctrl Pts',(2.60878583075759,-7.92178731750336,25.8513174296772));
#63286=CARTESIAN_POINT('Ctrl Pts',(2.73915198198545,-7.939912050948,25.8447165665306));
#63287=CARTESIAN_POINT('Ctrl Pts',(2.77255377534431,-7.94455588368756,25.8430253248644));
#63288=CARTESIAN_POINT('Ctrl Pts',(2.80595557540632,-7.94928459706181,25.8413031872238));
#63289=CARTESIAN_POINT('Ctrl Pts',(2.8393573637312,-7.95409821372544,25.8395501483932));
#63290=CARTESIAN_POINT('Ctrl Pts',(2.8711386411965,-7.95867829444779,25.8378821594538));
#63291=CARTESIAN_POINT('Ctrl Pts',(2.90291990800943,-7.96333524011162,25.8361861949494));
#63292=CARTESIAN_POINT('Ctrl Pts',(2.93470118017488,-7.96806902124732,25.8344622613891));
#63293=CARTESIAN_POINT('Ctrl Pts',(2.98358847136506,-7.97535072273512,25.8318104341899));
#63294=CARTESIAN_POINT('Ctrl Pts',(3.03247575908502,-7.98281424431422,25.8290924421403));
#63295=CARTESIAN_POINT('Ctrl Pts',(3.08136304923064,-7.99045953912554,25.8263083281147));
#63296=CARTESIAN_POINT('Ctrl Pts',(3.09765881261251,-7.99300797072931,25.8253802901061));
#63297=CARTESIAN_POINT('Ctrl Pts',(3.11203760285011,-7.99527205976141,25.8245558044054));
#63298=CARTESIAN_POINT('Ctrl Pts',(3.13025034020354,-7.99816542434384,25.8235021736296));
#63299=CARTESIAN_POINT('Ctrl Pts',(3.25878004893528,-8.01858428285028,25.8160665611734));
#63300=CARTESIAN_POINT('Ctrl Pts',(3.38588994776671,-8.04008769017049,25.808299088878));
#63301=CARTESIAN_POINT('Ctrl Pts',(3.5115662710351,-8.0625905343887,25.8002296274968));
#63302=CARTESIAN_POINT('Ctrl Pts',(3.71382498700818,-8.09880575981026,25.7872429418976));
#63303=CARTESIAN_POINT('Ctrl Pts',(3.91236990026725,-8.13760860679937,25.773474678434));
#63304=CARTESIAN_POINT('Ctrl Pts',(4.10716724986624,-8.17865262650198,25.7590464903351));
#63305=CARTESIAN_POINT('Ctrl Pts',(4.29251707950218,-8.21770604316864,25.7453180581382));
#63306=CARTESIAN_POINT('Ctrl Pts',(4.47447431949519,-8.25878866878335,25.7309921243262));
#63307=CARTESIAN_POINT('Ctrl Pts',(4.65302915034081,-8.30161628112533,25.7161694333478));
#63308=CARTESIAN_POINT('Ctrl Pts',(4.83066811792946,-8.34422421732446,25.7014227725612));
#63309=CARTESIAN_POINT('Ctrl Pts',(5.00493963976845,-8.38855938233988,25.6861844892871));
#63310=CARTESIAN_POINT('Ctrl Pts',(5.17584967464822,-8.43435907663826,25.6705507275121));
#63311=CARTESIAN_POINT('Ctrl Pts',(5.35322086172,-8.48189020113277,25.6543259406738));
#63312=CARTESIAN_POINT('Ctrl Pts',(5.52697168029971,-8.53099876652162,25.6376753760724));
#63313=CARTESIAN_POINT('Ctrl Pts',(5.69712367345923,-8.58141411828093,25.6207040708845));
#63314=CARTESIAN_POINT('Ctrl Pts',(5.87745455215751,-8.63484543291804,25.6027175029908));
#63315=CARTESIAN_POINT('Ctrl Pts',(6.0537431675926,-8.68974474910015,25.584371006453));
#63316=CARTESIAN_POINT('Ctrl Pts',(6.22602835761291,-8.74582172598816,25.565788475961));
#63317=CARTESIAN_POINT('Ctrl Pts',(6.24124881340971,-8.75077582069497,25.5641468108595));
#63318=CARTESIAN_POINT('Ctrl Pts',(6.25643802960122,-8.75573911480345,25.5625032922101));
#63319=CARTESIAN_POINT('Ctrl Pts',(6.27159604049145,-8.76071143385986,25.5608580131143));
#63320=CARTESIAN_POINT('Origin',(5.999999999061,-9.33250979146063,24.7867247845918));
#63321=CARTESIAN_POINT('Origin',(5.9999696860333,-9.33251391797614,24.7866936474829));
#63322=CARTESIAN_POINT('Ctrl Pts',(6.25606545383873,-3.90351699726741,15.8245348638446));
#63323=CARTESIAN_POINT('Ctrl Pts',(6.27805137190582,-3.90938776964027,15.8167706309341));
#63324=CARTESIAN_POINT('Ctrl Pts',(6.38303596649425,-3.94105812481732,15.7785558941617));
#63325=CARTESIAN_POINT('Ctrl Pts',(6.5644009396555,-4.02787637947969,15.7024427068931));
#63326=CARTESIAN_POINT('Ctrl Pts',(6.77569464165061,-4.20161916671313,15.5905393483866));
#63327=CARTESIAN_POINT('Ctrl Pts',(6.94551705571754,-4.42824393788803,15.4722330995486));
#63328=CARTESIAN_POINT('Ctrl Pts',(7.06116197196841,-4.69652825400431,15.3539457728218));
#63329=CARTESIAN_POINT('Ctrl Pts',(7.10123737675459,-4.92249133588564,15.2686302662615));
#63330=CARTESIAN_POINT('Ctrl Pts',(7.10450937548937,-5.05228130021626,15.2245558649972));
#63331=CARTESIAN_POINT('Ctrl Pts',(7.10419841572891,-5.08306982967337,15.214375952807));
#63332=CARTESIAN_POINT('Ctrl Pts',(6.05790170975049,-3.86072516060592,15.2131216290605));
#63333=CARTESIAN_POINT('Ctrl Pts',(6.0774019058006,-3.86578803164919,15.2062195803066));
#63334=CARTESIAN_POINT('Ctrl Pts',(6.17060154414674,-3.89313992573329,15.1722159993409));
#63335=CARTESIAN_POINT('Ctrl Pts',(6.33230417363677,-3.96853916358796,15.1042106702778));
#63336=CARTESIAN_POINT('Ctrl Pts',(6.52172609417125,-4.12063635096875,15.0038198058236));
#63337=CARTESIAN_POINT('Ctrl Pts',(6.67461078702923,-4.3201963578824,14.8975475181414));
#63338=CARTESIAN_POINT('Ctrl Pts',(6.77898374399282,-4.55736055760934,14.7914865810048));
#63339=CARTESIAN_POINT('Ctrl Pts',(6.81513903772793,-4.75736053874658,14.7154446390863));
#63340=CARTESIAN_POINT('Ctrl Pts',(6.81807628979981,-4.87201821631841,14.6764666609063));
#63341=CARTESIAN_POINT('Ctrl Pts',(6.81779568545588,-4.89919678109847,14.6674846276254));
#63342=CARTESIAN_POINT('Ctrl Pts',(6.04883558612803,-3.36577005918539,14.8011311726366));
#63343=CARTESIAN_POINT('Ctrl Pts',(6.07566935314429,-3.37269321401156,14.7918321486262));
#63344=CARTESIAN_POINT('Ctrl Pts',(6.20353926856132,-3.40998966365746,14.7462158572278));
#63345=CARTESIAN_POINT('Ctrl Pts',(6.42226858523589,-3.51153022966031,14.6566846143631));
#63346=CARTESIAN_POINT('Ctrl Pts',(6.67386632509817,-3.71204279852219,14.5274200429916));
#63347=CARTESIAN_POINT('Ctrl Pts',(6.87408391635468,-3.97082561139319,14.3925000997621));
#63348=CARTESIAN_POINT('Ctrl Pts',(7.0096100495298,-4.27508245854162,14.2585887417136));
#63349=CARTESIAN_POINT('Ctrl Pts',(7.05661851482608,-4.53102183000274,14.1620489883948));
#63350=CARTESIAN_POINT('Ctrl Pts',(7.06050233450235,-4.67877914994309,14.1118773452502));
#63351=CARTESIAN_POINT('Ctrl Pts',(7.06013777230322,-4.71389394697659,14.1002657353677));
#63352=CARTESIAN_POINT('Ctrl Pts',(6.23484754158759,-2.75271794669507,14.8662289006106));
#63353=CARTESIAN_POINT('Ctrl Pts',(6.27388224199307,-2.76291330524427,14.8528923137333));
#63354=CARTESIAN_POINT('Ctrl Pts',(6.45946683867096,-2.81770168594271,14.7876810214237));
#63355=CARTESIAN_POINT('Ctrl Pts',(6.77340486060312,-2.96529042143721,14.6615258505952));
#63356=CARTESIAN_POINT('Ctrl Pts',(7.12924177467691,-3.2515836066926,14.4824993052424));
#63357=CARTESIAN_POINT('Ctrl Pts',(7.40910112429138,-3.61588219559613,14.2975958045458));
#63358=CARTESIAN_POINT('Ctrl Pts',(7.59716915501324,-4.04013483631764,14.1145649290726));
#63359=CARTESIAN_POINT('Ctrl Pts',(7.66247539438356,-4.39613857922254,13.9815985925293));
#63360=CARTESIAN_POINT('Ctrl Pts',(7.66794792454828,-4.60287447369357,13.9115025369606));
#63361=CARTESIAN_POINT('Ctrl Pts',(7.66744178437245,-4.65211218126055,13.8952097092579));
#63362=CARTESIAN_POINT('',(6.999992922344,-4.92966736222272,14.7967908129515));
#63363=CARTESIAN_POINT('',(6.99999949429353,-3.16610543777311,14.5427473811435));
#63364=CARTESIAN_POINT('Ctrl Pts',(7.,-4.92966736222272,14.7967908129515));
#63365=CARTESIAN_POINT('Ctrl Pts',(7.,-4.82678420804455,14.7560363096686));
#63366=CARTESIAN_POINT('Ctrl Pts',(7.,-4.7336540376644,14.7215027168286));
#63367=CARTESIAN_POINT('Ctrl Pts',(7.,-4.65186515615285,14.6935521165994));
#63368=CARTESIAN_POINT('Ctrl Pts',(7.,-4.61097071539707,14.6795768164848));
#63369=CARTESIAN_POINT('Ctrl Pts',(7.,-4.5729198001806,14.6672023399456));
#63370=CARTESIAN_POINT('Ctrl Pts',(7.,-4.53794478179076,14.6562662959784));
#63371=CARTESIAN_POINT('Ctrl Pts',(7.,-4.52045727259585,14.6507982739948));
#63372=CARTESIAN_POINT('Ctrl Pts',(7.,-4.50373880126536,14.6456882660439));
#63373=CARTESIAN_POINT('Ctrl Pts',(7.,-4.48781746868666,14.6409089126752));
#63374=CARTESIAN_POINT('Ctrl Pts',(7.,-4.4798568023973,14.6385192359908));
#63375=CARTESIAN_POINT('Ctrl Pts',(7.,-4.4720954207959,14.636212222952));
#63376=CARTESIAN_POINT('Ctrl Pts',(7.,-4.46453666087317,14.6339841494894));
#63377=CARTESIAN_POINT('Ctrl Pts',(7.,-4.46075728091181,14.6328701127582));
#63378=CARTESIAN_POINT('Ctrl Pts',(7.,-4.45702855637012,14.631775810921));
#63379=CARTESIAN_POINT('Ctrl Pts',(7.,-4.4533508950384,14.6307007794326));
#63380=CARTESIAN_POINT('Ctrl Pts',(7.,-4.44967323370668,14.6296257479442));
#63381=CARTESIAN_POINT('Ctrl Pts',(7.,-4.44764784207163,14.6290344140039));
#63382=CARTESIAN_POINT('Ctrl Pts',(7.,-4.44247150462448,14.6275330288263));
#63383=CARTESIAN_POINT('Ctrl Pts',(7.,-4.35965010547007,14.603510865984));
#63384=CARTESIAN_POINT('Ctrl Pts',(7.,-4.27939235138988,14.583009037268));
#63385=CARTESIAN_POINT('Ctrl Pts',(7.,-4.20230683567458,14.5661068011664));
#63386=CARTESIAN_POINT('Ctrl Pts',(7.,-4.12522131995927,14.5492045650647));
#63387=CARTESIAN_POINT('Ctrl Pts',(7.,-4.05295459894647,14.5361280509262));
#63388=CARTESIAN_POINT('Ctrl Pts',(7.,-3.98140820749628,14.5256481770255));
#63389=CARTESIAN_POINT('Ctrl Pts',(7.,-3.8383154245959,14.5046884292241));
#63390=CARTESIAN_POINT('Ctrl Pts',(7.,-3.69579585817385,14.4945162284038));
#63391=CARTESIAN_POINT('Ctrl Pts',(7.,-3.55814223775101,14.4974061202244));
#63392=CARTESIAN_POINT('Ctrl Pts',(7.,-3.42048861732817,14.500296012045));
#63393=CARTESIAN_POINT('Ctrl Pts',(7.,-3.28795185895767,14.516219567648));
#63394=CARTESIAN_POINT('Ctrl Pts',(7.,-3.16610527255026,14.542746622232));
#63395=CARTESIAN_POINT('',(6.25003741340704,-2.76548799388388,14.8593558170211));
#63396=CARTESIAN_POINT('Ctrl Pts',(6.25007095100041,-2.7654967482904,14.8593452070851));
#63397=CARTESIAN_POINT('Ctrl Pts',(6.33587163725197,-2.78878256441424,14.8297752073987));
#63398=CARTESIAN_POINT('Ctrl Pts',(6.41875467614383,-2.81766749093033,14.7993819051698));
#63399=CARTESIAN_POINT('Ctrl Pts',(6.49900053547044,-2.85195696894397,14.7681022183498));
#63400=CARTESIAN_POINT('Ctrl Pts',(6.50620156545211,-2.85503400695321,14.7652952702469));
#63401=CARTESIAN_POINT('Ctrl Pts',(6.51338135583404,-2.85815456038784,14.7624811504726));
#63402=CARTESIAN_POINT('Ctrl Pts',(6.52054010747125,-2.86131848501783,14.7596597937132));
#63403=CARTESIAN_POINT('Ctrl Pts',(6.60751266789611,-2.89975739727608,14.7253827809508));
#63404=CARTESIAN_POINT('Ctrl Pts',(6.6913787906444,-2.94459799689971,14.6900381286337));
#63405=CARTESIAN_POINT('Ctrl Pts',(6.77140018943003,-2.99541632456422,14.6538748180838));
#63406=CARTESIAN_POINT('Ctrl Pts',(6.84311703907017,-3.04096077166697,14.6214645035361));
#63407=CARTESIAN_POINT('Ctrl Pts',(6.91174725714638,-3.09130726141184,14.5884002469452));
#63408=CARTESIAN_POINT('Ctrl Pts',(6.97733631082931,-3.14667082030927,14.5545423490562));
#63409=CARTESIAN_POINT('Ctrl Pts',(6.984931283593,-3.15308171813926,14.5506217281924));
#63410=CARTESIAN_POINT('Ctrl Pts',(6.99248547643967,-3.15955987192872,14.5466904104436));
#63411=CARTESIAN_POINT('Ctrl Pts',(6.9999989586745,-3.16610560191081,14.5427481350708));
#63412=CARTESIAN_POINT('',(6.26385797816486,-3.90573660195549,15.8144409703668));
#63413=CARTESIAN_POINT('Origin',(6.527982188659,-2.94130808174632,15.8037261610702));
#63414=CARTESIAN_POINT('Ctrl Pts',(6.2638990751077,-3.90574413173893,15.8144151702401));
#63415=CARTESIAN_POINT('Ctrl Pts',(6.2809593183397,-3.91053019376344,15.803450612777));
#63416=CARTESIAN_POINT('Ctrl Pts',(6.29796648298088,-3.91580576242035,15.7922459989039));
#63417=CARTESIAN_POINT('Ctrl Pts',(6.31489097527796,-3.92157938126428,15.7808042255943));
#63418=CARTESIAN_POINT('Ctrl Pts',(6.35719245850541,-3.93601010310817,15.752206382111));
#63419=CARTESIAN_POINT('Ctrl Pts',(6.39898060511237,-3.95355296513967,15.7221256451606));
#63420=CARTESIAN_POINT('Ctrl Pts',(6.43981311987819,-3.97422893257098,15.6906354985908));
#63421=CARTESIAN_POINT('Ctrl Pts',(6.46987737873425,-3.98945228191695,15.6674498602994));
#63422=CARTESIAN_POINT('Ctrl Pts',(6.49942273048966,-4.00637382707713,15.64350052591));
#63423=CARTESIAN_POINT('Ctrl Pts',(6.52825572691364,-4.02500083391913,15.6188233092075));
#63424=CARTESIAN_POINT('Ctrl Pts',(6.53601349370777,-4.0300125910403,15.6121836908519));
#63425=CARTESIAN_POINT('Ctrl Pts',(6.54371960345473,-4.03514781599872,15.6054914107273));
#63426=CARTESIAN_POINT('Ctrl Pts',(6.55137068364015,-4.04040583335116,15.5987473160714));
#63427=CARTESIAN_POINT('Ctrl Pts',(6.58876385834978,-4.06610337627599,15.5657868577292));
#63428=CARTESIAN_POINT('Ctrl Pts',(6.6248461275891,-4.09473439723206,15.5315871554488));
#63429=CARTESIAN_POINT('Ctrl Pts',(6.65919837855307,-4.12621552301973,15.4962590980255));
#63430=CARTESIAN_POINT('Ctrl Pts',(6.67729063309629,-4.14279564586684,15.4776529167861));
#63431=CARTESIAN_POINT('Ctrl Pts',(6.6949022981319,-4.16016622314613,15.458734086895));
#63432=CARTESIAN_POINT('Ctrl Pts',(6.71196671988954,-4.1783148174862,15.4395211563086));
#63433=CARTESIAN_POINT('Ctrl Pts',(6.72110227292727,-4.18803078961281,15.4292353846091));
#63434=CARTESIAN_POINT('Ctrl Pts',(6.7300809057676,-4.19796975487159,15.4188653497671));
#63435=CARTESIAN_POINT('Ctrl Pts',(6.73889398719123,-4.20812767161503,15.4084142443932));
#63436=CARTESIAN_POINT('Ctrl Pts',(6.74831600968466,-4.21898745100916,15.39724101846));
#63437=CARTESIAN_POINT('Ctrl Pts',(6.75754881892868,-4.23009748370278,15.3859751293313));
#63438=CARTESIAN_POINT('Ctrl Pts',(6.76658149289953,-4.24145275839218,15.374620672648));
#63439=CARTESIAN_POINT('Ctrl Pts',(6.77109782988495,-4.24713039573687,15.3689434443064));
#63440=CARTESIAN_POINT('Ctrl Pts',(6.77556412974877,-4.25286934629214,15.363244074211));
#63441=CARTESIAN_POINT('Ctrl Pts',(6.77997898367324,-4.25866897270543,15.3575230980767));
#63442=CARTESIAN_POINT('Ctrl Pts',(6.7826892751254,-4.26222937994938,15.354010974464));
#63443=CARTESIAN_POINT('Ctrl Pts',(6.78572125911814,-4.26626855845317,15.3500426898254));
#63444=CARTESIAN_POINT('Ctrl Pts',(6.78844385144841,-4.26994887684661,15.346443289757));
#63445=CARTESIAN_POINT('Ctrl Pts',(6.79015615021608,-4.2722635108003,15.3441795471346));
#63446=CARTESIAN_POINT('Ctrl Pts',(6.79174708784231,-4.27443533134104,15.3420617997071));
#63447=CARTESIAN_POINT('Ctrl Pts',(6.79306778194254,-4.27624925256168,15.3402958895932));
#63448=CARTESIAN_POINT('Ctrl Pts',(6.8107996753019,-4.30060330823675,15.3165864402844));
#63449=CARTESIAN_POINT('Ctrl Pts',(6.82812764703875,-4.3266456655919,15.2918342165974));
#63450=CARTESIAN_POINT('Ctrl Pts',(6.84476100521714,-4.35446256236332,15.2660735832892));
#63451=CARTESIAN_POINT('Ctrl Pts',(6.84876408758397,-4.36115714127947,15.2598738769011));
#63452=CARTESIAN_POINT('Ctrl Pts',(6.85272673262482,-4.3679544288046,15.2536158504336));
#63453=CARTESIAN_POINT('Ctrl Pts',(6.85664448175611,-4.37485548642977,15.2473001551339));
#63454=CARTESIAN_POINT('Ctrl Pts',(6.87220142998755,-4.40225882253399,15.2222212280432));
#63455=CARTESIAN_POINT('Ctrl Pts',(6.88705311840915,-4.43130038235405,15.1962313701704));
#63456=CARTESIAN_POINT('Ctrl Pts',(6.90092818336887,-4.46200529431339,15.1693865861704));
#63457=CARTESIAN_POINT('Ctrl Pts',(6.91385297148164,-4.49060728516875,15.1443803504418));
#63458=CARTESIAN_POINT('Ctrl Pts',(6.92593042278619,-4.52065243222546,15.1186323058424));
#63459=CARTESIAN_POINT('Ctrl Pts',(6.93691038409135,-4.55214103784724,15.0922053172018));
#63460=CARTESIAN_POINT('Ctrl Pts',(6.94301470875026,-4.56964717165131,15.0775131963522));
#63461=CARTESIAN_POINT('Ctrl Pts',(6.94877927141611,-4.58759914596029,15.0626115450918));
#63462=CARTESIAN_POINT('Ctrl Pts',(6.95415625565575,-4.60599427316238,15.0475137604011));
#63463=CARTESIAN_POINT('Ctrl Pts',(6.96384063454289,-4.63912536924945,15.0203214420337));
#63464=CARTESIAN_POINT('Ctrl Pts',(6.97226953626585,-4.67369588112642,14.9924914495598));
#63465=CARTESIAN_POINT('Ctrl Pts',(6.9791776980466,-4.70964222664831,14.96412246903));
#63466=CARTESIAN_POINT('Ctrl Pts',(6.98573847263594,-4.74378095671348,14.9371800648866));
#63467=CARTESIAN_POINT('Ctrl Pts',(6.99092794841612,-4.77916047790126,14.9097514970841));
#63468=CARTESIAN_POINT('Ctrl Pts',(6.99448542380503,-4.81570149995584,14.8819428905447));
#63469=CARTESIAN_POINT('Ctrl Pts',(6.99588982850059,-4.83012700606452,14.8709647295368));
#63470=CARTESIAN_POINT('Ctrl Pts',(6.99703948106122,-4.84473325899142,14.8599275875814));
#63471=CARTESIAN_POINT('Ctrl Pts',(6.99791659494413,-4.85951430546009,14.8488390072659));
#63472=CARTESIAN_POINT('Ctrl Pts',(6.99928002608722,-4.88249072787875,14.8316023450382));
#63473=CARTESIAN_POINT('Ctrl Pts',(6.99998508666163,-4.90588992273367,14.8142411383093));
#63474=CARTESIAN_POINT('Ctrl Pts',(6.99997879767476,-4.9296673590521,14.7967908137217));
#63475=CARTESIAN_POINT('Ctrl Pts',(6.99990231887239,-4.95610622131399,14.6847031539405));
#63476=CARTESIAN_POINT('Ctrl Pts',(6.99990231887239,-4.91841584418849,15.0109950436589));
#63477=CARTESIAN_POINT('Ctrl Pts',(6.99990231887239,-4.85614473463976,15.898877282419));
#63478=CARTESIAN_POINT('Ctrl Pts',(6.99990231887239,-4.92998658103204,17.3517289669861));
#63479=CARTESIAN_POINT('Ctrl Pts',(6.99990231887239,-5.27368488295105,19.005709054627));
#63480=CARTESIAN_POINT('Ctrl Pts',(6.99990231887239,-5.86659897824408,20.5902694345695));
#63481=CARTESIAN_POINT('Ctrl Pts',(6.99990231887239,-6.69608062393941,22.0651427870248));
#63482=CARTESIAN_POINT('Ctrl Pts',(6.99990231887239,-7.73956505901654,23.3944794780462));
#63483=CARTESIAN_POINT('Ctrl Pts',(6.99990231887239,-8.69529347682775,24.2870566144972));
#63484=CARTESIAN_POINT('Ctrl Pts',(6.99990231887239,-9.28610929960213,24.7366528371348));
#63485=CARTESIAN_POINT('Ctrl Pts',(6.99990231887239,-9.4330769651433,24.8428619308663));
#63486=CARTESIAN_POINT('Ctrl Pts',(7.00659605346157,-4.4803994227663,14.6297385385056));
#63487=CARTESIAN_POINT('Ctrl Pts',(7.00659605346157,-4.44105701581783,14.9703190744433));
#63488=CARTESIAN_POINT('Ctrl Pts',(7.00659605346157,-4.37608979545098,15.8968441454591));
#63489=CARTESIAN_POINT('Ctrl Pts',(7.00659605346157,-4.45313232990638,17.4128498125714));
#63490=CARTESIAN_POINT('Ctrl Pts',(7.00659605346157,-4.8118677809658,19.1393645192062));
#63491=CARTESIAN_POINT('Ctrl Pts',(7.00659605346157,-5.43067059711262,20.792955990879));
#63492=CARTESIAN_POINT('Ctrl Pts',(7.00659605346157,-6.29622676552029,22.3320796939897));
#63493=CARTESIAN_POINT('Ctrl Pts',(7.00659605346157,-7.38549375785552,23.7196853446899));
#63494=CARTESIAN_POINT('Ctrl Pts',(7.00659605346157,-8.38271691158709,24.6510011090022));
#63495=CARTESIAN_POINT('Ctrl Pts',(7.00659605346157,-8.99921657562843,25.1201522854231));
#63496=CARTESIAN_POINT('Ctrl Pts',(7.00659605346157,-9.15258727145085,25.2309895948636));
#63497=CARTESIAN_POINT('Ctrl Pts',(6.71662481110376,-4.10164945528999,14.5859766112628));
#63498=CARTESIAN_POINT('Ctrl Pts',(6.71662481110376,-4.06099172923174,14.9379335334627));
#63499=CARTESIAN_POINT('Ctrl Pts',(6.71662481110376,-3.99387790955452,15.8952253950789));
#63500=CARTESIAN_POINT('Ctrl Pts',(6.71662481110376,-4.07346877946317,17.4615132295016));
#63501=CARTESIAN_POINT('Ctrl Pts',(6.71662481110376,-4.4441765625702,19.2457788126714));
#63502=CARTESIAN_POINT('Ctrl Pts',(6.71662481110376,-5.08359155456183,20.9543317098043));
#63503=CARTESIAN_POINT('Ctrl Pts',(6.71662481110376,-5.97786966754659,22.5446104905642));
#63504=CARTESIAN_POINT('Ctrl Pts',(6.71662481110376,-7.10358798268114,23.9786089333139));
#63505=CARTESIAN_POINT('Ctrl Pts',(6.71662481110376,-8.13384856604163,24.9407677591288));
#63506=CARTESIAN_POINT('Ctrl Pts',(6.71662481110376,-8.77079728415514,25.4254882697159));
#63507=CARTESIAN_POINT('Ctrl Pts',(6.71662481110376,-8.9292659678921,25.5400104887542));
#63508=CARTESIAN_POINT('Ctrl Pts',(6.2531283899648,-3.98117651752108,14.5720568003314));
#63509=CARTESIAN_POINT('Ctrl Pts',(6.2531283899648,-3.94010041424707,14.9276323279248));
#63510=CARTESIAN_POINT('Ctrl Pts',(6.2531283899648,-3.87230380342307,15.8947105023297));
#63511=CARTESIAN_POINT('Ctrl Pts',(6.2531283899648,-3.95270524886919,17.4769921081946));
#63512=CARTESIAN_POINT('Ctrl Pts',(6.2531283899648,-4.3272211960331,19.2796271127503));
#63513=CARTESIAN_POINT('Ctrl Pts',(6.2531283899648,-4.97319251697744,21.0056621615854));
#63514=CARTESIAN_POINT('Ctrl Pts',(6.2531283899648,-5.8766065173295,22.6122123694565));
#63515=CARTESIAN_POINT('Ctrl Pts',(6.2531283899648,-7.01391928347156,24.060967449636));
#63516=CARTESIAN_POINT('Ctrl Pts',(6.2531283899648,-8.05468842536693,25.0329368485149));
#63517=CARTESIAN_POINT('Ctrl Pts',(6.2531283899648,-8.69814158659636,25.5226096590011));
#63518=CARTESIAN_POINT('Ctrl Pts',(6.2531283899648,-8.85823184032323,25.6383039755253));
#63519=CARTESIAN_POINT('Ctrl Pts',(6.99999999975185,-4.9296673620658,14.796790812935));
#63520=CARTESIAN_POINT('Ctrl Pts',(6.99999999975348,-4.91224345485887,14.9628120759864));
#63521=CARTESIAN_POINT('Ctrl Pts',(6.99999999939381,-4.89864382295723,15.1287094595423));
#63522=CARTESIAN_POINT('Ctrl Pts',(6.99999999871008,-4.88880665235693,15.2945618318709));
#63523=CARTESIAN_POINT('Ctrl Pts',(6.99999999819781,-4.8814362670729,15.4188247865357));
#63524=CARTESIAN_POINT('Ctrl Pts',(6.99999999754847,-4.87617905224362,15.5430627452601));
#63525=CARTESIAN_POINT('Ctrl Pts',(6.99999999746782,-4.87302807566252,15.6673106186318));
#63526=CARTESIAN_POINT('Ctrl Pts',(6.99999999735979,-4.86880791455303,15.8337180893462));
#63527=CARTESIAN_POINT('Ctrl Pts',(6.9999999991915,-4.86836396390667,16.0001436878221));
#63528=CARTESIAN_POINT('Ctrl Pts',(6.99999999987961,-4.87172632728565,16.1667041269997));
#63529=CARTESIAN_POINT('Ctrl Pts',(6.99999999995425,-4.87209105600973,16.1847715901549));
#63530=CARTESIAN_POINT('Ctrl Pts',(7.00000000000036,-4.87250062239559,16.2028406354215));
#63531=CARTESIAN_POINT('Ctrl Pts',(7.00000000000036,-4.87295510160001,16.2209114079065));
#63532=CARTESIAN_POINT('Ctrl Pts',(7.00000000000036,-4.87820855291204,16.4297964844935));
#63533=CARTESIAN_POINT('Ctrl Pts',(6.99999999546741,-4.88938134704181,16.6388913171613));
#63534=CARTESIAN_POINT('Ctrl Pts',(6.99999999503646,-4.90651884891385,16.8476332056095));
#63535=CARTESIAN_POINT('Ctrl Pts',(6.99999999469247,-4.92019849279632,17.0142569480107));
#63536=CARTESIAN_POINT('Ctrl Pts',(6.99999999635954,-4.93767767490601,17.1806555717337));
#63537=CARTESIAN_POINT('Ctrl Pts',(6.99999999805387,-4.95895561846968,17.3465427176031));
#63538=CARTESIAN_POINT('Ctrl Pts',(6.99999999906433,-4.97164527214146,17.4454738207608));
#63539=CARTESIAN_POINT('Ctrl Pts',(7.00000000000036,-4.98568560133477,17.5442230216286));
#63540=CARTESIAN_POINT('Ctrl Pts',(7.00000000000036,-5.00106284847129,17.642730538889));
#63541=CARTESIAN_POINT('Ctrl Pts',(7.00000000000036,-5.04223781721342,17.9064997238446));
#63542=CARTESIAN_POINT('Ctrl Pts',(6.99999999769855,-5.09308746630109,18.1685325852661));
#63543=CARTESIAN_POINT('Ctrl Pts',(6.99999999858985,-5.15338945476548,18.4283220865757));
#63544=CARTESIAN_POINT('Ctrl Pts',(6.99999999924453,-5.19768253375072,18.6191429399849));
#63545=CARTESIAN_POINT('Ctrl Pts',(6.99999999995143,-5.24707642416826,18.8087537576797));
#63546=CARTESIAN_POINT('Ctrl Pts',(6.999999999996,-5.30150085813403,18.9969550513234));
#63547=CARTESIAN_POINT('Ctrl Pts',(6.99999999999901,-5.30518090424346,19.0096807590248));
#63548=CARTESIAN_POINT('Ctrl Pts',(7.00000000000036,-5.30888395639083,19.0224000221251));
#63549=CARTESIAN_POINT('Ctrl Pts',(7.00000000000036,-5.31260999009508,19.0351127794273));
#63550=CARTESIAN_POINT('Ctrl Pts',(7.00000000000036,-5.41493715266357,19.3842401589443));
#63551=CARTESIAN_POINT('Ctrl Pts',(6.99999999999506,-5.53457243760421,19.7284577210467));
#63552=CARTESIAN_POINT('Ctrl Pts',(6.99999999997255,-5.67103026820396,20.0659276985029));
#63553=CARTESIAN_POINT('Ctrl Pts',(6.99999999996562,-5.71306956633135,20.1698938903218));
#63554=CARTESIAN_POINT('Ctrl Pts',(7.00000000000035,-5.75670516944874,20.2732194901111));
#63555=CARTESIAN_POINT('Ctrl Pts',(7.00000000000035,-5.80192197421819,20.3758503481523));
#63556=CARTESIAN_POINT('Ctrl Pts',(7.00000000000035,-5.83171073986062,20.4434634091251));
#63557=CARTESIAN_POINT('Ctrl Pts',(6.99999999997079,-5.86218350081567,20.510776266759));
#63558=CARTESIAN_POINT('Ctrl Pts',(6.9999999999295,-5.89333513423436,20.5777738225602));
#63559=CARTESIAN_POINT('Ctrl Pts',(6.99999999970464,-6.06295587913339,20.942575730976));
#63560=CARTESIAN_POINT('Ctrl Pts',(7.00000000000036,-6.25270756111132,21.2980264726989));
#63561=CARTESIAN_POINT('Ctrl Pts',(7.00000000000036,-6.46120307607831,21.6419501662451));
#63562=CARTESIAN_POINT('Ctrl Pts',(7.00000000000036,-6.54468519845901,21.7796580679176));
#63563=CARTESIAN_POINT('Ctrl Pts',(6.99999999962042,-6.63117389391976,21.9155174566697));
#63564=CARTESIAN_POINT('Ctrl Pts',(6.99999999912255,-6.72060835796162,22.0494162477555));
#63565=CARTESIAN_POINT('Ctrl Pts',(6.99999999824675,-6.87793233894469,22.2849573346076));
#63566=CARTESIAN_POINT('Ctrl Pts',(6.9999999988619,-7.04437018592607,22.5144339817016));
#63567=CARTESIAN_POINT('Ctrl Pts',(6.99999999981869,-7.21957967785347,22.7372465183685));
#63568=CARTESIAN_POINT('Ctrl Pts',(6.99999999992587,-7.23920763462172,22.7622072370432));
#63569=CARTESIAN_POINT('Ctrl Pts',(7.00000000000036,-7.25894570336743,22.7870842781222));
#63570=CARTESIAN_POINT('Ctrl Pts',(7.00000000000036,-7.27879342491422,22.811876764014));
#63571=CARTESIAN_POINT('Ctrl Pts',(7.00000000000036,-7.41703735932601,22.9845621166103));
#63572=CARTESIAN_POINT('Ctrl Pts',(6.99999999634334,-7.56056958524369,23.1531795030631));
#63573=CARTESIAN_POINT('Ctrl Pts',(6.99999999541996,-7.70901246660694,23.3172462117123));
#63574=CARTESIAN_POINT('Ctrl Pts',(6.99999999531015,-7.72666492377434,23.3367566154476));
#63575=CARTESIAN_POINT('Ctrl Pts',(6.99999999523504,-7.74438678100536,23.3562027086881));
#63576=CARTESIAN_POINT('Ctrl Pts',(6.99999999519958,-7.76217736879295,23.3755837147586));
#63577=CARTESIAN_POINT('Ctrl Pts',(6.99999999489101,-7.91698551942648,23.5442311896495));
#63578=CARTESIAN_POINT('Ctrl Pts',(7.00000000000036,-8.07700088558281,23.7079464463786));
#63579=CARTESIAN_POINT('Ctrl Pts',(7.00000000000036,-8.24167851282883,23.8663282373223));
#63580=CARTESIAN_POINT('Ctrl Pts',(7.00000000000036,-8.36437153139225,23.9843305448691));
#63581=CARTESIAN_POINT('Ctrl Pts',(6.99999999741532,-8.48968648772239,24.0993265809265));
#63582=CARTESIAN_POINT('Ctrl Pts',(6.99999999745853,-8.61766942749797,24.2114123910189));
#63583=CARTESIAN_POINT('Ctrl Pts',(6.99999999749976,-8.73980227281244,24.3183747637381));
#63584=CARTESIAN_POINT('Ctrl Pts',(6.99999999865195,-8.86436525968121,24.4226868685668));
#63585=CARTESIAN_POINT('Ctrl Pts',(6.99999999924104,-8.99142942748623,24.5244006129468));
#63586=CARTESIAN_POINT('Ctrl Pts',(6.9999999997591,-9.10317157848991,24.6138492181672));
#63587=CARTESIAN_POINT('Ctrl Pts',(6.99999999990898,-9.2168486419286,24.7012880171126));
#63588=CARTESIAN_POINT('Ctrl Pts',(6.99999999989432,-9.33251047983013,24.7867157006585));
#63589=CARTESIAN_POINT('Ctrl Pts',(6.26386081957825,-3.90572621560986,15.814440855933));
#63590=CARTESIAN_POINT('Ctrl Pts',(6.26460716030619,-3.90306652820293,16.0736422380589));
#63591=CARTESIAN_POINT('Ctrl Pts',(6.26531569223296,-3.90881658977334,16.3306845724835));
#63592=CARTESIAN_POINT('Ctrl Pts',(6.2659863977903,-3.92256349692468,16.5850748047761));
#63593=CARTESIAN_POINT('Ctrl Pts',(6.26666475020584,-3.93646713551864,16.8423653947753));
#63594=CARTESIAN_POINT('Ctrl Pts',(6.26730440882618,-3.95855099096231,17.096943119821));
#63595=CARTESIAN_POINT('Ctrl Pts',(6.2679053588221,-3.98839441038359,17.3483506398906));
#63596=CARTESIAN_POINT('Ctrl Pts',(6.26800177816493,-3.99318263387662,17.3886876862903));
#63597=CARTESIAN_POINT('Ctrl Pts',(6.26809720105533,-3.99817062217637,17.4289432315441));
#63598=CARTESIAN_POINT('Ctrl Pts',(6.26819162743929,-4.00335665371818,17.4691155096931));
#63599=CARTESIAN_POINT('Ctrl Pts',(6.26876871870475,-4.0350513282325,17.7146302679753));
#63600=CARTESIAN_POINT('Ctrl Pts',(6.26930858925204,-4.07414146028354,17.9570309131006));
#63601=CARTESIAN_POINT('Ctrl Pts',(6.26981122824073,-4.12011022476256,18.1959089254361));
#63602=CARTESIAN_POINT('Ctrl Pts',(6.27017913019625,-4.15375663645253,18.3707534755957));
#63603=CARTESIAN_POINT('Ctrl Pts',(6.27052708587458,-4.19108861036826,18.5437118696551));
#63604=CARTESIAN_POINT('Ctrl Pts',(6.27085509181305,-4.23191018794964,18.7146402529524));
#63605=CARTESIAN_POINT('Ctrl Pts',(6.27121137657533,-4.27625117193226,18.9003051183254));
#63606=CARTESIAN_POINT('Ctrl Pts',(6.27154412268532,-4.32470931376187,19.08357463927));
#63607=CARTESIAN_POINT('Ctrl Pts',(6.27185332606288,-4.37704085982857,19.2642821899259));
#63608=CARTESIAN_POINT('Ctrl Pts',(6.27227096752176,-4.44772515641576,19.5083641455751));
#63609=CARTESIAN_POINT('Ctrl Pts',(6.27264565767329,-4.52547485758646,19.7477703759114));
#63610=CARTESIAN_POINT('Ctrl Pts',(6.27297738858458,-4.60968094217816,19.9821807438504));
#63611=CARTESIAN_POINT('Ctrl Pts',(6.27330911949587,-4.69388702676985,20.2165911117894));
#63612=CARTESIAN_POINT('Ctrl Pts',(6.27359789118611,-4.78454955978446,20.4460058025126));
#63613=CARTESIAN_POINT('Ctrl Pts',(6.27384369786499,-4.8810873310656,20.6701561528923));
#63614=CARTESIAN_POINT('Ctrl Pts',(6.27395596416794,-4.92517864187066,20.7725314473961));
#63615=CARTESIAN_POINT('Ctrl Pts',(6.27405926809239,-4.97049589580692,20.8738092985562));
#63616=CARTESIAN_POINT('Ctrl Pts',(6.27415361626388,-5.01698560251817,20.9739675362492));
#63617=CARTESIAN_POINT('Ctrl Pts',(6.27415652037485,-5.0184165922798,20.9770504856335));
#63618=CARTESIAN_POINT('Ctrl Pts',(6.27415941593985,-5.01984869290736,20.9801323742789));
#63619=CARTESIAN_POINT('Ctrl Pts',(6.27416230296468,-5.02128190286476,20.9832132015813));
#63620=CARTESIAN_POINT('Ctrl Pts',(6.27420631248003,-5.04312961089931,21.0301770222397));
#63621=CARTESIAN_POINT('Ctrl Pts',(6.27424833746245,-5.06523509446001,21.076894204489));
#63622=CARTESIAN_POINT('Ctrl Pts',(6.2742883985241,-5.0875921193759,21.1233630648912));
#63623=CARTESIAN_POINT('Ctrl Pts',(6.27431785022144,-5.10402833709297,21.1575255847035));
#63624=CARTESIAN_POINT('Ctrl Pts',(6.27434670120188,-5.12089353968899,21.192152832586));
#63625=CARTESIAN_POINT('Ctrl Pts',(6.27437398730189,-5.1375803959525,21.2260036828553));
#63626=CARTESIAN_POINT('Ctrl Pts',(6.27438625132226,-5.145080476395,21.2412182982423));
#63627=CARTESIAN_POINT('Ctrl Pts',(6.27439819921371,-5.15254388406323,21.256276383525));
#63628=CARTESIAN_POINT('Ctrl Pts',(6.27440974343164,-5.15991241649642,21.2710667690669));
#63629=CARTESIAN_POINT('Ctrl Pts',(6.27456064753034,-5.25623264816907,21.4644042314235));
#63630=CARTESIAN_POINT('Ctrl Pts',(6.27467736557741,-5.35907886487503,21.6577055885389));
#63631=CARTESIAN_POINT('Ctrl Pts',(6.2747598958331,-5.46870158665621,21.8504720742369));
#63632=CARTESIAN_POINT('Ctrl Pts',(6.27484107259586,-5.5765265001261,22.0400771971764));
#63633=CARTESIAN_POINT('Ctrl Pts',(6.27488917373459,-5.69090753982229,22.2291648994148));
#63634=CARTESIAN_POINT('Ctrl Pts',(6.27490419856597,-5.81206786878456,22.4172123727217));
#63635=CARTESIAN_POINT('Ctrl Pts',(6.27490863259839,-5.84782393232077,22.4727077436981));
#63636=CARTESIAN_POINT('Ctrl Pts',(6.27491018595364,-5.88417031203136,22.5281121924229));
#63637=CARTESIAN_POINT('Ctrl Pts',(6.27490885862982,-5.92111247084116,22.583411450356));
#63638=CARTESIAN_POINT('Ctrl Pts',(6.27490450996821,-6.04214469049153,22.7645863504783));
#63639=CARTESIAN_POINT('Ctrl Pts',(6.27486924032986,-6.16957355860617,22.9446356521944));
#63640=CARTESIAN_POINT('Ctrl Pts',(6.2748030501825,-6.30354337953915,23.1230248298937));
#63641=CARTESIAN_POINT('Ctrl Pts',(6.27475277160487,-6.40530795191046,23.2585307091866));
#63642=CARTESIAN_POINT('Ctrl Pts',(6.27468465176775,-6.51084628860725,23.3930777864523));
#63643=CARTESIAN_POINT('Ctrl Pts',(6.27459869119746,-6.62021326700212,23.5264134452897));
#63644=CARTESIAN_POINT('Ctrl Pts',(6.27448994699812,-6.75856768297465,23.6950893790818));
#63645=CARTESIAN_POINT('Ctrl Pts',(6.27435265036365,-6.90304997541691,23.8618280950501));
#63646=CARTESIAN_POINT('Ctrl Pts',(6.2741868037742,-7.05375344156325,24.0260801484426));
#63647=CARTESIAN_POINT('Ctrl Pts',(6.27401315425445,-7.21154736790509,24.1980601106643));
#63648=CARTESIAN_POINT('Ctrl Pts',(6.27380820507056,-7.37616248254101,24.3673132447826));
#63649=CARTESIAN_POINT('Ctrl Pts',(6.27357196000059,-7.54763091708786,24.5332701712914));
#63650=CARTESIAN_POINT('Ctrl Pts',(6.27333930797839,-7.71649149075496,24.6967030613646));
#63651=CARTESIAN_POINT('Ctrl Pts',(6.27307630478399,-7.89199856689717,24.8569392626461));
#63652=CARTESIAN_POINT('Ctrl Pts',(6.27278295501666,-8.0741504976575,25.0133963364823));
#63653=CARTESIAN_POINT('Ctrl Pts',(6.27261682411597,-8.17730743756334,25.1020016721282));
#63654=CARTESIAN_POINT('Ctrl Pts',(6.27244096040682,-8.2825949371111,25.1893942510749));
#63655=CARTESIAN_POINT('Ctrl Pts',(6.27225536487834,-8.39000786644608,25.2754626135137));
#63656=CARTESIAN_POINT('Ctrl Pts',(6.27204648957659,-8.51089390399926,25.3723267746377));
#63657=CARTESIAN_POINT('Ctrl Pts',(6.27182528795732,-8.63447217814325,25.467513907671));
#63658=CARTESIAN_POINT('Ctrl Pts',(6.27159176161367,-8.76072156035792,25.5608443099372));
#63659=CARTESIAN_POINT('Ctrl Pts',(-6.390310997314,-3.94960676120434,15.4604112548065));
#63660=CARTESIAN_POINT('Ctrl Pts',(-4.260207331542,-3.32899290723404,16.2184975538162));
#63661=CARTESIAN_POINT('Ctrl Pts',(0.0001535201380647,-2.70682847609605,
16.976602560809));
#63662=CARTESIAN_POINT('Ctrl Pts',(4.260514371819,-3.32903774766832,16.2184429159229));
#63663=CARTESIAN_POINT('Ctrl Pts',(6.390771557728,-3.949740952065,15.4602473392485));
#63664=CARTESIAN_POINT('Ctrl Pts',(-6.390310997314,-3.91824203061707,16.2404119010483));
#63665=CARTESIAN_POINT('Ctrl Pts',(-4.260207331542,-3.34435482128984,16.9591696862112));
#63666=CARTESIAN_POINT('Ctrl Pts',(0.0001535201380647,-2.7685203922099,
17.6779350698092));
#63667=CARTESIAN_POINT('Ctrl Pts',(4.260514371819,-3.34439632263995,16.9591178835817));
#63668=CARTESIAN_POINT('Ctrl Pts',(6.390771557728,-3.9183661181109,16.2402564892191));
#63669=CARTESIAN_POINT('Ctrl Pts',(-6.390310997314,-4.02653939109499,18.1258674862954));
#63670=CARTESIAN_POINT('Ctrl Pts',(-4.260207331542,-3.53814955008341,18.7395147188676));
#63671=CARTESIAN_POINT('Ctrl Pts',(0.0001535201380647,-3.05107310998534,
19.3531400775061));
#63672=CARTESIAN_POINT('Ctrl Pts',(4.260514371819,-3.53818465449488,18.7394704938521));
#63673=CARTESIAN_POINT('Ctrl Pts',(6.390771557728,-4.02664499212973,18.1257348017601));
#63674=CARTESIAN_POINT('Ctrl Pts',(-6.390310997314,-4.89945800151002,21.0044951210507));
#63675=CARTESIAN_POINT('Ctrl Pts',(-4.260207331542,-4.44478850539311,21.4424839510742));
#63676=CARTESIAN_POINT('Ctrl Pts',(0.0001535201380647,-3.98943347064956,
21.8807678511962));
#63677=CARTESIAN_POINT('Ctrl Pts',(4.260514371819,-4.44482132359356,21.4424523632204));
#63678=CARTESIAN_POINT('Ctrl Pts',(6.390771557728,-4.89955631142349,21.0044004178757));
#63679=CARTESIAN_POINT('Ctrl Pts',(-6.390310997314,-6.63374323540806,23.7052269015879));
#63680=CARTESIAN_POINT('Ctrl Pts',(-4.260207331542,-6.0952579924294,23.9981305004778));
#63681=CARTESIAN_POINT('Ctrl Pts',(0.0001535201380647,-5.55782051180541,
24.2900535316613));
#63682=CARTESIAN_POINT('Ctrl Pts',(4.260514371819,-6.09529672644794,23.9981094610928));
#63683=CARTESIAN_POINT('Ctrl Pts',(6.390771557728,-6.63385966821385,23.7051635691471));
#63684=CARTESIAN_POINT('Ctrl Pts',(-6.390310997314,-8.18394441798506,25.1149801838822));
#63685=CARTESIAN_POINT('Ctrl Pts',(-4.260207331542,-7.53598553401078,25.3660543259899));
#63686=CARTESIAN_POINT('Ctrl Pts',(0.0001535201380647,-6.88615455534451,
25.6190325570298));
#63687=CARTESIAN_POINT('Ctrl Pts',(4.260514371819,-7.536032368418,25.366036093427));
#63688=CARTESIAN_POINT('Ctrl Pts',(6.390771557728,-8.18408452146462,25.1149258959381));
#63689=CARTESIAN_POINT('Ctrl Pts',(-6.390310997314,-8.98425336235418,25.6807325212854));
#63690=CARTESIAN_POINT('Ctrl Pts',(-4.260207331542,-8.27686663367918,25.9287944450768));
#63691=CARTESIAN_POINT('Ctrl Pts',(0.0001535201380647,-7.56887097380373,
26.1774616570061));
#63692=CARTESIAN_POINT('Ctrl Pts',(4.260514371819,-8.2769176601128,25.9287765232156));
#63693=CARTESIAN_POINT('Ctrl Pts',(6.390771557728,-8.9844063154964,25.680678884635));
#63694=CARTESIAN_POINT('Ctrl Pts',(-6.26386060032414,-3.90573753027274,
15.8144217558848));
#63695=CARTESIAN_POINT('Ctrl Pts',(-5.97426230930331,-3.82545376840559,
15.9107534531458));
#63696=CARTESIAN_POINT('Ctrl Pts',(-5.68272415002883,-3.75014409027891,
15.9997900251984));
#63697=CARTESIAN_POINT('Ctrl Pts',(-5.38973713287711,-3.68009451384404,
16.0816096133529));
#63698=CARTESIAN_POINT('Ctrl Pts',(-5.1148963508353,-3.61438347805748,16.1583616818006));
#63699=CARTESIAN_POINT('Ctrl Pts',(-4.8387806239847,-3.55330174463071,16.2287627175083));
#63700=CARTESIAN_POINT('Ctrl Pts',(-4.56179526395762,-3.49706393515746,
16.2929147389837));
#63701=CARTESIAN_POINT('Ctrl Pts',(-4.30450523531574,-3.44482497347112,
16.3525051644172));
#63702=CARTESIAN_POINT('Ctrl Pts',(-4.04646484891085,-3.39676582845628,
16.4067035756603));
#63703=CARTESIAN_POINT('Ctrl Pts',(-3.78799895819672,-3.35303372379852,
16.4556278903896));
#63704=CARTESIAN_POINT('Ctrl Pts',(-3.57232101449432,-3.31654128612985,
16.4964529894721));
#63705=CARTESIAN_POINT('Ctrl Pts',(-3.35634678627636,-3.28306154818238,
16.5336061380409));
#63706=CARTESIAN_POINT('Ctrl Pts',(-3.14026502702693,-3.25266330082624,
16.5671782502199));
#63707=CARTESIAN_POINT('Ctrl Pts',(-2.90080112829706,-3.21897566864598,
16.6043831901413));
#63708=CARTESIAN_POINT('Ctrl Pts',(-2.66120552935244,-3.18907472968854,
16.6372138404118));
#63709=CARTESIAN_POINT('Ctrl Pts',(-2.42172500293894,-3.16301823790052,
16.6656906330402));
#63710=CARTESIAN_POINT('Ctrl Pts',(-2.18568576270281,-3.13733617256948,
16.6937582199836));
#63711=CARTESIAN_POINT('Ctrl Pts',(-1.94975831162179,-3.11538890068632,
16.7175961664648));
#63712=CARTESIAN_POINT('Ctrl Pts',(-1.71417893635696,-3.09719944592268,
16.737263052464));
#63713=CARTESIAN_POINT('Ctrl Pts',(-1.4801385381641,-3.0791288180037,16.7568014599553));
#63714=CARTESIAN_POINT('Ctrl Pts',(-1.24644168286964,-3.06476712988494,
16.7722230853077));
#63715=CARTESIAN_POINT('Ctrl Pts',(-1.01332005652778,-3.05410406159889,
16.7836246209729));
#63716=CARTESIAN_POINT('Ctrl Pts',(-0.781833519416523,-3.04351578289111,
16.7949461875317));
#63717=CARTESIAN_POINT('Ctrl Pts',(-0.5509141703719,-3.03657445544106,16.8023038449724));
#63718=CARTESIAN_POINT('Ctrl Pts',(-0.32078885450044,-3.03323674555433,
16.8058315010754));
#63719=CARTESIAN_POINT('Ctrl Pts',(-0.213870712629672,-3.03168601769182,
16.8074704795349));
#63720=CARTESIAN_POINT('Ctrl Pts',(-0.107123971484708,-3.03091269623866,
16.8082832675462));
#63721=CARTESIAN_POINT('Ctrl Pts',(-0.000571381538524201,-3.03090994562974,
16.8082862144943));
#63722=CARTESIAN_POINT('Ctrl Pts',(-0.000380921640730136,-3.0309099407131,
16.8082862197619));
#63723=CARTESIAN_POINT('Ctrl Pts',(-0.000190461127502138,-3.03090993825803,
16.8082862224426));
#63724=CARTESIAN_POINT('Ctrl Pts',(1.03384559906101E-12,-3.03090993826458,
16.8082862225363));
#63725=CARTESIAN_POINT('Ctrl Pts',(0.230288294953843,-3.0309099461773,16.8082863358534));
#63726=CARTESIAN_POINT('Ctrl Pts',(0.461476135630093,-3.03451153042456,
16.8045011076514));
#63727=CARTESIAN_POINT('Ctrl Pts',(0.693339238579527,-3.04177406743476,
16.7967768846798));
#63728=CARTESIAN_POINT('Ctrl Pts',(0.927160087319404,-3.04909792597943,
16.788987441909));
#63729=CARTESIAN_POINT('Ctrl Pts',(1.1616676496846,-3.06014480501952,16.7771922026878));
#63730=CARTESIAN_POINT('Ctrl Pts',(1.39663191288004,-3.07494113876898,16.7612740817315));
#63731=CARTESIAN_POINT('Ctrl Pts',(1.6331435537806,-3.08983491506843,16.7452511305974));
#63732=CARTESIAN_POINT('Ctrl Pts',(1.87011793060501,-3.10852764050927,16.7250508490044));
#63733=CARTESIAN_POINT('Ctrl Pts',(2.10732045625743,-3.13101204586718,16.7005944302589));
#63734=CARTESIAN_POINT('Ctrl Pts',(2.34747479622559,-3.15377625342971,16.6758336690247));
#63735=CARTESIAN_POINT('Ctrl Pts',(2.58786299864806,-3.18042705182343,16.6467102007614));
#63736=CARTESIAN_POINT('Ctrl Pts',(2.82824160919085,-3.21092262617489,16.613183394872));
#63737=CARTESIAN_POINT('Ctrl Pts',(2.93189543141303,-3.22407264328853,16.5987262783694));
#63738=CARTESIAN_POINT('Ctrl Pts',(3.03554747009574,-3.23793714373867,16.5834509066644));
#63739=CARTESIAN_POINT('Ctrl Pts',(3.13917820496035,-3.25251088491731,16.5673563184501));
#63740=CARTESIAN_POINT('Ctrl Pts',(3.40197375645711,-3.28946820607705,16.5265423051997));
#63741=CARTESIAN_POINT('Ctrl Pts',(3.66462147904948,-3.33098599837418,16.4804289673528));
#63742=CARTESIAN_POINT('Ctrl Pts',(3.92678119996645,-3.37693833074301,16.4288554486851));
#63743=CARTESIAN_POINT('Ctrl Pts',(4.19748597231201,-3.42438847155465,16.3756008999651));
#63744=CARTESIAN_POINT('Ctrl Pts',(4.4676704118551,-3.47656651974571,16.3165247605884));
#63745=CARTESIAN_POINT('Ctrl Pts',(4.73695998620211,-3.53329768778599,16.251498714715));
#63746=CARTESIAN_POINT('Ctrl Pts',(5.03194795561124,-3.59544273035955,16.1802672113141));
#63747=CARTESIAN_POINT('Ctrl Pts',(5.32586211575626,-3.66305099399998,16.1018960658767));
#63748=CARTESIAN_POINT('Ctrl Pts',(5.61821015094397,-3.73585595945423,16.0162717568522));
#63749=CARTESIAN_POINT('Ctrl Pts',(5.83434844010851,-3.78968201190525,15.9529681274928));
#63750=CARTESIAN_POINT('Ctrl Pts',(6.04963069831582,-3.84634765920576,15.8857012380644));
#63751=CARTESIAN_POINT('Ctrl Pts',(6.26385797816486,-3.90573660195549,15.8144409703668));
#63752=CARTESIAN_POINT('Ctrl Pts',(-6.38351709471616,-3.93920782693273,
15.7749258978406));
#63753=CARTESIAN_POINT('Ctrl Pts',(-6.08740745253563,-3.85548476926818,
15.881473813723));
#63754=CARTESIAN_POINT('Ctrl Pts',(-5.13142578697123,-3.60387668806693,
16.1968376701999));
#63755=CARTESIAN_POINT('Ctrl Pts',(-3.40211712930966,-3.25762303527195,
16.6110525573658));
#63756=CARTESIAN_POINT('Ctrl Pts',(-1.16426938927718,-3.02328203047528,
16.878951814368));
#63757=CARTESIAN_POINT('Ctrl Pts',(1.16113505781623,-3.02310888355152,16.8791462423432));
#63758=CARTESIAN_POINT('Ctrl Pts',(3.39945869805431,-3.25719731223483,16.6115486323221));
#63759=CARTESIAN_POINT('Ctrl Pts',(5.12988614343298,-3.6034988213486,16.1973036504942));
#63760=CARTESIAN_POINT('Ctrl Pts',(6.08676115286924,-3.85530247941335,15.8817056622505));
#63761=CARTESIAN_POINT('Ctrl Pts',(6.38348326401547,-3.93919827240965,15.7749380472911));
#63762=CARTESIAN_POINT('Ctrl Pts',(-6.17631081322735,-3.89089882940664,
15.1504194794343));
#63763=CARTESIAN_POINT('Ctrl Pts',(-5.88965655823781,-3.81103185421913,
15.2535318539487));
#63764=CARTESIAN_POINT('Ctrl Pts',(-4.96426339598262,-3.57096639928173,
15.5587423966376));
#63765=CARTESIAN_POINT('Ctrl Pts',(-3.29074409978021,-3.24047405664135,
15.95962814198));
#63766=CARTESIAN_POINT('Ctrl Pts',(-1.1260028682163,-3.01678341201172,16.218861585521));
#63767=CARTESIAN_POINT('Ctrl Pts',(1.12297142654902,-3.0166181415462,16.219049702787));
#63768=CARTESIAN_POINT('Ctrl Pts',(3.28817192979132,-3.24006767592172,15.9601082192533));
#63769=CARTESIAN_POINT('Ctrl Pts',(4.96277311007818,-3.5706058011467,15.5591933938224));
#63770=CARTESIAN_POINT('Ctrl Pts',(5.88903089909969,-3.81085796060267,15.2537562258459));
#63771=CARTESIAN_POINT('Ctrl Pts',(6.17627806349228,-3.89088971520562,15.1504312367114));
#63772=CARTESIAN_POINT('Ctrl Pts',(-6.17621381887775,-3.37750417917966,
14.7398362123642));
#63773=CARTESIAN_POINT('Ctrl Pts',(-5.89023958152254,-3.29860736714451,
14.841735137595));
#63774=CARTESIAN_POINT('Ctrl Pts',(-4.96677349652124,-3.06133287700747,
15.1434924061647));
#63775=CARTESIAN_POINT('Ctrl Pts',(-3.29476494977961,-2.73403327557292,
15.5405123166288));
#63776=CARTESIAN_POINT('Ctrl Pts',(-1.12803856271859,-2.51194808909339,
15.7978000261188));
#63777=CARTESIAN_POINT('Ctrl Pts',(1.12500219242395,-2.51178381698562,15.7979869150338));
#63778=CARTESIAN_POINT('Ctrl Pts',(3.29219295119216,-2.73363027885014,15.5409883200213));
#63779=CARTESIAN_POINT('Ctrl Pts',(4.96528590892401,-3.06097626156985,15.1439385253728));
#63780=CARTESIAN_POINT('Ctrl Pts',(5.8896153942606,-3.29843557903911,14.8419568740436));
#63781=CARTESIAN_POINT('Ctrl Pts',(6.17618114388549,-3.37749517511435,14.7398478327077));
#63782=CARTESIAN_POINT('Ctrl Pts',(-6.37985701943049,-2.76049912597563,
14.8225434715735));
#63783=CARTESIAN_POINT('Ctrl Pts',(-6.08546444017595,-2.67906593471349,
14.9262503141624));
#63784=CARTESIAN_POINT('Ctrl Pts',(-5.1344116261327,-2.43405279620404,15.2335227068454));
#63785=CARTESIAN_POINT('Ctrl Pts',(-3.40949469842141,-2.09538588962233,
15.6386468844809));
#63786=CARTESIAN_POINT('Ctrl Pts',(-1.16830514728113,-1.86490505714411,
15.9019381804586));
#63787=CARTESIAN_POINT('Ctrl Pts',(1.16516121475652,-1.86473433147697,15.9021296854872));
#63788=CARTESIAN_POINT('Ctrl Pts',(3.40683809148816,-2.09496825154861,15.6391333471311));
#63789=CARTESIAN_POINT('Ctrl Pts',(5.13287899229569,-2.43368435366994,15.2339772467715));
#63790=CARTESIAN_POINT('Ctrl Pts',(6.08482185993278,-2.67888861493498,14.9264759920189));
#63791=CARTESIAN_POINT('Ctrl Pts',(6.37982337814739,-2.76048983145035,14.822555300347));
#63792=CARTESIAN_POINT('Ctrl Pts',(-6.24994586082225,-2.76546765008493,
14.8593861744158));
#63793=CARTESIAN_POINT('Ctrl Pts',(-5.99627373449832,-2.69661205562347,
14.946811432374));
#63794=CARTESIAN_POINT('Ctrl Pts',(-5.7377440125489,-2.63061153982227,15.0295063433286));
#63795=CARTESIAN_POINT('Ctrl Pts',(-5.4744339766703,-2.56798096496872,15.1071490882542));
#63796=CARTESIAN_POINT('Ctrl Pts',(-5.27195631093415,-2.51981989675213,
15.1668540732975));
#63797=CARTESIAN_POINT('Ctrl Pts',(-5.06665225396755,-2.47365226106918,
15.2235711883174));
#63798=CARTESIAN_POINT('Ctrl Pts',(-4.85859706661085,-2.42973038675524,
15.2771463537608));
#63799=CARTESIAN_POINT('Ctrl Pts',(-4.61928783915712,-2.37921057062411,
15.338769577944));
#63800=CARTESIAN_POINT('Ctrl Pts',(-4.37632859149279,-2.33164851275368,
15.396241002441));
#63801=CARTESIAN_POINT('Ctrl Pts',(-4.12983623086809,-2.28736457460126,
15.4493265339033));
#63802=CARTESIAN_POINT('Ctrl Pts',(-4.00659005055573,-2.26522260552506,
15.4758692996345));
#63803=CARTESIAN_POINT('Ctrl Pts',(-3.88246099670014,-2.2438995742547,15.5013154231866));
#63804=CARTESIAN_POINT('Ctrl Pts',(-3.75746623583399,-2.22343165156168,
15.5256346174406));
#63805=CARTESIAN_POINT('Ctrl Pts',(-3.69496885540091,-2.21319769021516,
15.5377942145676));
#63806=CARTESIAN_POINT('Ctrl Pts',(-3.63225504686568,-2.20317750452444,
15.5496720675799));
#63807=CARTESIAN_POINT('Ctrl Pts',(-3.56932715761033,-2.19337530198695,
15.5612643283527));
#63808=CARTESIAN_POINT('Ctrl Pts',(-3.53786321298266,-2.18847420071821,
15.5670604587391));
#63809=CARTESIAN_POINT('Ctrl Pts',(-3.5063457481126,-2.18362759514885,15.5727851903465));
#63810=CARTESIAN_POINT('Ctrl Pts',(-3.4747750621384,-2.17883600094445,15.5784380382115));
#63811=CARTESIAN_POINT('Ctrl Pts',(-3.46643034044414,-2.17756949314224,
15.5799321914349));
#63812=CARTESIAN_POINT('Ctrl Pts',(-3.45808190106549,-2.17630682803461,
15.5814213225294));
#63813=CARTESIAN_POINT('Ctrl Pts',(-3.44972974845269,-2.17504801628272,
15.582905422515));
#63814=CARTESIAN_POINT('Ctrl Pts',(-3.44228250133664,-2.17392558921229,
15.5842287291942));
#63815=CARTESIAN_POINT('Ctrl Pts',(-3.43483230201171,-2.17280622575502,
15.5855480358875));
#63816=CARTESIAN_POINT('Ctrl Pts',(-3.42737915554867,-2.17168993150639,
15.5868633367423));
#63817=CARTESIAN_POINT('Ctrl Pts',(-3.41156724030373,-2.16932170351904,
15.5896537589808));
#63818=CARTESIAN_POINT('Ctrl Pts',(-3.39713125426695,-2.16717258148387,
15.592184569876));
#63819=CARTESIAN_POINT('Ctrl Pts',(-3.37990364855089,-2.16462676050287,
15.5951804590587));
#63820=CARTESIAN_POINT('Ctrl Pts',(-3.08243670618948,-2.12066838372666,
15.6469101079446));
#63821=CARTESIAN_POINT('Ctrl Pts',(-2.78280714443239,-2.08213371852645,
15.6918061299537));
#63822=CARTESIAN_POINT('Ctrl Pts',(-2.48135671024121,-2.04930088083302,
15.7298141593332));
#63823=CARTESIAN_POINT('Ctrl Pts',(-2.18489990185431,-2.01701192991811,
15.7671925731781));
#63824=CARTESIAN_POINT('Ctrl Pts',(-1.88668153319448,-1.99023730879995,
15.7979092668204));
#63825=CARTESIAN_POINT('Ctrl Pts',(-1.58702423552026,-1.96927461093504,
15.821874900134));
#63826=CARTESIAN_POINT('Ctrl Pts',(-1.44871564458144,-1.9595991542501,15.8329363793648));
#63827=CARTESIAN_POINT('Ctrl Pts',(-1.31010052600959,-1.95116231486475,
15.8425591270519));
#63828=CARTESIAN_POINT('Ctrl Pts',(-1.17121088137433,-1.94399593480486,
15.8507316176886));
#63829=CARTESIAN_POINT('Ctrl Pts',(-0.870280897974668,-1.92846865314091,
15.8684388231329));
#63830=CARTESIAN_POINT('Ctrl Pts',(-0.568061182732521,-1.9189035036577,
15.8793402084787));
#63831=CARTESIAN_POINT('Ctrl Pts',(-0.264946396586357,-1.91537688572319,
15.8833583473097));
#63832=CARTESIAN_POINT('Ctrl Pts',(-0.176893607935623,-1.91435242714238,
15.8845255893758));
#63833=CARTESIAN_POINT('Ctrl Pts',(-0.0887653799340636,-1.91383774912774,
15.8851117379332));
#63834=CARTESIAN_POINT('Ctrl Pts',(-0.000571644969191336,-1.9138352439744,
15.8851143000971));
#63835=CARTESIAN_POINT('Ctrl Pts',(0.298411593004284,-1.91382675132062,
15.885122986021));
#63836=CARTESIAN_POINT('Ctrl Pts',(0.596636753996419,-1.91967815635201,
15.8784305185147));
#63837=CARTESIAN_POINT('Ctrl Pts',(0.893741083173373,-1.93132463844706,
15.8651185988725));
#63838=CARTESIAN_POINT('Ctrl Pts',(0.985253235876338,-1.93491191248944,
15.861018347535));
#63839=CARTESIAN_POINT('Ctrl Pts',(1.0766591370822,-1.93904921940413,15.8562898183046));
#63840=CARTESIAN_POINT('Ctrl Pts',(1.16794837273084,-1.94373530482249,15.8509346664032));
#63841=CARTESIAN_POINT('Ctrl Pts',(1.3473991887541,-1.95294692595509,15.840407835153));
#63842=CARTESIAN_POINT('Ctrl Pts',(1.5263991835423,-1.9642787774411,15.8274599788759));
#63843=CARTESIAN_POINT('Ctrl Pts',(1.70488263911043,-1.9776671612215,15.8121140552086));
#63844=CARTESIAN_POINT('Ctrl Pts',(1.98691438642767,-1.99882289949046,15.7878650980584));
#63845=CARTESIAN_POINT('Ctrl Pts',(2.26764243136529,-2.02514654777305,15.7576264894017));
#63846=CARTESIAN_POINT('Ctrl Pts',(2.54678456470886,-2.05638855538998,15.7214699774126));
#63847=CARTESIAN_POINT('Ctrl Pts',(2.68635563138065,-2.07200955919844,15.7033917214181));
#63848=CARTESIAN_POINT('Ctrl Pts',(2.82553043280264,-2.08885858665511,15.6838337769631));
#63849=CARTESIAN_POINT('Ctrl Pts',(2.96427493797265,-2.10689523241144,15.6628038899662));
#63850=CARTESIAN_POINT('Ctrl Pts',(3.03364719055766,-2.1159135552896,15.6522889464677));
#63851=CARTESIAN_POINT('Ctrl Pts',(3.10291186552976,-2.125228779693,15.6414059949692));
#63852=CARTESIAN_POINT('Ctrl Pts',(3.17206480176733,-2.13483519380386,15.6301559451082));
#63853=CARTESIAN_POINT('Ctrl Pts',(3.20664126988611,-2.13963840085929,15.6245309201777));
#63854=CARTESIAN_POINT('Ctrl Pts',(3.24118980305764,-2.14451440514934,15.6188141193533));
#63855=CARTESIAN_POINT('Ctrl Pts',(3.2757098827992,-2.14946247489551,15.6130056505027));
#63856=CARTESIAN_POINT('Ctrl Pts',(3.29296992266997,-2.1519365097686,15.6101014160774));
#63857=CARTESIAN_POINT('Ctrl Pts',(3.31022284916438,-2.15442856099336,15.6071742645679));
#63858=CARTESIAN_POINT('Ctrl Pts',(3.32746859777775,-2.15693853479366,15.6042242092418));
#63859=CARTESIAN_POINT('Ctrl Pts',(3.34471434639113,-2.15944850859396,15.6012741539158));
#63860=CARTESIAN_POINT('Ctrl Pts',(3.36334195791706,-2.1621816194904,15.5980596952111));
#63861=CARTESIAN_POINT('Ctrl Pts',(3.37918424551883,-2.16452212943542,15.5953053448536));
#63862=CARTESIAN_POINT('Ctrl Pts',(3.40180447282053,-2.16786399951689,15.5913725775209));
#63863=CARTESIAN_POINT('Ctrl Pts',(3.42439771599313,-2.17123483076243,15.587402831826));
#63864=CARTESIAN_POINT('Ctrl Pts',(3.44696382211482,-2.17463439951978,15.5833962810123));
#63865=CARTESIAN_POINT('Ctrl Pts',(3.72166647695343,-2.2160181702915,15.5346235712079));
#63866=CARTESIAN_POINT('Ctrl Pts',(3.99234601765621,-2.26165697685362,15.4803988058823));
#63867=CARTESIAN_POINT('Ctrl Pts',(4.25883451373603,-2.31107032049297,15.4210479140662));
#63868=CARTESIAN_POINT('Ctrl Pts',(4.53188464578493,-2.36170034844608,15.3602356497996));
#63869=CARTESIAN_POINT('Ctrl Pts',(4.80053488116735,-2.4162931606847,15.2940417166047));
#63870=CARTESIAN_POINT('Ctrl Pts',(5.06462595783161,-2.47437565815115,15.2227911584299));
#63871=CARTESIAN_POINT('Ctrl Pts',(5.20181840798739,-2.50454888565751,15.1857772661983));
#63872=CARTESIAN_POINT('Ctrl Pts',(5.33778082244635,-2.53566457398629,15.1473983324778));
#63873=CARTESIAN_POINT('Ctrl Pts',(5.47249295507274,-2.56766076945225,15.1076973074869));
#63874=CARTESIAN_POINT('Ctrl Pts',(5.73647117932479,-2.63035964220599,15.0299002607491));
#63875=CARTESIAN_POINT('Ctrl Pts',(5.99564777821735,-2.69643720778191,14.9470280121331));
#63876=CARTESIAN_POINT('Ctrl Pts',(6.24994450567097,-2.76546231685323,14.859387545079));
#63877=CARTESIAN_POINT('Ctrl Pts',(7.0000012587911,8.04447766145535,12.5220647156823));
#63878=CARTESIAN_POINT('Ctrl Pts',(7.00000125879157,10.7706828754762,10.7706844567013));
#63879=CARTESIAN_POINT('Ctrl Pts',(7.00000125879419,12.5220635346855,8.04447949979687));
#63880=CARTESIAN_POINT('Ctrl Pts',(4.44295390839243E-7,9.2830316114314,
14.4500025344128));
#63881=CARTESIAN_POINT('Ctrl Pts',(4.44295937338156E-7,12.4289722487314,
12.4289740734016));
#63882=CARTESIAN_POINT('Ctrl Pts',(4.44298966301522E-7,14.4500011715914,
9.28303373280449));
#63883=CARTESIAN_POINT('Ctrl Pts',(-7.00000045620705,8.04447780346309,12.5220649367283));
#63884=CARTESIAN_POINT('Ctrl Pts',(-7.00000045620657,10.7706830656127,10.7706846468282));
#63885=CARTESIAN_POINT('Ctrl Pts',(-7.00000045620395,12.5220637557412,8.04447964179496));
#63886=CARTESIAN_POINT('Origin',(7.,0.,0.));
#63887=CARTESIAN_POINT('Origin',(-7.,0.,0.));
#63888=CARTESIAN_POINT('Ctrl Pts',(7.00000187330025,14.5427410982365,3.16613343860038));
#63889=CARTESIAN_POINT('Ctrl Pts',(7.00000187328746,15.2320474980471,-1.12398530161775E-6));
#63890=CARTESIAN_POINT('Ctrl Pts',(7.00000187329306,14.5427406309767,-3.16613558484275));
#63891=CARTESIAN_POINT('Ctrl Pts',(-6.61390457865313E-8,16.781789433929,
3.65360177478736));
#63892=CARTESIAN_POINT('Ctrl Pts',(-6.61538026439186E-8,17.5772237182236,
-1.29702851949525E-6));
#63893=CARTESIAN_POINT('Ctrl Pts',(-6.61473378705373E-8,16.7817888947284,
-3.65360425145376));
#63894=CARTESIAN_POINT('Ctrl Pts',(-7.00000199277579,14.5427410600111,3.16613343033478));
#63895=CARTESIAN_POINT('Ctrl Pts',(-7.00000199278858,15.2320474580187,-1.12396941171523E-6));
#63896=CARTESIAN_POINT('Ctrl Pts',(-7.00000199278298,14.5427405927513,-3.16613557654537));
#63897=CARTESIAN_POINT('Origin',(7.,0.,0.));
#63898=CARTESIAN_POINT('Origin',(-7.,0.,0.));
#63899=CARTESIAN_POINT('Ctrl Pts',(7.00000121187377,12.5220644953863,-8.04447803276786));
#63900=CARTESIAN_POINT('Ctrl Pts',(7.00000121181499,10.7706831479978,-10.7706847672647));
#63901=CARTESIAN_POINT('Ctrl Pts',(7.00000121183722,8.04447615020803,-12.5220657048102));
#63902=CARTESIAN_POINT('Ctrl Pts',(2.20648454367741E-7,14.4500023126704,
-9.28303206059653));
#63903=CARTESIAN_POINT('Ctrl Pts',(2.20580622652342E-7,12.4289725910948,
-12.4289744596026));
#63904=CARTESIAN_POINT('Ctrl Pts',(2.20606280418553E-7,9.28302988825824,
-14.4500037082345));
#63905=CARTESIAN_POINT('Ctrl Pts',(-7.00000081329343,12.52206460531,-8.04447810308367));
#63906=CARTESIAN_POINT('Ctrl Pts',(-7.00000081335221,10.7706832424739,-10.7706848616264));
#63907=CARTESIAN_POINT('Ctrl Pts',(-7.00000081332997,8.04447622063808,-12.5220658146196));
#63908=CARTESIAN_POINT('Origin',(7.,0.,0.));
#63909=CARTESIAN_POINT('Origin',(-7.,0.,0.));
#63910=CARTESIAN_POINT('Ctrl Pts',(7.00000130830393,3.16613101538807,-14.5427418150896));
#63911=CARTESIAN_POINT('Ctrl Pts',(7.00000130833239,3.0400473190149E-7,
-15.2320468148857));
#63912=CARTESIAN_POINT('Ctrl Pts',(7.00000130832594,-3.16613043489078,-14.5427419414591));
#63913=CARTESIAN_POINT('Ctrl Pts',(2.16205911596409E-9,3.65359888466782,
-16.7817898306923));
#63914=CARTESIAN_POINT('Ctrl Pts',(2.19489398097225E-9,3.50781807877837E-7,
-17.5772224790036));
#63915=CARTESIAN_POINT('Ctrl Pts',(2.18745987262781E-9,-3.65359821485225,
-16.7817899765181));
#63916=CARTESIAN_POINT('Ctrl Pts',(-7.00000130439666,3.16613101553883,-14.54274181636));
#63917=CARTESIAN_POINT('Ctrl Pts',(-7.0000013043682,3.03956066118533E-7,
-15.2320468161995));
#63918=CARTESIAN_POINT('Ctrl Pts',(-7.00000130437465,-3.16613043513888,
-14.5427419427295));
#63919=CARTESIAN_POINT('Origin',(7.,0.,0.));
#63920=CARTESIAN_POINT('Origin',(-7.,0.,0.));
#63921=CARTESIAN_POINT('Ctrl Pts',(7.00000187325864,-8.04449920362268,-12.52205063737));
#63922=CARTESIAN_POINT('Ctrl Pts',(7.00000187329277,-10.7706925366761,-10.7706713519787));
#63923=CARTESIAN_POINT('Ctrl Pts',(7.00000187328255,-12.5220664599442,-8.04447457416177));
#63924=CARTESIAN_POINT('Ctrl Pts',(3.27183161877263E-7,-9.28305673692403,
-14.4499867034266));
#63925=CARTESIAN_POINT('Ctrl Pts',(3.27222544072347E-7,-12.4289837543079,
-12.4289593079015));
#63926=CARTESIAN_POINT('Ctrl Pts',(3.27210751979541E-7,-14.4500049621397,
-9.283028315387));
#63927=CARTESIAN_POINT('Ctrl Pts',(-7.00000128222652,-8.04449930831836,
-12.5220508000662));
#63928=CARTESIAN_POINT('Ctrl Pts',(-7.00000128219239,-10.7706926767314,
-10.770671491959));
#63929=CARTESIAN_POINT('Ctrl Pts',(-7.00000128220261,-12.5220666227154,
-8.04447467878238));
#63930=CARTESIAN_POINT('Origin',(7.,0.,0.));
#63931=CARTESIAN_POINT('Origin',(-7.,0.,0.));
#63932=CARTESIAN_POINT('Ctrl Pts',(7.00000077642591,-14.5427415801911,-3.16613291281688));
#63933=CARTESIAN_POINT('Ctrl Pts',(7.00000077642943,-15.2320476743123,8.76418954263501E-7));
#63934=CARTESIAN_POINT('Ctrl Pts',(7.00000077642958,-14.5427412158444,3.16613458633202));
#63935=CARTESIAN_POINT('Ctrl Pts',(-5.53471878720152E-8,-16.7817891933195,
-3.65360099454467));
#63936=CARTESIAN_POINT('Ctrl Pts',(-5.53431341970486E-8,-17.5772230870879,
1.01135997016723E-6));
#63937=CARTESIAN_POINT('Ctrl Pts',(-5.53429606034401E-8,-16.7817887728767,
3.65360292572906));
#63938=CARTESIAN_POINT('Ctrl Pts',(-7.0000008764059,-14.5427415482134,-3.16613290583942));
#63939=CARTESIAN_POINT('Ctrl Pts',(-7.00000087640238,-15.2320476408173,
8.76427051435137E-7));
#63940=CARTESIAN_POINT('Ctrl Pts',(-7.00000087640223,-14.5427411838667,
3.16613457937076));
#63941=CARTESIAN_POINT('Origin',(7.,0.,0.));
#63942=CARTESIAN_POINT('Origin',(-7.,0.,0.));
#63943=CARTESIAN_POINT('Ctrl Pts',(7.00000122676011,-12.5220654507218,8.0444765366914));
#63944=CARTESIAN_POINT('Ctrl Pts',(7.00000122674705,-10.770694459262,10.7706678660607));
#63945=CARTESIAN_POINT('Ctrl Pts',(7.00000122675059,-8.04450745410184,12.522045588584));
#63946=CARTESIAN_POINT('Ctrl Pts',(-4.2404238558542E-7,-14.4500036018478,
9.28303045429202));
#63947=CARTESIAN_POINT('Ctrl Pts',(-4.24057452036573E-7,-12.4289858045474,
12.4289551169526));
#63948=CARTESIAN_POINT('Ctrl Pts',(-4.24053364237652E-7,-9.28306613186535,
14.4499806816531));
#63949=CARTESIAN_POINT('Ctrl Pts',(-7.00000199275941,-12.5220652397833,
8.04447640111238));
#63950=CARTESIAN_POINT('Ctrl Pts',(-7.00000199277246,-10.7706942778114,
10.7706676845808));
#63951=CARTESIAN_POINT('Ctrl Pts',(-7.00000199276892,-8.04450731855204,
12.5220453776161));
#63952=CARTESIAN_POINT('Origin',(7.,0.,0.));
#63953=CARTESIAN_POINT('Origin',(-7.,0.,0.));
#63954=CARTESIAN_POINT('Ctrl Pts',(7.00000059287425,-3.16610548810897,14.5427476123492));
#63955=CARTESIAN_POINT('Ctrl Pts',(7.00000059287546,1.45624626939507E-5,
15.2320444588135));
#63956=CARTESIAN_POINT('Ctrl Pts',(7.00000059287604,3.16613329503596,14.5427415584669));
#63957=CARTESIAN_POINT('Ctrl Pts',(-6.39446721752374E-8,-3.65356931914349,
16.7817960242083));
#63958=CARTESIAN_POINT('Ctrl Pts',(-6.39432701116918E-8,1.68045488070068E-5,
17.5772192403596));
#63959=CARTESIAN_POINT('Ctrl Pts',(-6.39426012170821E-8,3.65360140731941,
16.7817890382507));
#63960=CARTESIAN_POINT('Ctrl Pts',(-7.00000070838506,-3.16610548005986,
14.5427475754022));
#63961=CARTESIAN_POINT('Ctrl Pts',(-7.00000070838384,1.45624666247567E-5,
15.232044420115));
#63962=CARTESIAN_POINT('Ctrl Pts',(-7.00000070838326,3.16613328699471,14.5427415215199));
#63963=CARTESIAN_POINT('Origin',(7.,0.,0.));
#63964=CARTESIAN_POINT('Origin',(-7.,0.,0.));
#63965=CARTESIAN_POINT('Origin',(-8.3,0.,0.));
#63966=CARTESIAN_POINT('',(-8.3,-16.1678918187026,-6.69696006698037));
#63967=CARTESIAN_POINT('Origin',(-8.3,-18.0156508836972,-7.46232693177812));
#63968=CARTESIAN_POINT('Origin',(-7.,-18.0156508836972,-7.46232693177812));
#63969=CARTESIAN_POINT('',(-7.,-16.1678918187026,-6.69696006698037));
#63970=CARTESIAN_POINT('Origin',(-7.,-18.0156508836972,-7.46232693177812));
#63971=CARTESIAN_POINT('',(-7.,-16.1678918187026,-6.69696006698036));
#63972=CARTESIAN_POINT('Origin',(-8.3,0.,0.));
#63973=CARTESIAN_POINT('',(-8.3,6.69696006698037,-16.1678918187026));
#63974=CARTESIAN_POINT('Origin',(-8.3,7.46232693177812,-18.0156508836972));
#63975=CARTESIAN_POINT('Origin',(-7.,7.46232693177812,-18.0156508836972));
#63976=CARTESIAN_POINT('',(-7.,6.69696006698037,-16.1678918187026));
#63977=CARTESIAN_POINT('Origin',(-7.,7.46232693177812,-18.0156508836972));
#63978=CARTESIAN_POINT('',(-7.,6.69696006698036,-16.1678918187026));
#63979=CARTESIAN_POINT('Origin',(-8.3,0.,0.));
#63980=CARTESIAN_POINT('',(-8.3,16.1678918187026,6.69696006698037));
#63981=CARTESIAN_POINT('Origin',(-8.3,18.0156508836972,7.46232693177812));
#63982=CARTESIAN_POINT('Origin',(-7.,18.0156508836972,7.46232693177812));
#63983=CARTESIAN_POINT('',(-7.,16.1678918187026,6.69696006698037));
#63984=CARTESIAN_POINT('Origin',(-7.,18.0156508836972,7.46232693177812));
#63985=CARTESIAN_POINT('',(-7.,16.1678918187026,6.69696006698036));
#63986=CARTESIAN_POINT('Origin',(-7.,0.,0.));
#63987=CARTESIAN_POINT('',(-7.,-5.16622633738485,12.4723736887134));
#63988=CARTESIAN_POINT('Origin',(-7.,0.,0.));
#63989=CARTESIAN_POINT('Origin',(-7.7,0.,0.));
#63990=CARTESIAN_POINT('',(7.,-5.16622633738485,12.4723736887134));
#63991=CARTESIAN_POINT('Origin',(7.,0.,0.));
#63992=CARTESIAN_POINT('',(-7.7,-5.16622633738485,12.4723736887134));
#63993=CARTESIAN_POINT('Origin',(8.3,0.,0.));
#63994=CARTESIAN_POINT('',(8.3,-6.69696006579904,-16.1678918191954));
#63995=CARTESIAN_POINT('Origin',(8.3,-7.46232693046164,-18.015650884246));
#63996=CARTESIAN_POINT('Origin',(8.3,-7.46232693046164,-18.015650884246));
#63997=CARTESIAN_POINT('',(7.,-6.69696006579904,-16.1678918191954));
#63998=CARTESIAN_POINT('',(8.3,-6.69696006579904,-16.1678918191954));
#63999=CARTESIAN_POINT('Origin',(7.,-7.46232693046164,-18.015650884246));
#64000=CARTESIAN_POINT('Origin',(8.3,0.,0.));
#64001=CARTESIAN_POINT('',(8.3,16.1678918191954,-6.69696006579904));
#64002=CARTESIAN_POINT('Origin',(8.3,18.015650884246,-7.46232693046164));
#64003=CARTESIAN_POINT('Origin',(8.3,18.015650884246,-7.46232693046164));
#64004=CARTESIAN_POINT('',(7.,16.1678918191954,-6.69696006579904));
#64005=CARTESIAN_POINT('',(8.3,16.1678918191954,-6.69696006579904));
#64006=CARTESIAN_POINT('Origin',(7.,18.015650884246,-7.46232693046164));
#64007=CARTESIAN_POINT('Origin',(8.3,0.,0.));
#64008=CARTESIAN_POINT('',(8.3,6.69696006579904,16.1678918191954));
#64009=CARTESIAN_POINT('Origin',(8.3,7.46232693046164,18.015650884246));
#64010=CARTESIAN_POINT('Origin',(8.3,7.46232693046164,18.015650884246));
#64011=CARTESIAN_POINT('',(7.,6.69696006579904,16.1678918191954));
#64012=CARTESIAN_POINT('',(8.3,6.69696006579904,16.1678918191954));
#64013=CARTESIAN_POINT('Origin',(7.,7.46232693046164,18.015650884246));
#64014=CARTESIAN_POINT('Origin',(7.,0.,0.));
#66666=UNCERTAINTY_MEASURE_WITH_UNIT(LENGTH_MEASURE(0.01),#66722,
'DISTANCE_ACCURACY_VALUE',
'Maximum model space distance between geometric entities at asserted c
onnectivities');
#66680=UNCERTAINTY_MEASURE_WITH_UNIT(LENGTH_MEASURE(0.01),#66722,
'DISTANCE_ACCURACY_VALUE',
'Maximum model space distance between geometric entities at asserted c
onnectivities');
#66707=(
GEOMETRIC_REPRESENTATION_CONTEXT(3)
GLOBAL_UNCERTAINTY_ASSIGNED_CONTEXT((#66666))
GLOBAL_UNIT_ASSIGNED_CONTEXT((#66722,#66724,#66725))
REPRESENTATION_CONTEXT('','3D')
);
#66721=(
GEOMETRIC_REPRESENTATION_CONTEXT(3)
GLOBAL_UNCERTAINTY_ASSIGNED_CONTEXT((#66680))
GLOBAL_UNIT_ASSIGNED_CONTEXT((#66722,#66724,#66725))
REPRESENTATION_CONTEXT('','3D')
);
#66722=(
LENGTH_UNIT()
NAMED_UNIT(*)
SI_UNIT(.MILLI.,.METRE.)
);
#66724=(
NAMED_UNIT(*)
PLANE_ANGLE_UNIT()
SI_UNIT($,.RADIAN.)
);
#66725=(
NAMED_UNIT(*)
SI_UNIT($,.STERADIAN.)
SOLID_ANGLE_UNIT()
);
#66752=SHAPE_DEFINITION_REPRESENTATION(#66812,#66916);
#66812=PRODUCT_DEFINITION_SHAPE('',$,#66957);
#66916=SHAPE_REPRESENTATION('',(#27714),#66707);
#66930=PRODUCT_DEFINITION_CONTEXT('part definition',#67052,'design');
#66957=PRODUCT_DEFINITION('Coupling Spider','Coupling Spider',#66997,#66930);
#66997=PRODUCT_DEFINITION_FORMATION('',$,#67080);
#67052=APPLICATION_CONTEXT(
'Core Data for Automotive Mechanical Design Process');
#67053=PRODUCT_CONTEXT('part definition',#67052,'mechanical');
#67080=PRODUCT('Coupling Spider','Coupling Spider',$,(#67053));
#67095=PRESENTATION_STYLE_ASSIGNMENT((#67097));
#67097=SURFACE_STYLE_USAGE(.BOTH.,#67099);
#67099=SURFACE_SIDE_STYLE('',(#67101));
#67101=SURFACE_STYLE_FILL_AREA(#67103);
#67103=FILL_AREA_STYLE('Opaque(202,209,238)',(#67105));
#67105=FILL_AREA_STYLE_COLOUR('Opaque(202,209,238)',#67107);
#67107=COLOUR_RGB('Opaque(202,209,238)',0.792156862745098,0.819607843137255,
0.933333333333333);
ENDSEC;
END-ISO-10303-21;
